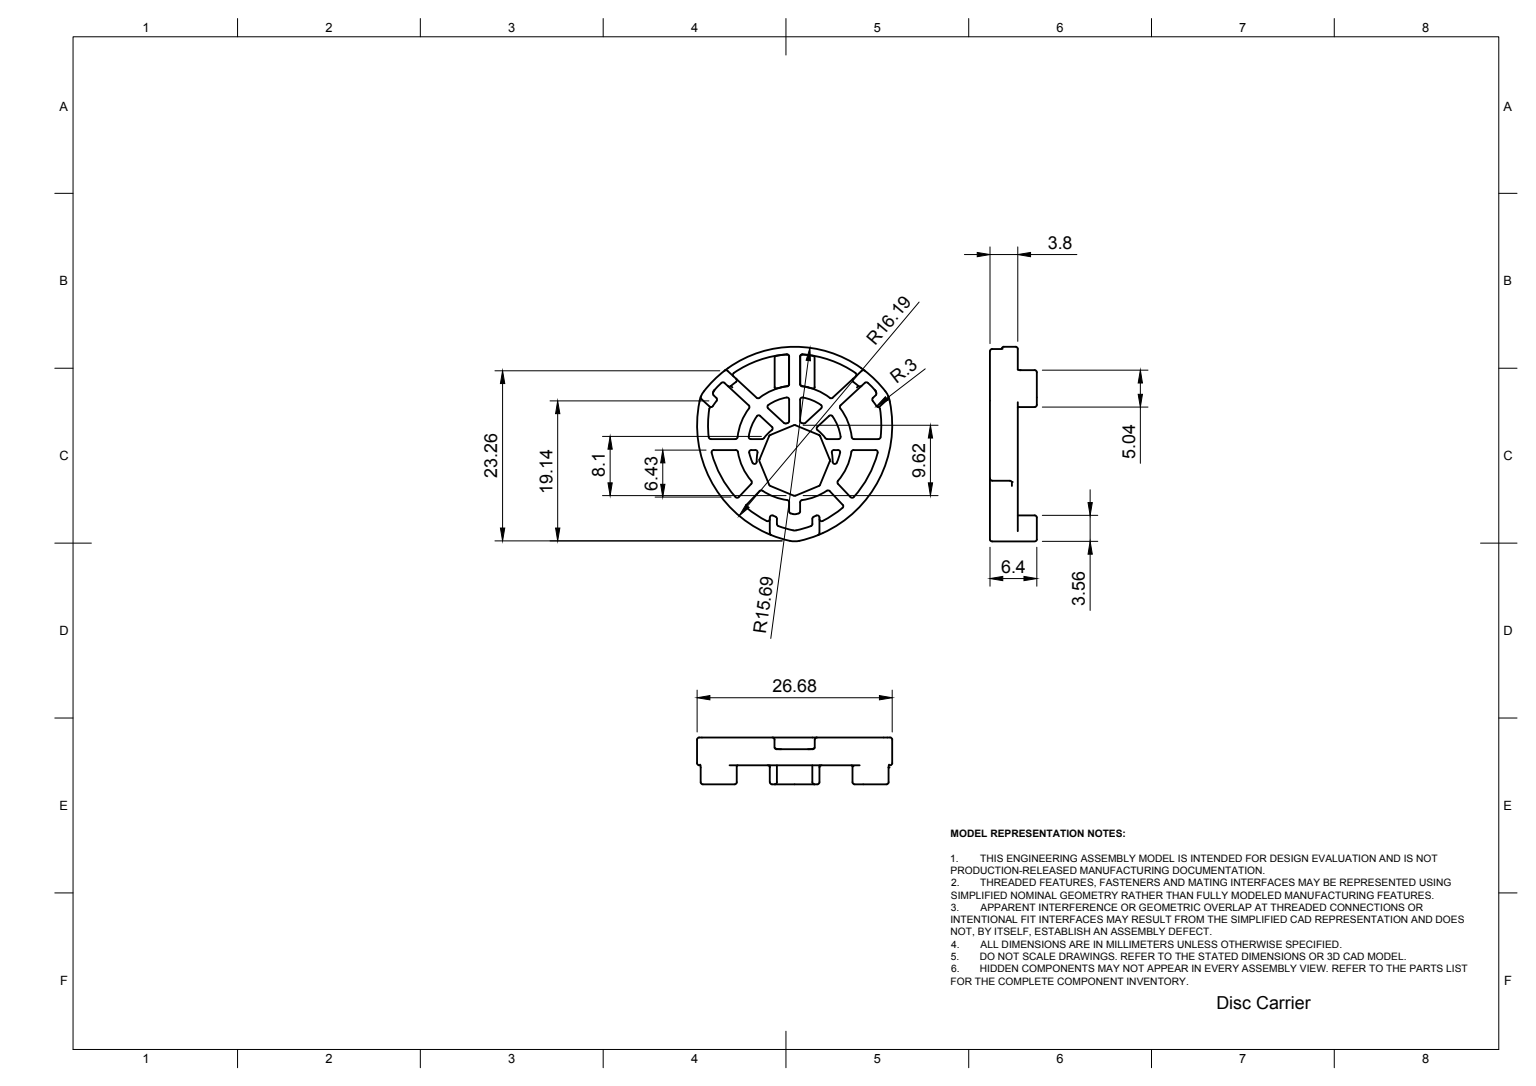
ISO-10303-21;
HEADER;
/* Generated by software containing ST-Developer
 * from STEP Tools, Inc. (www.steptools.com) 
 */

FILE_DESCRIPTION(
/* description */ ('STEP AP214'),
/* implementation_level */ '2;1');

FILE_NAME(
/* name */ 'Disc Carrier.step',
/* time_stamp */ '2026-10-06T00:19:40-07:00',
/* author */ (''),
/* organization */ (''),
/* preprocessor_version */ 'ST-DEVELOPER v20.2',
/* originating_system */ 'Autodesk Translation Framework v15.15.0.0',
/* authorisation */ '');

FILE_SCHEMA (('AUTOMOTIVE_DESIGN { 1 0 10303 214 3 1 1 }'));
ENDSEC;

DATA;
#10=MECHANICAL_DESIGN_GEOMETRIC_PRESENTATION_REPRESENTATION('',(#2070),#98302);
#217=TOROIDAL_SURFACE('',#36633,13.816744254,0.3);
#218=TOROIDAL_SURFACE('',#36640,0.6,0.3);
#219=TOROIDAL_SURFACE('',#36644,14.9875296363,0.3);
#220=TOROIDAL_SURFACE('',#36648,0.6,0.3);
#221=TOROIDAL_SURFACE('',#36651,14.9875296363,0.3);
#222=TOROIDAL_SURFACE('',#36655,0.6,0.3);
#223=TOROIDAL_SURFACE('',#36662,13.816744254,0.3);
#224=TOROIDAL_SURFACE('',#36692,13.9462109523,0.3);
#225=TOROIDAL_SURFACE('',#36699,0.6,0.3);
#226=TOROIDAL_SURFACE('',#36702,14.9875296363,0.3);
#227=TOROIDAL_SURFACE('',#36707,15.8875296363,0.3);
#228=TOROIDAL_SURFACE('',#36711,8.14541841273,0.3);
#229=TOROIDAL_SURFACE('',#36717,14.3875296363,0.3);
#230=TOROIDAL_SURFACE('',#36742,7.54541841273,0.3);
#231=TOROIDAL_SURFACE('',#36753,14.9875296363,0.3);
#232=TOROIDAL_SURFACE('',#36757,0.6,0.3);
#233=TOROIDAL_SURFACE('',#36763,0.6,0.3);
#234=TOROIDAL_SURFACE('',#36765,0.6,0.3);
#235=TOROIDAL_SURFACE('',#36767,0.6,0.3);
#236=TOROIDAL_SURFACE('',#36769,12.2256279976,0.3);
#237=TOROIDAL_SURFACE('',#36775,14.9875296363,0.3);
#238=TOROIDAL_SURFACE('',#36803,15.3875296363,0.3);
#239=TOROIDAL_SURFACE('',#36831,4.89295371933,0.3);
#240=TOROIDAL_SURFACE('',#36836,0.6,0.3);
#241=TOROIDAL_SURFACE('',#36842,0.6,0.3);
#242=TOROIDAL_SURFACE('',#36846,6.64541841273,0.3);
#243=TOROIDAL_SURFACE('',#36850,0.6,0.3);
#244=TOROIDAL_SURFACE('',#36854,0.6,0.3);
#245=TOROIDAL_SURFACE('',#36859,6.64541841273,0.3);
#246=TOROIDAL_SURFACE('',#36866,0.6,0.3);
#247=TOROIDAL_SURFACE('',#36875,4.89295371933,0.3);
#248=TOROIDAL_SURFACE('',#36879,0.6,0.3);
#249=TOROIDAL_SURFACE('',#36883,0.6,0.3);
#250=TOROIDAL_SURFACE('',#36894,4.89295371933,0.3);
#251=TOROIDAL_SURFACE('',#36900,0.6,0.3);
#252=TOROIDAL_SURFACE('',#36906,0.6,0.3);
#253=TOROIDAL_SURFACE('',#36910,6.64541841273,0.3);
#254=TOROIDAL_SURFACE('',#36914,0.6,0.3);
#255=TOROIDAL_SURFACE('',#36918,0.6,0.3);
#256=TOROIDAL_SURFACE('',#36926,6.04541841273,0.3);
#257=TOROIDAL_SURFACE('',#36933,5.49295371933,0.3);
#258=TOROIDAL_SURFACE('',#36946,5.49295371933,0.3);
#259=TOROIDAL_SURFACE('',#36950,0.6,0.3);
#260=TOROIDAL_SURFACE('',#36954,7.54541841273,0.3);
#261=TOROIDAL_SURFACE('',#36958,0.6,0.3);
#262=TOROIDAL_SURFACE('',#36962,0.6,0.3);
#263=TOROIDAL_SURFACE('',#36973,12.8256279976,0.3);
#264=TOROIDAL_SURFACE('',#36978,5.49295371933,0.3);
#265=TOROIDAL_SURFACE('',#36984,15.8875296363,0.3);
#266=TOROIDAL_SURFACE('',#36988,15.3875296363,0.3);
#267=TOROIDAL_SURFACE('',#36993,15.8875296363,0.3);
#268=TOROIDAL_SURFACE('',#36996,0.985778366608,0.3);
#269=TOROIDAL_SURFACE('',#37005,2.7,0.3);
#270=TOROIDAL_SURFACE('',#37007,2.7,0.3);
#271=TOROIDAL_SURFACE('',#37013,15.8875296363,0.3);
#272=TOROIDAL_SURFACE('',#37039,8.14541841273,0.3);
#273=TOROIDAL_SURFACE('',#37053,14.3875296363,0.3);
#274=TOROIDAL_SURFACE('',#37091,6.04541841273,0.3);
#275=TOROIDAL_SURFACE('',#37112,6.04541841273,0.3);
#276=TOROIDAL_SURFACE('',#37118,0.385778366608,0.3);
#277=TOROIDAL_SURFACE('',#37119,0.6,0.3);
#278=TOROIDAL_SURFACE('',#37129,8.14541841273,0.3);
#279=TOROIDAL_SURFACE('',#37134,0.6,0.3);
#280=TOROIDAL_SURFACE('',#37137,13.3462109523,0.3);
#281=TOROIDAL_SURFACE('',#37140,0.6,0.3);
#282=TOROIDAL_SURFACE('',#37149,14.3875296363,0.3);
#283=TOROIDAL_SURFACE('',#37154,14.3875296363,0.3);
#284=TOROIDAL_SURFACE('',#37170,0.6,0.3);
#285=TOROIDAL_SURFACE('',#37173,7.54541841273,0.3);
#286=TOROIDAL_SURFACE('',#37176,0.6,0.3);
#287=TOROIDAL_SURFACE('',#37182,0.6,0.3);
#288=TOROIDAL_SURFACE('',#37185,0.6,0.3);
#289=TOROIDAL_SURFACE('',#37188,14.9875296363,0.3);
#290=TOROIDAL_SURFACE('',#37190,0.6,0.3);
#291=TOROIDAL_SURFACE('',#37193,13.216744254,0.3);
#292=TOROIDAL_SURFACE('',#37205,15.8875296363,0.3);
#293=TOROIDAL_SURFACE('',#37207,1.3,0.3);
#294=TOROIDAL_SURFACE('',#37211,14.9875296363,0.3);
#295=TOROIDAL_SURFACE('',#37215,0.6,0.3);
#296=TOROIDAL_SURFACE('',#37221,0.6,0.3);
#297=TOROIDAL_SURFACE('',#37225,7.54541841273,0.3);
#298=TOROIDAL_SURFACE('',#37229,0.6,0.3);
#299=TOROIDAL_SURFACE('',#37261,14.3875296363,0.3);
#300=TOROIDAL_SURFACE('',#37264,0.7,0.3);
#301=TOROIDAL_SURFACE('',#37270,14.3875296363,0.3);
#302=TOROIDAL_SURFACE('',#37275,14.3875296363,0.3);
#303=TOROIDAL_SURFACE('',#37282,8.14541841273,0.3);
#304=TOROIDAL_SURFACE('',#37289,0.6,0.3);
#305=TOROIDAL_SURFACE('',#37292,13.216744254,0.3);
#306=TOROIDAL_SURFACE('',#37295,0.6,0.3);
#307=TOROIDAL_SURFACE('',#37328,13.816744254,0.3);
#308=TOROIDAL_SURFACE('',#37335,0.6,0.3);
#309=TOROIDAL_SURFACE('',#37339,14.9875296363,0.3);
#310=TOROIDAL_SURFACE('',#37343,0.6,0.3);
#311=TOROIDAL_SURFACE('',#37346,14.9875296363,0.3);
#312=TOROIDAL_SURFACE('',#37350,0.6,0.3);
#313=TOROIDAL_SURFACE('',#37357,13.816744254,0.3);
#314=TOROIDAL_SURFACE('',#37389,13.9462109523,0.3);
#315=TOROIDAL_SURFACE('',#37396,0.6,0.3);
#316=TOROIDAL_SURFACE('',#37400,14.9875296363,0.3);
#317=TOROIDAL_SURFACE('',#37406,15.8875296363,0.3);
#318=TOROIDAL_SURFACE('',#37412,8.14541841273,0.3);
#319=TOROIDAL_SURFACE('',#37417,14.3875296363,0.3);
#320=TOROIDAL_SURFACE('',#37442,7.54541841273,0.3);
#321=TOROIDAL_SURFACE('',#37453,14.9875296363,0.3);
#322=TOROIDAL_SURFACE('',#37457,0.6,0.3);
#323=TOROIDAL_SURFACE('',#37463,0.6,0.3);
#324=TOROIDAL_SURFACE('',#37465,0.6,0.3);
#325=TOROIDAL_SURFACE('',#37467,0.6,0.3);
#326=TOROIDAL_SURFACE('',#37470,12.2256279976,0.3);
#327=TOROIDAL_SURFACE('',#37476,14.9875296363,0.3);
#328=TOROIDAL_SURFACE('',#37511,15.3875296363,0.3);
#329=TOROIDAL_SURFACE('',#37543,4.89295371933,0.3);
#330=TOROIDAL_SURFACE('',#37548,0.6,0.3);
#331=TOROIDAL_SURFACE('',#37554,0.6,0.3);
#332=TOROIDAL_SURFACE('',#37558,6.64541841273,0.3);
#333=TOROIDAL_SURFACE('',#37562,0.6,0.3);
#334=TOROIDAL_SURFACE('',#37566,0.6,0.3);
#335=TOROIDAL_SURFACE('',#37571,6.64541841273,0.3);
#336=TOROIDAL_SURFACE('',#37578,0.6,0.3);
#337=TOROIDAL_SURFACE('',#37586,4.89295371933,0.3);
#338=TOROIDAL_SURFACE('',#37590,0.6,0.3);
#339=TOROIDAL_SURFACE('',#37594,0.6,0.3);
#340=TOROIDAL_SURFACE('',#37605,4.89295371933,0.3);
#341=TOROIDAL_SURFACE('',#37611,0.6,0.3);
#342=TOROIDAL_SURFACE('',#37617,0.6,0.3);
#343=TOROIDAL_SURFACE('',#37621,6.64541841273,0.3);
#344=TOROIDAL_SURFACE('',#37625,0.6,0.3);
#345=TOROIDAL_SURFACE('',#37629,0.6,0.3);
#346=TOROIDAL_SURFACE('',#37637,6.04541841273,0.3);
#347=TOROIDAL_SURFACE('',#37643,5.49295371933,0.3);
#348=TOROIDAL_SURFACE('',#37656,5.49295371933,0.3);
#349=TOROIDAL_SURFACE('',#37659,0.6,0.3);
#350=TOROIDAL_SURFACE('',#37663,7.54541841273,0.3);
#351=TOROIDAL_SURFACE('',#37667,0.6,0.3);
#352=TOROIDAL_SURFACE('',#37671,0.6,0.3);
#353=TOROIDAL_SURFACE('',#37684,12.8256279976,0.3);
#354=TOROIDAL_SURFACE('',#37689,5.49295371933,0.3);
#355=TOROIDAL_SURFACE('',#37696,15.8875296363,0.3);
#356=TOROIDAL_SURFACE('',#37700,15.3875296363,0.3);
#357=TOROIDAL_SURFACE('',#37710,0.4,0.1);
#358=TOROIDAL_SURFACE('',#37715,0.4,0.1);
#359=TOROIDAL_SURFACE('',#37720,0.4,0.1);
#360=TOROIDAL_SURFACE('',#37722,0.4,0.1);
#361=TOROIDAL_SURFACE('',#37727,0.4,0.1);
#362=TOROIDAL_SURFACE('',#37732,0.4,0.1);
#363=TOROIDAL_SURFACE('',#37737,0.4,0.1);
#364=TOROIDAL_SURFACE('',#37742,0.4,0.1);
#365=TOROIDAL_SURFACE('',#37749,15.8875296363,0.3);
#366=TOROIDAL_SURFACE('',#37750,0.985778366608,0.3);
#367=TOROIDAL_SURFACE('',#37759,2.7,0.3);
#368=TOROIDAL_SURFACE('',#37761,2.7,0.3);
#369=TOROIDAL_SURFACE('',#37766,15.8875296363,0.3);
#370=TOROIDAL_SURFACE('',#37779,15.3875296363,0.3);
#371=TOROIDAL_SURFACE('',#37803,8.14541841273,0.3);
#372=TOROIDAL_SURFACE('',#37814,14.3875296363,0.3);
#373=TOROIDAL_SURFACE('',#37850,6.04541841273,0.3);
#374=TOROIDAL_SURFACE('',#37871,6.04541841273,0.3);
#375=TOROIDAL_SURFACE('',#37877,0.385778366608,0.3);
#376=TOROIDAL_SURFACE('',#37878,0.6,0.3);
#377=TOROIDAL_SURFACE('',#37886,8.14541841273,0.3);
#378=TOROIDAL_SURFACE('',#37891,0.6,0.3);
#379=TOROIDAL_SURFACE('',#37894,13.3462109523,0.3);
#380=TOROIDAL_SURFACE('',#37897,0.6,0.3);
#381=TOROIDAL_SURFACE('',#37909,14.3875296363,0.3);
#382=TOROIDAL_SURFACE('',#37914,14.3875296363,0.3);
#383=TOROIDAL_SURFACE('',#37930,0.6,0.3);
#384=TOROIDAL_SURFACE('',#37933,7.54541841273,0.3);
#385=TOROIDAL_SURFACE('',#37936,0.6,0.3);
#386=TOROIDAL_SURFACE('',#37942,0.6,0.3);
#387=TOROIDAL_SURFACE('',#37945,0.6,0.3);
#388=TOROIDAL_SURFACE('',#37948,14.9875296363,0.3);
#389=TOROIDAL_SURFACE('',#37950,0.6,0.3);
#390=TOROIDAL_SURFACE('',#37953,13.216744254,0.3);
#391=TOROIDAL_SURFACE('',#37965,15.8875296363,0.3);
#392=TOROIDAL_SURFACE('',#37967,15.3875296363,0.3);
#393=TOROIDAL_SURFACE('',#37977,0.4,0.1);
#394=TOROIDAL_SURFACE('',#37979,0.4,0.1);
#395=TOROIDAL_SURFACE('',#37984,0.4,0.1);
#396=TOROIDAL_SURFACE('',#37991,0.4,0.1);
#397=TOROIDAL_SURFACE('',#37999,1.3,0.3);
#398=TOROIDAL_SURFACE('',#38003,14.9875296363,0.3);
#399=TOROIDAL_SURFACE('',#38006,0.6,0.3);
#400=TOROIDAL_SURFACE('',#38011,0.6,0.3);
#401=TOROIDAL_SURFACE('',#38014,7.54541841273,0.3);
#402=TOROIDAL_SURFACE('',#38017,0.6,0.3);
#403=TOROIDAL_SURFACE('',#38048,14.3875296363,0.3);
#404=TOROIDAL_SURFACE('',#38051,0.7,0.3);
#405=TOROIDAL_SURFACE('',#38057,14.3875296363,0.3);
#406=TOROIDAL_SURFACE('',#38062,14.3875296363,0.3);
#407=TOROIDAL_SURFACE('',#38071,8.14541841273,0.3);
#408=TOROIDAL_SURFACE('',#38079,0.6,0.3);
#409=TOROIDAL_SURFACE('',#38082,13.216744254,0.3);
#410=TOROIDAL_SURFACE('',#38085,0.6,0.3);
#636=ELLIPSE('',#36609,0.616948377444998,0.596990574629877);
#637=ELLIPSE('',#36774,0.298848892782947,0.2969053606671);
#638=ELLIPSE('',#36784,0.723457342561266,0.612142527579512);
#639=ELLIPSE('',#36787,0.839901750727128,0.325201544662394);
#640=ELLIPSE('',#36791,0.839902765005034,0.32520200920329);
#641=ELLIPSE('',#36792,0.855720879944736,0.334538055133644);
#642=ELLIPSE('',#36796,0.978504400650312,0.43206650732588);
#643=ELLIPSE('',#36807,0.298987522088764,0.297463090341305);
#644=ELLIPSE('',#36864,0.0996163073938246,0.0989684771695573);
#645=ELLIPSE('',#36865,0.0996064607576122,0.098921046723739);
#646=ELLIPSE('',#36870,0.0996019636355457,0.0988979538729398);
#647=ELLIPSE('',#36871,0.83480328877623,0.449020774204173);
#648=ELLIPSE('',#36872,0.0996163010870433,0.0989684579736212);
#649=ELLIPSE('',#36873,0.0996019611035896,0.0988979479073979);
#650=ELLIPSE('',#36874,0.95881614661924,0.545128833125042);
#651=ELLIPSE('',#36888,0.0996019636635876,0.0988979539393061);
#652=ELLIPSE('',#36889,0.834793007766825,0.449012007377356);
#653=ELLIPSE('',#36890,0.0996163011297496,0.0989684580705834);
#654=ELLIPSE('',#36891,0.0996019612880109,0.0988979483606112);
#655=ELLIPSE('',#36892,0.0996163073978892,0.0989684771734698);
#656=ELLIPSE('',#36893,0.842981617008318,0.456043592675208);
#657=ELLIPSE('',#37011,0.298848927783278,0.296905444507015);
#658=ELLIPSE('',#37012,0.299091836143122,0.297812318683333);
#659=ELLIPSE('',#37015,0.299092017159912,0.297812365396506);
#660=ELLIPSE('',#37030,0.298848921977966,0.296905430756493);
#661=ELLIPSE('',#37033,0.358196202460482,0.312309449719818);
#662=ELLIPSE('',#37114,0.299085253265536,0.297791465794382);
#663=ELLIPSE('',#37167,0.298848922572082,0.296905433095193);
#664=ELLIPSE('',#37196,0.48575646188926,0.315209432805966);
#665=ELLIPSE('',#37197,0.298848922223572,0.296905431591445);
#666=ELLIPSE('',#37198,0.298976384440305,0.297423661821599);
#667=ELLIPSE('',#37201,0.298848893179516,0.296905361743558);
#668=ELLIPSE('',#37203,0.298849004322787,0.296905465668005);
#669=ELLIPSE('',#37209,0.299077289129448,0.297765861381808);
#670=ELLIPSE('',#37233,0.2988599234424,0.296955631862372);
#671=ELLIPSE('',#37234,0.311781310291398,0.301461130998388);
#672=ELLIPSE('',#37302,0.616948377444998,0.596990574629877);
#673=ELLIPSE('',#37475,0.298848921980292,0.296905430856554);
#674=ELLIPSE('',#37488,0.723457342561266,0.612142527579512);
#675=ELLIPSE('',#37496,0.855721443648946,0.334538377478706);
#676=ELLIPSE('',#37500,0.839900853126743,0.325201217495182);
#677=ELLIPSE('',#37501,0.855721622372424,0.334538483108095);
#678=ELLIPSE('',#37576,0.0996064588793403,0.0989210426276871);
#679=ELLIPSE('',#37577,0.0996163153029603,0.0989684770999027);
#680=ELLIPSE('',#37582,0.0996163073887366,0.0989684771505584);
#681=ELLIPSE('',#37583,0.842986353714893,0.456047441690848);
#682=ELLIPSE('',#37584,0.0996019612459525,0.0988979482541347);
#683=ELLIPSE('',#37585,0.0996019632515573,0.0988979536268878);
#684=ELLIPSE('',#37599,0.0996163073858426,0.0989684771452112);
#685=ELLIPSE('',#37600,0.84298514231536,0.456046449061635);
#686=ELLIPSE('',#37601,0.0996019612550026,0.0988979482814453);
#687=ELLIPSE('',#37602,0.0996019632510724,0.0988979536158697);
#688=ELLIPSE('',#37603,0.83479393416711,0.449012748427101);
#689=ELLIPSE('',#37604,0.0996163011297535,0.0989684580706061);
#690=ELLIPSE('',#37764,0.299091892234915,0.297812430528943);
#691=ELLIPSE('',#37765,0.298848892822638,0.296905360819338);
#692=ELLIPSE('',#37767,0.298848925852848,0.296905440053724);
#693=ELLIPSE('',#37768,0.299092010660396,0.29781235080905);
#694=ELLIPSE('',#37796,0.358196201537078,0.312309449169694);
#695=ELLIPSE('',#37927,0.298848900003069,0.29690537960284);
#696=ELLIPSE('',#37955,0.298848922307858,0.296905431614744);
#697=ELLIPSE('',#37956,0.298976199239788,0.29742370304314);
#698=ELLIPSE('',#37957,0.298848893194714,0.296905361846251);
#699=ELLIPSE('',#37958,0.48575646188926,0.315209432805966);
#700=ELLIPSE('',#37960,0.298848918312141,0.296905422207127);
#701=ELLIPSE('',#37961,0.298848927446579,0.29690544380809);
#702=ELLIPSE('',#37963,0.298849777080326,0.296906780571315);
#703=ELLIPSE('',#38001,0.299077129594657,0.297765592394515);
#704=ELLIPSE('',#38020,0.311781310291398,0.301461130998388);
#705=ELLIPSE('',#38021,0.2988599234424,0.296955631862372);
#759=SPHERICAL_SURFACE('',#36631,0.3);
#760=SPHERICAL_SURFACE('',#36636,0.3);
#761=SPHERICAL_SURFACE('',#36660,0.3);
#762=SPHERICAL_SURFACE('',#36665,0.3);
#763=SPHERICAL_SURFACE('',#36690,0.3);
#764=SPHERICAL_SURFACE('',#36695,0.3);
#765=SPHERICAL_SURFACE('',#36705,0.3);
#766=SPHERICAL_SURFACE('',#36721,0.3);
#767=SPHERICAL_SURFACE('',#36724,0.3);
#768=SPHERICAL_SURFACE('',#36728,0.3);
#769=SPHERICAL_SURFACE('',#36731,0.3);
#770=SPHERICAL_SURFACE('',#36759,0.3);
#771=SPHERICAL_SURFACE('',#36800,0.3);
#772=SPHERICAL_SURFACE('',#36930,0.3);
#773=SPHERICAL_SURFACE('',#36936,0.3);
#774=SPHERICAL_SURFACE('',#36939,0.3);
#775=SPHERICAL_SURFACE('',#36942,0.3);
#776=SPHERICAL_SURFACE('',#36966,0.3);
#777=SPHERICAL_SURFACE('',#36971,0.3);
#778=SPHERICAL_SURFACE('',#37003,0.3);
#779=SPHERICAL_SURFACE('',#37016,0.3);
#780=SPHERICAL_SURFACE('',#37021,0.3);
#781=SPHERICAL_SURFACE('',#37037,0.3);
#782=SPHERICAL_SURFACE('',#37043,0.3);
#783=SPHERICAL_SURFACE('',#37048,0.3);
#784=SPHERICAL_SURFACE('',#37050,0.3);
#785=SPHERICAL_SURFACE('',#37057,0.3);
#786=SPHERICAL_SURFACE('',#37089,0.3);
#787=SPHERICAL_SURFACE('',#37093,0.3);
#788=SPHERICAL_SURFACE('',#37095,0.3);
#789=SPHERICAL_SURFACE('',#37100,0.3);
#790=SPHERICAL_SURFACE('',#37101,0.3);
#791=SPHERICAL_SURFACE('',#37110,0.3);
#792=SPHERICAL_SURFACE('',#37117,0.3);
#793=SPHERICAL_SURFACE('',#37122,0.3);
#794=SPHERICAL_SURFACE('',#37145,0.3);
#795=SPHERICAL_SURFACE('',#37152,0.3);
#796=SPHERICAL_SURFACE('',#37162,0.3);
#797=SPHERICAL_SURFACE('',#37258,0.3);
#798=SPHERICAL_SURFACE('',#37267,0.3);
#799=SPHERICAL_SURFACE('',#37272,0.3);
#800=SPHERICAL_SURFACE('',#37277,0.3);
#801=SPHERICAL_SURFACE('',#37280,0.3);
#802=SPHERICAL_SURFACE('',#37284,0.3);
#803=SPHERICAL_SURFACE('',#37326,0.3);
#804=SPHERICAL_SURFACE('',#37331,0.3);
#805=SPHERICAL_SURFACE('',#37355,0.3);
#806=SPHERICAL_SURFACE('',#37360,0.3);
#807=SPHERICAL_SURFACE('',#37387,0.3);
#808=SPHERICAL_SURFACE('',#37392,0.3);
#809=SPHERICAL_SURFACE('',#37403,0.3);
#810=SPHERICAL_SURFACE('',#37421,0.3);
#811=SPHERICAL_SURFACE('',#37424,0.3);
#812=SPHERICAL_SURFACE('',#37428,0.3);
#813=SPHERICAL_SURFACE('',#37431,0.3);
#814=SPHERICAL_SURFACE('',#37459,0.3);
#815=SPHERICAL_SURFACE('',#37508,0.3);
#816=SPHERICAL_SURFACE('',#37640,0.3);
#817=SPHERICAL_SURFACE('',#37646,0.3);
#818=SPHERICAL_SURFACE('',#37649,0.3);
#819=SPHERICAL_SURFACE('',#37652,0.3);
#820=SPHERICAL_SURFACE('',#37675,0.3);
#821=SPHERICAL_SURFACE('',#37682,0.3);
#822=SPHERICAL_SURFACE('',#37757,0.3);
#823=SPHERICAL_SURFACE('',#37769,0.3);
#824=SPHERICAL_SURFACE('',#37787,0.3);
#825=SPHERICAL_SURFACE('',#37801,0.3);
#826=SPHERICAL_SURFACE('',#37806,0.3);
#827=SPHERICAL_SURFACE('',#37810,0.3);
#828=SPHERICAL_SURFACE('',#37812,0.3);
#829=SPHERICAL_SURFACE('',#37817,0.3);
#830=SPHERICAL_SURFACE('',#37848,0.3);
#831=SPHERICAL_SURFACE('',#37852,0.3);
#832=SPHERICAL_SURFACE('',#37854,0.3);
#833=SPHERICAL_SURFACE('',#37859,0.3);
#834=SPHERICAL_SURFACE('',#37860,0.3);
#835=SPHERICAL_SURFACE('',#37869,0.3);
#836=SPHERICAL_SURFACE('',#37876,0.3);
#837=SPHERICAL_SURFACE('',#37879,0.3);
#838=SPHERICAL_SURFACE('',#37905,0.3);
#839=SPHERICAL_SURFACE('',#37911,0.3);
#840=SPHERICAL_SURFACE('',#37922,0.3);
#841=SPHERICAL_SURFACE('',#38045,0.3);
#842=SPHERICAL_SURFACE('',#38054,0.3);
#843=SPHERICAL_SURFACE('',#38059,0.3);
#844=SPHERICAL_SURFACE('',#38065,0.3);
#845=SPHERICAL_SURFACE('',#38069,0.3);
#846=SPHERICAL_SURFACE('',#38074,0.3);
#1192=B_SPLINE_SURFACE_WITH_KNOTS('',5,5,((#86287,#86288,#86289,#86290,
#86291,#86292),(#86293,#86294,#86295,#86296,#86297,#86298),(#86299,#86300,
#86301,#86302,#86303,#86304),(#86305,#86306,#86307,#86308,#86309,#86310),
(#86311,#86312,#86313,#86314,#86315,#86316),(#86317,#86318,#86319,#86320,
#86321,#86322),(#86323,#86324,#86325,#86326,#86327,#86328),(#86329,#86330,
#86331,#86332,#86333,#86334),(#86335,#86336,#86337,#86338,#86339,#86340)),
 .UNSPECIFIED.,.F.,.F.,.F.,(6,3,6),(6,6),(1.75158458902,2.2812742412,2.90384942405),
(0.,0.3),.UNSPECIFIED.);
#1193=B_SPLINE_SURFACE_WITH_KNOTS('',5,5,((#86882,#86883,#86884,#86885,
#86886,#86887),(#86888,#86889,#86890,#86891,#86892,#86893),(#86894,#86895,
#86896,#86897,#86898,#86899),(#86900,#86901,#86902,#86903,#86904,#86905),
(#86906,#86907,#86908,#86909,#86910,#86911),(#86912,#86913,#86914,#86915,
#86916,#86917)),.UNSPECIFIED.,.F.,.F.,.F.,(6,6),(6,6),(1.0735101225,1.1089775272),
(0.,0.1),.UNSPECIFIED.);
#1194=B_SPLINE_SURFACE_WITH_KNOTS('',5,5,((#86931,#86932,#86933,#86934,
#86935,#86936),(#86937,#86938,#86939,#86940,#86941,#86942),(#86943,#86944,
#86945,#86946,#86947,#86948),(#86949,#86950,#86951,#86952,#86953,#86954),
(#86955,#86956,#86957,#86958,#86959,#86960),(#86961,#86962,#86963,#86964,
#86965,#86966)),.UNSPECIFIED.,.F.,.F.,.F.,(6,6),(6,6),(1.62703155549,1.68203627825),
(0.,0.1),.UNSPECIFIED.);
#1195=B_SPLINE_SURFACE_WITH_KNOTS('',5,5,((#86972,#86973,#86974,#86975,
#86976,#86977),(#86978,#86979,#86980,#86981,#86982,#86983),(#86984,#86985,
#86986,#86987,#86988,#86989),(#86990,#86991,#86992,#86993,#86994,#86995),
(#86996,#86997,#86998,#86999,#87000,#87001),(#87002,#87003,#87004,#87005,
#87006,#87007)),.UNSPECIFIED.,.F.,.F.,.F.,(6,6),(6,6),(0.205332243373231,
0.603435556801337),(-5.32516463369809E-5,0.1),.UNSPECIFIED.);
#1196=B_SPLINE_SURFACE_WITH_KNOTS('',4,5,((#87038,#87039,#87040,#87041,
#87042,#87043),(#87044,#87045,#87046,#87047,#87048,#87049),(#87050,#87051,
#87052,#87053,#87054,#87055),(#87056,#87057,#87058,#87059,#87060,#87061),
(#87062,#87063,#87064,#87065,#87066,#87067)),.UNSPECIFIED.,.F.,.F.,.F.,
(5,5),(6,6),(2.44731088148,2.46511887948),(0.,0.1),.UNSPECIFIED.);
#1197=B_SPLINE_SURFACE_WITH_KNOTS('',5,5,((#87090,#87091,#87092,#87093,
#87094,#87095),(#87096,#87097,#87098,#87099,#87100,#87101),(#87102,#87103,
#87104,#87105,#87106,#87107),(#87108,#87109,#87110,#87111,#87112,#87113),
(#87114,#87115,#87116,#87117,#87118,#87119),(#87120,#87121,#87122,#87123,
#87124,#87125)),.UNSPECIFIED.,.F.,.F.,.F.,(6,6),(6,6),(1.62703155549,1.68203627825),
(0.,0.1),.UNSPECIFIED.);
#1198=B_SPLINE_SURFACE_WITH_KNOTS('',5,5,((#87131,#87132,#87133,#87134,
#87135,#87136),(#87137,#87138,#87139,#87140,#87141,#87142),(#87143,#87144,
#87145,#87146,#87147,#87148),(#87149,#87150,#87151,#87152,#87153,#87154),
(#87155,#87156,#87157,#87158,#87159,#87160),(#87161,#87162,#87163,#87164,
#87165,#87166)),.UNSPECIFIED.,.F.,.F.,.F.,(6,6),(6,6),(0.205332100976151,
0.60343837439054),(-5.32318455396895E-5,0.1),.UNSPECIFIED.);
#1199=B_SPLINE_SURFACE_WITH_KNOTS('',5,5,((#87197,#87198,#87199,#87200,
#87201,#87202),(#87203,#87204,#87205,#87206,#87207,#87208),(#87209,#87210,
#87211,#87212,#87213,#87214),(#87215,#87216,#87217,#87218,#87219,#87220),
(#87221,#87222,#87223,#87224,#87225,#87226),(#87227,#87228,#87229,#87230,
#87231,#87232)),.UNSPECIFIED.,.F.,.F.,.F.,(6,6),(6,6),(2.44531347319,2.50031756413),
(0.,0.1),.UNSPECIFIED.);
#1200=B_SPLINE_SURFACE_WITH_KNOTS('',5,5,((#88026,#88027,#88028,#88029,
#88030,#88031),(#88032,#88033,#88034,#88035,#88036,#88037),(#88038,#88039,
#88040,#88041,#88042,#88043),(#88044,#88045,#88046,#88047,#88048,#88049),
(#88050,#88051,#88052,#88053,#88054,#88055),(#88056,#88057,#88058,#88059,
#88060,#88061),(#88062,#88063,#88064,#88065,#88066,#88067),(#88068,#88069,
#88070,#88071,#88072,#88073),(#88074,#88075,#88076,#88077,#88078,#88079)),
 .UNSPECIFIED.,.F.,.F.,.F.,(6,3,6),(6,6),(2.86241645295004,3.3764526533,
4.04046842116996),(0.,0.300992369259961),.UNSPECIFIED.);
#1201=B_SPLINE_SURFACE_WITH_KNOTS('',5,5,((#88128,#88129,#88130,#88131,
#88132,#88133),(#88134,#88135,#88136,#88137,#88138,#88139),(#88140,#88141,
#88142,#88143,#88144,#88145),(#88146,#88147,#88148,#88149,#88150,#88151),
(#88152,#88153,#88154,#88155,#88156,#88157),(#88158,#88159,#88160,#88161,
#88162,#88163),(#88164,#88165,#88166,#88167,#88168,#88169),(#88170,#88171,
#88172,#88173,#88174,#88175),(#88176,#88177,#88178,#88179,#88180,#88181)),
 .UNSPECIFIED.,.F.,.F.,.F.,(6,3,6),(6,6),(4.76185240083,5.31344541544,5.93786871511),
(0.,0.3),.UNSPECIFIED.);
#1202=B_SPLINE_SURFACE_WITH_KNOTS('',5,5,((#88250,#88251,#88252,#88253,
#88254,#88255),(#88256,#88257,#88258,#88259,#88260,#88261),(#88262,#88263,
#88264,#88265,#88266,#88267),(#88268,#88269,#88270,#88271,#88272,#88273),
(#88274,#88275,#88276,#88277,#88278,#88279),(#88280,#88281,#88282,#88283,
#88284,#88285),(#88286,#88287,#88288,#88289,#88290,#88291),(#88292,#88293,
#88294,#88295,#88296,#88297),(#88298,#88299,#88300,#88301,#88302,#88303)),
 .UNSPECIFIED.,.F.,.F.,.F.,(6,3,6),(6,6),(1.64208556101,2.12883652195,2.73162696034),
(0.,0.3),.UNSPECIFIED.);
#1203=B_SPLINE_SURFACE_WITH_KNOTS('',5,5,((#88685,#88686,#88687,#88688,
#88689,#88690),(#88691,#88692,#88693,#88694,#88695,#88696),(#88697,#88698,
#88699,#88700,#88701,#88702),(#88703,#88704,#88705,#88706,#88707,#88708),
(#88709,#88710,#88711,#88712,#88713,#88714),(#88715,#88716,#88717,#88718,
#88719,#88720)),.UNSPECIFIED.,.F.,.F.,.F.,(6,6),(6,6),(0.138174465866154,
1.09237668281),(-0.000329517642285316,0.3),.UNSPECIFIED.);
#1204=B_SPLINE_SURFACE_WITH_KNOTS('',5,5,((#88985,#88986,#88987,#88988,
#88989,#88990),(#88991,#88992,#88993,#88994,#88995,#88996),(#88997,#88998,
#88999,#89000,#89001,#89002),(#89003,#89004,#89005,#89006,#89007,#89008),
(#89009,#89010,#89011,#89012,#89013,#89014),(#89015,#89016,#89017,#89018,
#89019,#89020),(#89021,#89022,#89023,#89024,#89025,#89026),(#89027,#89028,
#89029,#89030,#89031,#89032),(#89033,#89034,#89035,#89036,#89037,#89038),
(#89039,#89040,#89041,#89042,#89043,#89044),(#89045,#89046,#89047,#89048,
#89049,#89050),(#89051,#89052,#89053,#89054,#89055,#89056),(#89057,#89058,
#89059,#89060,#89061,#89062),(#89063,#89064,#89065,#89066,#89067,#89068),
(#89069,#89070,#89071,#89072,#89073,#89074),(#89075,#89076,#89077,#89078,
#89079,#89080),(#89081,#89082,#89083,#89084,#89085,#89086),(#89087,#89088,
#89089,#89090,#89091,#89092)),.UNSPECIFIED.,.F.,.F.,.F.,(6,3,3,3,3,6),(6,
6),(0.,0.630653457813,0.794370029612,0.931886828419,1.04715733204,1.10981746796917),
(0.,0.300159997979174),.UNSPECIFIED.);
#1205=B_SPLINE_SURFACE_WITH_KNOTS('',5,5,((#89179,#89180,#89181,#89182,
#89183,#89184),(#89185,#89186,#89187,#89188,#89189,#89190),(#89191,#89192,
#89193,#89194,#89195,#89196),(#89197,#89198,#89199,#89200,#89201,#89202),
(#89203,#89204,#89205,#89206,#89207,#89208),(#89209,#89210,#89211,#89212,
#89213,#89214),(#89215,#89216,#89217,#89218,#89219,#89220),(#89221,#89222,
#89223,#89224,#89225,#89226),(#89227,#89228,#89229,#89230,#89231,#89232)),
 .UNSPECIFIED.,.F.,.F.,.F.,(6,3,6),(6,6),(0.,0.323534265941,0.647068531882),
(0.,0.538062533561),.UNSPECIFIED.);
#1206=B_SPLINE_SURFACE_WITH_KNOTS('',5,5,((#89332,#89333,#89334,#89335,
#89336,#89337),(#89338,#89339,#89340,#89341,#89342,#89343),(#89344,#89345,
#89346,#89347,#89348,#89349),(#89350,#89351,#89352,#89353,#89354,#89355),
(#89356,#89357,#89358,#89359,#89360,#89361),(#89362,#89363,#89364,#89365,
#89366,#89367)),.UNSPECIFIED.,.F.,.F.,.F.,(6,6),(6,6),(2.77894816417,3.04318822375),
(0.,0.3),.UNSPECIFIED.);
#1207=B_SPLINE_SURFACE_WITH_KNOTS('',5,5,((#89373,#89374,#89375,#89376,
#89377,#89378),(#89379,#89380,#89381,#89382,#89383,#89384),(#89385,#89386,
#89387,#89388,#89389,#89390),(#89391,#89392,#89393,#89394,#89395,#89396),
(#89397,#89398,#89399,#89400,#89401,#89402),(#89403,#89404,#89405,#89406,
#89407,#89408),(#89409,#89410,#89411,#89412,#89413,#89414),(#89415,#89416,
#89417,#89418,#89419,#89420),(#89421,#89422,#89423,#89424,#89425,#89426)),
 .UNSPECIFIED.,.F.,.F.,.F.,(6,3,6),(6,6),(1.25405163269,1.6430233414,2.19239180857),
(0.,0.3),.UNSPECIFIED.);
#1208=B_SPLINE_SURFACE_WITH_KNOTS('',5,5,((#89440,#89441,#89442,#89443,
#89444,#89445),(#89446,#89447,#89448,#89449,#89450,#89451),(#89452,#89453,
#89454,#89455,#89456,#89457),(#89458,#89459,#89460,#89461,#89462,#89463),
(#89464,#89465,#89466,#89467,#89468,#89469),(#89470,#89471,#89472,#89473,
#89474,#89475),(#89476,#89477,#89478,#89479,#89480,#89481),(#89482,#89483,
#89484,#89485,#89486,#89487),(#89488,#89489,#89490,#89491,#89492,#89493)),
 .UNSPECIFIED.,.F.,.F.,.F.,(6,3,6),(6,6),(1.69812247662,2.37608580106,2.83469359842),
(0.,0.3),.UNSPECIFIED.);
#1209=B_SPLINE_SURFACE_WITH_KNOTS('',5,5,((#89507,#89508,#89509,#89510,
#89511,#89512),(#89513,#89514,#89515,#89516,#89517,#89518),(#89519,#89520,
#89521,#89522,#89523,#89524),(#89525,#89526,#89527,#89528,#89529,#89530),
(#89531,#89532,#89533,#89534,#89535,#89536),(#89537,#89538,#89539,#89540,
#89541,#89542)),.UNSPECIFIED.,.F.,.F.,.F.,(6,6),(6,6),(1.6338579571,2.7257140478),
(0.,0.3),.UNSPECIFIED.);
#1210=B_SPLINE_SURFACE_WITH_KNOTS('',5,5,((#89651,#89652,#89653,#89654,
#89655,#89656),(#89657,#89658,#89659,#89660,#89661,#89662),(#89663,#89664,
#89665,#89666,#89667,#89668),(#89669,#89670,#89671,#89672,#89673,#89674),
(#89675,#89676,#89677,#89678,#89679,#89680),(#89681,#89682,#89683,#89684,
#89685,#89686),(#89687,#89688,#89689,#89690,#89691,#89692),(#89693,#89694,
#89695,#89696,#89697,#89698),(#89699,#89700,#89701,#89702,#89703,#89704)),
 .UNSPECIFIED.,.F.,.F.,.F.,(6,3,6),(6,6),(1.37442826527,1.83079344184,2.19966814328),
(0.,0.3),.UNSPECIFIED.);
#1211=B_SPLINE_SURFACE_WITH_KNOTS('',5,5,((#89748,#89749,#89750,#89751,
#89752,#89753),(#89754,#89755,#89756,#89757,#89758,#89759),(#89760,#89761,
#89762,#89763,#89764,#89765),(#89766,#89767,#89768,#89769,#89770,#89771),
(#89772,#89773,#89774,#89775,#89776,#89777),(#89778,#89779,#89780,#89781,
#89782,#89783)),.UNSPECIFIED.,.F.,.F.,.F.,(6,6),(6,6),(1.66778051169,1.825176882),
(0.,0.3),.UNSPECIFIED.);
#1212=B_SPLINE_SURFACE_WITH_KNOTS('',5,5,((#89821,#89822,#89823,#89824,
#89825,#89826),(#89827,#89828,#89829,#89830,#89831,#89832),(#89833,#89834,
#89835,#89836,#89837,#89838),(#89839,#89840,#89841,#89842,#89843,#89844),
(#89845,#89846,#89847,#89848,#89849,#89850),(#89851,#89852,#89853,#89854,
#89855,#89856)),.UNSPECIFIED.,.F.,.F.,.F.,(6,6),(6,6),(1.19509008928,1.27929234824),
(0.,0.3),.UNSPECIFIED.);
#1213=B_SPLINE_SURFACE_WITH_KNOTS('',5,5,((#89860,#89861,#89862,#89863,
#89864,#89865),(#89866,#89867,#89868,#89869,#89870,#89871),(#89872,#89873,
#89874,#89875,#89876,#89877),(#89878,#89879,#89880,#89881,#89882,#89883),
(#89884,#89885,#89886,#89887,#89888,#89889),(#89890,#89891,#89892,#89893,
#89894,#89895)),.UNSPECIFIED.,.F.,.F.,.F.,(6,6),(6,6),(0.176101352323,1.24191828283),
(0.,0.3),.UNSPECIFIED.);
#1214=B_SPLINE_SURFACE_WITH_KNOTS('',5,5,((#90678,#90679,#90680,#90681,
#90682,#90683),(#90684,#90685,#90686,#90687,#90688,#90689),(#90690,#90691,
#90692,#90693,#90694,#90695),(#90696,#90697,#90698,#90699,#90700,#90701),
(#90702,#90703,#90704,#90705,#90706,#90707),(#90708,#90709,#90710,#90711,
#90712,#90713)),.UNSPECIFIED.,.F.,.F.,.F.,(6,6),(6,6),(0.,0.788174979856),
(0.,1.),.UNSPECIFIED.);
#1215=B_SPLINE_SURFACE_WITH_KNOTS('',5,5,((#90776,#90777,#90778,#90779,
#90780,#90781),(#90782,#90783,#90784,#90785,#90786,#90787),(#90788,#90789,
#90790,#90791,#90792,#90793),(#90794,#90795,#90796,#90797,#90798,#90799),
(#90800,#90801,#90802,#90803,#90804,#90805),(#90806,#90807,#90808,#90809,
#90810,#90811),(#90812,#90813,#90814,#90815,#90816,#90817),(#90818,#90819,
#90820,#90821,#90822,#90823),(#90824,#90825,#90826,#90827,#90828,#90829),
(#90830,#90831,#90832,#90833,#90834,#90835),(#90836,#90837,#90838,#90839,
#90840,#90841),(#90842,#90843,#90844,#90845,#90846,#90847)),
 .UNSPECIFIED.,.F.,.F.,.F.,(6,3,3,6),(6,6),(0.144241926362,0.436612428829,
0.752300010655,1.24832448076),(0.,3.),.UNSPECIFIED.);
#1216=B_SPLINE_SURFACE_WITH_KNOTS('',5,5,((#91395,#91396,#91397,#91398,
#91399,#91400),(#91401,#91402,#91403,#91404,#91405,#91406),(#91407,#91408,
#91409,#91410,#91411,#91412),(#91413,#91414,#91415,#91416,#91417,#91418),
(#91419,#91420,#91421,#91422,#91423,#91424),(#91425,#91426,#91427,#91428,
#91429,#91430)),.UNSPECIFIED.,.F.,.F.,.F.,(6,6),(6,6),(5.32377368294E-13,
0.720782737349),(0.,1.),.UNSPECIFIED.);
#1217=B_SPLINE_SURFACE_WITH_KNOTS('',5,5,((#91495,#91496,#91497,#91498,
#91499,#91500),(#91501,#91502,#91503,#91504,#91505,#91506),(#91507,#91508,
#91509,#91510,#91511,#91512),(#91513,#91514,#91515,#91516,#91517,#91518),
(#91519,#91520,#91521,#91522,#91523,#91524),(#91525,#91526,#91527,#91528,
#91529,#91530),(#91531,#91532,#91533,#91534,#91535,#91536),(#91537,#91538,
#91539,#91540,#91541,#91542),(#91543,#91544,#91545,#91546,#91547,#91548)),
 .UNSPECIFIED.,.F.,.F.,.F.,(6,3,6),(6,6),(1.75158458902,2.2812742412,2.90384942405),
(0.,0.3),.UNSPECIFIED.);
#1218=B_SPLINE_SURFACE_WITH_KNOTS('',4,5,((#92139,#92140,#92141,#92142,
#92143,#92144),(#92145,#92146,#92147,#92148,#92149,#92150),(#92151,#92152,
#92153,#92154,#92155,#92156),(#92157,#92158,#92159,#92160,#92161,#92162),
(#92163,#92164,#92165,#92166,#92167,#92168)),.UNSPECIFIED.,.F.,.F.,.F.,
(5,5),(6,6),(1.00826496187,1.04373195388),(0.,0.1),.UNSPECIFIED.);
#1219=B_SPLINE_SURFACE_WITH_KNOTS('',5,5,((#92182,#92183,#92184,#92185,
#92186,#92187),(#92188,#92189,#92190,#92191,#92192,#92193),(#92194,#92195,
#92196,#92197,#92198,#92199),(#92200,#92201,#92202,#92203,#92204,#92205),
(#92206,#92207,#92208,#92209,#92210,#92211),(#92212,#92213,#92214,#92215,
#92216,#92217)),.UNSPECIFIED.,.F.,.F.,.F.,(6,6),(6,6),(2.44531347353,2.50031756447),
(0.,0.1),.UNSPECIFIED.);
#1220=B_SPLINE_SURFACE_WITH_KNOTS('',5,5,((#92223,#92224,#92225,#92226,
#92227,#92228),(#92229,#92230,#92231,#92232,#92233,#92234),(#92235,#92236,
#92237,#92238,#92239,#92240),(#92241,#92242,#92243,#92244,#92245,#92246),
(#92247,#92248,#92249,#92250,#92251,#92252),(#92253,#92254,#92255,#92256,
#92257,#92258)),.UNSPECIFIED.,.F.,.F.,.F.,(6,6),(6,6),(0.205331513734207,
0.603439035907376),(-5.33254607926776E-5,0.1),.UNSPECIFIED.);
#1221=B_SPLINE_SURFACE_WITH_KNOTS('',3,5,((#92289,#92290,#92291,#92292,
#92293,#92294),(#92295,#92296,#92297,#92298,#92299,#92300),(#92301,#92302,
#92303,#92304,#92305,#92306),(#92307,#92308,#92309,#92310,#92311,#92312)),
 .UNSPECIFIED.,.F.,.F.,.F.,(4,4),(6,6),(1.66422823568,1.68203627824),(0.,
0.1),.UNSPECIFIED.);
#1222=B_SPLINE_SURFACE_WITH_KNOTS('',5,5,((#92338,#92339,#92340,#92341,
#92342,#92343),(#92344,#92345,#92346,#92347,#92348,#92349),(#92350,#92351,
#92352,#92353,#92354,#92355),(#92356,#92357,#92358,#92359,#92360,#92361),
(#92362,#92363,#92364,#92365,#92366,#92367),(#92368,#92369,#92370,#92371,
#92372,#92373)),.UNSPECIFIED.,.F.,.F.,.F.,(6,6),(6,6),(2.4453134732,2.50031756414),
(0.,0.1),.UNSPECIFIED.);
#1223=B_SPLINE_SURFACE_WITH_KNOTS('',5,5,((#92379,#92380,#92381,#92382,
#92383,#92384),(#92385,#92386,#92387,#92388,#92389,#92390),(#92391,#92392,
#92393,#92394,#92395,#92396),(#92397,#92398,#92399,#92400,#92401,#92402),
(#92403,#92404,#92405,#92406,#92407,#92408),(#92409,#92410,#92411,#92412,
#92413,#92414)),.UNSPECIFIED.,.F.,.F.,.F.,(6,6),(6,6),(0.205331513735948,
0.603439035886987),(-5.3325460052425E-5,0.1),.UNSPECIFIED.);
#1224=B_SPLINE_SURFACE_WITH_KNOTS('',5,5,((#92445,#92446,#92447,#92448,
#92449,#92450),(#92451,#92452,#92453,#92454,#92455,#92456),(#92457,#92458,
#92459,#92460,#92461,#92462),(#92463,#92464,#92465,#92466,#92467,#92468),
(#92469,#92470,#92471,#92472,#92473,#92474),(#92475,#92476,#92477,#92478,
#92479,#92480)),.UNSPECIFIED.,.F.,.F.,.F.,(6,6),(6,6),(1.6270315555,1.68203627826),
(0.,0.1),.UNSPECIFIED.);
#1225=B_SPLINE_SURFACE_WITH_KNOTS('',5,5,((#93064,#93065,#93066,#93067,
#93068,#93069),(#93070,#93071,#93072,#93073,#93074,#93075),(#93076,#93077,
#93078,#93079,#93080,#93081),(#93082,#93083,#93084,#93085,#93086,#93087),
(#93088,#93089,#93090,#93091,#93092,#93093),(#93094,#93095,#93096,#93097,
#93098,#93099)),.UNSPECIFIED.,.F.,.F.,.F.,(6,6),(6,6),(0.,0.833577451733),
(0.,1.),.UNSPECIFIED.);
#1226=B_SPLINE_SURFACE_WITH_KNOTS('',5,5,((#93322,#93323,#93324,#93325,
#93326,#93327),(#93328,#93329,#93330,#93331,#93332,#93333),(#93334,#93335,
#93336,#93337,#93338,#93339),(#93340,#93341,#93342,#93343,#93344,#93345),
(#93346,#93347,#93348,#93349,#93350,#93351),(#93352,#93353,#93354,#93355,
#93356,#93357),(#93358,#93359,#93360,#93361,#93362,#93363),(#93364,#93365,
#93366,#93367,#93368,#93369),(#93370,#93371,#93372,#93373,#93374,#93375),
(#93376,#93377,#93378,#93379,#93380,#93381),(#93382,#93383,#93384,#93385,
#93386,#93387),(#93388,#93389,#93390,#93391,#93392,#93393),(#93394,#93395,
#93396,#93397,#93398,#93399),(#93400,#93401,#93402,#93403,#93404,#93405),
(#93406,#93407,#93408,#93409,#93410,#93411)),.UNSPECIFIED.,.F.,.F.,.F.,
(6,3,3,3,6),(6,6),(0.,0.314441419907,0.663953725274,0.811338767061,1.10181448416),
(0.,3.),.UNSPECIFIED.);
#1227=B_SPLINE_SURFACE_WITH_KNOTS('',5,5,((#93576,#93577,#93578,#93579,
#93580,#93581),(#93582,#93583,#93584,#93585,#93586,#93587),(#93588,#93589,
#93590,#93591,#93592,#93593),(#93594,#93595,#93596,#93597,#93598,#93599),
(#93600,#93601,#93602,#93603,#93604,#93605),(#93606,#93607,#93608,#93609,
#93610,#93611),(#93612,#93613,#93614,#93615,#93616,#93617),(#93618,#93619,
#93620,#93621,#93622,#93623),(#93624,#93625,#93626,#93627,#93628,#93629)),
 .UNSPECIFIED.,.F.,.F.,.F.,(6,3,6),(6,6),(2.86340882221,3.3764526533,4.03947605191),
(0.,0.3),.UNSPECIFIED.);
#1228=B_SPLINE_SURFACE_WITH_KNOTS('',5,5,((#93696,#93697,#93698,#93699,
#93700,#93701),(#93702,#93703,#93704,#93705,#93706,#93707),(#93708,#93709,
#93710,#93711,#93712,#93713),(#93714,#93715,#93716,#93717,#93718,#93719),
(#93720,#93721,#93722,#93723,#93724,#93725),(#93726,#93727,#93728,#93729,
#93730,#93731),(#93732,#93733,#93734,#93735,#93736,#93737),(#93738,#93739,
#93740,#93741,#93742,#93743),(#93744,#93745,#93746,#93747,#93748,#93749)),
 .UNSPECIFIED.,.F.,.F.,.F.,(6,3,6),(6,6),(4.76185240083,5.31344541544,5.93786871511),
(0.,0.3),.UNSPECIFIED.);
#1229=B_SPLINE_SURFACE_WITH_KNOTS('',5,5,((#93875,#93876,#93877,#93878,
#93879,#93880),(#93881,#93882,#93883,#93884,#93885,#93886),(#93887,#93888,
#93889,#93890,#93891,#93892),(#93893,#93894,#93895,#93896,#93897,#93898),
(#93899,#93900,#93901,#93902,#93903,#93904),(#93905,#93906,#93907,#93908,
#93909,#93910),(#93911,#93912,#93913,#93914,#93915,#93916),(#93917,#93918,
#93919,#93920,#93921,#93922),(#93923,#93924,#93925,#93926,#93927,#93928)),
 .UNSPECIFIED.,.F.,.F.,.F.,(6,3,6),(6,6),(1.64208556101,2.12883652195,2.73162696034),
(0.,0.3),.UNSPECIFIED.);
#1230=B_SPLINE_SURFACE_WITH_KNOTS('',5,5,((#94274,#94275,#94276,#94277,
#94278,#94279),(#94280,#94281,#94282,#94283,#94284,#94285),(#94286,#94287,
#94288,#94289,#94290,#94291),(#94292,#94293,#94294,#94295,#94296,#94297),
(#94298,#94299,#94300,#94301,#94302,#94303),(#94304,#94305,#94306,#94307,
#94308,#94309)),.UNSPECIFIED.,.F.,.F.,.F.,(6,6),(6,6),(0.138284020234617,
1.09237668281),(0.,0.300010819481383),.UNSPECIFIED.);
#1231=B_SPLINE_SURFACE_WITH_KNOTS('',4,5,((#94593,#94594,#94595,#94596,
#94597,#94598),(#94599,#94600,#94601,#94602,#94603,#94604),(#94605,#94606,
#94607,#94608,#94609,#94610),(#94611,#94612,#94613,#94614,#94615,#94616),
(#94617,#94618,#94619,#94620,#94621,#94622)),.UNSPECIFIED.,.F.,.F.,.F.,
(5,5),(6,6),(8.31692747129E-16,0.70510501139),(0.,1.),.UNSPECIFIED.);
#1232=B_SPLINE_SURFACE_WITH_KNOTS('',5,5,((#94701,#94702,#94703,#94704,
#94705,#94706),(#94707,#94708,#94709,#94710,#94711,#94712),(#94713,#94714,
#94715,#94716,#94717,#94718),(#94719,#94720,#94721,#94722,#94723,#94724),
(#94725,#94726,#94727,#94728,#94729,#94730),(#94731,#94732,#94733,#94734,
#94735,#94736),(#94737,#94738,#94739,#94740,#94741,#94742),(#94743,#94744,
#94745,#94746,#94747,#94748),(#94749,#94750,#94751,#94752,#94753,#94754),
(#94755,#94756,#94757,#94758,#94759,#94760),(#94761,#94762,#94763,#94764,
#94765,#94766),(#94767,#94768,#94769,#94770,#94771,#94772),(#94773,#94774,
#94775,#94776,#94777,#94778),(#94779,#94780,#94781,#94782,#94783,#94784),
(#94785,#94786,#94787,#94788,#94789,#94790),(#94791,#94792,#94793,#94794,
#94795,#94796),(#94797,#94798,#94799,#94800,#94801,#94802),(#94803,#94804,
#94805,#94806,#94807,#94808)),.UNSPECIFIED.,.F.,.F.,.F.,(6,3,3,3,3,6),(6,
6),(0.,0.630653457813,0.794370029612,0.931886828419,1.04715733204,1.10965746999),
(0.,0.3),.UNSPECIFIED.);
#1233=B_SPLINE_SURFACE_WITH_KNOTS('',5,5,((#94849,#94850,#94851,#94852,
#94853,#94854),(#94855,#94856,#94857,#94858,#94859,#94860),(#94861,#94862,
#94863,#94864,#94865,#94866),(#94867,#94868,#94869,#94870,#94871,#94872),
(#94873,#94874,#94875,#94876,#94877,#94878),(#94879,#94880,#94881,#94882,
#94883,#94884),(#94885,#94886,#94887,#94888,#94889,#94890),(#94891,#94892,
#94893,#94894,#94895,#94896),(#94897,#94898,#94899,#94900,#94901,#94902)),
 .UNSPECIFIED.,.F.,.F.,.F.,(6,3,6),(6,6),(0.,0.323534265941,0.647068531882),
(0.,0.538062533561),.UNSPECIFIED.);
#1234=B_SPLINE_SURFACE_WITH_KNOTS('',5,5,((#94932,#94933,#94934,#94935,
#94936,#94937),(#94938,#94939,#94940,#94941,#94942,#94943),(#94944,#94945,
#94946,#94947,#94948,#94949),(#94950,#94951,#94952,#94953,#94954,#94955),
(#94956,#94957,#94958,#94959,#94960,#94961),(#94962,#94963,#94964,#94965,
#94966,#94967)),.UNSPECIFIED.,.F.,.F.,.F.,(6,6),(6,6),(2.77894816417,3.04318822375),
(0.,0.3),.UNSPECIFIED.);
#1235=B_SPLINE_SURFACE_WITH_KNOTS('',5,5,((#94973,#94974,#94975,#94976,
#94977,#94978),(#94979,#94980,#94981,#94982,#94983,#94984),(#94985,#94986,
#94987,#94988,#94989,#94990),(#94991,#94992,#94993,#94994,#94995,#94996),
(#94997,#94998,#94999,#95000,#95001,#95002),(#95003,#95004,#95005,#95006,
#95007,#95008),(#95009,#95010,#95011,#95012,#95013,#95014),(#95015,#95016,
#95017,#95018,#95019,#95020),(#95021,#95022,#95023,#95024,#95025,#95026)),
 .UNSPECIFIED.,.F.,.F.,.F.,(6,3,6),(6,6),(1.25405163269,1.6430233414,2.19239180857),
(0.,0.3),.UNSPECIFIED.);
#1236=B_SPLINE_SURFACE_WITH_KNOTS('',5,5,((#95059,#95060,#95061,#95062,
#95063,#95064),(#95065,#95066,#95067,#95068,#95069,#95070),(#95071,#95072,
#95073,#95074,#95075,#95076),(#95077,#95078,#95079,#95080,#95081,#95082),
(#95083,#95084,#95085,#95086,#95087,#95088),(#95089,#95090,#95091,#95092,
#95093,#95094),(#95095,#95096,#95097,#95098,#95099,#95100),(#95101,#95102,
#95103,#95104,#95105,#95106),(#95107,#95108,#95109,#95110,#95111,#95112)),
 .UNSPECIFIED.,.F.,.F.,.F.,(6,3,6),(6,6),(1.69812247662,2.37608580106,2.83469359842),
(0.,0.3),.UNSPECIFIED.);
#1237=B_SPLINE_SURFACE_WITH_KNOTS('',5,5,((#95160,#95161,#95162,#95163,
#95164,#95165),(#95166,#95167,#95168,#95169,#95170,#95171),(#95172,#95173,
#95174,#95175,#95176,#95177),(#95178,#95179,#95180,#95181,#95182,#95183),
(#95184,#95185,#95186,#95187,#95188,#95189),(#95190,#95191,#95192,#95193,
#95194,#95195)),.UNSPECIFIED.,.F.,.F.,.F.,(6,6),(6,6),(1.6338579571,2.7257140478),
(0.,0.3),.UNSPECIFIED.);
#1238=B_SPLINE_SURFACE_WITH_KNOTS('',5,5,((#95325,#95326,#95327,#95328,
#95329,#95330),(#95331,#95332,#95333,#95334,#95335,#95336),(#95337,#95338,
#95339,#95340,#95341,#95342),(#95343,#95344,#95345,#95346,#95347,#95348),
(#95349,#95350,#95351,#95352,#95353,#95354),(#95355,#95356,#95357,#95358,
#95359,#95360),(#95361,#95362,#95363,#95364,#95365,#95366),(#95367,#95368,
#95369,#95370,#95371,#95372),(#95373,#95374,#95375,#95376,#95377,#95378)),
 .UNSPECIFIED.,.F.,.F.,.F.,(6,3,6),(6,6),(1.37442826527,1.83079344184,2.19966814328),
(0.,0.3),.UNSPECIFIED.);
#1239=B_SPLINE_SURFACE_WITH_KNOTS('',5,5,((#95504,#95505,#95506,#95507,
#95508,#95509),(#95510,#95511,#95512,#95513,#95514,#95515),(#95516,#95517,
#95518,#95519,#95520,#95521),(#95522,#95523,#95524,#95525,#95526,#95527),
(#95528,#95529,#95530,#95531,#95532,#95533),(#95534,#95535,#95536,#95537,
#95538,#95539)),.UNSPECIFIED.,.F.,.F.,.F.,(6,6),(6,6),(1.66778051169,1.825176882),
(0.,0.3),.UNSPECIFIED.);
#1240=B_SPLINE_SURFACE_WITH_KNOTS('',5,5,((#95565,#95566,#95567,#95568,
#95569,#95570),(#95571,#95572,#95573,#95574,#95575,#95576),(#95577,#95578,
#95579,#95580,#95581,#95582),(#95583,#95584,#95585,#95586,#95587,#95588),
(#95589,#95590,#95591,#95592,#95593,#95594),(#95595,#95596,#95597,#95598,
#95599,#95600)),.UNSPECIFIED.,.F.,.F.,.F.,(6,6),(6,6),(1.19509008928,1.27929234824),
(0.,0.3),.UNSPECIFIED.);
#1241=B_SPLINE_SURFACE_WITH_KNOTS('',5,5,((#95604,#95605,#95606,#95607,
#95608,#95609),(#95610,#95611,#95612,#95613,#95614,#95615),(#95616,#95617,
#95618,#95619,#95620,#95621),(#95622,#95623,#95624,#95625,#95626,#95627),
(#95628,#95629,#95630,#95631,#95632,#95633),(#95634,#95635,#95636,#95637,
#95638,#95639)),.UNSPECIFIED.,.F.,.F.,.F.,(6,6),(6,6),(0.176101352323,1.24191828283),
(0.,0.3),.UNSPECIFIED.);
#1309=FACE_BOUND('',#7201,.T.);
#1310=FACE_BOUND('',#7339,.T.);
#1311=FACE_BOUND('',#7340,.T.);
#1312=FACE_BOUND('',#7341,.T.);
#1313=FACE_BOUND('',#7342,.T.);
#1314=FACE_BOUND('',#7343,.T.);
#1874=B_SPLINE_CURVE_WITH_KNOTS('',5,(#85191,#85192,#85193,#85194,#85195,
#85196,#85197,#85198,#85199,#85200,#85201,#85202,#85203,#85204,#85205,#85206,
#85207,#85208),.UNSPECIFIED.,.F.,.F.,(6,3,3,3,3,6),(0.,0.0563238113023862,
0.160203167534755,0.284130417633147,0.431668352740704,1.),.UNSPECIFIED.);
#1875=B_SPLINE_CURVE_WITH_KNOTS('',3,(#85226,#85227,#85228,#85229,#85230,
#85231,#85232,#85233,#85234,#85235,#85236,#85237,#85238,#85239,#85240,#85241,
#85242,#85243,#85244,#85245,#85246,#85247,#85248,#85249,#85250,#85251,#85252,
#85253,#85254,#85255,#85256,#85257,#85258,#85259,#85260,#85261,#85262,#85263,
#85264,#85265,#85266,#85267,#85268,#85269,#85270,#85271,#85272,#85273,#85274),
 .UNSPECIFIED.,.F.,.F.,(4,3,3,3,3,3,3,3,3,3,3,3,3,3,3,3,4),(0.,0.0625,0.127496488131178,
0.198782619245015,0.25,0.34219327047516,0.429444619020733,0.5,0.567975901527668,
0.632411690271494,0.692807754146875,0.75,0.806943714649852,0.861664292573192,
0.915319845265426,0.967555934138337,1.),.UNSPECIFIED.);
#1876=B_SPLINE_CURVE_WITH_KNOTS('',3,(#85286,#85287,#85288,#85289,#85290,
#85291,#85292,#85293,#85294,#85295,#85296,#85297,#85298,#85299,#85300),
 .UNSPECIFIED.,.F.,.F.,(4,2,2,3,2,2,4),(-0.00622622250198344,-0.00386052358474924,
-0.00164759382340911,0.,0.00161285720621331,0.00376992579683336,0.00622515821920392),
 .UNSPECIFIED.);
#1877=B_SPLINE_CURVE_WITH_KNOTS('',3,(#85334,#85335,#85336,#85337,#85338,
#85339,#85340,#85341,#85342,#85343,#85344,#85345,#85346,#85347,#85348,#85349,
#85350,#85351,#85352,#85353,#85354,#85355,#85356,#85357,#85358,#85359,#85360,
#85361,#85362,#85363,#85364,#85365,#85366,#85367,#85368,#85369,#85370,#85371,
#85372,#85373,#85374,#85375,#85376,#85377,#85378,#85379,#85380,#85381,#85382,
#85383,#85384,#85385,#85386,#85387,#85388),.UNSPECIFIED.,.F.,.F.,(4,3,3,
3,3,3,3,3,3,3,3,3,3,3,3,3,3,3,4),(2.67419613751012E-11,0.0720732721924963,
0.164826904591394,0.250000000000005,0.333767822910639,0.408022771354064,
0.444958736785786,0.468749999999991,0.486035361760652,0.499999999999984,
0.550902044618006,0.620498810264917,0.703215974839016,0.777411981129262,
0.842930292554886,0.899989318083444,0.949994659041722,0.991475269880567,
1.),.UNSPECIFIED.);
#1878=B_SPLINE_CURVE_WITH_KNOTS('',3,(#85403,#85404,#85405,#85406,#85407,
#85408,#85409,#85410,#85411,#85412,#85413,#85414,#85415,#85416,#85417,#85418,
#85419,#85420,#85421,#85422,#85423,#85424,#85425,#85426,#85427,#85428,#85429,
#85430,#85431,#85432,#85433,#85434,#85435,#85436,#85437,#85438,#85439,#85440,
#85441,#85442,#85443,#85444,#85445,#85446,#85447,#85448,#85449,#85450,#85451,
#85452,#85453,#85454),.UNSPECIFIED.,.F.,.F.,(4,3,3,3,3,3,3,3,3,3,3,3,3,
3,3,3,3,4),(0.,0.117683452141709,0.231772170622364,0.250000000000002,0.359974894834341,
0.37499999999999,0.437499999999986,0.468749999999984,0.48313769999903,0.499999999999981,
0.584430981722446,0.667215490861218,0.744913217773219,0.749999999999991,
0.823394141625011,0.894590151515514,0.962832104312354,1.),.UNSPECIFIED.);
#1879=B_SPLINE_CURVE_WITH_KNOTS('',3,(#85511,#85512,#85513,#85514,#85515,
#85516,#85517,#85518,#85519,#85520,#85521,#85522,#85523,#85524,#85525,#85526,
#85527,#85528,#85529,#85530,#85531,#85532,#85533,#85534,#85535,#85536,#85537,
#85538,#85539,#85540,#85541,#85542,#85543,#85544,#85545,#85546,#85547,#85548,
#85549,#85550,#85551,#85552,#85553),.UNSPECIFIED.,.F.,.F.,(4,3,3,3,3,3,
3,3,3,3,3,3,3,3,4),(0.,0.0665912841326879,0.134925436752382,0.20631186892184,
0.249999999999947,0.326272372957872,0.374999999999915,0.437499999999907,
0.468749999999907,0.484929812616762,0.499999999999907,0.610160130828769,
0.730077716451813,0.8574587793753,1.),.UNSPECIFIED.);
#1880=B_SPLINE_CURVE_WITH_KNOTS('',3,(#85570,#85571,#85572,#85573,#85574,
#85575,#85576,#85577,#85578,#85579,#85580,#85581,#85582,#85583,#85584,#85585,
#85586,#85587,#85588,#85589,#85590,#85591,#85592,#85593,#85594,#85595,#85596,
#85597,#85598,#85599,#85600,#85601,#85602,#85603,#85604,#85605,#85606,#85607,
#85608,#85609,#85610,#85611,#85612),.UNSPECIFIED.,.F.,.F.,(4,3,3,3,3,3,
3,3,3,3,3,3,3,3,4),(1.75158458902,1.82585854461461,1.90397349676335,1.93627831766,
2.01926759576981,2.10594778966711,2.14030218981,2.22559412880545,2.2812742412,
2.38564669191982,2.42220846454,2.53792768505673,2.67402562128176,2.83070830556877,
2.90384942405),.UNSPECIFIED.);
#1881=B_SPLINE_CURVE_WITH_KNOTS('',3,(#85645,#85646,#85647,#85648,#85649,
#85650,#85651,#85652,#85653,#85654,#85655,#85656,#85657,#85658,#85659,#85660,
#85661,#85662,#85663,#85664,#85665,#85666,#85667,#85668,#85669,#85670,#85671,
#85672,#85673,#85674,#85675,#85676,#85677,#85678,#85679,#85680,#85681),
 .UNSPECIFIED.,.F.,.F.,(4,3,3,3,3,3,3,3,3,3,3,3,4),(0.,0.0838435767709854,
0.171312435754512,0.25,0.323221763664416,0.398257191635949,0.478149991450796,
0.5,0.613728058543987,0.7328575589571,0.853783659825959,0.974765098059976,
1.),.UNSPECIFIED.);
#1882=B_SPLINE_CURVE_WITH_KNOTS('',5,(#85713,#85714,#85715,#85716,#85717,
#85718),.UNSPECIFIED.,.F.,.F.,(6,6),(0.,1.),.UNSPECIFIED.);
#1883=B_SPLINE_CURVE_WITH_KNOTS('',3,(#85726,#85727,#85728,#85729,#85730,
#85731,#85732,#85733,#85734,#85735,#85736,#85737,#85738,#85739,#85740,#85741,
#85742,#85743,#85744,#85745,#85746,#85747,#85748,#85749,#85750,#85751,#85752,
#85753,#85754,#85755,#85756,#85757,#85758,#85759,#85760,#85761,#85762,#85763,
#85764,#85765,#85766,#85767,#85768,#85769,#85770,#85771,#85772,#85773,#85774,
#85775,#85776,#85777,#85778,#85779,#85780,#85781,#85782,#85783,#85784,#85785,
#85786,#85787,#85788,#85789,#85790,#85791,#85792,#85793,#85794,#85795,#85796,
#85797,#85798,#85799,#85800,#85801,#85802,#85803,#85804,#85805,#85806,#85807,
#85808,#85809,#85810,#85811,#85812,#85813,#85814,#85815,#85816,#85817,#85818,
#85819),.UNSPECIFIED.,.F.,.F.,(4,3,3,3,3,3,3,3,3,3,3,3,3,3,3,3,3,3,3,3,
3,3,3,3,3,3,3,3,3,3,3,4),(0.,0.0748276374910851,0.125000000000074,0.187500000000111,
0.218750000000129,0.250000000000147,0.300925328069866,0.355808241698709,
0.37500000000022,0.429937897165098,0.437500000000255,0.46875000000027,0.484375000000277,
0.492187500000278,0.499376491125885,0.500000000000278,0.575416119571093,
0.625000000000229,0.687500000000202,0.718750000000192,0.731094508404207,
0.734375000000187,0.74218750000018,0.748059577436124,0.750000000000173,
0.777151942597279,0.820855228447611,0.860696859758832,0.905081076278559,
0.952540538139279,0.994179803577402,1.),.UNSPECIFIED.);
#1884=B_SPLINE_CURVE_WITH_KNOTS('',3,(#85827,#85828,#85829,#85830,#85831,
#85832,#85833,#85834,#85835,#85836,#85837,#85838,#85839,#85840,#85841,#85842,
#85843,#85844,#85845,#85846,#85847,#85848,#85849,#85850,#85851,#85852,#85853,
#85854,#85855,#85856,#85857,#85858,#85859,#85860,#85861,#85862,#85863,#85864,
#85865,#85866,#85867,#85868,#85869,#85870,#85871,#85872,#85873,#85874,#85875,
#85876,#85877,#85878,#85879,#85880,#85881,#85882,#85883,#85884,#85885,#85886,
#85887,#85888,#85889,#85890,#85891,#85892,#85893,#85894,#85895,#85896,#85897,
#85898,#85899,#85900,#85901,#85902),.UNSPECIFIED.,.F.,.F.,(4,3,3,3,3,3,
3,3,3,3,3,3,3,3,3,3,3,3,3,3,3,3,3,3,3,4),(0.,0.0240929222738366,0.0491054078753616,
0.0625000000000391,0.088020898963512,0.0937500000000545,0.109375000000062,
0.117187500000066,0.12500000000007,0.175258665507682,0.18750000000008,0.218750000000081,
0.2319234838028,0.245688962683513,0.250000000000082,0.326444716335682,0.375000000000072,
0.437500000000073,0.464386992567282,0.492751176174476,0.500000000000074,
0.592825659779259,0.68928762721816,0.789845932118812,0.894922966059406,
1.),.UNSPECIFIED.);
#1885=B_SPLINE_CURVE_WITH_KNOTS('',3,(#85905,#85906,#85907,#85908,#85909,
#85910,#85911,#85912,#85913,#85914,#85915,#85916,#85917,#85918,#85919,#85920,
#85921,#85922,#85923,#85924,#85925,#85926,#85927,#85928,#85929,#85930,#85931,
#85932,#85933,#85934,#85935,#85936,#85937,#85938,#85939,#85940,#85941,#85942,
#85943,#85944,#85945,#85946,#85947,#85948,#85949,#85950,#85951,#85952,#85953,
#85954,#85955,#85956,#85957,#85958,#85959),.UNSPECIFIED.,.F.,.F.,(4,3,3,
3,3,3,3,3,3,3,3,3,3,3,3,3,3,3,4),(0.,0.0980794130832024,0.195976664920974,
0.250000000000032,0.352035387886095,0.375000000000048,0.437500000000056,
0.465353490760474,0.494109597840485,0.500000000000065,0.57233409034639,
0.641941684786156,0.707653647662655,0.750000000000032,0.812500000000024,
0.87286251821144,0.931708475455832,0.98870050755195,1.),.UNSPECIFIED.);
#1886=B_SPLINE_CURVE_WITH_KNOTS('',3,(#85964,#85965,#85966,#85967,#85968,
#85969,#85970,#85971,#85972,#85973,#85974,#85975,#85976,#85977,#85978,#85979,
#85980,#85981,#85982,#85983,#85984,#85985,#85986,#85987,#85988,#85989,#85990,
#85991,#85992,#85993,#85994,#85995,#85996,#85997,#85998,#85999,#86000,#86001,
#86002,#86003,#86004,#86005,#86006,#86007,#86008,#86009,#86010,#86011,#86012,
#86013,#86014,#86015,#86016,#86017,#86018,#86019,#86020,#86021),
 .UNSPECIFIED.,.F.,.F.,(4,3,3,3,3,3,3,3,3,3,3,3,3,3,3,3,3,3,3,4),(0.,0.099452164972226,
0.198552648607838,0.249999999999997,0.320807489597197,0.390438911073157,
0.456941024049377,0.499999999999994,0.580883873456206,0.624999999999999,
0.687500000000001,0.718750000000002,0.73273662702563,0.747996545880403,
0.750000000000003,0.8052526318332,0.857501453743751,0.907936862272324,0.955604058949788,
1.),.UNSPECIFIED.);
#1887=B_SPLINE_CURVE_WITH_KNOTS('',3,(#86029,#86030,#86031,#86032,#86033,
#86034,#86035,#86036,#86037,#86038,#86039,#86040,#86041,#86042,#86043,#86044,
#86045,#86046,#86047,#86048,#86049,#86050,#86051,#86052,#86053,#86054,#86055,
#86056,#86057,#86058,#86059,#86060,#86061,#86062,#86063,#86064,#86065,#86066,
#86067,#86068,#86069,#86070,#86071,#86072,#86073,#86074),.UNSPECIFIED.,
 .F.,.F.,(4,3,3,3,3,3,3,3,3,3,3,3,3,3,3,4),(0.,0.12308642460795,0.217602621418341,
0.233320563260424,0.330691107811757,0.415188069702116,0.486802780982227,
0.545527895202698,0.591357388167948,0.624286558555176,0.644312028400629,
0.651431743486894,0.746696799313277,0.841963369757472,0.920978246085679,
1.),.UNSPECIFIED.);
#1888=B_SPLINE_CURVE_WITH_KNOTS('',3,(#86082,#86083,#86084,#86085,#86086,
#86087,#86088,#86089,#86090,#86091,#86092,#86093,#86094,#86095,#86096,#86097,
#86098,#86099,#86100,#86101,#86102,#86103,#86104,#86105,#86106,#86107,#86108,
#86109,#86110,#86111,#86112,#86113,#86114,#86115,#86116,#86117,#86118,#86119,
#86120,#86121,#86122,#86123,#86124,#86125,#86126,#86127,#86128,#86129,#86130,
#86131,#86132,#86133,#86134,#86135,#86136,#86137,#86138,#86139,#86140,#86141,
#86142,#86143,#86144,#86145,#86146,#86147,#86148,#86149,#86150,#86151,#86152,
#86153,#86154,#86155,#86156,#86157,#86158,#86159,#86160,#86161,#86162,#86163,
#86164,#86165,#86166,#86167,#86168,#86169,#86170,#86171,#86172,#86173,#86174,
#86175,#86176,#86177,#86178,#86179,#86180,#86181,#86182,#86183,#86184,#86185,
#86186,#86187,#86188,#86189,#86190),.UNSPECIFIED.,.F.,.F.,(4,3,3,3,3,3,
3,3,3,3,3,3,3,3,3,3,3,3,3,3,3,3,3,3,3,3,3,3,3,3,3,3,3,3,3,3,4),(0.,0.0355919704945219,
0.0625000000000467,0.0937500000000701,0.109375000000085,0.117187500000093,
0.124095624449358,0.125000000000101,0.147837211789802,0.179510913752234,
0.187500000000158,0.212407992374527,0.218750000000188,0.234375000000198,
0.242558143933212,0.250000000000209,0.29895865159147,0.312500000000223,
0.343750000000233,0.358265386399709,0.372173812649809,0.375000000000243,
0.396581328937065,0.421228179308561,0.43750000000025,0.468750000000241,
0.482453344550044,0.496856148402139,0.500000000000232,0.618014487413222,
0.625000000000166,0.667542699814932,0.711630271843116,0.750000000000099,
0.849282816651991,0.949069247991813,1.),.UNSPECIFIED.);
#1889=B_SPLINE_CURVE_WITH_KNOTS('',5,(#86275,#86276,#86277,#86278,#86279,
#86280),.UNSPECIFIED.,.F.,.F.,(6,6),(0.,1.),.UNSPECIFIED.);
#1890=B_SPLINE_CURVE_WITH_KNOTS('',5,(#86342,#86343,#86344,#86345,#86346,
#86347),.UNSPECIFIED.,.F.,.F.,(6,6),(0.,1.),.UNSPECIFIED.);
#1891=B_SPLINE_CURVE_WITH_KNOTS('',3,(#86350,#86351,#86352,#86353,#86354,
#86355,#86356,#86357,#86358,#86359,#86360,#86361,#86362,#86363,#86364,#86365,
#86366,#86367,#86368,#86369,#86370,#86371,#86372,#86373,#86374,#86375,#86376,
#86377,#86378,#86379,#86380,#86381,#86382,#86383,#86384,#86385,#86386,#86387,
#86388,#86389,#86390,#86391,#86392,#86393,#86394,#86395,#86396,#86397,#86398,
#86399,#86400,#86401,#86402,#86403,#86404,#86405,#86406,#86407,#86408,#86409,
#86410,#86411,#86412,#86413,#86414,#86415,#86416,#86417,#86418,#86419,#86420,
#86421,#86422,#86423,#86424,#86425),.UNSPECIFIED.,.F.,.F.,(4,3,3,3,3,3,
3,3,3,3,3,3,3,3,3,3,3,3,3,3,3,3,3,3,3,4),(0.,0.0979906433443701,0.199916167668728,
0.24999999999997,0.34212271718657,0.374999999999957,0.437499999999956,0.464543924780552,
0.468749999999952,0.483028853555349,0.498667542585192,0.499999999999948,
0.584290236907723,0.624999999999926,0.687499999999915,0.718749999999904,
0.734374999999899,0.742187499999895,0.748091694014882,0.749999999999891,
0.80006377933794,0.850047834503455,0.898722268222934,0.94559281701662,0.989236405049239,
1.),.UNSPECIFIED.);
#1892=B_SPLINE_CURVE_WITH_KNOTS('',3,(#86448,#86449,#86450,#86451,#86452,
#86453,#86454,#86455,#86456,#86457,#86458,#86459,#86460,#86461,#86462,#86463,
#86464,#86465,#86466,#86467,#86468,#86469,#86470,#86471,#86472,#86473,#86474,
#86475,#86476,#86477,#86478,#86479,#86480,#86481,#86482,#86483,#86484,#86485,
#86486,#86487,#86488,#86489,#86490,#86491,#86492,#86493,#86494,#86495,#86496,
#86497,#86498,#86499,#86500,#86501,#86502,#86503,#86504,#86505),
 .UNSPECIFIED.,.F.,.F.,(4,3,3,3,3,3,3,3,3,3,3,3,3,3,3,3,3,3,3,4),(2.86340882221,
2.96038236608017,2.9912183572,3.08700311846,3.18278787972,3.27460804500358,
3.3634673030912,3.3764526533,3.45865940729474,3.54085709160535,3.57484410128,
3.65773122998381,3.67917202515,3.75805208465002,3.78350088337,3.86115067208,
3.93423338613357,3.93880046079,4.01498217619638,4.03947605191),
 .UNSPECIFIED.);
#1893=B_SPLINE_CURVE_WITH_KNOTS('',3,(#86509,#86510,#86511,#86512,#86513,
#86514,#86515,#86516,#86517,#86518,#86519,#86520,#86521,#86522,#86523,#86524,
#86525,#86526,#86527,#86528,#86529,#86530,#86531,#86532,#86533,#86534,#86535,
#86536,#86537,#86538,#86539,#86540,#86541,#86542,#86543,#86544,#86545,#86546,
#86547,#86548,#86549,#86550,#86551,#86552,#86553,#86554,#86555,#86556,#86557,
#86558,#86559,#86560,#86561,#86562,#86563,#86564,#86565,#86566),
 .UNSPECIFIED.,.F.,.F.,(4,3,3,3,3,3,3,3,3,3,3,3,3,3,3,3,3,3,3,4),(4.76185240083,
4.83763310355387,4.8511070755,4.9237368026632,4.94035737066,5.01616912552097,
5.04125309343,5.11983939701062,5.14214350511,5.21975609722012,5.29603838282238,
5.31344541544,5.40219520324995,5.47351631749,5.56538841319371,5.65858597861109,
5.75320413758695,5.78071175361,5.87661154462981,5.93786871511),
 .UNSPECIFIED.);
#1894=B_SPLINE_CURVE_WITH_KNOTS('',3,(#86577,#86578,#86579,#86580,#86581,
#86582,#86583,#86584,#86585,#86586,#86587,#86588,#86589,#86590,#86591,#86592,
#86593,#86594,#86595,#86596,#86597,#86598,#86599,#86600,#86601,#86602,#86603,
#86604,#86605,#86606,#86607,#86608,#86609,#86610,#86611,#86612,#86613,#86614,
#86615,#86616),.UNSPECIFIED.,.F.,.F.,(4,3,3,3,3,3,3,3,3,3,3,3,3,4),(1.69812247662,
1.82517827643346,1.94835352449351,2.04354239572,2.1493981491557,2.2504202018726,
2.34618007075805,2.37608580106,2.46390218046495,2.55211800019734,2.6379844451379,
2.6897944832,2.77017696446133,2.83469359842),.UNSPECIFIED.);
#1895=B_SPLINE_CURVE_WITH_KNOTS('',3,(#86634,#86635,#86636,#86637,#86638,
#86639,#86640,#86641,#86642,#86643,#86644,#86645,#86646,#86647,#86648,#86649,
#86650,#86651,#86652,#86653,#86654,#86655,#86656,#86657,#86658,#86659,#86660,
#86661,#86662,#86663,#86664,#86665,#86666,#86667,#86668,#86669,#86670,#86671,
#86672,#86673),.UNSPECIFIED.,.F.,.F.,(4,3,3,3,3,3,3,3,3,3,3,3,3,4),(9.16642701788228E-11,
0.0777685045691623,0.155298490954937,0.235788513859965,0.249999999999996,
0.374999999999999,0.425782059261454,0.476666286858019,0.492264924606089,
0.500315380842036,0.647629842965568,0.788859013702841,0.917371668501292,
1.),.UNSPECIFIED.);
#1896=B_SPLINE_CURVE_WITH_KNOTS('',3,(#86689,#86690,#86691,#86692,#86693,
#86694,#86695,#86696,#86697,#86698,#86699,#86700,#86701,#86702,#86703,#86704,
#86705,#86706,#86707,#86708,#86709,#86710,#86711,#86712,#86713,#86714,#86715,
#86716,#86717,#86718,#86719,#86720,#86721,#86722,#86723,#86724,#86725,#86726,
#86727,#86728),.UNSPECIFIED.,.F.,.F.,(4,3,3,3,3,3,3,3,3,3,3,3,3,4),(0.,
0.0777737453085021,0.155308734732268,0.235802705737845,0.250000000000003,
0.375000000000003,0.425780378411465,0.476662994638966,0.49226568581941,
0.500315400257842,0.647633193305892,0.788863146805967,0.917372111358519,
1.),.UNSPECIFIED.);
#1897=B_SPLINE_CURVE_WITH_KNOTS('',5,(#86737,#86738,#86739,#86740,#86741,
#86742),.UNSPECIFIED.,.F.,.F.,(6,6),(-1.1089775272,-1.0735101225),
 .UNSPECIFIED.);
#1898=B_SPLINE_CURVE_WITH_KNOTS('',5,(#86802,#86803,#86804,#86805,#86806,
#86807),.UNSPECIFIED.,.F.,.F.,(6,6),(0.,1.),.UNSPECIFIED.);
#1899=B_SPLINE_CURVE_WITH_KNOTS('',3,(#86921,#86922,#86923,#86924),
 .UNSPECIFIED.,.F.,.F.,(4,4),(-1.1089775272,-1.07351012327562),
 .UNSPECIFIED.);
#1900=B_SPLINE_CURVE_WITH_KNOTS('',3,(#87010,#87011,#87012,#87013,#87014,
#87015,#87016,#87017,#87018,#87019,#87020,#87021,#87022,#87023,#87024,#87025,
#87026,#87027,#87028,#87029,#87030,#87031,#87032,#87033,#87034,#87035,#87036,
#87037),.UNSPECIFIED.,.F.,.F.,(4,3,3,3,3,3,3,3,3,4),(1.39576967731014E-10,
0.1505103555998,0.288268426485318,0.376933003975363,0.503523155116763,0.532699752981522,
0.664316984007422,0.802626544765739,0.950088550067854,1.),.UNSPECIFIED.);
#1901=B_SPLINE_CURVE_WITH_KNOTS('',3,(#87169,#87170,#87171,#87172,#87173,
#87174,#87175,#87176,#87177,#87178,#87179,#87180,#87181,#87182,#87183,#87184,
#87185,#87186,#87187,#87188,#87189,#87190,#87191,#87192,#87193,#87194,#87195,
#87196),.UNSPECIFIED.,.F.,.F.,(4,3,3,3,3,3,3,3,3,4),(3.99334178330209E-9,
0.150506684297317,0.288263057281987,0.376930108117779,0.503520614101364,
0.532697581088335,0.664314707972964,0.802621307209367,0.950075916205342,
1.),.UNSPECIFIED.);
#1902=B_SPLINE_CURVE_WITH_KNOTS('',3,(#87293,#87294,#87295,#87296,#87297,
#87298,#87299,#87300,#87301,#87302,#87303,#87304,#87305,#87306,#87307,#87308,
#87309,#87310,#87311,#87312,#87313,#87314,#87315,#87316,#87317,#87318,#87319,
#87320,#87321,#87322,#87323,#87324,#87325,#87326,#87327,#87328,#87329,#87330,
#87331,#87332,#87333,#87334,#87335,#87336,#87337,#87338,#87339,#87340,#87341,
#87342,#87343,#87344,#87345,#87346,#87347,#87348,#87349,#87350,#87351,#87352,
#87353,#87354,#87355,#87356,#87357,#87358,#87359,#87360,#87361,#87362,#87363,
#87364,#87365,#87366,#87367,#87368,#87369,#87370,#87371),.UNSPECIFIED.,
 .F.,.F.,(4,3,3,3,3,3,3,3,3,3,3,3,3,3,3,3,3,3,3,3,3,3,3,3,3,3,4),(0.,0.0355362144885678,
0.0624999999999996,0.0937499999999993,0.107276596424941,0.120331439252964,
0.124999999999999,0.163762141652132,0.203173805928779,0.244559237814547,
0.249999999999999,0.325460882975541,0.375,0.415174481039151,0.457587240519576,
0.497815749000596,0.5,0.552880648155298,0.608960672555796,0.625,0.675510724434953,
0.724578356810552,0.750000000000001,0.809241727425364,0.871851356636048,
0.935925678318024,1.),.UNSPECIFIED.);
#1903=B_SPLINE_CURVE_WITH_KNOTS('',3,(#87376,#87377,#87378,#87379,#87380,
#87381,#87382,#87383,#87384,#87385,#87386,#87387,#87388,#87389,#87390,#87391,
#87392,#87393,#87394,#87395,#87396,#87397,#87398,#87399,#87400,#87401,#87402,
#87403,#87404,#87405,#87406,#87407,#87408,#87409,#87410,#87411,#87412,#87413,
#87414,#87415,#87416,#87417,#87418,#87419,#87420,#87421,#87422,#87423,#87424,
#87425,#87426,#87427,#87428,#87429,#87430,#87431,#87432,#87433,#87434,#87435,
#87436),.UNSPECIFIED.,.F.,.F.,(4,3,3,3,3,3,3,3,3,3,3,3,3,3,3,3,3,3,3,3,
4),(0.,0.124999999999991,0.242509431927007,0.249999999999983,0.364359301276675,
0.374999999999985,0.422328004362009,0.469735704085969,0.499999999999987,
0.585785621366277,0.624999999999989,0.687499999999998,0.718749999999998,
0.732488337520169,0.74772746595688,0.749999999999999,0.812499999999999,
0.869532237334179,0.924605486450739,0.976916884333088,1.),.UNSPECIFIED.);
#1904=B_SPLINE_CURVE_WITH_KNOTS('',3,(#87443,#87444,#87445,#87446,#87447,
#87448,#87449,#87450,#87451,#87452,#87453,#87454,#87455,#87456,#87457,#87458,
#87459,#87460,#87461,#87462,#87463,#87464,#87465,#87466,#87467,#87468,#87469,
#87470,#87471,#87472,#87473,#87474,#87475,#87476,#87477,#87478,#87479,#87480,
#87481,#87482,#87483,#87484,#87485,#87486,#87487,#87488,#87489,#87490,#87491,
#87492,#87493,#87494,#87495,#87496,#87497,#87498,#87499,#87500,#87501,#87502,
#87503,#87504,#87505,#87506,#87507,#87508,#87509,#87510,#87511,#87512,#87513,
#87514,#87515,#87516,#87517,#87518,#87519,#87520,#87521,#87522,#87523,#87524,
#87525,#87526,#87527,#87528,#87529,#87530,#87531,#87532,#87533,#87534,#87535,
#87536,#87537,#87538,#87539,#87540,#87541,#87542),.UNSPECIFIED.,.F.,.F.,
(4,3,3,3,3,3,3,3,3,3,3,3,3,3,3,3,3,3,3,3,3,3,3,3,3,3,3,3,3,3,3,3,3,4),(0.,
0.0958472142403171,0.183853112222453,0.249999999999939,0.374999999999948,
0.437499999999953,0.469467566143704,0.49837783867004,0.499999999999958,
0.5841637537743,0.624999999999968,0.687499999999974,0.718749999999991,0.734374999999999,
0.744227145958902,0.750000000000008,0.78820713890752,0.812499999999997,
0.843749999999993,0.859374999999992,0.867187499999991,0.87441427028628,
0.87499999999999,0.896435606631704,0.906249999999993,0.921874999999993,
0.929687499999994,0.933825830539164,0.937499999999995,0.951631947114754,
0.965077849015114,0.978069978143163,0.990363804263242,1.),.UNSPECIFIED.);
#1905=B_SPLINE_CURVE_WITH_KNOTS('',3,(#87555,#87556,#87557,#87558,#87559,
#87560,#87561,#87562,#87563,#87564,#87565,#87566,#87567,#87568,#87569,#87570,
#87571,#87572,#87573,#87574,#87575,#87576,#87577,#87578,#87579,#87580,#87581,
#87582,#87583,#87584,#87585,#87586,#87587,#87588,#87589,#87590,#87591,#87592,
#87593,#87594,#87595,#87596,#87597,#87598,#87599,#87600,#87601,#87602,#87603,
#87604,#87605,#87606,#87607,#87608,#87609,#87610,#87611,#87612,#87613,#87614,
#87615,#87616,#87617,#87618,#87619,#87620,#87621,#87622,#87623,#87624,#87625,
#87626,#87627),.UNSPECIFIED.,.F.,.F.,(4,3,3,3,3,3,3,3,3,3,3,3,3,3,3,3,3,
3,3,3,3,3,3,3,4),(0.,0.0966099788589137,0.125000000000007,0.17130877196425,
0.215592241170992,0.250000000000015,0.361544036934436,0.375000000000022,
0.437500000000026,0.465511784233522,0.492096554438188,0.50000000000003,
0.57608153399594,0.62500000000002,0.687500000000008,0.718750000000006,0.733471387992378,
0.749161313096158,0.750000000000005,0.799727105623058,0.849795329217294,
0.894862691334285,0.93837411729665,0.979784735280439,1.),.UNSPECIFIED.);
#1906=B_SPLINE_CURVE_WITH_KNOTS('',3,(#87689,#87690,#87691,#87692,#87693,
#87694,#87695,#87696,#87697,#87698,#87699,#87700,#87701,#87702,#87703,#87704,
#87705,#87706,#87707,#87708,#87709,#87710,#87711,#87712,#87713,#87714,#87715,
#87716,#87717,#87718),.UNSPECIFIED.,.F.,.F.,(4,2,2,1,1,2,2,2,1,1,2,2,2,
1,1,2,2,4),(0.,0.124999999999985,0.187499999999977,0.218749999999974,0.234374999999974,
0.242187499999973,0.249999999999972,0.374999999999976,0.437499999999979,
0.468749999999981,0.484374999999981,0.499999999999982,0.624999999999999,
0.687500000000007,0.718750000000012,0.734375000000014,0.750000000000015,
1.),.UNSPECIFIED.);
#1907=B_SPLINE_CURVE_WITH_KNOTS('',5,(#87719,#87720,#87721,#87722,#87723,
#87724),.UNSPECIFIED.,.F.,.F.,(6,6),(0.,1.),.UNSPECIFIED.);
#1908=B_SPLINE_CURVE_WITH_KNOTS('',3,(#87738,#87739,#87740,#87741,#87742,
#87743,#87744,#87745,#87746,#87747,#87748,#87749,#87750,#87751,#87752,#87753,
#87754,#87755,#87756,#87757,#87758,#87759,#87760,#87761,#87762,#87763,#87764,
#87765,#87766,#87767,#87768,#87769,#87770,#87771,#87772,#87773,#87774,#87775,
#87776,#87777,#87778,#87779,#87780,#87781,#87782,#87783,#87784,#87785,#87786,
#87787,#87788,#87789,#87790,#87791,#87792,#87793,#87794,#87795),
 .UNSPECIFIED.,.F.,.F.,(4,3,3,3,3,3,3,3,3,3,3,3,3,3,3,3,3,3,3,4),(0.,0.100609639419896,
0.200720123081653,0.249999999999981,0.32470459539465,0.398051288913321,
0.468246679183588,0.499999999999963,0.581413825455905,0.624999999999953,
0.687499999999949,0.718749999999946,0.732699964043024,0.747947399939569,
0.749999999999944,0.805776737616528,0.858544229418813,0.909482024872923,
0.9576486572329,1.),.UNSPECIFIED.);
#1909=B_SPLINE_CURVE_WITH_KNOTS('',3,(#87819,#87820,#87821,#87822,#87823,
#87824,#87825,#87826,#87827,#87828,#87829,#87830,#87831,#87832,#87833,#87834,
#87835,#87836,#87837,#87838,#87839,#87840,#87841,#87842,#87843,#87844,#87845,
#87846,#87847,#87848,#87849,#87850,#87851,#87852,#87853,#87854,#87855,#87856,
#87857,#87858,#87859,#87860,#87861,#87862,#87863,#87864,#87865,#87866,#87867,
#87868,#87869,#87870,#87871,#87872,#87873,#87874,#87875,#87876,#87877,#87878,
#87879,#87880,#87881,#87882,#87883,#87884,#87885,#87886,#87887,#87888,#87889,
#87890,#87891,#87892,#87893,#87894,#87895,#87896,#87897,#87898,#87899,#87900,
#87901,#87902,#87903,#87904,#87905,#87906,#87907,#87908,#87909),
 .UNSPECIFIED.,.F.,.F.,(4,3,3,3,3,3,3,3,3,3,3,3,3,3,3,3,3,3,3,3,3,3,3,3,
3,3,3,3,3,3,4),(0.,0.0397814237123525,0.0877360660119328,0.124999999999976,
0.165730845336603,0.187499999999964,0.218749999999958,0.234374999999955,
0.242187499999953,0.247641935945892,0.249999999999951,0.267411966703376,
0.322992096802285,0.374999999999974,0.411075296464987,0.437499999999989,
0.468749999999994,0.484374999999995,0.492187499999993,0.498855130311395,
0.499999999999992,0.567142758786176,0.624999999999997,0.687499999999998,
0.718742348599412,0.723042232423563,0.749999999999999,0.817189597240934,
0.893554069690658,0.97480672873194,1.),.UNSPECIFIED.);
#1910=B_SPLINE_CURVE_WITH_KNOTS('',3,(#87915,#87916,#87917,#87918,#87919,
#87920,#87921,#87922,#87923,#87924,#87925,#87926,#87927,#87928,#87929,#87930,
#87931,#87932,#87933,#87934,#87935,#87936,#87937,#87938,#87939,#87940,#87941,
#87942,#87943,#87944,#87945,#87946,#87947,#87948,#87949,#87950,#87951,#87952,
#87953,#87954,#87955,#87956,#87957,#87958,#87959,#87960,#87961,#87962,#87963,
#87964,#87965,#87966,#87967,#87968,#87969,#87970,#87971,#87972),
 .UNSPECIFIED.,.F.,.F.,(4,3,3,3,3,3,3,3,3,3,3,3,3,3,3,3,3,3,3,4),(0.,0.0356451281179679,
0.0693279121910458,0.100412016848408,0.125000000000114,0.161875456310924,
0.187500000000171,0.2187500000002,0.234375000000204,0.243649194272616,0.250000000000208,
0.30872348200964,0.371020762472332,0.437204595886178,0.500000000000135,
0.5983757256371,0.703843588454204,0.81350499211572,0.93003274416397,1.),
 .UNSPECIFIED.);
#1911=B_SPLINE_CURVE_WITH_KNOTS('',3,(#87992,#87993,#87994,#87995,#87996,
#87997,#87998,#87999,#88000,#88001,#88002,#88003,#88004,#88005,#88006,#88007,
#88008,#88009,#88010,#88011,#88012,#88013,#88014,#88015,#88016,#88017,#88018,
#88019,#88020,#88021,#88022,#88023,#88024,#88025),.UNSPECIFIED.,.F.,.F.,
(4,3,3,3,3,3,3,3,3,3,3,4),(1.25405163269,1.32643264163,1.4055803165725,
1.48574465294545,1.56752327448427,1.6430233414,1.72858124378027,1.81406569145,
1.90733041601598,1.99715560017,2.09477370437,2.19239180857),
 .UNSPECIFIED.);
#1912=B_SPLINE_CURVE_WITH_KNOTS('',3,(#88081,#88082,#88083,#88084,#88085,
#88086,#88087,#88088,#88089,#88090,#88091,#88092,#88093,#88094,#88095,#88096,
#88097,#88098,#88099,#88100,#88101,#88102,#88103,#88104,#88105,#88106,#88107,
#88108,#88109,#88110,#88111,#88112,#88113,#88114,#88115,#88116,#88117,#88118,
#88119,#88120,#88121,#88122,#88123),.UNSPECIFIED.,.F.,.F.,(4,3,3,3,3,3,
3,3,3,3,3,3,3,3,4),(4.39679769916515E-10,0.0896494939985405,0.177741271167206,
0.265221869705284,0.352748440567542,0.43623682229533,0.506707219508413,
0.574976714664183,0.643034716691638,0.710667694098751,0.77742624196382,
0.842035244579551,0.905067000126942,0.965268347329118,1.),.UNSPECIFIED.);
#1913=B_SPLINE_CURVE_WITH_KNOTS('',3,(#88183,#88184,#88185,#88186,#88187,
#88188,#88189,#88190,#88191,#88192,#88193,#88194,#88195,#88196,#88197,#88198,
#88199,#88200,#88201,#88202,#88203,#88204,#88205,#88206,#88207,#88208,#88209,
#88210,#88211,#88212,#88213,#88214,#88215,#88216,#88217,#88218,#88219,#88220,
#88221,#88222),.UNSPECIFIED.,.F.,.F.,(4,3,3,3,3,3,3,3,3,3,3,3,3,4),(0.,
0.0586293965389953,0.118458772750461,0.181450715788032,0.248647653214792,
0.323992525315228,0.399761183556369,0.469035172311963,0.559603022429232,
0.654066796784159,0.752582807186012,0.8505413511493,0.944145001536187,1.),
 .UNSPECIFIED.);
#1914=B_SPLINE_CURVE_WITH_KNOTS('',5,(#88305,#88306,#88307,#88308,#88309,
#88310,#88311,#88312,#88313),.UNSPECIFIED.,.F.,.F.,(6,3,6),(0.,0.446748477147653,
1.),.UNSPECIFIED.);
#1915=B_SPLINE_CURVE_WITH_KNOTS('',3,(#88316,#88317,#88318,#88319,#88320,
#88321,#88322,#88323,#88324,#88325,#88326,#88327,#88328,#88329,#88330,#88331,
#88332,#88333,#88334,#88335,#88336,#88337,#88338,#88339,#88340,#88341,#88342,
#88343,#88344,#88345,#88346,#88347,#88348,#88349,#88350,#88351,#88352,#88353,
#88354,#88355),.UNSPECIFIED.,.F.,.F.,(4,3,3,3,3,3,3,3,3,3,3,3,3,4),(1.81673175559521E-10,
0.0836057555609339,0.174429967985735,0.268968220557755,0.366735443263493,
0.446902605260138,0.500000000000001,0.597735980402653,0.707686006743452,
0.75,0.824579319188729,0.899060478571651,0.971802328054873,1.),
 .UNSPECIFIED.);
#1916=B_SPLINE_CURVE_WITH_KNOTS('',3,(#88364,#88365,#88366,#88367,#88368,
#88369,#88370,#88371,#88372,#88373,#88374,#88375,#88376,#88377,#88378,#88379,
#88380,#88381,#88382,#88383,#88384,#88385,#88386),.UNSPECIFIED.,.F.,.F.,
(4,2,2,2,3,2,2,2,2,2,4),(0.223210461888191,0.223397147217863,0.223717290566587,
0.224391037089802,0.228125629041838,0.234943871134553,0.243585952736414,
0.25309083829967,0.263261316553702,0.27431000560614,0.277820240597038),
 .UNSPECIFIED.);
#1917=B_SPLINE_CURVE_WITH_KNOTS('',3,(#88401,#88402,#88403,#88404,#88405,
#88406,#88407,#88408,#88409,#88410,#88411,#88412,#88413,#88414,#88415,#88416),
 .UNSPECIFIED.,.F.,.F.,(4,2,2,2,2,2,2,4),(0.0329698156679733,0.0333695174810278,
0.0386982857933801,0.0439884179233323,0.0499284327972441,0.0577713467846448,
0.0633464558735427,0.0721131672795402),.UNSPECIFIED.);
#1918=B_SPLINE_CURVE_WITH_KNOTS('',3,(#88418,#88419,#88420,#88421,#88422,
#88423,#88424,#88425,#88426,#88427),.UNSPECIFIED.,.F.,.F.,(4,2,2,2,4),(0.271351380209749,
0.293031113526595,0.302969887271488,0.308596889767683,0.311849694512603),
 .UNSPECIFIED.);
#1919=B_SPLINE_CURVE_WITH_KNOTS('',3,(#88520,#88521,#88522,#88523,#88524,
#88525,#88526,#88527,#88528,#88529,#88530,#88531,#88532,#88533,#88534,#88535,
#88536,#88537,#88538,#88539,#88540,#88541,#88542,#88543,#88544,#88545,#88546,
#88547,#88548,#88549,#88550,#88551,#88552,#88553,#88554,#88555,#88556,#88557,
#88558,#88559,#88560,#88561,#88562,#88563,#88564,#88565,#88566,#88567,#88568,
#88569,#88570,#88571,#88572,#88573,#88574,#88575,#88576,#88577),
 .UNSPECIFIED.,.F.,.F.,(4,3,3,3,3,3,3,3,3,3,3,3,3,3,3,3,3,3,3,4),(0.,0.0897308056971427,
0.179444739745368,0.250000000000193,0.336421147132234,0.375000000000287,
0.437500000000334,0.468750000000357,0.484375000000361,0.493366966257959,
0.500000000000365,0.607568988871737,0.625000000000288,0.687500000000249,
0.714210713960481,0.742118754756523,0.750000000000211,0.864717251909047,
0.990112105797021,1.),.UNSPECIFIED.);
#1920=B_SPLINE_CURVE_WITH_KNOTS('',3,(#88604,#88605,#88606,#88607,#88608,
#88609,#88610,#88611,#88612,#88613,#88614,#88615,#88616,#88617,#88618,#88619,
#88620,#88621,#88622,#88623,#88624,#88625,#88626,#88627,#88628,#88629,#88630,
#88631,#88632,#88633,#88634,#88635,#88636,#88637,#88638,#88639,#88640,#88641,
#88642,#88643,#88644,#88645,#88646,#88647,#88648,#88649,#88650,#88651,#88652,
#88653,#88654,#88655,#88656,#88657,#88658,#88659,#88660,#88661,#88662,#88663,
#88664,#88665,#88666,#88667,#88668,#88669,#88670,#88671,#88672,#88673,#88674,
#88675,#88676,#88677,#88678,#88679,#88680,#88681,#88682),.UNSPECIFIED.,
 .F.,.F.,(4,3,3,3,3,3,3,3,3,3,3,3,3,3,3,3,3,3,3,3,3,3,3,3,3,3,4),(0.,0.0355771815476919,
0.0624999999999976,0.0937499999999986,0.10728274018591,0.120341032646476,
0.125,0.16393206809617,0.203518656130192,0.245075225467878,0.250000000000004,
0.32548942661256,0.375000000000008,0.415134282467528,0.45756714123377,0.497745693090781,
0.500000000000012,0.552904193134679,0.60901082343741,0.625000000000016,
0.675540464737087,0.72463970904679,0.75000000000002,0.809244134152876,0.871848389017905,
0.935924194508953,1.),.UNSPECIFIED.);
#1921=B_SPLINE_CURVE_WITH_KNOTS('',3,(#88721,#88722,#88723,#88724,#88725,
#88726,#88727,#88728,#88729,#88730,#88731,#88732,#88733,#88734,#88735,#88736,
#88737,#88738,#88739,#88740,#88741,#88742,#88743,#88744,#88745,#88746,#88747,
#88748,#88749,#88750,#88751,#88752,#88753,#88754,#88755,#88756,#88757,#88758,
#88759,#88760,#88761,#88762,#88763,#88764,#88765,#88766,#88767,#88768,#88769),
 .UNSPECIFIED.,.F.,.F.,(4,3,3,3,3,3,3,3,3,3,3,3,3,3,3,3,4),(0.,0.0648620446179728,
0.132474572992778,0.205862839558522,0.25,0.336375995977143,0.420555151483361,
0.5,0.569903495187839,0.636422109127358,0.69901012047123,0.75,0.80922275929286,
0.866139446326761,0.921929236615715,0.976271344364284,1.),.UNSPECIFIED.);
#1922=B_SPLINE_CURVE_WITH_KNOTS('',3,(#88771,#88772,#88773,#88774,#88775,
#88776,#88777,#88778,#88779,#88780,#88781,#88782,#88783,#88784,#88785,#88786,
#88787,#88788,#88789,#88790,#88791,#88792,#88793,#88794,#88795,#88796,#88797,
#88798,#88799,#88800,#88801,#88802,#88803,#88804,#88805,#88806,#88807,#88808,
#88809,#88810,#88811,#88812,#88813,#88814,#88815,#88816,#88817,#88818,#88819,
#88820,#88821,#88822),.UNSPECIFIED.,.F.,.F.,(4,3,3,3,3,3,3,3,3,3,3,3,3,
3,3,3,3,4),(0.,0.0899334399923707,0.179889344622198,0.250000000000184,0.33993343999114,
0.375000000000275,0.437500000000322,0.468750000000345,0.484375000000349,
0.493754678879357,0.500000000000354,0.625000000000273,0.687500000000233,
0.716107443505401,0.746125713318513,0.750000000000193,0.922212000166891,
1.),.UNSPECIFIED.);
#1923=B_SPLINE_CURVE_WITH_KNOTS('',3,(#88877,#88878,#88879,#88880,#88881,
#88882,#88883,#88884,#88885,#88886,#88887,#88888,#88889,#88890,#88891,#88892,
#88893,#88894,#88895,#88896,#88897,#88898,#88899,#88900,#88901,#88902,#88903,
#88904,#88905,#88906,#88907,#88908,#88909,#88910,#88911,#88912,#88913,#88914,
#88915,#88916,#88917,#88918,#88919,#88920,#88921,#88922,#88923,#88924,#88925,
#88926,#88927,#88928,#88929,#88930,#88931,#88932,#88933,#88934,#88935,#88936,
#88937,#88938,#88939,#88940,#88941,#88942,#88943,#88944,#88945,#88946,#88947,
#88948,#88949,#88950,#88951,#88952),.UNSPECIFIED.,.F.,.F.,(4,3,3,3,3,3,
3,3,3,3,3,3,3,3,3,3,3,3,3,3,3,3,3,3,3,4),(0.,0.0242541900995737,0.0494242354737045,
0.0625000000000132,0.0881719402073255,0.0937500000000197,0.109375000000023,
0.117187500000025,0.125000000000026,0.175610976137408,0.18750000000002,
0.218750000000019,0.232039870493069,0.245916517104364,0.250000000000018,
0.326620952260722,0.375000000000008,0.437500000000007,0.464652777920398,
0.493263921870045,0.500000000000005,0.592910275330305,0.68947296384216,
0.79016606190966,0.89508303095483,1.),.UNSPECIFIED.);
#1924=B_SPLINE_CURVE_WITH_KNOTS('',4,(#88961,#88962,#88963,#88964,#88965),
 .UNSPECIFIED.,.F.,.F.,(5,5),(0.,1.),.UNSPECIFIED.);
#1925=B_SPLINE_CURVE_WITH_KNOTS('',3,(#89095,#89096,#89097,#89098,#89099,
#89100,#89101,#89102,#89103,#89104,#89105,#89106,#89107,#89108,#89109,#89110,
#89111,#89112,#89113,#89114,#89115,#89116,#89117,#89118,#89119,#89120,#89121,
#89122,#89123,#89124,#89125,#89126,#89127,#89128,#89129,#89130,#89131,#89132,
#89133,#89134,#89135,#89136,#89137,#89138,#89139,#89140,#89141,#89142,#89143,
#89144,#89145,#89146,#89147,#89148,#89149,#89150,#89151,#89152,#89153,#89154,
#89155,#89156,#89157,#89158),.UNSPECIFIED.,.F.,.F.,(4,3,3,3,3,3,3,3,3,3,
3,3,3,3,3,3,3,3,3,3,3,4),(0.,0.0770514482651851,0.124999999999956,0.187499999999936,
0.218749999999927,0.234374999999922,0.242981604744465,0.249999999999918,
0.349959099836821,0.374999999999869,0.437499999999847,0.468749999999839,
0.484374999999837,0.492187499999836,0.49913066454904,0.499999999999836,
0.599155572574395,0.699366679430796,0.788911175184783,0.875447489871574,
0.957947680405176,1.),.UNSPECIFIED.);
#1926=B_SPLINE_CURVE_WITH_KNOTS('',3,(#89235,#89236,#89237,#89238,#89239,
#89240,#89241,#89242,#89243,#89244,#89245,#89246,#89247,#89248,#89249,#89250,
#89251,#89252,#89253,#89254,#89255,#89256,#89257,#89258,#89259,#89260,#89261,
#89262,#89263,#89264,#89265,#89266,#89267,#89268,#89269,#89270,#89271,#89272,
#89273,#89274,#89275,#89276,#89277,#89278,#89279,#89280,#89281,#89282,#89283,
#89284,#89285,#89286,#89287,#89288,#89289,#89290,#89291,#89292,#89293,#89294,
#89295,#89296,#89297,#89298,#89299,#89300,#89301,#89302,#89303,#89304,#89305,
#89306,#89307,#89308,#89309,#89310,#89311,#89312,#89313),.UNSPECIFIED.,
 .F.,.F.,(4,3,3,3,3,3,3,3,3,3,3,3,3,3,3,3,3,3,3,3,3,3,3,3,3,3,4),(0.,0.0229442921754058,
0.0473003732270936,0.0624999999999992,0.124999999999998,0.201744637631312,
0.249999999999976,0.273460893851431,0.298548973900594,0.312499999999973,
0.37499999999997,0.458890962622535,0.499232024585504,0.499999999999961,
0.525549380903742,0.551794820739131,0.562499999999962,0.624999999999963,
0.687812610496059,0.749999999999973,0.772533298335757,0.796386956349032,
0.809112771577217,0.815844489583874,0.907922244791937,0.984801127701866,
1.),.UNSPECIFIED.);
#1927=B_SPLINE_CURVE_WITH_KNOTS('',5,(#89427,#89428,#89429,#89430,#89431,
#89432,#89433,#89434,#89435),.UNSPECIFIED.,.F.,.F.,(6,3,6),(0.,0.414531657823574,
1.),.UNSPECIFIED.);
#1928=B_SPLINE_CURVE_WITH_KNOTS('',5,(#89495,#89496,#89497,#89498,#89499,
#89500,#89501,#89502,#89503),.UNSPECIFIED.,.F.,.F.,(6,3,6),(0.,0.596498812468772,
1.),.UNSPECIFIED.);
#1929=B_SPLINE_CURVE_WITH_KNOTS('',3,(#89544,#89545,#89546,#89547,#89548,
#89549,#89550,#89551,#89552,#89553,#89554,#89555,#89556,#89557,#89558,#89559,
#89560,#89561,#89562,#89563,#89564,#89565,#89566,#89567,#89568,#89569,#89570,
#89571,#89572,#89573,#89574),.UNSPECIFIED.,.F.,.F.,(4,3,3,3,3,3,3,3,3,3,
4),(0.,0.113410126173201,0.231212941658119,0.348973287565832,0.464312568640331,
0.575973606578693,0.68198020493402,0.784775801213408,0.884955399662714,
0.981955778398047,1.),.UNSPECIFIED.);
#1930=B_SPLINE_CURVE_WITH_KNOTS('',3,(#89576,#89577,#89578,#89579,#89580,
#89581,#89582,#89583,#89584,#89585,#89586,#89587,#89588,#89589,#89590,#89591,
#89592,#89593,#89594,#89595,#89596,#89597,#89598,#89599,#89600,#89601,#89602,
#89603,#89604,#89605,#89606,#89607,#89608,#89609,#89610,#89611,#89612,#89613,
#89614,#89615,#89616,#89617,#89618,#89619,#89620,#89621),.UNSPECIFIED.,
 .F.,.F.,(4,3,3,3,3,3,3,3,3,3,3,3,3,3,3,4),(0.,0.0726706660714167,0.146103743511138,
0.220234233777271,0.294302581364791,0.36741929699253,0.43789481134854,0.499999999999996,
0.562499999999997,0.624791030327762,0.68739551516388,0.749999999999998,
0.819280964853742,0.888670436886782,0.956283877925322,1.),.UNSPECIFIED.);
#1931=B_SPLINE_CURVE_WITH_KNOTS('',3,(#89629,#89630,#89631,#89632,#89633,
#89634,#89635,#89636,#89637,#89638),.UNSPECIFIED.,.F.,.F.,(4,3,3,4),(0.,
0.1405201788765,0.24888377189969,0.281040357753),.UNSPECIFIED.);
#1932=B_SPLINE_CURVE_WITH_KNOTS('',3,(#89640,#89641,#89642,#89643,#89644,
#89645,#89646,#89647,#89648,#89649),.UNSPECIFIED.,.F.,.F.,(4,3,3,4),(0.,
0.143504699996,0.239445459249327,0.287009399992),.UNSPECIFIED.);
#1933=B_SPLINE_CURVE_WITH_KNOTS('',5,(#89708,#89709,#89710,#89711,#89712,
#89713,#89714,#89715,#89716),.UNSPECIFIED.,.F.,.F.,(6,3,6),(0.,0.446990882614049,
1.),.UNSPECIFIED.);
#1934=B_SPLINE_CURVE_WITH_KNOTS('',3,(#89717,#89718,#89719,#89720,#89721,
#89722,#89723,#89724,#89725,#89726,#89727,#89728,#89729,#89730,#89731,#89732,
#89733,#89734,#89735,#89736,#89737,#89738,#89739,#89740,#89741,#89742,#89743,
#89744,#89745,#89746,#89747),.UNSPECIFIED.,.F.,.F.,(4,3,3,3,3,3,3,3,3,3,
4),(0.,0.103606039248823,0.209200414240004,0.317311627182045,0.426434884947521,
0.535929191910951,0.645077668364686,0.752572851887125,0.858664995979,0.962443523493216,
0.99999999982195),.UNSPECIFIED.);
#1935=B_SPLINE_CURVE_WITH_KNOTS('',3,(#89896,#89897,#89898,#89899,#89900,
#89901,#89902,#89903,#89904,#89905,#89906,#89907,#89908,#89909,#89910,#89911,
#89912,#89913,#89914,#89915,#89916,#89917,#89918,#89919,#89920,#89921,#89922,
#89923,#89924,#89925,#89926,#89927,#89928,#89929,#89930,#89931,#89932,#89933,
#89934,#89935,#89936,#89937,#89938,#89939,#89940,#89941,#89942,#89943,#89944,
#89945,#89946,#89947,#89948,#89949,#89950,#89951,#89952,#89953,#89954,#89955,
#89956,#89957,#89958,#89959),.UNSPECIFIED.,.F.,.F.,(4,3,3,3,3,3,3,3,3,3,
3,3,3,3,3,3,3,3,3,3,3,4),(0.,0.0373481272818948,0.0788425197254873,0.126446182104601,
0.184791907568511,0.249999999999852,0.345027571690437,0.37499999999978,
0.437499999999744,0.46874999999973,0.484374999999732,0.492187499999735,
0.496093749999737,0.499999999999739,0.558498464864831,0.635836688781905,
0.709773405775254,0.774182065715002,0.837817143450719,0.903585214268584,
0.976677578999226,1.),.UNSPECIFIED.);
#1936=B_SPLINE_CURVE_WITH_KNOTS('',3,(#90034,#90035,#90036,#90037,#90038,
#90039,#90040,#90041,#90042,#90043,#90044,#90045,#90046,#90047,#90048,#90049,
#90050,#90051,#90052,#90053,#90054,#90055,#90056,#90057,#90058,#90059,#90060,
#90061,#90062,#90063,#90064,#90065,#90066,#90067,#90068,#90069,#90070,#90071,
#90072,#90073,#90074,#90075,#90076,#90077,#90078,#90079,#90080,#90081,#90082,
#90083,#90084,#90085,#90086,#90087,#90088),.UNSPECIFIED.,.F.,.F.,(4,3,3,
3,3,3,3,3,3,3,3,3,3,3,3,3,3,3,4),(0.,0.098399225567126,0.19657706045254,
0.249999999999997,0.352225838661693,0.374999999999982,0.437499999999986,
0.465071769090119,0.493567955054625,0.499999999999991,0.572560372932883,
0.642387385962301,0.708319172777275,0.749999999999995,0.812499999999996,
0.873077503807693,0.932131369198034,0.989328858099031,1.),.UNSPECIFIED.);
#1937=B_SPLINE_CURVE_WITH_KNOTS('',3,(#90094,#90095,#90096,#90097,#90098,
#90099,#90100,#90101,#90102,#90103,#90104,#90105,#90106,#90107,#90108,#90109,
#90110,#90111,#90112,#90113,#90114,#90115,#90116,#90117,#90118,#90119,#90120,
#90121,#90122,#90123,#90124,#90125,#90126,#90127,#90128,#90129,#90130,#90131,
#90132,#90133,#90134,#90135,#90136,#90137,#90138,#90139,#90140,#90141,#90142,
#90143,#90144,#90145,#90146,#90147,#90148),.UNSPECIFIED.,.F.,.F.,(4,3,3,
3,3,3,3,3,3,3,3,3,3,3,3,3,3,3,4),(0.,0.0982911914765156,0.196374277996715,
0.249999999999955,0.352161291291609,0.374999999999919,0.437499999999913,
0.46516384899836,0.49374496091657,0.499999999999907,0.572485440727802,0.642240217270967,
0.708099740992737,0.749999999999953,0.812499999999965,0.873008011417871,
0.931994642694371,0.989124166280261,1.),.UNSPECIFIED.);
#1938=B_SPLINE_CURVE_WITH_KNOTS('',3,(#90154,#90155,#90156,#90157,#90158,
#90159,#90160,#90161,#90162,#90163,#90164,#90165,#90166,#90167,#90168,#90169,
#90170,#90171,#90172,#90173,#90174,#90175,#90176,#90177,#90178,#90179,#90180,
#90181,#90182,#90183,#90184,#90185,#90186,#90187,#90188,#90189,#90190,#90191,
#90192,#90193,#90194,#90195,#90196,#90197,#90198,#90199,#90200,#90201,#90202,
#90203,#90204,#90205,#90206,#90207,#90208),.UNSPECIFIED.,.F.,.F.,(4,3,3,
3,3,3,3,3,3,3,3,3,3,3,3,3,3,3,4),(0.,0.0979870042878743,0.195803163964628,
0.250000000000044,0.35198064201211,0.375000000000053,0.437500000000046,
0.465440224692129,0.49427640578226,0.500000000000039,0.572265990346262,
0.641807673307847,0.707452286294341,0.750000000000019,0.812500000000015,
0.872799047234052,0.931582772210694,0.988509432123743,1.),.UNSPECIFIED.);
#1939=B_SPLINE_CURVE_WITH_KNOTS('',3,(#90238,#90239,#90240,#90241,#90242,
#90243,#90244,#90245,#90246,#90247,#90248,#90249,#90250,#90251,#90252,#90253,
#90254,#90255,#90256,#90257,#90258,#90259,#90260,#90261,#90262,#90263,#90264,
#90265,#90266,#90267,#90268,#90269,#90270,#90271,#90272,#90273,#90274,#90275,
#90276,#90277,#90278,#90279,#90280,#90281,#90282,#90283,#90284,#90285,#90286,
#90287,#90288,#90289,#90290,#90291,#90292,#90293,#90294,#90295,#90296,#90297,
#90298,#90299,#90300,#90301),.UNSPECIFIED.,.F.,.F.,(4,3,3,3,3,3,3,3,3,3,
3,3,3,3,3,3,3,3,3,3,3,4),(0.,0.0770564969196051,0.125000000000011,0.187500000000016,
0.218750000000018,0.23437500000002,0.242979652755323,0.250000000000023,
0.349688054350686,0.37500000000004,0.437500000000054,0.468750000000063,
0.484375000000066,0.492187500000072,0.499123753949107,0.500000000000079,
0.599066518850846,0.694261407782884,0.783895704985616,0.870510325616442,
0.953023907192251,1.),.UNSPECIFIED.);
#1940=B_SPLINE_CURVE_WITH_KNOTS('',3,(#90315,#90316,#90317,#90318,#90319,
#90320,#90321,#90322,#90323,#90324,#90325,#90326,#90327,#90328,#90329,#90330,
#90331,#90332,#90333,#90334,#90335,#90336,#90337,#90338,#90339,#90340,#90341,
#90342,#90343,#90344,#90345,#90346,#90347,#90348,#90349,#90350,#90351,#90352,
#90353,#90354,#90355,#90356,#90357,#90358,#90359,#90360,#90361,#90362,#90363,
#90364,#90365,#90366,#90367,#90368,#90369,#90370,#90371,#90372,#90373,#90374,
#90375,#90376,#90377,#90378,#90379,#90380,#90381,#90382,#90383,#90384,#90385,
#90386,#90387),.UNSPECIFIED.,.F.,.F.,(4,3,3,3,3,3,3,3,3,3,3,3,3,3,3,3,3,
3,3,3,3,3,3,3,4),(0.,0.037326049608827,0.0787965281334718,0.126371615676831,
0.184686823653943,0.249999999999854,0.344927243284897,0.37499999999978,
0.437499999999741,0.468749999999728,0.484374999999721,0.492187499999724,
0.496093749999726,0.498062133788789,0.499042481183733,0.499846118883597,
0.500303114481398,0.558840468960887,0.636460597139664,0.710206569093606,
0.774575228181004,0.838206096083458,0.903983913595566,0.977097659626974,
1.),.UNSPECIFIED.);
#1941=B_SPLINE_CURVE_WITH_KNOTS('',3,(#90391,#90392,#90393,#90394,#90395,
#90396,#90397,#90398,#90399,#90400,#90401,#90402,#90403,#90404,#90405),
 .UNSPECIFIED.,.F.,.F.,(4,2,2,3,2,2,4),(0.0594203506933311,0.0618755831119208,
0.064032651702581,0.0656455089088016,0.0672931027322027,0.0695060324935049,
0.0718717314145315),.UNSPECIFIED.);
#1942=B_SPLINE_CURVE_WITH_KNOTS('',3,(#90414,#90415,#90416,#90417,#90418,
#90419,#90420,#90421,#90422,#90423,#90424,#90425,#90426,#90427,#90428,#90429,
#90430,#90431,#90432,#90433,#90434,#90435,#90436,#90437,#90438,#90439,#90440,
#90441,#90442,#90443,#90444,#90445,#90446,#90447),.UNSPECIFIED.,.F.,.F.,
(4,3,3,3,3,3,3,3,3,3,3,4),(0.,0.0934837719039178,0.19091394803162,0.250000000000001,
0.32133120909575,0.39420774789555,0.471882415487507,0.500000000000003,0.625000000000002,
0.750831352586427,0.878474380660453,1.),.UNSPECIFIED.);
#1943=B_SPLINE_CURVE_WITH_KNOTS('',5,(#90477,#90478,#90479,#90480,#90481,
#90482,#90483,#90484,#90485),.UNSPECIFIED.,.F.,.F.,(6,3,6),(0.,0.446990882614049,
1.),.UNSPECIFIED.);
#1944=B_SPLINE_CURVE_WITH_KNOTS('',3,(#90570,#90571,#90572,#90573,#90574,
#90575,#90576,#90577,#90578,#90579,#90580,#90581,#90582,#90583,#90584,#90585,
#90586,#90587,#90588,#90589,#90590,#90591,#90592,#90593,#90594,#90595,#90596,
#90597,#90598,#90599,#90600,#90601,#90602,#90603,#90604,#90605,#90606,#90607,
#90608,#90609,#90610,#90611,#90612),.UNSPECIFIED.,.F.,.F.,(4,3,3,3,3,3,
3,3,3,3,3,3,3,3,4),(1.75158458902,1.82585854461461,1.90397349676335,1.93627831766,
2.01926759576981,2.10594778966711,2.14030218981,2.22559412880545,2.2812742412,
2.38564669191982,2.42220846454,2.53792768505673,2.67402562128176,2.83070830556877,
2.90384942405),.UNSPECIFIED.);
#1945=B_SPLINE_CURVE_WITH_KNOTS('',3,(#90716,#90717,#90718,#90719,#90720,
#90721,#90722,#90723,#90724,#90725,#90726,#90727,#90728,#90729,#90730,#90731,
#90732,#90733,#90734,#90735,#90736,#90737,#90738,#90739,#90740,#90741,#90742,
#90743,#90744,#90745,#90746,#90747,#90748,#90749,#90750,#90751,#90752,#90753,
#90754,#90755,#90756,#90757,#90758,#90759,#90760,#90761,#90762,#90763,#90764,
#90765,#90766,#90767,#90768,#90769,#90770),.UNSPECIFIED.,.F.,.F.,(4,3,3,
3,3,3,3,3,3,3,3,3,3,3,3,3,3,3,4),(1.90916034578814E-14,0.0632531835392224,
0.125000000000021,0.187500000000027,0.21717261086244,0.245838615885173,
0.250000000000034,0.330431396343107,0.375000000000042,0.437500000000041,
0.468750000000041,0.484375000000041,0.498404612002756,0.500000000000041,
0.600061730332378,0.710615960364526,0.819438906035603,0.918207455217059,
1.),.UNSPECIFIED.);
#1946=B_SPLINE_CURVE_WITH_KNOTS('',3,(#90849,#90850,#90851,#90852,#90853,
#90854,#90855,#90856,#90857,#90858,#90859,#90860,#90861,#90862,#90863,#90864,
#90865,#90866,#90867,#90868,#90869,#90870,#90871,#90872,#90873,#90874,#90875,
#90876,#90877,#90878,#90879,#90880,#90881,#90882,#90883,#90884,#90885,#90886,
#90887,#90888,#90889,#90890,#90891,#90892,#90893,#90894,#90895,#90896,#90897,
#90898,#90899,#90900,#90901,#90902,#90903,#90904,#90905,#90906),
 .UNSPECIFIED.,.F.,.F.,(4,3,3,3,3,3,3,3,3,3,3,3,3,3,3,3,3,3,3,4),(0.,0.0968230900403072,
0.201906635741557,0.306544326813906,0.403561202366286,0.449263932419849,
0.499999999999999,0.574890464499785,0.62962833045408,0.678442829509228,
0.722855417361369,0.73519144804672,0.7684367799326,0.803987925548705,0.841333943790706,
0.877807153721906,0.91063890722932,0.941813275174746,0.970955904576958,
1.),.UNSPECIFIED.);
#1947=B_SPLINE_CURVE_WITH_KNOTS('',3,(#90919,#90920,#90921,#90922,#90923,
#90924,#90925,#90926,#90927,#90928,#90929,#90930,#90931,#90932,#90933,#90934,
#90935,#90936,#90937,#90938,#90939,#90940,#90941,#90942,#90943,#90944,#90945,
#90946,#90947,#90948,#90949,#90950,#90951,#90952,#90953,#90954,#90955,#90956,
#90957,#90958,#90959,#90960,#90961,#90962,#90963,#90964,#90965,#90966,#90967,
#90968,#90969,#90970,#90971,#90972,#90973,#90974,#90975,#90976,#90977,#90978,
#90979,#90980,#90981,#90982,#90983,#90984,#90985,#90986,#90987,#90988,#90989,
#90990,#90991,#90992,#90993,#90994,#90995,#90996,#90997,#90998,#90999,#91000,
#91001,#91002,#91003,#91004,#91005,#91006,#91007,#91008,#91009,#91010,#91011,
#91012,#91013,#91014,#91015,#91016,#91017,#91018,#91019,#91020,#91021,#91022,
#91023,#91024,#91025,#91026,#91027,#91028,#91029,#91030,#91031,#91032,#91033,
#91034,#91035,#91036,#91037,#91038,#91039,#91040,#91041,#91042,#91043,#91044,
#91045,#91046,#91047,#91048,#91049,#91050,#91051,#91052,#91053,#91054,#91055,
#91056,#91057),.UNSPECIFIED.,.F.,.F.,(4,3,3,3,3,3,3,3,3,3,3,3,3,3,3,3,3,
3,3,3,3,3,3,3,3,3,3,3,3,3,3,3,3,3,3,3,3,3,3,3,3,3,3,3,3,3,4),(0.,0.0625000000000785,
0.086696354991142,0.11143417047313,0.125000000000157,0.187500000000235,
0.218750000000271,0.234375000000292,0.242187500000302,0.24708318045769,
0.250000000000312,0.262692941916091,0.265625000000332,0.273437500000337,
0.278246584391903,0.281250000000343,0.300621388827372,0.312500000000354,
0.343750000000357,0.375000000000361,0.403949752381917,0.433650417141628,
0.437500000000369,0.468750000000382,0.484375000000398,0.492502293593455,
0.500000000000413,0.521207465216726,0.531250000000391,0.546875000000378,
0.554732671383366,0.562500000000365,0.614860839166667,0.625000000000341,
0.687500000000317,0.718750000000291,0.734375000000279,0.743278564543908,
0.750000000000267,0.772730668789083,0.781250000000243,0.796875000000232,
0.805294656260953,0.812500000000222,0.856624166056844,0.875000000000148,
1.),.UNSPECIFIED.);
#1948=B_SPLINE_CURVE_WITH_KNOTS('',3,(#91061,#91062,#91063,#91064,#91065,
#91066,#91067,#91068,#91069,#91070,#91071,#91072,#91073,#91074,#91075,#91076,
#91077,#91078,#91079,#91080,#91081,#91082,#91083,#91084,#91085,#91086,#91087,
#91088,#91089,#91090,#91091,#91092,#91093,#91094,#91095,#91096,#91097,#91098,
#91099,#91100,#91101,#91102,#91103,#91104,#91105,#91106,#91107,#91108,#91109,
#91110,#91111,#91112,#91113,#91114,#91115),.UNSPECIFIED.,.F.,.F.,(4,3,3,
3,3,3,3,3,3,3,3,3,3,3,3,3,3,3,4),(0.,0.0980793331889885,0.195976519023509,
0.250000000000014,0.352035260039166,0.375000000000008,0.437500000000004,
0.465353490595414,0.494109597505518,0.500000000000001,0.572333705374357,
0.641941232753823,0.707651845844047,0.75,0.8125,0.872864157449969,0.931710851416161,
0.988699096048787,1.),.UNSPECIFIED.);
#1949=B_SPLINE_CURVE_WITH_KNOTS('',3,(#91123,#91124,#91125,#91126,#91127,
#91128,#91129,#91130,#91131,#91132,#91133,#91134,#91135,#91136,#91137,#91138,
#91139,#91140,#91141,#91142,#91143,#91144,#91145,#91146,#91147,#91148,#91149,
#91150,#91151,#91152,#91153,#91154,#91155,#91156,#91157,#91158,#91159,#91160,
#91161,#91162,#91163,#91164,#91165,#91166,#91167,#91168,#91169,#91170,#91171,
#91172,#91173,#91174,#91175,#91176,#91177,#91178,#91179,#91180),
 .UNSPECIFIED.,.F.,.F.,(4,3,3,3,3,3,3,3,3,3,3,3,3,3,3,3,3,3,3,4),(0.,0.0994522270089912,
0.19855275762107,0.249999999999961,0.320807500310168,0.390438933372071,
0.456941047442724,0.499999999999922,0.580884161076493,0.624999999999912,
0.687499999999914,0.718749999999915,0.732736627016244,0.747996545903896,
0.749999999999915,0.805252631848376,0.857501453771511,0.90793686231154,
0.955604059001085,1.),.UNSPECIFIED.);
#1950=B_SPLINE_CURVE_WITH_KNOTS('',3,(#91184,#91185,#91186,#91187,#91188,
#91189,#91190,#91191,#91192,#91193,#91194,#91195,#91196,#91197,#91198,#91199,
#91200,#91201,#91202,#91203,#91204,#91205,#91206,#91207,#91208,#91209,#91210,
#91211,#91212,#91213,#91214,#91215,#91216,#91217,#91218,#91219,#91220,#91221,
#91222,#91223,#91224,#91225,#91226,#91227,#91228,#91229,#91230,#91231,#91232,
#91233,#91234,#91235,#91236,#91237,#91238,#91239,#91240,#91241,#91242,#91243,
#91244,#91245,#91246,#91247,#91248,#91249,#91250),.UNSPECIFIED.,.F.,.F.,
(4,3,3,3,3,3,3,3,3,3,3,3,3,3,3,3,3,3,3,3,3,3,4),(0.,0.0338071905107698,
0.0625000000000105,0.0937500000000157,0.109375000000018,0.118222061923896,
0.125000000000021,0.171255468817826,0.220321915300574,0.250000000000024,
0.320854902327379,0.375000000000027,0.437500000000027,0.46328755320113,
0.490851192655088,0.500000000000028,0.625000000000029,0.669712733186267,
0.715775887477275,0.75000000000003,0.845897353941236,0.944150142413249,
1.),.UNSPECIFIED.);
#1951=B_SPLINE_CURVE_WITH_KNOTS('',3,(#91254,#91255,#91256,#91257,#91258,
#91259,#91260,#91261,#91262,#91263,#91264,#91265,#91266,#91267,#91268,#91269,
#91270,#91271,#91272,#91273,#91274,#91275,#91276,#91277,#91278,#91279,#91280,
#91281,#91282,#91283,#91284,#91285,#91286,#91287,#91288,#91289,#91290,#91291,
#91292,#91293,#91294,#91295,#91296,#91297,#91298,#91299,#91300,#91301,#91302,
#91303,#91304,#91305,#91306,#91307,#91308,#91309,#91310,#91311),
 .UNSPECIFIED.,.F.,.F.,(4,3,3,3,3,3,3,3,3,3,3,3,3,3,3,3,3,3,3,4),(0.,0.0451092776599689,
0.0925039027641494,0.12500000000001,0.174913836077685,0.187500000000022,
0.218750000000022,0.234375000000022,0.248604010257293,0.250000000000022,
0.318607877079331,0.375000000000026,0.41738420156605,0.462520462216422,
0.50000000000003,0.59283675164862,0.689308660068251,0.789872400074604,0.894936200037302,
1.),.UNSPECIFIED.);
#1952=B_SPLINE_CURVE_WITH_KNOTS('',3,(#91433,#91434,#91435,#91436,#91437,
#91438,#91439,#91440,#91441,#91442,#91443,#91444,#91445,#91446,#91447,#91448,
#91449,#91450,#91451,#91452,#91453,#91454,#91455,#91456,#91457,#91458,#91459,
#91460,#91461,#91462,#91463,#91464,#91465,#91466,#91467,#91468,#91469,#91470,
#91471,#91472,#91473,#91474,#91475,#91476,#91477,#91478,#91479,#91480,#91481,
#91482,#91483,#91484,#91485,#91486,#91487),.UNSPECIFIED.,.F.,.F.,(4,3,3,
3,3,3,3,3,3,3,3,3,3,3,3,3,3,3,4),(0.,0.102320181390481,0.201694320732233,
0.249999999999988,0.345937965973561,0.374999999999982,0.43749999999998,
0.468749999999972,0.484374999999968,0.492839606007928,0.499999999999964,
0.576579098012344,0.651305076097686,0.722730977064833,0.749999999999982,
0.81633078076096,0.880405936123099,0.941174730499775,1.),.UNSPECIFIED.);
#1953=B_SPLINE_CURVE_WITH_KNOTS('',5,(#91551,#91552,#91553,#91554,#91555,
#91556,#91557,#91558,#91559),.UNSPECIFIED.,.F.,.F.,(6,3,6),(0.,0.459694365459143,
1.),.UNSPECIFIED.);
#1954=B_SPLINE_CURVE_WITH_KNOTS('',3,(#91561,#91562,#91563,#91564,#91565,
#91566,#91567,#91568,#91569,#91570,#91571,#91572,#91573,#91574,#91575,#91576,
#91577,#91578,#91579,#91580,#91581,#91582,#91583,#91584,#91585,#91586,#91587,
#91588,#91589,#91590,#91591,#91592,#91593,#91594,#91595,#91596,#91597),
 .UNSPECIFIED.,.F.,.F.,(4,3,3,3,3,3,3,3,3,3,3,3,4),(0.,0.0831702685280121,
0.167847262437448,0.25483900256361,0.342953378583159,0.432342539351743,
0.5,0.589502114356238,0.678232387149981,0.76504398598027,0.850564991306322,
0.933989360303386,1.),.UNSPECIFIED.);
#1955=B_SPLINE_CURVE_WITH_KNOTS('',3,(#91622,#91623,#91624,#91625,#91626,
#91627,#91628,#91629,#91630,#91631,#91632,#91633,#91634,#91635,#91636,#91637,
#91638,#91639,#91640,#91641,#91642,#91643,#91644,#91645,#91646,#91647,#91648,
#91649,#91650,#91651,#91652,#91653,#91654,#91655,#91656,#91657,#91658,#91659,
#91660,#91661),.UNSPECIFIED.,.F.,.F.,(4,3,3,3,3,3,3,3,3,3,3,3,3,4),(1.69812247662,
1.82517827643346,1.94835352449351,2.04354239572,2.1493981491557,2.2504202018726,
2.34618007075805,2.37608580106,2.46390218046495,2.55211800019734,2.6379844451379,
2.6897944832,2.77017696446133,2.83469359842),.UNSPECIFIED.);
#1956=B_SPLINE_CURVE_WITH_KNOTS('',3,(#91673,#91674,#91675,#91676,#91677,
#91678,#91679,#91680,#91681,#91682,#91683,#91684,#91685,#91686,#91687,#91688,
#91689,#91690,#91691,#91692,#91693,#91694,#91695,#91696,#91697,#91698,#91699,
#91700,#91701,#91702,#91703,#91704,#91705,#91706,#91707,#91708,#91709,#91710,
#91711,#91712,#91713,#91714,#91715,#91716,#91717,#91718,#91719,#91720,#91721,
#91722,#91723,#91724,#91725,#91726,#91727,#91728,#91729,#91730),
 .UNSPECIFIED.,.F.,.F.,(4,3,3,3,3,3,3,3,3,3,3,3,3,3,3,3,3,3,3,4),(4.76185240083,
4.83763310355387,4.8511070755,4.9237368026632,4.94035737066,5.01616912552097,
5.04125309343,5.11983939701062,5.14214350511,5.21975609722012,5.29603838282238,
5.31344541544,5.40219520324995,5.47351631749,5.56538841319371,5.65858597861109,
5.75320413758695,5.78071175361,5.87661154462981,5.93786871511),
 .UNSPECIFIED.);
#1957=B_SPLINE_CURVE_WITH_KNOTS('',3,(#91734,#91735,#91736,#91737,#91738,
#91739,#91740,#91741,#91742,#91743,#91744,#91745,#91746,#91747,#91748,#91749,
#91750,#91751,#91752,#91753,#91754,#91755,#91756,#91757,#91758,#91759,#91760,
#91761,#91762,#91763,#91764,#91765,#91766,#91767,#91768,#91769,#91770,#91771,
#91772,#91773,#91774,#91775,#91776,#91777,#91778,#91779,#91780,#91781,#91782,
#91783,#91784,#91785,#91786,#91787,#91788,#91789,#91790,#91791),
 .UNSPECIFIED.,.F.,.F.,(4,3,3,3,3,3,3,3,3,3,3,3,3,3,3,3,3,3,3,4),(2.86340882221,
2.96038236608018,2.9912183572,3.08700311846,3.18278787972,3.27460804500352,
3.36346730309093,3.3764526533,3.45865940729478,3.54085709160542,3.57484410128,
3.65773122998382,3.67917202515,3.75805208465001,3.78350088337,3.86115067208,
3.93423338613355,3.93880046079,4.01498217619634,4.03947605191),
 .UNSPECIFIED.);
#1958=B_SPLINE_CURVE_WITH_KNOTS('',3,(#91813,#91814,#91815,#91816,#91817,
#91818,#91819,#91820,#91821,#91822,#91823,#91824,#91825,#91826,#91827,#91828,
#91829,#91830,#91831,#91832,#91833,#91834,#91835,#91836,#91837,#91838,#91839,
#91840,#91841,#91842,#91843,#91844,#91845,#91846,#91847,#91848,#91849),
 .UNSPECIFIED.,.F.,.F.,(4,3,3,3,3,3,3,3,3,3,3,3,4),(9.16687616257107E-11,
0.0777713091928336,0.155304544748419,0.235796293739508,0.250000000000001,
0.375000000000002,0.426033233674526,0.476997002990943,0.500000000000003,
0.647319737369125,0.788544793198841,0.917036474768495,1.),.UNSPECIFIED.);
#1959=B_SPLINE_CURVE_WITH_KNOTS('',3,(#91865,#91866,#91867,#91868,#91869,
#91870,#91871,#91872,#91873,#91874,#91875,#91876,#91877,#91878,#91879,#91880,
#91881,#91882,#91883,#91884,#91885,#91886,#91887,#91888,#91889,#91890,#91891,
#91892,#91893,#91894,#91895,#91896,#91897,#91898,#91899,#91900,#91901),
 .UNSPECIFIED.,.F.,.F.,(4,3,3,3,3,3,3,3,3,3,3,3,4),(9.16667455825459E-11,
0.0777713111959483,0.1553045487284,0.235796299444816,0.249999999999999,
0.374999999999999,0.426033234695566,0.476997005066265,0.499999999999998,
0.647319737403808,0.788544793261829,0.917036474850319,1.),.UNSPECIFIED.);
#1960=B_SPLINE_CURVE_WITH_KNOTS('',3,(#91905,#91906,#91907,#91908),
 .UNSPECIFIED.,.F.,.F.,(4,4),(-1.68203627824,-1.66422823568),
 .UNSPECIFIED.);
#1961=B_SPLINE_CURVE_WITH_KNOTS('',3,(#91910,#91911,#91912,#91913),
 .UNSPECIFIED.,.F.,.F.,(4,4),(-1.04373195388,-1.00826496187),
 .UNSPECIFIED.);
#1962=B_SPLINE_CURVE_WITH_KNOTS('',5,(#91938,#91939,#91940,#91941,#91942,
#91943),.UNSPECIFIED.,.F.,.F.,(6,6),(0.,1.),.UNSPECIFIED.);
#1963=B_SPLINE_CURVE_WITH_KNOTS('',3,(#91948,#91949,#91950,#91951,#91952,
#91953,#91954,#91955,#91956,#91957,#91958,#91959,#91960,#91961,#91962,#91963,
#91964,#91965,#91966,#91967,#91968,#91969,#91970,#91971,#91972,#91973,#91974,
#91975,#91976,#91977,#91978,#91979,#91980,#91981,#91982,#91983,#91984,#91985,
#91986,#91987),.UNSPECIFIED.,.F.,.F.,(4,3,3,3,3,3,3,3,3,3,3,3,3,4),(1.64208556101,
1.72926070554228,1.73827899693,1.8278907907593,1.92154711062456,2.01700443389081,
2.1132071936736,2.12883652195,2.23557388803073,2.32877794125,2.44459839436569,
2.5306802585,2.66108985588594,2.73162696034),.UNSPECIFIED.);
#1964=B_SPLINE_CURVE_WITH_KNOTS('',3,(#92031,#92032,#92033,#92034,#92035,
#92036,#92037,#92038,#92039,#92040,#92041,#92042,#92043,#92044,#92045,#92046,
#92047,#92048,#92049,#92050,#92051,#92052,#92053,#92054,#92055,#92056,#92057,
#92058,#92059,#92060,#92061),.UNSPECIFIED.,.F.,.F.,(4,3,3,3,3,3,3,3,3,3,
4),(0.,0.0955467215590676,0.196660041169301,0.296253107708768,0.398126553854384,
0.5,0.601416708013665,0.701415344786851,0.800181615448635,0.900090807724317,
1.),.UNSPECIFIED.);
#1965=B_SPLINE_CURVE_WITH_KNOTS('',3,(#92172,#92173,#92174,#92175),
 .UNSPECIFIED.,.F.,.F.,(4,4),(-1.04373195388,-1.00826496187),
 .UNSPECIFIED.);
#1966=B_SPLINE_CURVE_WITH_KNOTS('',3,(#92260,#92261,#92262,#92263,#92264,
#92265,#92266,#92267,#92268,#92269,#92270,#92271,#92272,#92273,#92274,#92275,
#92276,#92277,#92278,#92279,#92280,#92281,#92282,#92283,#92284,#92285,#92286,
#92287),.UNSPECIFIED.,.F.,.F.,(4,3,3,3,3,3,3,3,3,4),(3.98942132494305E-9,
0.150497117185246,0.288254537029539,0.376907505501659,0.503498889679138,
0.532680629126244,0.664294493152615,0.802603697848191,0.950070961802982,
1.),.UNSPECIFIED.);
#1967=B_SPLINE_CURVE_WITH_KNOTS('',3,(#92313,#92314,#92315,#92316),
 .UNSPECIFIED.,.F.,.F.,(4,4),(-1.68203627824,-1.66422823568),
 .UNSPECIFIED.);
#1968=B_SPLINE_CURVE_WITH_KNOTS('',3,(#92416,#92417,#92418,#92419,#92420,
#92421,#92422,#92423,#92424,#92425,#92426,#92427,#92428,#92429,#92430,#92431,
#92432,#92433,#92434,#92435,#92436,#92437,#92438,#92439,#92440,#92441,#92442,
#92443),.UNSPECIFIED.,.F.,.F.,(4,3,3,3,3,3,3,3,3,4),(3.98063301892076E-9,
0.150497117191435,0.288254537058802,0.376907505472153,0.503498889669673,
0.532680629104115,0.664294493113039,0.802603697754453,0.950070961594217,
1.),.UNSPECIFIED.);
#1969=B_SPLINE_CURVE_WITH_KNOTS('',3,(#92536,#92537,#92538,#92539,#92540,
#92541,#92542,#92543,#92544,#92545,#92546,#92547,#92548,#92549,#92550,#92551,
#92552,#92553,#92554,#92555,#92556,#92557,#92558,#92559,#92560,#92561,#92562,
#92563,#92564,#92565,#92566,#92567,#92568,#92569,#92570,#92571,#92572,#92573,
#92574,#92575,#92576,#92577,#92578,#92579,#92580,#92581,#92582,#92583,#92584,
#92585,#92586,#92587,#92588,#92589,#92590,#92591,#92592,#92593,#92594,#92595,
#92596,#92597,#92598,#92599,#92600,#92601,#92602,#92603,#92604,#92605,#92606,
#92607,#92608,#92609,#92610,#92611),.UNSPECIFIED.,.F.,.F.,(4,3,3,3,3,3,
3,3,3,3,3,3,3,3,3,3,3,3,3,3,3,3,3,3,3,4),(0.,0.0937499999999247,0.183615921210463,
0.273457967111046,0.363302606689923,0.374999999999699,0.437499999999654,
0.468749999999633,0.481912351571244,0.496444815995831,0.499999999999611,
0.562499999999591,0.593749999999593,0.609374999999607,0.618302120244718,
0.624999999999621,0.650015547301732,0.656249999999664,0.671050151688994,
0.685059338020028,0.687499999999707,0.714547929086675,0.744158092899608,
0.749999999999772,0.922985773999486,1.),.UNSPECIFIED.);
#1970=B_SPLINE_CURVE_WITH_KNOTS('',3,(#92615,#92616,#92617,#92618,#92619,
#92620,#92621,#92622,#92623,#92624,#92625,#92626,#92627,#92628,#92629,#92630,
#92631,#92632,#92633,#92634,#92635,#92636,#92637,#92638,#92639,#92640,#92641,
#92642,#92643,#92644,#92645,#92646,#92647,#92648,#92649,#92650,#92651,#92652,
#92653,#92654,#92655,#92656,#92657,#92658,#92659,#92660,#92661,#92662,#92663,
#92664,#92665,#92666,#92667,#92668,#92669,#92670,#92671,#92672),
 .UNSPECIFIED.,.F.,.F.,(4,3,3,3,3,3,3,3,3,3,3,3,3,3,3,3,3,3,3,4),(0.,0.0443451168985777,
0.0909483516403088,0.125000000000021,0.174152759844734,0.187500000000031,
0.21875000000003,0.234375000000029,0.248688920390979,0.250000000000029,
0.318111984407296,0.375000000000013,0.415894282087958,0.459570458469752,
0.499999999999998,0.592678771259659,0.688958966630604,0.78925342781995,
0.894626713909975,1.),.UNSPECIFIED.);
#1971=B_SPLINE_CURVE_WITH_KNOTS('',3,(#92683,#92684,#92685,#92686,#92687,
#92688,#92689,#92690,#92691,#92692,#92693,#92694,#92695,#92696,#92697,#92698,
#92699,#92700,#92701,#92702,#92703,#92704,#92705,#92706,#92707,#92708,#92709,
#92710,#92711,#92712,#92713,#92714,#92715,#92716,#92717,#92718,#92719,#92720,
#92721,#92722,#92723,#92724,#92725,#92726,#92727,#92728,#92729,#92730,#92731,
#92732,#92733,#92734,#92735,#92736,#92737,#92738,#92739,#92740,#92741,#92742,
#92743,#92744,#92745,#92746,#92747,#92748,#92749,#92750,#92751,#92752,#92753,
#92754,#92755),.UNSPECIFIED.,.F.,.F.,(4,3,3,3,3,3,3,3,3,3,3,3,3,3,3,3,3,
3,3,3,3,3,3,3,4),(0.,0.0943040666939272,0.18898259270498,0.250000000000074,
0.350492487940872,0.375000000000096,0.437500000000093,0.464977671236868,
0.490762671002707,0.500000000000091,0.579331802709907,0.625000000000066,
0.665840272931786,0.707920136465913,0.745842552516937,0.750000000000041,
0.812500000000029,0.843750000000022,0.856467201676309,0.870123765069302,
0.875000000000016,0.912439301208134,0.948859469697768,0.983548250663145,
1.),.UNSPECIFIED.);
#1972=B_SPLINE_CURVE_WITH_KNOTS('',3,(#92759,#92760,#92761,#92762,#92763,
#92764,#92765,#92766,#92767,#92768,#92769,#92770,#92771,#92772,#92773,#92774,
#92775,#92776,#92777,#92778,#92779,#92780,#92781,#92782,#92783,#92784,#92785,
#92786,#92787,#92788,#92789,#92790,#92791,#92792,#92793,#92794,#92795,#92796,
#92797,#92798,#92799,#92800,#92801,#92802,#92803,#92804,#92805,#92806,#92807,
#92808,#92809,#92810,#92811,#92812,#92813,#92814,#92815,#92816,#92817,#92818,
#92819,#92820,#92821,#92822,#92823,#92824,#92825),.UNSPECIFIED.,.F.,.F.,
(4,3,3,3,3,3,3,3,3,3,3,3,3,3,3,3,3,3,3,3,3,3,4),(0.,0.12499999999999,0.188571899414555,
0.24999999999998,0.37499999999997,0.437500000000004,0.466500812528174,0.50000000000004,
0.541171395769626,0.583085697884828,0.62500000000003,0.665266761660683,
0.704453084784077,0.741405254291436,0.776868942642716,0.810906560932425,
0.843624402352047,0.875137715833154,0.906353286874866,0.935335899732279,
0.963556417430368,0.990779891878734,1.),.UNSPECIFIED.);
#1973=B_SPLINE_CURVE_WITH_KNOTS('',3,(#92834,#92835,#92836,#92837,#92838,
#92839,#92840,#92841,#92842,#92843,#92844,#92845,#92846,#92847,#92848,#92849,
#92850,#92851,#92852,#92853,#92854,#92855,#92856,#92857,#92858,#92859,#92860,
#92861,#92862,#92863,#92864,#92865,#92866,#92867,#92868,#92869,#92870,#92871,
#92872,#92873,#92874,#92875,#92876,#92877,#92878,#92879,#92880,#92881,#92882,
#92883,#92884,#92885,#92886,#92887,#92888,#92889,#92890,#92891,#92892,#92893,
#92894,#92895,#92896,#92897,#92898,#92899,#92900,#92901,#92902,#92903,#92904,
#92905,#92906,#92907,#92908,#92909,#92910,#92911,#92912,#92913,#92914,#92915,
#92916,#92917,#92918,#92919,#92920,#92921,#92922,#92923,#92924,#92925,#92926,
#92927,#92928,#92929,#92930,#92931,#92932,#92933,#92934,#92935,#92936,#92937,
#92938,#92939,#92940,#92941,#92942,#92943,#92944,#92945),.UNSPECIFIED.,
 .F.,.F.,(4,3,3,3,3,3,3,3,3,3,3,3,3,3,3,3,3,3,3,3,3,3,3,3,3,3,3,3,3,3,3,
3,3,3,3,3,3,4),(0.,0.125000000002865,0.187500000004281,0.216128186234356,
0.243284284702797,0.250000000005696,0.352348172379624,0.375000000008529,
0.437500000009947,0.462030398295331,0.485130811504489,0.500000000011365,
0.562500000012783,0.593750000013494,0.609375000013851,0.617187500014019,
0.622662434262975,0.625000000014188,0.642795177114311,0.656250000014155,
0.671875000014138,0.678967911692179,0.686342149067149,0.687500000014121,
0.718750000014078,0.734375000014051,0.742187500014035,0.747488512167396,
0.75000000001402,0.781436979920065,0.813065815197281,0.844518835992743,
0.87500000000701,0.904533702371711,0.932006850722208,0.958333127878501,
0.983097804372786,1.),.UNSPECIFIED.);
#1974=B_SPLINE_CURVE_WITH_KNOTS('',3,(#92966,#92967,#92968,#92969,#92970,
#92971,#92972,#92973,#92974,#92975,#92976,#92977,#92978,#92979,#92980,#92981,
#92982,#92983,#92984,#92985,#92986,#92987,#92988,#92989,#92990,#92991,#92992,
#92993,#92994,#92995,#92996,#92997,#92998,#92999,#93000,#93001,#93002,#93003,
#93004,#93005,#93006,#93007,#93008,#93009,#93010,#93011,#93012,#93013,#93014,
#93015,#93016,#93017,#93018,#93019,#93020,#93021,#93022,#93023),
 .UNSPECIFIED.,.F.,.F.,(4,3,3,3,3,3,3,3,3,3,3,3,3,3,3,3,3,3,3,4),(0.,0.125000000000002,
0.250000000000005,0.365236498453909,0.375000000000007,0.421011993194877,
0.467170215472028,0.50000000000001,0.58605609992678,0.625000000000013,0.687500000000008,
0.71875,0.73247917279936,0.747722802633476,0.749999999999991,0.812499999999993,
0.869829956013398,0.925192869595088,0.977789571163086,1.),.UNSPECIFIED.);
#1975=B_SPLINE_CURVE_WITH_KNOTS('',3,(#93100,#93101,#93102,#93103,#93104,
#93105,#93106,#93107,#93108,#93109,#93110,#93111,#93112,#93113,#93114,#93115,
#93116,#93117,#93118,#93119,#93120,#93121,#93122,#93123,#93124,#93125,#93126,
#93127,#93128,#93129,#93130,#93131,#93132,#93133,#93134,#93135,#93136,#93137,
#93138,#93139,#93140,#93141,#93142,#93143,#93144,#93145,#93146,#93147,#93148,
#93149,#93150,#93151,#93152,#93153,#93154,#93155,#93156,#93157,#93158,#93159,
#93160,#93161,#93162,#93163),.UNSPECIFIED.,.F.,.F.,(4,3,3,3,3,3,3,3,3,3,
3,3,3,3,3,3,3,3,3,3,3,4),(1.30569972989664E-13,0.0394023736834368,0.0822011868417158,
0.124999999999995,0.167289105223367,0.187499999999992,0.209945720373917,
0.23456433282999,0.249999999999988,0.325623787343657,0.374999999999979,
0.437499999999978,0.468749999999984,0.484374999999988,0.493888833934045,
0.499999999999991,0.597586484903761,0.69843638032809,0.791729532747611,
0.881731622630255,0.968663051431044,1.),.UNSPECIFIED.);
#1976=B_SPLINE_CURVE_WITH_KNOTS('',3,(#93166,#93167,#93168,#93169,#93170,
#93171,#93172,#93173,#93174,#93175,#93176,#93177,#93178,#93179,#93180,#93181,
#93182,#93183,#93184,#93185,#93186,#93187,#93188,#93189,#93190,#93191,#93192,
#93193,#93194,#93195,#93196,#93197,#93198,#93199,#93200,#93201,#93202,#93203,
#93204,#93205,#93206,#93207,#93208,#93209,#93210,#93211,#93212,#93213,#93214),
 .UNSPECIFIED.,.F.,.F.,(4,3,3,3,3,3,3,3,3,3,3,3,3,3,3,3,4),(0.,0.0646375542710448,
0.131986214404462,0.205237786349825,0.25,0.3363751967743,0.420131595217952,
0.5,0.569501845294344,0.635666297979706,0.697934450928747,0.75,0.808915454001482,
0.865550018011427,0.92107127627776,0.975154358484857,1.),.UNSPECIFIED.);
#1977=B_SPLINE_CURVE_WITH_KNOTS('',3,(#93412,#93413,#93414,#93415,#93416,
#93417,#93418,#93419,#93420,#93421,#93422,#93423,#93424,#93425,#93426,#93427,
#93428,#93429,#93430,#93431,#93432,#93433,#93434,#93435,#93436,#93437,#93438,
#93439,#93440,#93441,#93442,#93443,#93444,#93445,#93446,#93447,#93448,#93449,
#93450,#93451,#93452,#93453,#93454,#93455,#93456,#93457,#93458,#93459,#93460,
#93461,#93462,#93463,#93464,#93465,#93466,#93467,#93468,#93469,#93470,#93471,
#93472,#93473,#93474,#93475),.UNSPECIFIED.,.F.,.F.,(4,3,3,3,3,3,3,3,3,3,
3,3,3,3,3,3,3,3,3,3,3,4),(0.,0.0313265556561311,0.0639694708706069,0.0991532878456469,
0.125000000000003,0.161981198945146,0.197636162313631,0.230727451571766,
0.250000000000005,0.263633961320155,0.302088741633232,0.352565680645548,
0.397399712184553,0.468832078691233,0.500000000000002,0.586077893149075,
0.674777857656565,0.714614915280701,0.807100572165139,0.903550286082569,
0.980940289322871,1.),.UNSPECIFIED.);
#1978=B_SPLINE_CURVE_WITH_KNOTS('',3,(#93477,#93478,#93479,#93480,#93481,
#93482,#93483,#93484,#93485,#93486,#93487,#93488,#93489,#93490,#93491,#93492,
#93493,#93494,#93495,#93496,#93497,#93498,#93499,#93500,#93501,#93502,#93503,
#93504,#93505,#93506,#93507,#93508,#93509,#93510,#93511,#93512,#93513,#93514,
#93515,#93516,#93517,#93518,#93519,#93520,#93521,#93522),.UNSPECIFIED.,
 .F.,.F.,(4,3,3,3,3,3,3,3,3,3,3,3,3,3,3,4),(0.,0.0676469801677771,0.137106796073644,
0.209683116828569,0.250000000000043,0.327522831121316,0.375000000000065,
0.437500000000081,0.468750000000089,0.484661840756592,0.500000000000098,
0.609757695881578,0.72628120414161,0.847292917845917,0.975661564746343,
1.),.UNSPECIFIED.);
#1979=B_SPLINE_CURVE_WITH_KNOTS('',3,(#93542,#93543,#93544,#93545,#93546,
#93547,#93548,#93549,#93550,#93551,#93552,#93553,#93554,#93555,#93556,#93557,
#93558,#93559,#93560,#93561,#93562,#93563,#93564,#93565,#93566,#93567,#93568,
#93569,#93570,#93571,#93572,#93573,#93574,#93575),.UNSPECIFIED.,.F.,.F.,
(4,3,3,3,3,3,3,3,3,3,3,4),(1.25405163269,1.32643264163,1.4055803165725,
1.48574465294545,1.56752327448427,1.6430233414,1.72858124378027,1.81406569145,
1.90733041601598,1.99715560017,2.09477370437,2.19239180857),
 .UNSPECIFIED.);
#1980=B_SPLINE_CURVE_WITH_KNOTS('',3,(#93633,#93634,#93635,#93636,#93637,
#93638,#93639,#93640,#93641,#93642,#93643,#93644,#93645,#93646,#93647,#93648,
#93649,#93650,#93651,#93652,#93653,#93654,#93655,#93656,#93657,#93658,#93659,
#93660,#93661,#93662,#93663,#93664,#93665,#93666,#93667,#93668,#93669,#93670,
#93671,#93672,#93673,#93674,#93675,#93676,#93677,#93678,#93679,#93680,#93681,
#93682,#93683,#93684,#93685,#93686,#93687,#93688,#93689,#93690,#93691,#93692,
#93693),.UNSPECIFIED.,.F.,.F.,(4,3,3,3,3,3,3,3,3,3,3,3,3,3,3,3,3,3,3,3,
4),(0.,0.0757360115643633,0.153309514148711,0.232749548769837,0.249999999999913,
0.329782774192022,0.374999999999877,0.42601283745248,0.437499999999857,
0.468749999999847,0.484374999999842,0.493943320438178,0.499999999999837,
0.562810053136719,0.62772503823603,0.695349843164152,0.749999999999919,
0.823320223135299,0.899885323406126,0.981080192972812,1.),.UNSPECIFIED.);
#1981=B_SPLINE_CURVE_WITH_KNOTS('',3,(#93752,#93753,#93754,#93755,#93756,
#93757,#93758,#93759,#93760,#93761,#93762,#93763,#93764,#93765,#93766,#93767,
#93768,#93769,#93770,#93771,#93772,#93773,#93774,#93775,#93776,#93777,#93778,
#93779,#93780,#93781,#93782,#93783,#93784,#93785,#93786,#93787,#93788,#93789,
#93790,#93791,#93792,#93793,#93794,#93795,#93796,#93797,#93798,#93799,#93800,
#93801,#93802,#93803,#93804,#93805,#93806,#93807,#93808,#93809),
 .UNSPECIFIED.,.F.,.F.,(4,3,3,3,3,3,3,3,3,3,3,3,3,3,3,3,3,3,3,4),(0.,0.0795529238434195,
0.156039645963624,0.227878159961086,0.250000000000057,0.319021097031273,
0.375000000000083,0.4375000000001,0.468750000000104,0.474796994033287,0.484375000000107,
0.493485330168561,0.500000000000109,0.585436846623337,0.667718423311696,
0.750000000000055,0.829338336199628,0.906967603645166,0.981482011220185,
1.),.UNSPECIFIED.);
#1982=B_SPLINE_CURVE_WITH_KNOTS('',3,(#93826,#93827,#93828,#93829,#93830,
#93831,#93832,#93833,#93834,#93835,#93836,#93837),.UNSPECIFIED.,.F.,.F.,
(4,2,2,2,2,4),(-0.2526817413658,-0.252144968685117,-0.231701265952628,-0.221146902348503,
-0.215214602553632,-0.211845320308325),.UNSPECIFIED.);
#1983=B_SPLINE_CURVE_WITH_KNOTS('',5,(#93866,#93867,#93868,#93869,#93870,
#93871),.UNSPECIFIED.,.F.,.F.,(6,6),(0.,0.999999959271343),
 .UNSPECIFIED.);
#1984=B_SPLINE_CURVE_WITH_KNOTS('',3,(#93929,#93930,#93931,#93932,#93933,
#93934,#93935,#93936,#93937,#93938,#93939,#93940,#93941,#93942,#93943,#93944,
#93945,#93946,#93947,#93948,#93949,#93950,#93951,#93952,#93953,#93954,#93955,
#93956,#93957,#93958,#93959,#93960,#93961,#93962,#93963,#93964,#93965,#93966,
#93967,#93968,#93969,#93970,#93971,#93972,#93973,#93974,#93975,#93976,#93977,
#93978,#93979,#93980,#93981,#93982,#93983,#93984,#93985,#93986,#93987,#93988,
#93989,#93990,#93991,#93992),.UNSPECIFIED.,.F.,.F.,(4,3,3,3,3,3,3,3,3,3,
3,3,3,3,3,3,3,3,3,3,3,4),(0.,0.103653379061186,0.20361411417021,0.249999999999959,
0.345078024193049,0.374999999999938,0.437499999999928,0.452274762523055,
0.468749999999922,0.483386774211928,0.499999999999916,0.578583158147426,
0.624999999999938,0.671874999999946,0.684061297709991,0.690640429806601,
0.714634449294438,0.732469796213536,0.74919043395019,0.752709571352447,
0.878649898165962,1.),.UNSPECIFIED.);
#1985=B_SPLINE_CURVE_WITH_KNOTS('',3,(#93995,#93996,#93997,#93998,#93999,
#94000,#94001,#94002,#94003,#94004,#94005,#94006,#94007,#94008,#94009,#94010,
#94011,#94012,#94013,#94014,#94015,#94016,#94017),.UNSPECIFIED.,.F.,.F.,
(4,2,2,2,3,2,2,2,2,2,4),(-0.00491026743302993,-0.00473849995762558,-0.00442749851885031,
-0.00379135806062017,0.,0.00898521807370431,0.01430350641162,0.0224007619062803,
0.0339277546976348,0.0458917612396366,0.0502751707719722),.UNSPECIFIED.);
#1986=B_SPLINE_CURVE_WITH_KNOTS('',3,(#94032,#94033,#94034,#94035,#94036,
#94037,#94038,#94039,#94040,#94041,#94042,#94043,#94044,#94045,#94046,#94047),
 .UNSPECIFIED.,.F.,.F.,(4,2,2,2,2,2,2,4),(-0.120393885459129,-0.119994183646075,
-0.114665415333723,-0.109375283203773,-0.103435268329857,-0.0955923543424567,
-0.0900172452535582,-0.0812505338475646),.UNSPECIFIED.);
#1987=B_SPLINE_CURVE_WITH_KNOTS('',3,(#94132,#94133,#94134,#94135,#94136,
#94137,#94138,#94139,#94140,#94141,#94142,#94143,#94144,#94145,#94146,#94147,
#94148,#94149,#94150,#94151,#94152,#94153,#94154,#94155,#94156,#94157,#94158,
#94159,#94160,#94161,#94162,#94163,#94164,#94165,#94166,#94167,#94168,#94169,
#94170,#94171,#94172,#94173,#94174,#94175,#94176,#94177,#94178,#94179,#94180,
#94181,#94182,#94183,#94184,#94185,#94186,#94187,#94188,#94189,#94190,#94191,
#94192,#94193,#94194,#94195,#94196,#94197,#94198,#94199,#94200,#94201,#94202,
#94203,#94204),.UNSPECIFIED.,.F.,.F.,(4,3,3,3,3,3,3,3,3,3,3,3,3,3,3,3,3,
3,3,3,3,3,3,3,4),(0.,0.0392604588675547,0.0796928782844232,0.121900173659216,
0.124999999999999,0.170760900465759,0.187499999999994,0.218749999999994,
0.234374999999993,0.248731529201415,0.249999999999993,0.315888335880771,
0.375000000000004,0.437500000000008,0.462804796365139,0.489494576915244,
0.500000000000012,0.596805346167588,0.625000000000016,0.666607772440218,
0.70933182444373,0.75000000000002,0.841508009635831,0.936057229296371,1.),
 .UNSPECIFIED.);
#1988=B_SPLINE_CURVE_WITH_KNOTS('',3,(#94232,#94233,#94234,#94235,#94236,
#94237,#94238,#94239,#94240,#94241,#94242,#94243,#94244,#94245,#94246,#94247,
#94248,#94249,#94250,#94251,#94252,#94253,#94254,#94255,#94256,#94257,#94258,
#94259,#94260,#94261,#94262,#94263,#94264,#94265,#94266,#94267,#94268,#94269,
#94270,#94271),.UNSPECIFIED.,.F.,.F.,(4,3,3,3,3,3,3,3,3,3,3,3,3,4),(0.,
0.0879907258885037,0.106017412003521,0.203661923636243,0.212034824007045,
0.318052236010566,0.424069648014091,0.530087060017611,0.636104472021133,
0.699133885047539,0.756356915627061,0.859124793049096,0.929561688516431,
1.),.UNSPECIFIED.);
#1989=B_SPLINE_CURVE_WITH_KNOTS('',3,(#94310,#94311,#94312,#94313,#94314,
#94315,#94316,#94317,#94318,#94319,#94320,#94321,#94322,#94323,#94324,#94325,
#94326,#94327,#94328,#94329,#94330,#94331),.UNSPECIFIED.,.F.,.F.,(4,2,2,
1,1,2,2,2,1,1,2,2,4),(0.,0.250000000000018,0.375000000000027,0.437500000000035,
0.468750000000039,0.484375000000039,0.500000000000038,0.625000000000014,
0.687500000000002,0.71874999999999,0.734374999999992,0.749999999999994,
1.),.UNSPECIFIED.);
#1990=B_SPLINE_CURVE_WITH_KNOTS('',3,(#94333,#94334,#94335,#94336,#94337,
#94338,#94339,#94340,#94341,#94342,#94343,#94344,#94345,#94346,#94347,#94348,
#94349,#94350,#94351,#94352,#94353,#94354,#94355,#94356,#94357,#94358,#94359,
#94360,#94361,#94362,#94363,#94364,#94365,#94366,#94367,#94368,#94369,#94370,
#94371,#94372,#94373,#94374,#94375,#94376,#94377,#94378,#94379,#94380,#94381,
#94382,#94383,#94384,#94385,#94386,#94387,#94388,#94389,#94390,#94391,#94392,
#94393,#94394,#94395,#94396,#94397,#94398,#94399,#94400,#94401,#94402),
 .UNSPECIFIED.,.F.,.F.,(4,3,3,3,3,3,3,3,3,3,3,3,3,3,3,3,3,3,3,3,3,3,3,4),
(0.,0.0421685283686954,0.0866369744043819,0.125000000000004,0.17094832665189,
0.187500000000006,0.218750000000007,0.234375000000007,0.249140524228546,
0.250000000000008,0.321912311030012,0.37500000000001,0.437500000000019,
0.463805676895858,0.491767464400642,0.500000000000027,0.610538966377814,
0.62500000000002,0.669599302244168,0.715427682662428,0.750000000000014,
0.84562680526609,0.943611528143267,1.),.UNSPECIFIED.);
#1991=B_SPLINE_CURVE_WITH_KNOTS('',3,(#94457,#94458,#94459,#94460,#94461,
#94462,#94463,#94464,#94465,#94466,#94467,#94468,#94469,#94470,#94471,#94472,
#94473,#94474,#94475,#94476,#94477,#94478,#94479,#94480,#94481,#94482,#94483,
#94484,#94485,#94486,#94487,#94488,#94489,#94490,#94491,#94492,#94493,#94494,
#94495,#94496,#94497,#94498,#94499,#94500,#94501,#94502,#94503,#94504,#94505,
#94506,#94507,#94508,#94509,#94510,#94511,#94512,#94513,#94514,#94515,#94516,
#94517,#94518,#94519,#94520,#94521,#94522,#94523,#94524,#94525,#94526,#94527,
#94528,#94529,#94530,#94531,#94532,#94533,#94534,#94535,#94536,#94537,#94538,
#94539,#94540,#94541,#94542,#94543,#94544,#94545,#94546,#94547,#94548,#94549,
#94550,#94551,#94552,#94553,#94554,#94555,#94556,#94557,#94558,#94559,#94560,
#94561,#94562,#94563,#94564,#94565,#94566,#94567,#94568,#94569,#94570,#94571,
#94572,#94573,#94574,#94575,#94576,#94577,#94578,#94579,#94580,#94581,#94582,
#94583,#94584,#94585,#94586,#94587,#94588,#94589),.UNSPECIFIED.,.F.,.F.,
(4,3,3,3,3,3,3,3,3,3,3,3,3,3,3,3,3,3,3,3,3,3,3,3,3,3,3,3,3,3,3,3,3,3,3,
3,3,3,3,3,3,3,3,3,4),(0.,0.0624999999997391,0.086998109193101,0.11203275765394,
0.124999999999478,0.187499999999217,0.218749999999087,0.234374999999018,
0.242187499998983,0.247169612134524,0.249999999998949,0.277080795441728,
0.304102886341549,0.312499999998351,0.339182658907482,0.343749999998052,
0.359374999997902,0.367187499997823,0.371093749997786,0.373793883282339,
0.374999999997749,0.402703373425489,0.430374081715073,0.437499999998162,
0.464932402230747,0.468749999998366,0.484374999998472,0.492187499998521,
0.496849922230597,0.49999999999857,0.562499999998951,0.593749999999141,
0.609374999999225,0.618172379943541,0.62499999999931,0.649448676894499,
0.656249999999368,0.670823410234943,0.684559368754563,0.687499999999426,
0.713282747156612,0.741514803940786,0.749999999999541,0.912813131310412,
1.),.UNSPECIFIED.);
#1992=B_SPLINE_CURVE_WITH_KNOTS('',3,(#94624,#94625,#94626,#94627,#94628,
#94629,#94630,#94631,#94632,#94633,#94634,#94635,#94636,#94637,#94638,#94639,
#94640,#94641,#94642,#94643,#94644,#94645,#94646,#94647,#94648,#94649,#94650,
#94651,#94652,#94653,#94654,#94655,#94656,#94657,#94658,#94659,#94660,#94661,
#94662,#94663,#94664,#94665,#94666,#94667,#94668,#94669,#94670,#94671,#94672,
#94673,#94674,#94675,#94676,#94677,#94678),.UNSPECIFIED.,.F.,.F.,(4,3,3,
3,3,3,3,3,3,3,3,3,3,3,3,3,3,3,4),(0.,0.104226424951023,0.205570362215172,
0.250000000000015,0.348038393048773,0.375000000000023,0.437500000000026,
0.468750000000028,0.484375000000025,0.49311565096605,0.500000000000022,
0.578310819460716,0.654062706344688,0.726911775043978,0.795296105809942,
0.861362444821956,0.925281294150355,0.98649217487535,1.),.UNSPECIFIED.);
#1993=B_SPLINE_CURVE_WITH_KNOTS('',5,(#94810,#94811,#94812,#94813,#94814,
#94815,#94816,#94817,#94818,#94819,#94820,#94821,#94822,#94823,#94824,#94825,
#94826,#94827),.UNSPECIFIED.,.F.,.F.,(6,3,3,3,3,6),(0.,0.0563238113023862,
0.160203167534755,0.284130417633147,0.431668352740704,1.),.UNSPECIFIED.);
#1994=B_SPLINE_CURVE_WITH_KNOTS('',5,(#94904,#94905,#94906,#94907,#94908,
#94909,#94910,#94911,#94912),.UNSPECIFIED.,.F.,.F.,(6,3,6),(0.,0.5,1.),
 .UNSPECIFIED.);
#1995=B_SPLINE_CURVE_WITH_KNOTS('',3,(#95027,#95028,#95029,#95030,#95031,
#95032,#95033,#95034,#95035,#95036,#95037,#95038,#95039,#95040,#95041,#95042,
#95043,#95044,#95045,#95046,#95047,#95048,#95049,#95050,#95051,#95052,#95053,
#95054),.UNSPECIFIED.,.F.,.F.,(4,3,3,3,3,3,3,3,3,4),(0.,0.117491825204254,
0.243957063533135,0.37738327291059,0.43527831132456,0.5,0.625775888363041,
0.755819993836895,0.89307218585744,1.),.UNSPECIFIED.);
#1996=B_SPLINE_CURVE_WITH_KNOTS('',3,(#95115,#95116,#95117,#95118,#95119,
#95120,#95121,#95122,#95123,#95124,#95125,#95126,#95127,#95128,#95129,#95130,
#95131,#95132,#95133,#95134,#95135,#95136,#95137,#95138,#95139,#95140,#95141,
#95142,#95143,#95144,#95145,#95146,#95147,#95148,#95149,#95150,#95151,#95152,
#95153,#95154,#95155,#95156,#95157),.UNSPECIFIED.,.F.,.F.,(4,3,3,3,3,3,
3,3,3,3,3,3,3,3,4),(0.,0.0808464238153753,0.164273806551171,0.252181192896881,
0.34484059644842,0.437499999999959,0.468749999999961,0.484374999999962,
0.49822022793353,0.499999999999963,0.589386967039654,0.695533234255982,
0.797674047058454,0.898837023529225,0.999999999999996),.UNSPECIFIED.);
#1997=B_SPLINE_CURVE_WITH_KNOTS('',3,(#95198,#95199,#95200,#95201,#95202,
#95203,#95204,#95205,#95206,#95207,#95208,#95209,#95210,#95211,#95212,#95213,
#95214,#95215,#95216,#95217,#95218,#95219,#95220,#95221,#95222,#95223,#95224,
#95225,#95226,#95227,#95228,#95229,#95230,#95231,#95232,#95233,#95234,#95235,
#95236,#95237,#95238,#95239,#95240),.UNSPECIFIED.,.F.,.F.,(4,3,3,3,3,3,
3,3,3,3,3,3,3,3,4),(0.,0.0938007173938139,0.185901855972414,0.249999999999996,
0.343989025885857,0.374999999999996,0.437499999999994,0.46874999999999,
0.485689475824231,0.499999999999987,0.611288654097174,0.721466525856065,
0.831135504101467,0.939753775588306,1.),.UNSPECIFIED.);
#1998=B_SPLINE_CURVE_WITH_KNOTS('',3,(#95305,#95306,#95307,#95308,#95309,
#95310,#95311,#95312,#95313,#95314),.UNSPECIFIED.,.F.,.F.,(4,3,3,4),(0.,
0.143504699996,0.239445459249329,0.287009399992),.UNSPECIFIED.);
#1999=B_SPLINE_CURVE_WITH_KNOTS('',3,(#95315,#95316,#95317,#95318,#95319,
#95320,#95321,#95322,#95323,#95324),.UNSPECIFIED.,.F.,.F.,(4,3,3,4),(0.,
0.1405201788765,0.248883771899673,0.281040357753),.UNSPECIFIED.);
#2000=B_SPLINE_CURVE_WITH_KNOTS('',3,(#95380,#95381,#95382,#95383,#95384,
#95385,#95386,#95387,#95388,#95389,#95390,#95391,#95392,#95393,#95394,#95395,
#95396,#95397,#95398,#95399,#95400,#95401,#95402,#95403,#95404,#95405,#95406,
#95407,#95408,#95409,#95410),.UNSPECIFIED.,.F.,.F.,(4,3,3,3,3,3,3,3,3,3,
4),(0.,0.103606039248823,0.209200414239989,0.317311627182029,0.426434884947508,
0.535929191910942,0.645077668364674,0.752572851887113,0.858664995978984,
0.962443523493205,0.999999999821951),.UNSPECIFIED.);
#2001=B_SPLINE_CURVE_WITH_KNOTS('',3,(#95412,#95413,#95414,#95415,#95416,
#95417,#95418,#95419,#95420,#95421,#95422,#95423,#95424,#95425,#95426,#95427,
#95428,#95429,#95430,#95431,#95432,#95433,#95434,#95435,#95436,#95437,#95438,
#95439,#95440,#95441,#95442,#95443,#95444,#95445,#95446,#95447,#95448,#95449,
#95450,#95451,#95452,#95453,#95454,#95455,#95456,#95457,#95458,#95459,#95460,
#95461,#95462,#95463,#95464,#95465,#95466,#95467,#95468,#95469,#95470,#95471,
#95472,#95473,#95474,#95475,#95476,#95477,#95478,#95479,#95480,#95481,#95482,
#95483,#95484,#95485,#95486,#95487,#95488,#95489,#95490,#95491,#95492,#95493,
#95494,#95495,#95496,#95497,#95498,#95499,#95500,#95501,#95502),
 .UNSPECIFIED.,.F.,.F.,(4,3,3,3,3,3,3,3,3,3,3,3,3,3,3,3,3,3,3,3,3,3,3,3,
3,3,3,3,3,3,4),(0.,0.0913074651431097,0.114032014272892,0.126273024521462,
0.171275187346726,0.215654286164605,0.250000000000023,0.298193111621357,
0.344962894394445,0.375000000000034,0.437500000000026,0.445173235143761,
0.458879926357822,0.464179160278983,0.46791323451339,0.470646179065875,
0.486232403511859,0.500000000000003,0.55761265328308,0.613032492495676,
0.624999999999972,0.687499999999956,0.71874999999996,0.732930979089932,
0.745933459125306,0.749999999999964,0.825581397342451,0.901338193120674,
0.950669096560337,0.994252840936779,1.),.UNSPECIFIED.);
#2002=B_SPLINE_CURVE_WITH_KNOTS('',3,(#95640,#95641,#95642,#95643,#95644,
#95645,#95646,#95647,#95648,#95649,#95650,#95651,#95652,#95653,#95654,#95655,
#95656,#95657,#95658,#95659,#95660,#95661,#95662,#95663,#95664,#95665,#95666,
#95667,#95668,#95669,#95670,#95671,#95672,#95673,#95674,#95675,#95676,#95677,
#95678,#95679,#95680,#95681,#95682,#95683,#95684,#95685,#95686,#95687,#95688),
 .UNSPECIFIED.,.F.,.F.,(4,3,3,3,3,3,3,3,3,3,3,3,3,3,3,3,4),(0.,0.0625,0.127496392454565,
0.198782421033528,0.25,0.342193251507051,0.429444529148827,0.5,0.567975878480713,
0.632411656728602,0.69280772499897,0.75,0.806943791318981,0.86166436072903,
0.915319828375331,0.967555661113252,1.),.UNSPECIFIED.);
#2050=SHAPE_REPRESENTATION_RELATIONSHIP('SRR','None',#98347,#2060);
#2060=ADVANCED_BREP_SHAPE_REPRESENTATION('',(#2079),#98299);
#2070=STYLED_ITEM('',(#98399),#2079);
#2079=MANIFOLD_SOLID_BREP('Body1',#34176);
#2374=PLANE('',#36617);
#2375=PLANE('',#36627);
#2376=PLANE('',#36668);
#2377=PLANE('',#36671);
#2378=PLANE('',#36681);
#2379=PLANE('',#36723);
#2380=PLANE('',#36730);
#2381=PLANE('',#36773);
#2382=PLANE('',#36779);
#2383=PLANE('',#36786);
#2384=PLANE('',#36790);
#2385=PLANE('',#36795);
#2386=PLANE('',#36808);
#2387=PLANE('',#36819);
#2388=PLANE('',#36981);
#2389=PLANE('',#37029);
#2390=PLANE('',#37056);
#2391=PLANE('',#37059);
#2392=PLANE('',#37063);
#2393=PLANE('',#37070);
#2394=PLANE('',#37076);
#2395=PLANE('',#37079);
#2396=PLANE('',#37088);
#2397=PLANE('',#37098);
#2398=PLANE('',#37105);
#2399=PLANE('',#37106);
#2400=PLANE('',#37165);
#2401=PLANE('',#37248);
#2402=PLANE('',#37255);
#2403=PLANE('',#37297);
#2404=PLANE('',#37311);
#2405=PLANE('',#37321);
#2406=PLANE('',#37364);
#2407=PLANE('',#37367);
#2408=PLANE('',#37377);
#2409=PLANE('',#37409);
#2410=PLANE('',#37423);
#2411=PLANE('',#37430);
#2412=PLANE('',#37474);
#2413=PLANE('',#37483);
#2414=PLANE('',#37495);
#2415=PLANE('',#37499);
#2416=PLANE('',#37504);
#2417=PLANE('',#37520);
#2418=PLANE('',#37531);
#2419=PLANE('',#37693);
#2420=PLANE('',#37744);
#2421=PLANE('',#37776);
#2422=PLANE('',#37782);
#2423=PLANE('',#37794);
#2424=PLANE('',#37816);
#2425=PLANE('',#37818);
#2426=PLANE('',#37822);
#2427=PLANE('',#37829);
#2428=PLANE('',#37835);
#2429=PLANE('',#37838);
#2430=PLANE('',#37847);
#2431=PLANE('',#37857);
#2432=PLANE('',#37864);
#2433=PLANE('',#37865);
#2434=PLANE('',#37902);
#2435=PLANE('',#37925);
#2436=PLANE('',#37993);
#2437=PLANE('',#38035);
#2438=PLANE('',#38042);
#2439=PLANE('',#38087);
#2941=CYLINDRICAL_SURFACE('',#36603,0.3);
#2942=CYLINDRICAL_SURFACE('',#36606,13.516744254);
#2943=CYLINDRICAL_SURFACE('',#36610,0.3);
#2944=CYLINDRICAL_SURFACE('',#36612,0.300000000000001);
#2945=CYLINDRICAL_SURFACE('',#36614,0.3);
#2946=CYLINDRICAL_SURFACE('',#36618,0.3);
#2947=CYLINDRICAL_SURFACE('',#36621,13.516744254);
#2948=CYLINDRICAL_SURFACE('',#36624,0.3);
#2949=CYLINDRICAL_SURFACE('',#36629,0.3);
#2950=CYLINDRICAL_SURFACE('',#36638,0.3);
#2951=CYLINDRICAL_SURFACE('',#36658,0.3);
#2952=CYLINDRICAL_SURFACE('',#36667,0.300000000000002);
#2953=CYLINDRICAL_SURFACE('',#36672,0.3);
#2954=CYLINDRICAL_SURFACE('',#36675,13.6462109523);
#2955=CYLINDRICAL_SURFACE('',#36678,0.3);
#2956=CYLINDRICAL_SURFACE('',#36682,0.3);
#2957=CYLINDRICAL_SURFACE('',#36684,0.3);
#2958=CYLINDRICAL_SURFACE('',#36687,0.3);
#2959=CYLINDRICAL_SURFACE('',#36697,0.300000000000002);
#2960=CYLINDRICAL_SURFACE('',#36710,0.3);
#2961=CYLINDRICAL_SURFACE('',#36715,0.300000000000002);
#2962=CYLINDRICAL_SURFACE('',#36726,7.84541841273);
#2963=CYLINDRICAL_SURFACE('',#36733,14.6875296363);
#2964=CYLINDRICAL_SURFACE('',#36735,0.3);
#2965=CYLINDRICAL_SURFACE('',#36737,0.3);
#2966=CYLINDRICAL_SURFACE('',#36740,0.3);
#2967=CYLINDRICAL_SURFACE('',#36746,0.3);
#2968=CYLINDRICAL_SURFACE('',#36748,0.300000000000002);
#2969=CYLINDRICAL_SURFACE('',#36751,0.300000000000001);
#2970=CYLINDRICAL_SURFACE('',#36780,16.1875296363);
#2971=CYLINDRICAL_SURFACE('',#36788,0.3);
#2972=CYLINDRICAL_SURFACE('',#36793,0.3);
#2973=CYLINDRICAL_SURFACE('',#36797,0.3);
#2974=CYLINDRICAL_SURFACE('',#36806,0.3);
#2975=CYLINDRICAL_SURFACE('',#36810,0.3);
#2976=CYLINDRICAL_SURFACE('',#36813,7.84541841273);
#2977=CYLINDRICAL_SURFACE('',#36816,0.3);
#2978=CYLINDRICAL_SURFACE('',#36820,0.3);
#2979=CYLINDRICAL_SURFACE('',#36822,0.3);
#2980=CYLINDRICAL_SURFACE('',#36825,14.6875296363);
#2981=CYLINDRICAL_SURFACE('',#36828,0.3);
#2982=CYLINDRICAL_SURFACE('',#36840,0.300000000000002);
#2983=CYLINDRICAL_SURFACE('',#36858,0.300000000000002);
#2984=CYLINDRICAL_SURFACE('',#36887,0.3);
#2985=CYLINDRICAL_SURFACE('',#36904,0.299999999999999);
#2986=CYLINDRICAL_SURFACE('',#36922,0.300000000000002);
#2987=CYLINDRICAL_SURFACE('',#36923,0.3);
#2988=CYLINDRICAL_SURFACE('',#36925,0.300000000000002);
#2989=CYLINDRICAL_SURFACE('',#36945,0.3);
#2990=CYLINDRICAL_SURFACE('',#36969,12.5256279976);
#2991=CYLINDRICAL_SURFACE('',#36975,0.3);
#2992=CYLINDRICAL_SURFACE('',#37000,0.3);
#2993=CYLINDRICAL_SURFACE('',#37010,3.);
#2994=CYLINDRICAL_SURFACE('',#37018,0.3);
#2995=CYLINDRICAL_SURFACE('',#37019,0.3);
#2996=CYLINDRICAL_SURFACE('',#37025,0.3);
#2997=CYLINDRICAL_SURFACE('',#37027,0.3);
#2998=CYLINDRICAL_SURFACE('',#37031,0.3);
#2999=CYLINDRICAL_SURFACE('',#37034,0.299999999999999);
#3000=CYLINDRICAL_SURFACE('',#37046,0.3);
#3001=CYLINDRICAL_SURFACE('',#37060,5.19295371933);
#3002=CYLINDRICAL_SURFACE('',#37061,0.3);
#3003=CYLINDRICAL_SURFACE('',#37064,0.3);
#3004=CYLINDRICAL_SURFACE('',#37066,6.34541841273);
#3005=CYLINDRICAL_SURFACE('',#37068,0.3);
#3006=CYLINDRICAL_SURFACE('',#37069,0.3);
#3007=CYLINDRICAL_SURFACE('',#37071,6.34541841273);
#3008=CYLINDRICAL_SURFACE('',#37072,0.3);
#3009=CYLINDRICAL_SURFACE('',#37073,5.19295371933);
#3010=CYLINDRICAL_SURFACE('',#37074,0.3);
#3011=CYLINDRICAL_SURFACE('',#37075,0.3);
#3012=CYLINDRICAL_SURFACE('',#37077,5.19295371933);
#3013=CYLINDRICAL_SURFACE('',#37078,0.3);
#3014=CYLINDRICAL_SURFACE('',#37080,0.3);
#3015=CYLINDRICAL_SURFACE('',#37082,6.34541841273);
#3016=CYLINDRICAL_SURFACE('',#37084,0.3);
#3017=CYLINDRICAL_SURFACE('',#37086,0.3);
#3018=CYLINDRICAL_SURFACE('',#37097,0.300000000000002);
#3019=CYLINDRICAL_SURFACE('',#37107,0.3);
#3020=CYLINDRICAL_SURFACE('',#37108,0.685778366608);
#3021=CYLINDRICAL_SURFACE('',#37113,0.3);
#3022=CYLINDRICAL_SURFACE('',#37115,0.300000000000002);
#3023=CYLINDRICAL_SURFACE('',#37116,0.3);
#3024=CYLINDRICAL_SURFACE('',#37126,0.3);
#3025=CYLINDRICAL_SURFACE('',#37127,7.84541841273);
#3026=CYLINDRICAL_SURFACE('',#37131,0.3);
#3027=CYLINDRICAL_SURFACE('',#37143,0.300000000000002);
#3028=CYLINDRICAL_SURFACE('',#37157,0.3);
#3029=CYLINDRICAL_SURFACE('',#37158,14.6875296363);
#3030=CYLINDRICAL_SURFACE('',#37159,14.6875296363);
#3031=CYLINDRICAL_SURFACE('',#37160,0.3);
#3032=CYLINDRICAL_SURFACE('',#37164,0.300000000000002);
#3033=CYLINDRICAL_SURFACE('',#37166,0.300000000000002);
#3034=CYLINDRICAL_SURFACE('',#37168,0.299999999999999);
#3035=CYLINDRICAL_SURFACE('',#37179,0.3);
#3036=CYLINDRICAL_SURFACE('',#37199,0.300000000000002);
#3037=CYLINDRICAL_SURFACE('',#37202,0.3);
#3038=CYLINDRICAL_SURFACE('',#37204,0.299999999999999);
#3039=CYLINDRICAL_SURFACE('',#37219,0.3);
#3040=CYLINDRICAL_SURFACE('',#37235,0.300000000000002);
#3041=CYLINDRICAL_SURFACE('',#37236,14.6875296363);
#3042=CYLINDRICAL_SURFACE('',#37238,0.999999999999999);
#3043=CYLINDRICAL_SURFACE('',#37240,14.6875296363);
#3044=CYLINDRICAL_SURFACE('',#37242,0.3);
#3045=CYLINDRICAL_SURFACE('',#37244,14.6875296363);
#3046=CYLINDRICAL_SURFACE('',#37246,0.3);
#3047=CYLINDRICAL_SURFACE('',#37249,0.3);
#3048=CYLINDRICAL_SURFACE('',#37251,7.84541841273);
#3049=CYLINDRICAL_SURFACE('',#37253,0.3);
#3050=CYLINDRICAL_SURFACE('',#37256,0.3);
#3051=CYLINDRICAL_SURFACE('',#37279,0.3);
#3052=CYLINDRICAL_SURFACE('',#37286,0.300000000000002);
#3053=CYLINDRICAL_SURFACE('',#37287,0.3);
#3054=CYLINDRICAL_SURFACE('',#37298,0.3);
#3055=CYLINDRICAL_SURFACE('',#37301,13.516744254);
#3056=CYLINDRICAL_SURFACE('',#37305,0.3);
#3057=CYLINDRICAL_SURFACE('',#37307,0.300000000000001);
#3058=CYLINDRICAL_SURFACE('',#37309,0.3);
#3059=CYLINDRICAL_SURFACE('',#37312,0.3);
#3060=CYLINDRICAL_SURFACE('',#37315,13.516744254);
#3061=CYLINDRICAL_SURFACE('',#37318,0.3);
#3062=CYLINDRICAL_SURFACE('',#37323,0.3);
#3063=CYLINDRICAL_SURFACE('',#37333,0.3);
#3064=CYLINDRICAL_SURFACE('',#37353,0.3);
#3065=CYLINDRICAL_SURFACE('',#37362,0.300000000000002);
#3066=CYLINDRICAL_SURFACE('',#37368,0.3);
#3067=CYLINDRICAL_SURFACE('',#37371,13.6462109523);
#3068=CYLINDRICAL_SURFACE('',#37374,0.3);
#3069=CYLINDRICAL_SURFACE('',#37378,0.3);
#3070=CYLINDRICAL_SURFACE('',#37381,0.3);
#3071=CYLINDRICAL_SURFACE('',#37384,0.3);
#3072=CYLINDRICAL_SURFACE('',#37394,0.300000000000002);
#3073=CYLINDRICAL_SURFACE('',#37410,0.3);
#3074=CYLINDRICAL_SURFACE('',#37416,0.300000000000002);
#3075=CYLINDRICAL_SURFACE('',#37426,7.84541841273);
#3076=CYLINDRICAL_SURFACE('',#37433,14.6875296363);
#3077=CYLINDRICAL_SURFACE('',#37435,0.3);
#3078=CYLINDRICAL_SURFACE('',#37437,0.3);
#3079=CYLINDRICAL_SURFACE('',#37440,0.3);
#3080=CYLINDRICAL_SURFACE('',#37446,0.3);
#3081=CYLINDRICAL_SURFACE('',#37448,0.300000000000002);
#3082=CYLINDRICAL_SURFACE('',#37451,0.300000000000001);
#3083=CYLINDRICAL_SURFACE('',#37480,0.3);
#3084=CYLINDRICAL_SURFACE('',#37484,3.);
#3085=CYLINDRICAL_SURFACE('',#37486,16.1875296363);
#3086=CYLINDRICAL_SURFACE('',#37492,0.3);
#3087=CYLINDRICAL_SURFACE('',#37497,0.3);
#3088=CYLINDRICAL_SURFACE('',#37502,0.3);
#3089=CYLINDRICAL_SURFACE('',#37505,0.3);
#3090=CYLINDRICAL_SURFACE('',#37514,15.6875296363);
#3091=CYLINDRICAL_SURFACE('',#37518,0.3);
#3092=CYLINDRICAL_SURFACE('',#37522,0.3);
#3093=CYLINDRICAL_SURFACE('',#37525,7.84541841273);
#3094=CYLINDRICAL_SURFACE('',#37528,0.3);
#3095=CYLINDRICAL_SURFACE('',#37532,0.3);
#3096=CYLINDRICAL_SURFACE('',#37534,0.3);
#3097=CYLINDRICAL_SURFACE('',#37537,14.6875296363);
#3098=CYLINDRICAL_SURFACE('',#37540,0.3);
#3099=CYLINDRICAL_SURFACE('',#37552,0.300000000000002);
#3100=CYLINDRICAL_SURFACE('',#37570,0.300000000000002);
#3101=CYLINDRICAL_SURFACE('',#37598,0.3);
#3102=CYLINDRICAL_SURFACE('',#37615,0.299999999999999);
#3103=CYLINDRICAL_SURFACE('',#37633,0.300000000000002);
#3104=CYLINDRICAL_SURFACE('',#37634,0.3);
#3105=CYLINDRICAL_SURFACE('',#37635,0.300000000000002);
#3106=CYLINDRICAL_SURFACE('',#37655,0.3);
#3107=CYLINDRICAL_SURFACE('',#37678,1.);
#3108=CYLINDRICAL_SURFACE('',#37680,12.5256279976);
#3109=CYLINDRICAL_SURFACE('',#37686,0.3);
#3110=CYLINDRICAL_SURFACE('',#37704,0.0999999999999999);
#3111=CYLINDRICAL_SURFACE('',#37707,0.0999999999999999);
#3112=CYLINDRICAL_SURFACE('',#37713,0.0999999999999999);
#3113=CYLINDRICAL_SURFACE('',#37718,0.0999999999999999);
#3114=CYLINDRICAL_SURFACE('',#37725,0.0999999999999994);
#3115=CYLINDRICAL_SURFACE('',#37730,0.0999999999999994);
#3116=CYLINDRICAL_SURFACE('',#37735,0.0999999999999994);
#3117=CYLINDRICAL_SURFACE('',#37740,0.0999999999999994);
#3118=CYLINDRICAL_SURFACE('',#37754,0.3);
#3119=CYLINDRICAL_SURFACE('',#37763,3.);
#3120=CYLINDRICAL_SURFACE('',#37771,0.3);
#3121=CYLINDRICAL_SURFACE('',#37772,0.3);
#3122=CYLINDRICAL_SURFACE('',#37774,0.300000000000002);
#3123=CYLINDRICAL_SURFACE('',#37777,0.300000000000002);
#3124=CYLINDRICAL_SURFACE('',#37791,0.3);
#3125=CYLINDRICAL_SURFACE('',#37793,0.3);
#3126=CYLINDRICAL_SURFACE('',#37795,0.3);
#3127=CYLINDRICAL_SURFACE('',#37798,0.299999999999999);
#3128=CYLINDRICAL_SURFACE('',#37808,0.3);
#3129=CYLINDRICAL_SURFACE('',#37819,5.19295371933);
#3130=CYLINDRICAL_SURFACE('',#37820,0.3);
#3131=CYLINDRICAL_SURFACE('',#37823,0.3);
#3132=CYLINDRICAL_SURFACE('',#37825,6.34541841273);
#3133=CYLINDRICAL_SURFACE('',#37827,0.3);
#3134=CYLINDRICAL_SURFACE('',#37828,0.3);
#3135=CYLINDRICAL_SURFACE('',#37830,6.34541841273);
#3136=CYLINDRICAL_SURFACE('',#37831,0.3);
#3137=CYLINDRICAL_SURFACE('',#37832,5.19295371933);
#3138=CYLINDRICAL_SURFACE('',#37833,0.3);
#3139=CYLINDRICAL_SURFACE('',#37834,0.3);
#3140=CYLINDRICAL_SURFACE('',#37836,5.19295371933);
#3141=CYLINDRICAL_SURFACE('',#37837,0.3);
#3142=CYLINDRICAL_SURFACE('',#37839,0.3);
#3143=CYLINDRICAL_SURFACE('',#37841,6.34541841273);
#3144=CYLINDRICAL_SURFACE('',#37843,0.3);
#3145=CYLINDRICAL_SURFACE('',#37845,0.3);
#3146=CYLINDRICAL_SURFACE('',#37856,0.300000000000002);
#3147=CYLINDRICAL_SURFACE('',#37866,0.3);
#3148=CYLINDRICAL_SURFACE('',#37867,0.685778366608);
#3149=CYLINDRICAL_SURFACE('',#37872,0.3);
#3150=CYLINDRICAL_SURFACE('',#37874,0.300000000000002);
#3151=CYLINDRICAL_SURFACE('',#37875,0.3);
#3152=CYLINDRICAL_SURFACE('',#37883,0.3);
#3153=CYLINDRICAL_SURFACE('',#37884,7.84541841273);
#3154=CYLINDRICAL_SURFACE('',#37888,0.3);
#3155=CYLINDRICAL_SURFACE('',#37900,0.300000000000002);
#3156=CYLINDRICAL_SURFACE('',#37916,0.3);
#3157=CYLINDRICAL_SURFACE('',#37917,14.6875296363);
#3158=CYLINDRICAL_SURFACE('',#37918,0.999999999999999);
#3159=CYLINDRICAL_SURFACE('',#37919,14.6875296363);
#3160=CYLINDRICAL_SURFACE('',#37920,0.3);
#3161=CYLINDRICAL_SURFACE('',#37924,0.300000000000002);
#3162=CYLINDRICAL_SURFACE('',#37926,0.300000000000002);
#3163=CYLINDRICAL_SURFACE('',#37928,0.299999999999999);
#3164=CYLINDRICAL_SURFACE('',#37939,0.3);
#3165=CYLINDRICAL_SURFACE('',#37959,0.300000000000002);
#3166=CYLINDRICAL_SURFACE('',#37962,0.3);
#3167=CYLINDRICAL_SURFACE('',#37964,0.299999999999999);
#3168=CYLINDRICAL_SURFACE('',#37969,0.0999999999999994);
#3169=CYLINDRICAL_SURFACE('',#37972,0.0999999999999994);
#3170=CYLINDRICAL_SURFACE('',#37974,0.0999999999999994);
#3171=CYLINDRICAL_SURFACE('',#37975,0.0999999999999994);
#3172=CYLINDRICAL_SURFACE('',#37982,0.0999999999999999);
#3173=CYLINDRICAL_SURFACE('',#37987,0.0999999999999999);
#3174=CYLINDRICAL_SURFACE('',#37988,0.0999999999999999);
#3175=CYLINDRICAL_SURFACE('',#37989,0.0999999999999999);
#3176=CYLINDRICAL_SURFACE('',#38009,0.3);
#3177=CYLINDRICAL_SURFACE('',#38022,0.300000000000002);
#3178=CYLINDRICAL_SURFACE('',#38023,14.6875296363);
#3179=CYLINDRICAL_SURFACE('',#38025,0.999999999999999);
#3180=CYLINDRICAL_SURFACE('',#38027,14.6875296363);
#3181=CYLINDRICAL_SURFACE('',#38029,0.3);
#3182=CYLINDRICAL_SURFACE('',#38031,14.6875296363);
#3183=CYLINDRICAL_SURFACE('',#38033,0.3);
#3184=CYLINDRICAL_SURFACE('',#38036,0.3);
#3185=CYLINDRICAL_SURFACE('',#38038,7.84541841273);
#3186=CYLINDRICAL_SURFACE('',#38040,0.3);
#3187=CYLINDRICAL_SURFACE('',#38043,0.3);
#3188=CYLINDRICAL_SURFACE('',#38067,0.3);
#3189=CYLINDRICAL_SURFACE('',#38076,0.300000000000002);
#3190=CYLINDRICAL_SURFACE('',#38077,0.3);
#4537=FACE_OUTER_BOUND('',#6732,.T.);
#4538=FACE_OUTER_BOUND('',#6733,.T.);
#4539=FACE_OUTER_BOUND('',#6734,.T.);
#4540=FACE_OUTER_BOUND('',#6735,.T.);
#4541=FACE_OUTER_BOUND('',#6736,.T.);
#4542=FACE_OUTER_BOUND('',#6737,.T.);
#4543=FACE_OUTER_BOUND('',#6738,.T.);
#4544=FACE_OUTER_BOUND('',#6739,.T.);
#4545=FACE_OUTER_BOUND('',#6740,.T.);
#4546=FACE_OUTER_BOUND('',#6741,.T.);
#4547=FACE_OUTER_BOUND('',#6742,.T.);
#4548=FACE_OUTER_BOUND('',#6743,.T.);
#4549=FACE_OUTER_BOUND('',#6744,.T.);
#4550=FACE_OUTER_BOUND('',#6745,.T.);
#4551=FACE_OUTER_BOUND('',#6746,.T.);
#4552=FACE_OUTER_BOUND('',#6747,.T.);
#4553=FACE_OUTER_BOUND('',#6748,.T.);
#4554=FACE_OUTER_BOUND('',#6749,.T.);
#4555=FACE_OUTER_BOUND('',#6750,.T.);
#4556=FACE_OUTER_BOUND('',#6751,.T.);
#4557=FACE_OUTER_BOUND('',#6752,.T.);
#4558=FACE_OUTER_BOUND('',#6753,.T.);
#4559=FACE_OUTER_BOUND('',#6754,.T.);
#4560=FACE_OUTER_BOUND('',#6755,.T.);
#4561=FACE_OUTER_BOUND('',#6756,.T.);
#4562=FACE_OUTER_BOUND('',#6757,.T.);
#4563=FACE_OUTER_BOUND('',#6758,.T.);
#4564=FACE_OUTER_BOUND('',#6759,.T.);
#4565=FACE_OUTER_BOUND('',#6760,.T.);
#4566=FACE_OUTER_BOUND('',#6761,.T.);
#4567=FACE_OUTER_BOUND('',#6762,.T.);
#4568=FACE_OUTER_BOUND('',#6763,.T.);
#4569=FACE_OUTER_BOUND('',#6764,.T.);
#4570=FACE_OUTER_BOUND('',#6765,.T.);
#4571=FACE_OUTER_BOUND('',#6766,.T.);
#4572=FACE_OUTER_BOUND('',#6767,.T.);
#4573=FACE_OUTER_BOUND('',#6768,.T.);
#4574=FACE_OUTER_BOUND('',#6769,.T.);
#4575=FACE_OUTER_BOUND('',#6770,.T.);
#4576=FACE_OUTER_BOUND('',#6771,.T.);
#4577=FACE_OUTER_BOUND('',#6772,.T.);
#4578=FACE_OUTER_BOUND('',#6773,.T.);
#4579=FACE_OUTER_BOUND('',#6774,.T.);
#4580=FACE_OUTER_BOUND('',#6775,.T.);
#4581=FACE_OUTER_BOUND('',#6776,.T.);
#4582=FACE_OUTER_BOUND('',#6777,.T.);
#4583=FACE_OUTER_BOUND('',#6778,.T.);
#4584=FACE_OUTER_BOUND('',#6779,.T.);
#4585=FACE_OUTER_BOUND('',#6780,.T.);
#4586=FACE_OUTER_BOUND('',#6781,.T.);
#4587=FACE_OUTER_BOUND('',#6782,.T.);
#4588=FACE_OUTER_BOUND('',#6783,.T.);
#4589=FACE_OUTER_BOUND('',#6784,.T.);
#4590=FACE_OUTER_BOUND('',#6785,.T.);
#4591=FACE_OUTER_BOUND('',#6786,.T.);
#4592=FACE_OUTER_BOUND('',#6787,.T.);
#4593=FACE_OUTER_BOUND('',#6788,.T.);
#4594=FACE_OUTER_BOUND('',#6789,.T.);
#4595=FACE_OUTER_BOUND('',#6790,.T.);
#4596=FACE_OUTER_BOUND('',#6791,.T.);
#4597=FACE_OUTER_BOUND('',#6792,.T.);
#4598=FACE_OUTER_BOUND('',#6793,.T.);
#4599=FACE_OUTER_BOUND('',#6794,.T.);
#4600=FACE_OUTER_BOUND('',#6795,.T.);
#4601=FACE_OUTER_BOUND('',#6796,.T.);
#4602=FACE_OUTER_BOUND('',#6797,.T.);
#4603=FACE_OUTER_BOUND('',#6798,.T.);
#4604=FACE_OUTER_BOUND('',#6799,.T.);
#4605=FACE_OUTER_BOUND('',#6800,.T.);
#4606=FACE_OUTER_BOUND('',#6801,.T.);
#4607=FACE_OUTER_BOUND('',#6802,.T.);
#4608=FACE_OUTER_BOUND('',#6803,.T.);
#4609=FACE_OUTER_BOUND('',#6804,.T.);
#4610=FACE_OUTER_BOUND('',#6805,.T.);
#4611=FACE_OUTER_BOUND('',#6806,.T.);
#4612=FACE_OUTER_BOUND('',#6807,.T.);
#4613=FACE_OUTER_BOUND('',#6808,.T.);
#4614=FACE_OUTER_BOUND('',#6809,.T.);
#4615=FACE_OUTER_BOUND('',#6810,.T.);
#4616=FACE_OUTER_BOUND('',#6811,.T.);
#4617=FACE_OUTER_BOUND('',#6812,.T.);
#4618=FACE_OUTER_BOUND('',#6813,.T.);
#4619=FACE_OUTER_BOUND('',#6814,.T.);
#4620=FACE_OUTER_BOUND('',#6815,.T.);
#4621=FACE_OUTER_BOUND('',#6816,.T.);
#4622=FACE_OUTER_BOUND('',#6817,.T.);
#4623=FACE_OUTER_BOUND('',#6818,.T.);
#4624=FACE_OUTER_BOUND('',#6819,.T.);
#4625=FACE_OUTER_BOUND('',#6820,.T.);
#4626=FACE_OUTER_BOUND('',#6821,.T.);
#4627=FACE_OUTER_BOUND('',#6822,.T.);
#4628=FACE_OUTER_BOUND('',#6823,.T.);
#4629=FACE_OUTER_BOUND('',#6824,.T.);
#4630=FACE_OUTER_BOUND('',#6825,.T.);
#4631=FACE_OUTER_BOUND('',#6826,.T.);
#4632=FACE_OUTER_BOUND('',#6827,.T.);
#4633=FACE_OUTER_BOUND('',#6828,.T.);
#4634=FACE_OUTER_BOUND('',#6829,.T.);
#4635=FACE_OUTER_BOUND('',#6830,.T.);
#4636=FACE_OUTER_BOUND('',#6831,.T.);
#4637=FACE_OUTER_BOUND('',#6832,.T.);
#4638=FACE_OUTER_BOUND('',#6833,.T.);
#4639=FACE_OUTER_BOUND('',#6834,.T.);
#4640=FACE_OUTER_BOUND('',#6835,.T.);
#4641=FACE_OUTER_BOUND('',#6836,.T.);
#4642=FACE_OUTER_BOUND('',#6837,.T.);
#4643=FACE_OUTER_BOUND('',#6838,.T.);
#4644=FACE_OUTER_BOUND('',#6839,.T.);
#4645=FACE_OUTER_BOUND('',#6840,.T.);
#4646=FACE_OUTER_BOUND('',#6841,.T.);
#4647=FACE_OUTER_BOUND('',#6842,.T.);
#4648=FACE_OUTER_BOUND('',#6843,.T.);
#4649=FACE_OUTER_BOUND('',#6844,.T.);
#4650=FACE_OUTER_BOUND('',#6845,.T.);
#4651=FACE_OUTER_BOUND('',#6846,.T.);
#4652=FACE_OUTER_BOUND('',#6847,.T.);
#4653=FACE_OUTER_BOUND('',#6848,.T.);
#4654=FACE_OUTER_BOUND('',#6849,.T.);
#4655=FACE_OUTER_BOUND('',#6850,.T.);
#4656=FACE_OUTER_BOUND('',#6851,.T.);
#4657=FACE_OUTER_BOUND('',#6852,.T.);
#4658=FACE_OUTER_BOUND('',#6853,.T.);
#4659=FACE_OUTER_BOUND('',#6854,.T.);
#4660=FACE_OUTER_BOUND('',#6855,.T.);
#4661=FACE_OUTER_BOUND('',#6856,.T.);
#4662=FACE_OUTER_BOUND('',#6857,.T.);
#4663=FACE_OUTER_BOUND('',#6858,.T.);
#4664=FACE_OUTER_BOUND('',#6859,.T.);
#4665=FACE_OUTER_BOUND('',#6860,.T.);
#4666=FACE_OUTER_BOUND('',#6861,.T.);
#4667=FACE_OUTER_BOUND('',#6862,.T.);
#4668=FACE_OUTER_BOUND('',#6863,.T.);
#4669=FACE_OUTER_BOUND('',#6864,.T.);
#4670=FACE_OUTER_BOUND('',#6865,.T.);
#4671=FACE_OUTER_BOUND('',#6866,.T.);
#4672=FACE_OUTER_BOUND('',#6867,.T.);
#4673=FACE_OUTER_BOUND('',#6868,.T.);
#4674=FACE_OUTER_BOUND('',#6869,.T.);
#4675=FACE_OUTER_BOUND('',#6870,.T.);
#4676=FACE_OUTER_BOUND('',#6871,.T.);
#4677=FACE_OUTER_BOUND('',#6872,.T.);
#4678=FACE_OUTER_BOUND('',#6873,.T.);
#4679=FACE_OUTER_BOUND('',#6874,.T.);
#4680=FACE_OUTER_BOUND('',#6875,.T.);
#4681=FACE_OUTER_BOUND('',#6876,.T.);
#4682=FACE_OUTER_BOUND('',#6877,.T.);
#4683=FACE_OUTER_BOUND('',#6878,.T.);
#4684=FACE_OUTER_BOUND('',#6879,.T.);
#4685=FACE_OUTER_BOUND('',#6880,.T.);
#4686=FACE_OUTER_BOUND('',#6881,.T.);
#4687=FACE_OUTER_BOUND('',#6882,.T.);
#4688=FACE_OUTER_BOUND('',#6883,.T.);
#4689=FACE_OUTER_BOUND('',#6884,.T.);
#4690=FACE_OUTER_BOUND('',#6885,.T.);
#4691=FACE_OUTER_BOUND('',#6886,.T.);
#4692=FACE_OUTER_BOUND('',#6887,.T.);
#4693=FACE_OUTER_BOUND('',#6888,.T.);
#4694=FACE_OUTER_BOUND('',#6889,.T.);
#4695=FACE_OUTER_BOUND('',#6890,.T.);
#4696=FACE_OUTER_BOUND('',#6891,.T.);
#4697=FACE_OUTER_BOUND('',#6892,.T.);
#4698=FACE_OUTER_BOUND('',#6893,.T.);
#4699=FACE_OUTER_BOUND('',#6894,.T.);
#4700=FACE_OUTER_BOUND('',#6895,.T.);
#4701=FACE_OUTER_BOUND('',#6896,.T.);
#4702=FACE_OUTER_BOUND('',#6897,.T.);
#4703=FACE_OUTER_BOUND('',#6898,.T.);
#4704=FACE_OUTER_BOUND('',#6899,.T.);
#4705=FACE_OUTER_BOUND('',#6900,.T.);
#4706=FACE_OUTER_BOUND('',#6901,.T.);
#4707=FACE_OUTER_BOUND('',#6902,.T.);
#4708=FACE_OUTER_BOUND('',#6903,.T.);
#4709=FACE_OUTER_BOUND('',#6904,.T.);
#4710=FACE_OUTER_BOUND('',#6905,.T.);
#4711=FACE_OUTER_BOUND('',#6906,.T.);
#4712=FACE_OUTER_BOUND('',#6907,.T.);
#4713=FACE_OUTER_BOUND('',#6908,.T.);
#4714=FACE_OUTER_BOUND('',#6909,.T.);
#4715=FACE_OUTER_BOUND('',#6910,.T.);
#4716=FACE_OUTER_BOUND('',#6911,.T.);
#4717=FACE_OUTER_BOUND('',#6912,.T.);
#4718=FACE_OUTER_BOUND('',#6913,.T.);
#4719=FACE_OUTER_BOUND('',#6914,.T.);
#4720=FACE_OUTER_BOUND('',#6915,.T.);
#4721=FACE_OUTER_BOUND('',#6916,.T.);
#4722=FACE_OUTER_BOUND('',#6917,.T.);
#4723=FACE_OUTER_BOUND('',#6918,.T.);
#4724=FACE_OUTER_BOUND('',#6919,.T.);
#4725=FACE_OUTER_BOUND('',#6920,.T.);
#4726=FACE_OUTER_BOUND('',#6921,.T.);
#4727=FACE_OUTER_BOUND('',#6922,.T.);
#4728=FACE_OUTER_BOUND('',#6923,.T.);
#4729=FACE_OUTER_BOUND('',#6924,.T.);
#4730=FACE_OUTER_BOUND('',#6925,.T.);
#4731=FACE_OUTER_BOUND('',#6926,.T.);
#4732=FACE_OUTER_BOUND('',#6927,.T.);
#4733=FACE_OUTER_BOUND('',#6928,.T.);
#4734=FACE_OUTER_BOUND('',#6929,.T.);
#4735=FACE_OUTER_BOUND('',#6930,.T.);
#4736=FACE_OUTER_BOUND('',#6931,.T.);
#4737=FACE_OUTER_BOUND('',#6932,.T.);
#4738=FACE_OUTER_BOUND('',#6933,.T.);
#4739=FACE_OUTER_BOUND('',#6934,.T.);
#4740=FACE_OUTER_BOUND('',#6935,.T.);
#4741=FACE_OUTER_BOUND('',#6936,.T.);
#4742=FACE_OUTER_BOUND('',#6937,.T.);
#4743=FACE_OUTER_BOUND('',#6938,.T.);
#4744=FACE_OUTER_BOUND('',#6939,.T.);
#4745=FACE_OUTER_BOUND('',#6940,.T.);
#4746=FACE_OUTER_BOUND('',#6941,.T.);
#4747=FACE_OUTER_BOUND('',#6942,.T.);
#4748=FACE_OUTER_BOUND('',#6943,.T.);
#4749=FACE_OUTER_BOUND('',#6944,.T.);
#4750=FACE_OUTER_BOUND('',#6945,.T.);
#4751=FACE_OUTER_BOUND('',#6946,.T.);
#4752=FACE_OUTER_BOUND('',#6947,.T.);
#4753=FACE_OUTER_BOUND('',#6948,.T.);
#4754=FACE_OUTER_BOUND('',#6949,.T.);
#4755=FACE_OUTER_BOUND('',#6950,.T.);
#4756=FACE_OUTER_BOUND('',#6951,.T.);
#4757=FACE_OUTER_BOUND('',#6952,.T.);
#4758=FACE_OUTER_BOUND('',#6953,.T.);
#4759=FACE_OUTER_BOUND('',#6954,.T.);
#4760=FACE_OUTER_BOUND('',#6955,.T.);
#4761=FACE_OUTER_BOUND('',#6956,.T.);
#4762=FACE_OUTER_BOUND('',#6957,.T.);
#4763=FACE_OUTER_BOUND('',#6958,.T.);
#4764=FACE_OUTER_BOUND('',#6959,.T.);
#4765=FACE_OUTER_BOUND('',#6960,.T.);
#4766=FACE_OUTER_BOUND('',#6961,.T.);
#4767=FACE_OUTER_BOUND('',#6962,.T.);
#4768=FACE_OUTER_BOUND('',#6963,.T.);
#4769=FACE_OUTER_BOUND('',#6964,.T.);
#4770=FACE_OUTER_BOUND('',#6965,.T.);
#4771=FACE_OUTER_BOUND('',#6966,.T.);
#4772=FACE_OUTER_BOUND('',#6967,.T.);
#4773=FACE_OUTER_BOUND('',#6968,.T.);
#4774=FACE_OUTER_BOUND('',#6969,.T.);
#4775=FACE_OUTER_BOUND('',#6970,.T.);
#4776=FACE_OUTER_BOUND('',#6971,.T.);
#4777=FACE_OUTER_BOUND('',#6972,.T.);
#4778=FACE_OUTER_BOUND('',#6973,.T.);
#4779=FACE_OUTER_BOUND('',#6974,.T.);
#4780=FACE_OUTER_BOUND('',#6975,.T.);
#4781=FACE_OUTER_BOUND('',#6976,.T.);
#4782=FACE_OUTER_BOUND('',#6977,.T.);
#4783=FACE_OUTER_BOUND('',#6978,.T.);
#4784=FACE_OUTER_BOUND('',#6979,.T.);
#4785=FACE_OUTER_BOUND('',#6980,.T.);
#4786=FACE_OUTER_BOUND('',#6981,.T.);
#4787=FACE_OUTER_BOUND('',#6982,.T.);
#4788=FACE_OUTER_BOUND('',#6983,.T.);
#4789=FACE_OUTER_BOUND('',#6984,.T.);
#4790=FACE_OUTER_BOUND('',#6985,.T.);
#4791=FACE_OUTER_BOUND('',#6986,.T.);
#4792=FACE_OUTER_BOUND('',#6987,.T.);
#4793=FACE_OUTER_BOUND('',#6988,.T.);
#4794=FACE_OUTER_BOUND('',#6989,.T.);
#4795=FACE_OUTER_BOUND('',#6990,.T.);
#4796=FACE_OUTER_BOUND('',#6991,.T.);
#4797=FACE_OUTER_BOUND('',#6992,.T.);
#4798=FACE_OUTER_BOUND('',#6993,.T.);
#4799=FACE_OUTER_BOUND('',#6994,.T.);
#4800=FACE_OUTER_BOUND('',#6995,.T.);
#4801=FACE_OUTER_BOUND('',#6996,.T.);
#4802=FACE_OUTER_BOUND('',#6997,.T.);
#4803=FACE_OUTER_BOUND('',#6998,.T.);
#4804=FACE_OUTER_BOUND('',#6999,.T.);
#4805=FACE_OUTER_BOUND('',#7000,.T.);
#4806=FACE_OUTER_BOUND('',#7001,.T.);
#4807=FACE_OUTER_BOUND('',#7002,.T.);
#4808=FACE_OUTER_BOUND('',#7003,.T.);
#4809=FACE_OUTER_BOUND('',#7004,.T.);
#4810=FACE_OUTER_BOUND('',#7005,.T.);
#4811=FACE_OUTER_BOUND('',#7006,.T.);
#4812=FACE_OUTER_BOUND('',#7007,.T.);
#4813=FACE_OUTER_BOUND('',#7008,.T.);
#4814=FACE_OUTER_BOUND('',#7009,.T.);
#4815=FACE_OUTER_BOUND('',#7010,.T.);
#4816=FACE_OUTER_BOUND('',#7011,.T.);
#4817=FACE_OUTER_BOUND('',#7012,.T.);
#4818=FACE_OUTER_BOUND('',#7013,.T.);
#4819=FACE_OUTER_BOUND('',#7014,.T.);
#4820=FACE_OUTER_BOUND('',#7015,.T.);
#4821=FACE_OUTER_BOUND('',#7016,.T.);
#4822=FACE_OUTER_BOUND('',#7017,.T.);
#4823=FACE_OUTER_BOUND('',#7018,.T.);
#4824=FACE_OUTER_BOUND('',#7019,.T.);
#4825=FACE_OUTER_BOUND('',#7020,.T.);
#4826=FACE_OUTER_BOUND('',#7021,.T.);
#4827=FACE_OUTER_BOUND('',#7022,.T.);
#4828=FACE_OUTER_BOUND('',#7023,.T.);
#4829=FACE_OUTER_BOUND('',#7024,.T.);
#4830=FACE_OUTER_BOUND('',#7025,.T.);
#4831=FACE_OUTER_BOUND('',#7026,.T.);
#4832=FACE_OUTER_BOUND('',#7027,.T.);
#4833=FACE_OUTER_BOUND('',#7028,.T.);
#4834=FACE_OUTER_BOUND('',#7029,.T.);
#4835=FACE_OUTER_BOUND('',#7030,.T.);
#4836=FACE_OUTER_BOUND('',#7031,.T.);
#4837=FACE_OUTER_BOUND('',#7032,.T.);
#4838=FACE_OUTER_BOUND('',#7033,.T.);
#4839=FACE_OUTER_BOUND('',#7034,.T.);
#4840=FACE_OUTER_BOUND('',#7035,.T.);
#4841=FACE_OUTER_BOUND('',#7036,.T.);
#4842=FACE_OUTER_BOUND('',#7037,.T.);
#4843=FACE_OUTER_BOUND('',#7038,.T.);
#4844=FACE_OUTER_BOUND('',#7039,.T.);
#4845=FACE_OUTER_BOUND('',#7040,.T.);
#4846=FACE_OUTER_BOUND('',#7041,.T.);
#4847=FACE_OUTER_BOUND('',#7042,.T.);
#4848=FACE_OUTER_BOUND('',#7043,.T.);
#4849=FACE_OUTER_BOUND('',#7044,.T.);
#4850=FACE_OUTER_BOUND('',#7045,.T.);
#4851=FACE_OUTER_BOUND('',#7046,.T.);
#4852=FACE_OUTER_BOUND('',#7047,.T.);
#4853=FACE_OUTER_BOUND('',#7048,.T.);
#4854=FACE_OUTER_BOUND('',#7049,.T.);
#4855=FACE_OUTER_BOUND('',#7050,.T.);
#4856=FACE_OUTER_BOUND('',#7051,.T.);
#4857=FACE_OUTER_BOUND('',#7052,.T.);
#4858=FACE_OUTER_BOUND('',#7053,.T.);
#4859=FACE_OUTER_BOUND('',#7054,.T.);
#4860=FACE_OUTER_BOUND('',#7055,.T.);
#4861=FACE_OUTER_BOUND('',#7056,.T.);
#4862=FACE_OUTER_BOUND('',#7057,.T.);
#4863=FACE_OUTER_BOUND('',#7058,.T.);
#4864=FACE_OUTER_BOUND('',#7059,.T.);
#4865=FACE_OUTER_BOUND('',#7060,.T.);
#4866=FACE_OUTER_BOUND('',#7061,.T.);
#4867=FACE_OUTER_BOUND('',#7062,.T.);
#4868=FACE_OUTER_BOUND('',#7063,.T.);
#4869=FACE_OUTER_BOUND('',#7064,.T.);
#4870=FACE_OUTER_BOUND('',#7065,.T.);
#4871=FACE_OUTER_BOUND('',#7066,.T.);
#4872=FACE_OUTER_BOUND('',#7067,.T.);
#4873=FACE_OUTER_BOUND('',#7068,.T.);
#4874=FACE_OUTER_BOUND('',#7069,.T.);
#4875=FACE_OUTER_BOUND('',#7070,.T.);
#4876=FACE_OUTER_BOUND('',#7071,.T.);
#4877=FACE_OUTER_BOUND('',#7072,.T.);
#4878=FACE_OUTER_BOUND('',#7073,.T.);
#4879=FACE_OUTER_BOUND('',#7074,.T.);
#4880=FACE_OUTER_BOUND('',#7075,.T.);
#4881=FACE_OUTER_BOUND('',#7076,.T.);
#4882=FACE_OUTER_BOUND('',#7077,.T.);
#4883=FACE_OUTER_BOUND('',#7078,.T.);
#4884=FACE_OUTER_BOUND('',#7079,.T.);
#4885=FACE_OUTER_BOUND('',#7080,.T.);
#4886=FACE_OUTER_BOUND('',#7081,.T.);
#4887=FACE_OUTER_BOUND('',#7082,.T.);
#4888=FACE_OUTER_BOUND('',#7083,.T.);
#4889=FACE_OUTER_BOUND('',#7084,.T.);
#4890=FACE_OUTER_BOUND('',#7085,.T.);
#4891=FACE_OUTER_BOUND('',#7086,.T.);
#4892=FACE_OUTER_BOUND('',#7087,.T.);
#4893=FACE_OUTER_BOUND('',#7088,.T.);
#4894=FACE_OUTER_BOUND('',#7089,.T.);
#4895=FACE_OUTER_BOUND('',#7090,.T.);
#4896=FACE_OUTER_BOUND('',#7091,.T.);
#4897=FACE_OUTER_BOUND('',#7092,.T.);
#4898=FACE_OUTER_BOUND('',#7093,.T.);
#4899=FACE_OUTER_BOUND('',#7094,.T.);
#4900=FACE_OUTER_BOUND('',#7095,.T.);
#4901=FACE_OUTER_BOUND('',#7096,.T.);
#4902=FACE_OUTER_BOUND('',#7097,.T.);
#4903=FACE_OUTER_BOUND('',#7098,.T.);
#4904=FACE_OUTER_BOUND('',#7099,.T.);
#4905=FACE_OUTER_BOUND('',#7100,.T.);
#4906=FACE_OUTER_BOUND('',#7101,.T.);
#4907=FACE_OUTER_BOUND('',#7102,.T.);
#4908=FACE_OUTER_BOUND('',#7103,.T.);
#4909=FACE_OUTER_BOUND('',#7104,.T.);
#4910=FACE_OUTER_BOUND('',#7105,.T.);
#4911=FACE_OUTER_BOUND('',#7106,.T.);
#4912=FACE_OUTER_BOUND('',#7107,.T.);
#4913=FACE_OUTER_BOUND('',#7108,.T.);
#4914=FACE_OUTER_BOUND('',#7109,.T.);
#4915=FACE_OUTER_BOUND('',#7110,.T.);
#4916=FACE_OUTER_BOUND('',#7111,.T.);
#4917=FACE_OUTER_BOUND('',#7112,.T.);
#4918=FACE_OUTER_BOUND('',#7113,.T.);
#4919=FACE_OUTER_BOUND('',#7114,.T.);
#4920=FACE_OUTER_BOUND('',#7115,.T.);
#4921=FACE_OUTER_BOUND('',#7116,.T.);
#4922=FACE_OUTER_BOUND('',#7117,.T.);
#4923=FACE_OUTER_BOUND('',#7118,.T.);
#4924=FACE_OUTER_BOUND('',#7119,.T.);
#4925=FACE_OUTER_BOUND('',#7120,.T.);
#4926=FACE_OUTER_BOUND('',#7121,.T.);
#4927=FACE_OUTER_BOUND('',#7122,.T.);
#4928=FACE_OUTER_BOUND('',#7123,.T.);
#4929=FACE_OUTER_BOUND('',#7124,.T.);
#4930=FACE_OUTER_BOUND('',#7125,.T.);
#4931=FACE_OUTER_BOUND('',#7126,.T.);
#4932=FACE_OUTER_BOUND('',#7127,.T.);
#4933=FACE_OUTER_BOUND('',#7128,.T.);
#4934=FACE_OUTER_BOUND('',#7129,.T.);
#4935=FACE_OUTER_BOUND('',#7130,.T.);
#4936=FACE_OUTER_BOUND('',#7131,.T.);
#4937=FACE_OUTER_BOUND('',#7132,.T.);
#4938=FACE_OUTER_BOUND('',#7133,.T.);
#4939=FACE_OUTER_BOUND('',#7134,.T.);
#4940=FACE_OUTER_BOUND('',#7135,.T.);
#4941=FACE_OUTER_BOUND('',#7136,.T.);
#4942=FACE_OUTER_BOUND('',#7137,.T.);
#4943=FACE_OUTER_BOUND('',#7138,.T.);
#4944=FACE_OUTER_BOUND('',#7139,.T.);
#4945=FACE_OUTER_BOUND('',#7140,.T.);
#4946=FACE_OUTER_BOUND('',#7141,.T.);
#4947=FACE_OUTER_BOUND('',#7142,.T.);
#4948=FACE_OUTER_BOUND('',#7143,.T.);
#4949=FACE_OUTER_BOUND('',#7144,.T.);
#4950=FACE_OUTER_BOUND('',#7145,.T.);
#4951=FACE_OUTER_BOUND('',#7146,.T.);
#4952=FACE_OUTER_BOUND('',#7147,.T.);
#4953=FACE_OUTER_BOUND('',#7148,.T.);
#4954=FACE_OUTER_BOUND('',#7149,.T.);
#4955=FACE_OUTER_BOUND('',#7150,.T.);
#4956=FACE_OUTER_BOUND('',#7151,.T.);
#4957=FACE_OUTER_BOUND('',#7152,.T.);
#4958=FACE_OUTER_BOUND('',#7153,.T.);
#4959=FACE_OUTER_BOUND('',#7154,.T.);
#4960=FACE_OUTER_BOUND('',#7155,.T.);
#4961=FACE_OUTER_BOUND('',#7156,.T.);
#4962=FACE_OUTER_BOUND('',#7157,.T.);
#4963=FACE_OUTER_BOUND('',#7158,.T.);
#4964=FACE_OUTER_BOUND('',#7159,.T.);
#4965=FACE_OUTER_BOUND('',#7160,.T.);
#4966=FACE_OUTER_BOUND('',#7161,.T.);
#4967=FACE_OUTER_BOUND('',#7162,.T.);
#4968=FACE_OUTER_BOUND('',#7163,.T.);
#4969=FACE_OUTER_BOUND('',#7164,.T.);
#4970=FACE_OUTER_BOUND('',#7165,.T.);
#4971=FACE_OUTER_BOUND('',#7166,.T.);
#4972=FACE_OUTER_BOUND('',#7167,.T.);
#4973=FACE_OUTER_BOUND('',#7168,.T.);
#4974=FACE_OUTER_BOUND('',#7169,.T.);
#4975=FACE_OUTER_BOUND('',#7170,.T.);
#4976=FACE_OUTER_BOUND('',#7171,.T.);
#4977=FACE_OUTER_BOUND('',#7172,.T.);
#4978=FACE_OUTER_BOUND('',#7173,.T.);
#4979=FACE_OUTER_BOUND('',#7174,.T.);
#4980=FACE_OUTER_BOUND('',#7175,.T.);
#4981=FACE_OUTER_BOUND('',#7176,.T.);
#4982=FACE_OUTER_BOUND('',#7177,.T.);
#4983=FACE_OUTER_BOUND('',#7178,.T.);
#4984=FACE_OUTER_BOUND('',#7179,.T.);
#4985=FACE_OUTER_BOUND('',#7180,.T.);
#4986=FACE_OUTER_BOUND('',#7181,.T.);
#4987=FACE_OUTER_BOUND('',#7182,.T.);
#4988=FACE_OUTER_BOUND('',#7183,.T.);
#4989=FACE_OUTER_BOUND('',#7184,.T.);
#4990=FACE_OUTER_BOUND('',#7185,.T.);
#4991=FACE_OUTER_BOUND('',#7186,.T.);
#4992=FACE_OUTER_BOUND('',#7187,.T.);
#4993=FACE_OUTER_BOUND('',#7188,.T.);
#4994=FACE_OUTER_BOUND('',#7189,.T.);
#4995=FACE_OUTER_BOUND('',#7190,.T.);
#4996=FACE_OUTER_BOUND('',#7191,.T.);
#4997=FACE_OUTER_BOUND('',#7192,.T.);
#4998=FACE_OUTER_BOUND('',#7193,.T.);
#4999=FACE_OUTER_BOUND('',#7194,.T.);
#5000=FACE_OUTER_BOUND('',#7195,.T.);
#5001=FACE_OUTER_BOUND('',#7196,.T.);
#5002=FACE_OUTER_BOUND('',#7197,.T.);
#5003=FACE_OUTER_BOUND('',#7198,.T.);
#5004=FACE_OUTER_BOUND('',#7199,.T.);
#5005=FACE_OUTER_BOUND('',#7200,.T.);
#5006=FACE_OUTER_BOUND('',#7202,.T.);
#5007=FACE_OUTER_BOUND('',#7203,.T.);
#5008=FACE_OUTER_BOUND('',#7204,.T.);
#5009=FACE_OUTER_BOUND('',#7205,.T.);
#5010=FACE_OUTER_BOUND('',#7206,.T.);
#5011=FACE_OUTER_BOUND('',#7207,.T.);
#5012=FACE_OUTER_BOUND('',#7208,.T.);
#5013=FACE_OUTER_BOUND('',#7209,.T.);
#5014=FACE_OUTER_BOUND('',#7210,.T.);
#5015=FACE_OUTER_BOUND('',#7211,.T.);
#5016=FACE_OUTER_BOUND('',#7212,.T.);
#5017=FACE_OUTER_BOUND('',#7213,.T.);
#5018=FACE_OUTER_BOUND('',#7214,.T.);
#5019=FACE_OUTER_BOUND('',#7215,.T.);
#5020=FACE_OUTER_BOUND('',#7216,.T.);
#5021=FACE_OUTER_BOUND('',#7217,.T.);
#5022=FACE_OUTER_BOUND('',#7218,.T.);
#5023=FACE_OUTER_BOUND('',#7219,.T.);
#5024=FACE_OUTER_BOUND('',#7220,.T.);
#5025=FACE_OUTER_BOUND('',#7221,.T.);
#5026=FACE_OUTER_BOUND('',#7222,.T.);
#5027=FACE_OUTER_BOUND('',#7223,.T.);
#5028=FACE_OUTER_BOUND('',#7224,.T.);
#5029=FACE_OUTER_BOUND('',#7225,.T.);
#5030=FACE_OUTER_BOUND('',#7226,.T.);
#5031=FACE_OUTER_BOUND('',#7227,.T.);
#5032=FACE_OUTER_BOUND('',#7228,.T.);
#5033=FACE_OUTER_BOUND('',#7229,.T.);
#5034=FACE_OUTER_BOUND('',#7230,.T.);
#5035=FACE_OUTER_BOUND('',#7231,.T.);
#5036=FACE_OUTER_BOUND('',#7232,.T.);
#5037=FACE_OUTER_BOUND('',#7233,.T.);
#5038=FACE_OUTER_BOUND('',#7234,.T.);
#5039=FACE_OUTER_BOUND('',#7235,.T.);
#5040=FACE_OUTER_BOUND('',#7236,.T.);
#5041=FACE_OUTER_BOUND('',#7237,.T.);
#5042=FACE_OUTER_BOUND('',#7238,.T.);
#5043=FACE_OUTER_BOUND('',#7239,.T.);
#5044=FACE_OUTER_BOUND('',#7240,.T.);
#5045=FACE_OUTER_BOUND('',#7241,.T.);
#5046=FACE_OUTER_BOUND('',#7242,.T.);
#5047=FACE_OUTER_BOUND('',#7243,.T.);
#5048=FACE_OUTER_BOUND('',#7244,.T.);
#5049=FACE_OUTER_BOUND('',#7245,.T.);
#5050=FACE_OUTER_BOUND('',#7246,.T.);
#5051=FACE_OUTER_BOUND('',#7247,.T.);
#5052=FACE_OUTER_BOUND('',#7248,.T.);
#5053=FACE_OUTER_BOUND('',#7249,.T.);
#5054=FACE_OUTER_BOUND('',#7250,.T.);
#5055=FACE_OUTER_BOUND('',#7251,.T.);
#5056=FACE_OUTER_BOUND('',#7252,.T.);
#5057=FACE_OUTER_BOUND('',#7253,.T.);
#5058=FACE_OUTER_BOUND('',#7254,.T.);
#5059=FACE_OUTER_BOUND('',#7255,.T.);
#5060=FACE_OUTER_BOUND('',#7256,.T.);
#5061=FACE_OUTER_BOUND('',#7257,.T.);
#5062=FACE_OUTER_BOUND('',#7258,.T.);
#5063=FACE_OUTER_BOUND('',#7259,.T.);
#5064=FACE_OUTER_BOUND('',#7260,.T.);
#5065=FACE_OUTER_BOUND('',#7261,.T.);
#5066=FACE_OUTER_BOUND('',#7262,.T.);
#5067=FACE_OUTER_BOUND('',#7263,.T.);
#5068=FACE_OUTER_BOUND('',#7264,.T.);
#5069=FACE_OUTER_BOUND('',#7265,.T.);
#5070=FACE_OUTER_BOUND('',#7266,.T.);
#5071=FACE_OUTER_BOUND('',#7267,.T.);
#5072=FACE_OUTER_BOUND('',#7268,.T.);
#5073=FACE_OUTER_BOUND('',#7269,.T.);
#5074=FACE_OUTER_BOUND('',#7270,.T.);
#5075=FACE_OUTER_BOUND('',#7271,.T.);
#5076=FACE_OUTER_BOUND('',#7272,.T.);
#5077=FACE_OUTER_BOUND('',#7273,.T.);
#5078=FACE_OUTER_BOUND('',#7274,.T.);
#5079=FACE_OUTER_BOUND('',#7275,.T.);
#5080=FACE_OUTER_BOUND('',#7276,.T.);
#5081=FACE_OUTER_BOUND('',#7277,.T.);
#5082=FACE_OUTER_BOUND('',#7278,.T.);
#5083=FACE_OUTER_BOUND('',#7279,.T.);
#5084=FACE_OUTER_BOUND('',#7280,.T.);
#5085=FACE_OUTER_BOUND('',#7281,.T.);
#5086=FACE_OUTER_BOUND('',#7282,.T.);
#5087=FACE_OUTER_BOUND('',#7283,.T.);
#5088=FACE_OUTER_BOUND('',#7284,.T.);
#5089=FACE_OUTER_BOUND('',#7285,.T.);
#5090=FACE_OUTER_BOUND('',#7286,.T.);
#5091=FACE_OUTER_BOUND('',#7287,.T.);
#5092=FACE_OUTER_BOUND('',#7288,.T.);
#5093=FACE_OUTER_BOUND('',#7289,.T.);
#5094=FACE_OUTER_BOUND('',#7290,.T.);
#5095=FACE_OUTER_BOUND('',#7291,.T.);
#5096=FACE_OUTER_BOUND('',#7292,.T.);
#5097=FACE_OUTER_BOUND('',#7293,.T.);
#5098=FACE_OUTER_BOUND('',#7294,.T.);
#5099=FACE_OUTER_BOUND('',#7295,.T.);
#5100=FACE_OUTER_BOUND('',#7296,.T.);
#5101=FACE_OUTER_BOUND('',#7297,.T.);
#5102=FACE_OUTER_BOUND('',#7298,.T.);
#5103=FACE_OUTER_BOUND('',#7299,.T.);
#5104=FACE_OUTER_BOUND('',#7300,.T.);
#5105=FACE_OUTER_BOUND('',#7301,.T.);
#5106=FACE_OUTER_BOUND('',#7302,.T.);
#5107=FACE_OUTER_BOUND('',#7303,.T.);
#5108=FACE_OUTER_BOUND('',#7304,.T.);
#5109=FACE_OUTER_BOUND('',#7305,.T.);
#5110=FACE_OUTER_BOUND('',#7306,.T.);
#5111=FACE_OUTER_BOUND('',#7307,.T.);
#5112=FACE_OUTER_BOUND('',#7308,.T.);
#5113=FACE_OUTER_BOUND('',#7309,.T.);
#5114=FACE_OUTER_BOUND('',#7310,.T.);
#5115=FACE_OUTER_BOUND('',#7311,.T.);
#5116=FACE_OUTER_BOUND('',#7312,.T.);
#5117=FACE_OUTER_BOUND('',#7313,.T.);
#5118=FACE_OUTER_BOUND('',#7314,.T.);
#5119=FACE_OUTER_BOUND('',#7315,.T.);
#5120=FACE_OUTER_BOUND('',#7316,.T.);
#5121=FACE_OUTER_BOUND('',#7317,.T.);
#5122=FACE_OUTER_BOUND('',#7318,.T.);
#5123=FACE_OUTER_BOUND('',#7319,.T.);
#5124=FACE_OUTER_BOUND('',#7320,.T.);
#5125=FACE_OUTER_BOUND('',#7321,.T.);
#5126=FACE_OUTER_BOUND('',#7322,.T.);
#5127=FACE_OUTER_BOUND('',#7323,.T.);
#5128=FACE_OUTER_BOUND('',#7324,.T.);
#5129=FACE_OUTER_BOUND('',#7325,.T.);
#5130=FACE_OUTER_BOUND('',#7326,.T.);
#5131=FACE_OUTER_BOUND('',#7327,.T.);
#5132=FACE_OUTER_BOUND('',#7328,.T.);
#5133=FACE_OUTER_BOUND('',#7329,.T.);
#5134=FACE_OUTER_BOUND('',#7330,.T.);
#5135=FACE_OUTER_BOUND('',#7331,.T.);
#5136=FACE_OUTER_BOUND('',#7332,.T.);
#5137=FACE_OUTER_BOUND('',#7333,.T.);
#5138=FACE_OUTER_BOUND('',#7334,.T.);
#5139=FACE_OUTER_BOUND('',#7335,.T.);
#5140=FACE_OUTER_BOUND('',#7336,.T.);
#5141=FACE_OUTER_BOUND('',#7337,.T.);
#5142=FACE_OUTER_BOUND('',#7338,.T.);
#5143=FACE_OUTER_BOUND('',#7344,.T.);
#5144=FACE_OUTER_BOUND('',#7345,.T.);
#5145=FACE_OUTER_BOUND('',#7346,.T.);
#5146=FACE_OUTER_BOUND('',#7347,.T.);
#5147=FACE_OUTER_BOUND('',#7348,.T.);
#5148=FACE_OUTER_BOUND('',#7349,.T.);
#5149=FACE_OUTER_BOUND('',#7350,.T.);
#5150=FACE_OUTER_BOUND('',#7351,.T.);
#5151=FACE_OUTER_BOUND('',#7352,.T.);
#5152=FACE_OUTER_BOUND('',#7353,.T.);
#5153=FACE_OUTER_BOUND('',#7354,.T.);
#5154=FACE_OUTER_BOUND('',#7355,.T.);
#5155=FACE_OUTER_BOUND('',#7356,.T.);
#5156=FACE_OUTER_BOUND('',#7357,.T.);
#5157=FACE_OUTER_BOUND('',#7358,.T.);
#5158=FACE_OUTER_BOUND('',#7359,.T.);
#5159=FACE_OUTER_BOUND('',#7360,.T.);
#5160=FACE_OUTER_BOUND('',#7361,.T.);
#5161=FACE_OUTER_BOUND('',#7362,.T.);
#5162=FACE_OUTER_BOUND('',#7363,.T.);
#5163=FACE_OUTER_BOUND('',#7364,.T.);
#5164=FACE_OUTER_BOUND('',#7365,.T.);
#5165=FACE_OUTER_BOUND('',#7366,.T.);
#5166=FACE_OUTER_BOUND('',#7367,.T.);
#5167=FACE_OUTER_BOUND('',#7368,.T.);
#5168=FACE_OUTER_BOUND('',#7369,.T.);
#5169=FACE_OUTER_BOUND('',#7370,.T.);
#5170=FACE_OUTER_BOUND('',#7371,.T.);
#5171=FACE_OUTER_BOUND('',#7372,.T.);
#5172=FACE_OUTER_BOUND('',#7373,.T.);
#5173=FACE_OUTER_BOUND('',#7374,.T.);
#5174=FACE_OUTER_BOUND('',#7375,.T.);
#5175=FACE_OUTER_BOUND('',#7376,.T.);
#5176=FACE_OUTER_BOUND('',#7377,.T.);
#5177=FACE_OUTER_BOUND('',#7378,.T.);
#5178=FACE_OUTER_BOUND('',#7379,.T.);
#5179=FACE_OUTER_BOUND('',#7380,.T.);
#5180=FACE_OUTER_BOUND('',#7381,.T.);
#5181=FACE_OUTER_BOUND('',#7382,.T.);
#5182=FACE_OUTER_BOUND('',#7383,.T.);
#5183=FACE_OUTER_BOUND('',#7384,.T.);
#5184=FACE_OUTER_BOUND('',#7385,.T.);
#6732=EDGE_LOOP('',(#27993,#27994,#27995,#27996,#27997));
#6733=EDGE_LOOP('',(#27998,#27999,#28000,#28001,#28002));
#6734=EDGE_LOOP('',(#28003,#28004,#28005,#28006));
#6735=EDGE_LOOP('',(#28007,#28008,#28009,#28010));
#6736=EDGE_LOOP('',(#28011,#28012,#28013,#28014));
#6737=EDGE_LOOP('',(#28015,#28016,#28017,#28018));
#6738=EDGE_LOOP('',(#28019,#28020,#28021,#28022));
#6739=EDGE_LOOP('',(#28023,#28024,#28025,#28026));
#6740=EDGE_LOOP('',(#28027,#28028,#28029,#28030,#28031,#28032));
#6741=EDGE_LOOP('',(#28033,#28034,#28035,#28036,#28037));
#6742=EDGE_LOOP('',(#28038,#28039,#28040,#28041));
#6743=EDGE_LOOP('',(#28042,#28043,#28044));
#6744=EDGE_LOOP('',(#28045,#28046,#28047,#28048));
#6745=EDGE_LOOP('',(#28049,#28050,#28051));
#6746=EDGE_LOOP('',(#28052,#28053,#28054,#28055));
#6747=EDGE_LOOP('',(#28056,#28057,#28058,#28059));
#6748=EDGE_LOOP('',(#28060,#28061,#28062,#28063));
#6749=EDGE_LOOP('',(#28064,#28065,#28066,#28067));
#6750=EDGE_LOOP('',(#28068,#28069,#28070,#28071));
#6751=EDGE_LOOP('',(#28072,#28073,#28074,#28075));
#6752=EDGE_LOOP('',(#28076,#28077,#28078,#28079));
#6753=EDGE_LOOP('',(#28080,#28081,#28082));
#6754=EDGE_LOOP('',(#28083,#28084,#28085,#28086));
#6755=EDGE_LOOP('',(#28087,#28088,#28089));
#6756=EDGE_LOOP('',(#28090,#28091,#28092,#28093));
#6757=EDGE_LOOP('',(#28094,#28095,#28096,#28097,#28098,#28099,#28100,#28101,
#28102,#28103,#28104,#28105,#28106));
#6758=EDGE_LOOP('',(#28107,#28108,#28109,#28110,#28111,#28112,#28113));
#6759=EDGE_LOOP('',(#28114,#28115,#28116,#28117));
#6760=EDGE_LOOP('',(#28118,#28119,#28120,#28121));
#6761=EDGE_LOOP('',(#28122,#28123,#28124,#28125));
#6762=EDGE_LOOP('',(#28126,#28127,#28128,#28129));
#6763=EDGE_LOOP('',(#28130,#28131,#28132,#28133));
#6764=EDGE_LOOP('',(#28134,#28135,#28136,#28137));
#6765=EDGE_LOOP('',(#28138,#28139,#28140,#28141));
#6766=EDGE_LOOP('',(#28142,#28143,#28144));
#6767=EDGE_LOOP('',(#28145,#28146,#28147,#28148));
#6768=EDGE_LOOP('',(#28149,#28150,#28151));
#6769=EDGE_LOOP('',(#28152,#28153,#28154,#28155));
#6770=EDGE_LOOP('',(#28156,#28157,#28158,#28159));
#6771=EDGE_LOOP('',(#28160,#28161,#28162,#28163));
#6772=EDGE_LOOP('',(#28164,#28165,#28166));
#6773=EDGE_LOOP('',(#28167,#28168,#28169,#28170));
#6774=EDGE_LOOP('',(#28171,#28172,#28173,#28174));
#6775=EDGE_LOOP('',(#28175,#28176,#28177,#28178));
#6776=EDGE_LOOP('',(#28179,#28180,#28181,#28182));
#6777=EDGE_LOOP('',(#28183,#28184,#28185,#28186));
#6778=EDGE_LOOP('',(#28187,#28188,#28189));
#6779=EDGE_LOOP('',(#28190,#28191,#28192,#28193));
#6780=EDGE_LOOP('',(#28194,#28195,#28196));
#6781=EDGE_LOOP('',(#28197,#28198,#28199,#28200));
#6782=EDGE_LOOP('',(#28201,#28202,#28203));
#6783=EDGE_LOOP('',(#28204,#28205,#28206,#28207));
#6784=EDGE_LOOP('',(#28208,#28209,#28210));
#6785=EDGE_LOOP('',(#28211,#28212,#28213,#28214));
#6786=EDGE_LOOP('',(#28215,#28216,#28217,#28218));
#6787=EDGE_LOOP('',(#28219,#28220,#28221,#28222));
#6788=EDGE_LOOP('',(#28223,#28224,#28225,#28226));
#6789=EDGE_LOOP('',(#28227,#28228,#28229,#28230));
#6790=EDGE_LOOP('',(#28231,#28232,#28233,#28234));
#6791=EDGE_LOOP('',(#28235,#28236,#28237,#28238));
#6792=EDGE_LOOP('',(#28239,#28240,#28241,#28242));
#6793=EDGE_LOOP('',(#28243,#28244,#28245,#28246));
#6794=EDGE_LOOP('',(#28247,#28248,#28249,#28250));
#6795=EDGE_LOOP('',(#28251,#28252,#28253));
#6796=EDGE_LOOP('',(#28254,#28255,#28256,#28257));
#6797=EDGE_LOOP('',(#28258,#28259,#28260,#28261));
#6798=EDGE_LOOP('',(#28262,#28263,#28264,#28265));
#6799=EDGE_LOOP('',(#28266,#28267,#28268,#28269));
#6800=EDGE_LOOP('',(#28270,#28271,#28272,#28273));
#6801=EDGE_LOOP('',(#28274,#28275,#28276,#28277));
#6802=EDGE_LOOP('',(#28278,#28279,#28280,#28281));
#6803=EDGE_LOOP('',(#28282,#28283,#28284,#28285));
#6804=EDGE_LOOP('',(#28286,#28287,#28288,#28289,#28290,#28291,#28292,#28293,
#28294,#28295,#28296,#28297,#28298,#28299));
#6805=EDGE_LOOP('',(#28300,#28301,#28302,#28303,#28304));
#6806=EDGE_LOOP('',(#28305,#28306,#28307,#28308));
#6807=EDGE_LOOP('',(#28309,#28310,#28311,#28312,#28313,#28314));
#6808=EDGE_LOOP('',(#28315,#28316,#28317,#28318));
#6809=EDGE_LOOP('',(#28319,#28320,#28321,#28322,#28323,#28324));
#6810=EDGE_LOOP('',(#28325,#28326,#28327,#28328));
#6811=EDGE_LOOP('',(#28329,#28330,#28331));
#6812=EDGE_LOOP('',(#28332,#28333,#28334,#28335));
#6813=EDGE_LOOP('',(#28336,#28337,#28338,#28339));
#6814=EDGE_LOOP('',(#28340,#28341,#28342,#28343,#28344,#28345,#28346,#28347,
#28348));
#6815=EDGE_LOOP('',(#28349,#28350,#28351,#28352));
#6816=EDGE_LOOP('',(#28353,#28354,#28355,#28356));
#6817=EDGE_LOOP('',(#28357,#28358,#28359,#28360));
#6818=EDGE_LOOP('',(#28361,#28362,#28363,#28364));
#6819=EDGE_LOOP('',(#28365,#28366,#28367,#28368));
#6820=EDGE_LOOP('',(#28369,#28370,#28371,#28372));
#6821=EDGE_LOOP('',(#28373,#28374,#28375,#28376));
#6822=EDGE_LOOP('',(#28377,#28378,#28379,#28380));
#6823=EDGE_LOOP('',(#28381,#28382,#28383,#28384));
#6824=EDGE_LOOP('',(#28385,#28386,#28387,#28388));
#6825=EDGE_LOOP('',(#28389,#28390,#28391,#28392));
#6826=EDGE_LOOP('',(#28393,#28394,#28395,#28396));
#6827=EDGE_LOOP('',(#28397,#28398,#28399,#28400));
#6828=EDGE_LOOP('',(#28401,#28402,#28403,#28404));
#6829=EDGE_LOOP('',(#28405,#28406,#28407,#28408));
#6830=EDGE_LOOP('',(#28409,#28410,#28411,#28412));
#6831=EDGE_LOOP('',(#28413,#28414,#28415,#28416));
#6832=EDGE_LOOP('',(#28417,#28418,#28419,#28420));
#6833=EDGE_LOOP('',(#28421,#28422,#28423,#28424,#28425));
#6834=EDGE_LOOP('',(#28426,#28427,#28428,#28429));
#6835=EDGE_LOOP('',(#28430,#28431,#28432,#28433));
#6836=EDGE_LOOP('',(#28434,#28435,#28436,#28437));
#6837=EDGE_LOOP('',(#28438,#28439,#28440,#28441,#28442,#28443,#28444));
#6838=EDGE_LOOP('',(#28445,#28446,#28447,#28448));
#6839=EDGE_LOOP('',(#28449,#28450,#28451,#28452));
#6840=EDGE_LOOP('',(#28453,#28454,#28455,#28456));
#6841=EDGE_LOOP('',(#28457,#28458,#28459,#28460));
#6842=EDGE_LOOP('',(#28461,#28462,#28463,#28464));
#6843=EDGE_LOOP('',(#28465,#28466,#28467,#28468));
#6844=EDGE_LOOP('',(#28469,#28470,#28471,#28472,#28473,#28474,#28475,#28476));
#6845=EDGE_LOOP('',(#28477,#28478,#28479,#28480));
#6846=EDGE_LOOP('',(#28481,#28482,#28483,#28484));
#6847=EDGE_LOOP('',(#28485,#28486,#28487,#28488));
#6848=EDGE_LOOP('',(#28489,#28490,#28491,#28492));
#6849=EDGE_LOOP('',(#28493,#28494,#28495,#28496));
#6850=EDGE_LOOP('',(#28497,#28498,#28499,#28500));
#6851=EDGE_LOOP('',(#28501,#28502,#28503,#28504));
#6852=EDGE_LOOP('',(#28505,#28506,#28507,#28508));
#6853=EDGE_LOOP('',(#28509,#28510,#28511,#28512));
#6854=EDGE_LOOP('',(#28513,#28514,#28515,#28516));
#6855=EDGE_LOOP('',(#28517,#28518,#28519));
#6856=EDGE_LOOP('',(#28520,#28521,#28522,#28523));
#6857=EDGE_LOOP('',(#28524,#28525,#28526));
#6858=EDGE_LOOP('',(#28527,#28528,#28529));
#6859=EDGE_LOOP('',(#28530,#28531,#28532));
#6860=EDGE_LOOP('',(#28533,#28534,#28535,#28536));
#6861=EDGE_LOOP('',(#28537,#28538,#28539,#28540));
#6862=EDGE_LOOP('',(#28541,#28542,#28543,#28544));
#6863=EDGE_LOOP('',(#28545,#28546,#28547,#28548));
#6864=EDGE_LOOP('',(#28549,#28550,#28551,#28552));
#6865=EDGE_LOOP('',(#28553,#28554,#28555,#28556));
#6866=EDGE_LOOP('',(#28557,#28558,#28559));
#6867=EDGE_LOOP('',(#28560,#28561,#28562,#28563));
#6868=EDGE_LOOP('',(#28564,#28565,#28566));
#6869=EDGE_LOOP('',(#28567,#28568,#28569,#28570));
#6870=EDGE_LOOP('',(#28571,#28572,#28573,#28574));
#6871=EDGE_LOOP('',(#28575,#28576,#28577,#28578));
#6872=EDGE_LOOP('',(#28579,#28580));
#6873=EDGE_LOOP('',(#28581,#28582,#28583,#28584));
#6874=EDGE_LOOP('',(#28585,#28586,#28587,#28588));
#6875=EDGE_LOOP('',(#28589,#28590,#28591,#28592));
#6876=EDGE_LOOP('',(#28593,#28594,#28595,#28596));
#6877=EDGE_LOOP('',(#28597,#28598,#28599,#28600));
#6878=EDGE_LOOP('',(#28601,#28602,#28603));
#6879=EDGE_LOOP('',(#28604,#28605,#28606,#28607));
#6880=EDGE_LOOP('',(#28608,#28609,#28610,#28611));
#6881=EDGE_LOOP('',(#28612,#28613,#28614,#28615,#28616,#28617));
#6882=EDGE_LOOP('',(#28618,#28619,#28620,#28621));
#6883=EDGE_LOOP('',(#28622,#28623,#28624,#28625));
#6884=EDGE_LOOP('',(#28626,#28627,#28628,#28629));
#6885=EDGE_LOOP('',(#28630,#28631,#28632));
#6886=EDGE_LOOP('',(#28633,#28634,#28635,#28636));
#6887=EDGE_LOOP('',(#28637,#28638,#28639,#28640));
#6888=EDGE_LOOP('',(#28641,#28642,#28643,#28644,#28645));
#6889=EDGE_LOOP('',(#28646,#28647,#28648,#28649));
#6890=EDGE_LOOP('',(#28650,#28651,#28652,#28653));
#6891=EDGE_LOOP('',(#28654,#28655,#28656,#28657));
#6892=EDGE_LOOP('',(#28658,#28659,#28660,#28661));
#6893=EDGE_LOOP('',(#28662,#28663,#28664,#28665,#28666,#28667,#28668));
#6894=EDGE_LOOP('',(#28669,#28670,#28671,#28672));
#6895=EDGE_LOOP('',(#28673,#28674,#28675));
#6896=EDGE_LOOP('',(#28676,#28677,#28678,#28679,#28680,#28681,#28682,#28683));
#6897=EDGE_LOOP('',(#28684,#28685,#28686,#28687));
#6898=EDGE_LOOP('',(#28688,#28689,#28690,#28691));
#6899=EDGE_LOOP('',(#28692,#28693,#28694));
#6900=EDGE_LOOP('',(#28695,#28696,#28697,#28698));
#6901=EDGE_LOOP('',(#28699,#28700,#28701,#28702,#28703,#28704));
#6902=EDGE_LOOP('',(#28705,#28706,#28707,#28708));
#6903=EDGE_LOOP('',(#28709,#28710,#28711,#28712));
#6904=EDGE_LOOP('',(#28713,#28714,#28715,#28716));
#6905=EDGE_LOOP('',(#28717,#28718,#28719,#28720));
#6906=EDGE_LOOP('',(#28721,#28722,#28723,#28724));
#6907=EDGE_LOOP('',(#28725,#28726,#28727,#28728));
#6908=EDGE_LOOP('',(#28729,#28730,#28731,#28732));
#6909=EDGE_LOOP('',(#28733,#28734,#28735,#28736));
#6910=EDGE_LOOP('',(#28737,#28738,#28739,#28740));
#6911=EDGE_LOOP('',(#28741,#28742,#28743,#28744));
#6912=EDGE_LOOP('',(#28745,#28746,#28747,#28748));
#6913=EDGE_LOOP('',(#28749,#28750,#28751,#28752));
#6914=EDGE_LOOP('',(#28753,#28754,#28755,#28756));
#6915=EDGE_LOOP('',(#28757,#28758,#28759,#28760));
#6916=EDGE_LOOP('',(#28761,#28762,#28763,#28764));
#6917=EDGE_LOOP('',(#28765,#28766,#28767,#28768));
#6918=EDGE_LOOP('',(#28769,#28770,#28771,#28772));
#6919=EDGE_LOOP('',(#28773,#28774,#28775,#28776));
#6920=EDGE_LOOP('',(#28777,#28778,#28779,#28780));
#6921=EDGE_LOOP('',(#28781,#28782,#28783,#28784));
#6922=EDGE_LOOP('',(#28785,#28786,#28787,#28788));
#6923=EDGE_LOOP('',(#28789,#28790,#28791,#28792));
#6924=EDGE_LOOP('',(#28793,#28794,#28795,#28796));
#6925=EDGE_LOOP('',(#28797,#28798,#28799,#28800));
#6926=EDGE_LOOP('',(#28801,#28802,#28803,#28804));
#6927=EDGE_LOOP('',(#28805,#28806,#28807));
#6928=EDGE_LOOP('',(#28808,#28809,#28810,#28811));
#6929=EDGE_LOOP('',(#28812,#28813,#28814));
#6930=EDGE_LOOP('',(#28815,#28816,#28817));
#6931=EDGE_LOOP('',(#28818,#28819,#28820,#28821));
#6932=EDGE_LOOP('',(#28822,#28823,#28824,#28825));
#6933=EDGE_LOOP('',(#28826,#28827,#28828));
#6934=EDGE_LOOP('',(#28829,#28830,#28831));
#6935=EDGE_LOOP('',(#28832,#28833,#28834));
#6936=EDGE_LOOP('',(#28835,#28836,#28837,#28838));
#6937=EDGE_LOOP('',(#28839,#28840,#28841,#28842));
#6938=EDGE_LOOP('',(#28843,#28844,#28845,#28846));
#6939=EDGE_LOOP('',(#28847,#28848,#28849));
#6940=EDGE_LOOP('',(#28850,#28851,#28852,#28853));
#6941=EDGE_LOOP('',(#28854,#28855,#28856,#28857));
#6942=EDGE_LOOP('',(#28858,#28859,#28860));
#6943=EDGE_LOOP('',(#28861,#28862,#28863,#28864));
#6944=EDGE_LOOP('',(#28865,#28866,#28867,#28868));
#6945=EDGE_LOOP('',(#28869,#28870,#28871));
#6946=EDGE_LOOP('',(#28872,#28873,#28874,#28875));
#6947=EDGE_LOOP('',(#28876,#28877,#28878,#28879));
#6948=EDGE_LOOP('',(#28880,#28881,#28882));
#6949=EDGE_LOOP('',(#28883,#28884,#28885,#28886));
#6950=EDGE_LOOP('',(#28887,#28888,#28889,#28890));
#6951=EDGE_LOOP('',(#28891,#28892,#28893,#28894));
#6952=EDGE_LOOP('',(#28895,#28896,#28897,#28898));
#6953=EDGE_LOOP('',(#28899,#28900,#28901,#28902));
#6954=EDGE_LOOP('',(#28903,#28904,#28905,#28906));
#6955=EDGE_LOOP('',(#28907,#28908,#28909,#28910));
#6956=EDGE_LOOP('',(#28911,#28912,#28913,#28914));
#6957=EDGE_LOOP('',(#28915,#28916,#28917,#28918,#28919));
#6958=EDGE_LOOP('',(#28920,#28921,#28922,#28923));
#6959=EDGE_LOOP('',(#28924,#28925,#28926));
#6960=EDGE_LOOP('',(#28927,#28928,#28929,#28930));
#6961=EDGE_LOOP('',(#28931,#28932,#28933,#28934));
#6962=EDGE_LOOP('',(#28935,#28936,#28937,#28938));
#6963=EDGE_LOOP('',(#28939,#28940,#28941,#28942));
#6964=EDGE_LOOP('',(#28943,#28944,#28945,#28946));
#6965=EDGE_LOOP('',(#28947,#28948,#28949));
#6966=EDGE_LOOP('',(#28950,#28951,#28952,#28953));
#6967=EDGE_LOOP('',(#28954,#28955,#28956,#28957));
#6968=EDGE_LOOP('',(#28958,#28959,#28960,#28961));
#6969=EDGE_LOOP('',(#28962,#28963,#28964));
#6970=EDGE_LOOP('',(#28965,#28966,#28967,#28968));
#6971=EDGE_LOOP('',(#28969,#28970,#28971,#28972));
#6972=EDGE_LOOP('',(#28973,#28974,#28975,#28976));
#6973=EDGE_LOOP('',(#28977,#28978,#28979,#28980));
#6974=EDGE_LOOP('',(#28981,#28982,#28983,#28984));
#6975=EDGE_LOOP('',(#28985,#28986,#28987,#28988));
#6976=EDGE_LOOP('',(#28989,#28990,#28991));
#6977=EDGE_LOOP('',(#28992,#28993,#28994,#28995));
#6978=EDGE_LOOP('',(#28996,#28997,#28998,#28999));
#6979=EDGE_LOOP('',(#29000,#29001,#29002,#29003));
#6980=EDGE_LOOP('',(#29004,#29005,#29006,#29007));
#6981=EDGE_LOOP('',(#29008,#29009,#29010,#29011));
#6982=EDGE_LOOP('',(#29012,#29013,#29014,#29015));
#6983=EDGE_LOOP('',(#29016,#29017,#29018,#29019,#29020));
#6984=EDGE_LOOP('',(#29021,#29022,#29023,#29024));
#6985=EDGE_LOOP('',(#29025,#29026,#29027,#29028));
#6986=EDGE_LOOP('',(#29029,#29030,#29031,#29032));
#6987=EDGE_LOOP('',(#29033,#29034,#29035,#29036));
#6988=EDGE_LOOP('',(#29037,#29038,#29039,#29040));
#6989=EDGE_LOOP('',(#29041,#29042,#29043,#29044));
#6990=EDGE_LOOP('',(#29045,#29046,#29047,#29048));
#6991=EDGE_LOOP('',(#29049,#29050,#29051,#29052));
#6992=EDGE_LOOP('',(#29053,#29054,#29055,#29056,#29057));
#6993=EDGE_LOOP('',(#29058,#29059,#29060,#29061));
#6994=EDGE_LOOP('',(#29062,#29063,#29064,#29065));
#6995=EDGE_LOOP('',(#29066,#29067,#29068,#29069));
#6996=EDGE_LOOP('',(#29070,#29071,#29072,#29073));
#6997=EDGE_LOOP('',(#29074,#29075,#29076,#29077));
#6998=EDGE_LOOP('',(#29078,#29079,#29080,#29081));
#6999=EDGE_LOOP('',(#29082,#29083,#29084));
#7000=EDGE_LOOP('',(#29085,#29086,#29087,#29088,#29089));
#7001=EDGE_LOOP('',(#29090,#29091,#29092,#29093,#29094,#29095));
#7002=EDGE_LOOP('',(#29096,#29097,#29098,#29099));
#7003=EDGE_LOOP('',(#29100,#29101,#29102,#29103,#29104,#29105));
#7004=EDGE_LOOP('',(#29106,#29107,#29108,#29109));
#7005=EDGE_LOOP('',(#29110,#29111,#29112,#29113));
#7006=EDGE_LOOP('',(#29114,#29115,#29116,#29117));
#7007=EDGE_LOOP('',(#29118,#29119,#29120,#29121));
#7008=EDGE_LOOP('',(#29122,#29123,#29124,#29125));
#7009=EDGE_LOOP('',(#29126,#29127,#29128,#29129));
#7010=EDGE_LOOP('',(#29130,#29131,#29132,#29133));
#7011=EDGE_LOOP('',(#29134,#29135,#29136,#29137,#29138,#29139));
#7012=EDGE_LOOP('',(#29140,#29141,#29142,#29143));
#7013=EDGE_LOOP('',(#29144,#29145,#29146));
#7014=EDGE_LOOP('',(#29147,#29148,#29149,#29150));
#7015=EDGE_LOOP('',(#29151,#29152,#29153,#29154));
#7016=EDGE_LOOP('',(#29155,#29156,#29157));
#7017=EDGE_LOOP('',(#29158,#29159,#29160,#29161));
#7018=EDGE_LOOP('',(#29162,#29163,#29164));
#7019=EDGE_LOOP('',(#29165,#29166,#29167,#29168));
#7020=EDGE_LOOP('',(#29169,#29170,#29171));
#7021=EDGE_LOOP('',(#29172,#29173,#29174,#29175));
#7022=EDGE_LOOP('',(#29176,#29177,#29178));
#7023=EDGE_LOOP('',(#29179,#29180,#29181,#29182));
#7024=EDGE_LOOP('',(#29183,#29184,#29185));
#7025=EDGE_LOOP('',(#29186,#29187,#29188,#29189));
#7026=EDGE_LOOP('',(#29190,#29191,#29192,#29193));
#7027=EDGE_LOOP('',(#29194,#29195,#29196,#29197));
#7028=EDGE_LOOP('',(#29198,#29199,#29200,#29201));
#7029=EDGE_LOOP('',(#29202,#29203,#29204,#29205));
#7030=EDGE_LOOP('',(#29206,#29207,#29208,#29209,#29210,#29211,#29212,#29213,
#29214,#29215,#29216));
#7031=EDGE_LOOP('',(#29217,#29218,#29219,#29220,#29221));
#7032=EDGE_LOOP('',(#29222,#29223,#29224,#29225,#29226));
#7033=EDGE_LOOP('',(#29227,#29228,#29229,#29230));
#7034=EDGE_LOOP('',(#29231,#29232,#29233,#29234));
#7035=EDGE_LOOP('',(#29235,#29236,#29237,#29238));
#7036=EDGE_LOOP('',(#29239,#29240,#29241,#29242));
#7037=EDGE_LOOP('',(#29243,#29244,#29245,#29246));
#7038=EDGE_LOOP('',(#29247,#29248,#29249,#29250));
#7039=EDGE_LOOP('',(#29251,#29252,#29253,#29254,#29255,#29256));
#7040=EDGE_LOOP('',(#29257,#29258,#29259,#29260,#29261));
#7041=EDGE_LOOP('',(#29262,#29263,#29264,#29265));
#7042=EDGE_LOOP('',(#29266,#29267,#29268));
#7043=EDGE_LOOP('',(#29269,#29270,#29271,#29272));
#7044=EDGE_LOOP('',(#29273,#29274,#29275));
#7045=EDGE_LOOP('',(#29276,#29277,#29278,#29279));
#7046=EDGE_LOOP('',(#29280,#29281,#29282,#29283));
#7047=EDGE_LOOP('',(#29284,#29285,#29286,#29287));
#7048=EDGE_LOOP('',(#29288,#29289,#29290,#29291));
#7049=EDGE_LOOP('',(#29292,#29293,#29294,#29295));
#7050=EDGE_LOOP('',(#29296,#29297,#29298,#29299));
#7051=EDGE_LOOP('',(#29300,#29301,#29302,#29303));
#7052=EDGE_LOOP('',(#29304,#29305,#29306));
#7053=EDGE_LOOP('',(#29307,#29308,#29309,#29310));
#7054=EDGE_LOOP('',(#29311,#29312,#29313));
#7055=EDGE_LOOP('',(#29314,#29315,#29316,#29317));
#7056=EDGE_LOOP('',(#29318,#29319,#29320,#29321,#29322,#29323,#29324,#29325,
#29326,#29327,#29328,#29329,#29330));
#7057=EDGE_LOOP('',(#29331,#29332,#29333,#29334,#29335,#29336,#29337));
#7058=EDGE_LOOP('',(#29338,#29339,#29340,#29341));
#7059=EDGE_LOOP('',(#29342,#29343,#29344,#29345));
#7060=EDGE_LOOP('',(#29346,#29347,#29348,#29349));
#7061=EDGE_LOOP('',(#29350,#29351,#29352,#29353));
#7062=EDGE_LOOP('',(#29354,#29355,#29356,#29357));
#7063=EDGE_LOOP('',(#29358,#29359,#29360,#29361));
#7064=EDGE_LOOP('',(#29362,#29363,#29364,#29365));
#7065=EDGE_LOOP('',(#29366,#29367,#29368));
#7066=EDGE_LOOP('',(#29369,#29370,#29371,#29372));
#7067=EDGE_LOOP('',(#29373,#29374,#29375));
#7068=EDGE_LOOP('',(#29376,#29377,#29378,#29379));
#7069=EDGE_LOOP('',(#29380,#29381,#29382,#29383));
#7070=EDGE_LOOP('',(#29384,#29385,#29386));
#7071=EDGE_LOOP('',(#29387,#29388,#29389,#29390));
#7072=EDGE_LOOP('',(#29391,#29392,#29393));
#7073=EDGE_LOOP('',(#29394,#29395,#29396));
#7074=EDGE_LOOP('',(#29397,#29398,#29399,#29400));
#7075=EDGE_LOOP('',(#29401,#29402,#29403,#29404,#29405,#29406,#29407,#29408,
#29409,#29410,#29411,#29412));
#7076=EDGE_LOOP('',(#29413,#29414,#29415,#29416));
#7077=EDGE_LOOP('',(#29417,#29418,#29419,#29420));
#7078=EDGE_LOOP('',(#29421,#29422,#29423,#29424));
#7079=EDGE_LOOP('',(#29425,#29426,#29427,#29428));
#7080=EDGE_LOOP('',(#29429,#29430,#29431));
#7081=EDGE_LOOP('',(#29432,#29433,#29434,#29435));
#7082=EDGE_LOOP('',(#29436,#29437,#29438));
#7083=EDGE_LOOP('',(#29439,#29440,#29441,#29442));
#7084=EDGE_LOOP('',(#29443,#29444,#29445));
#7085=EDGE_LOOP('',(#29446,#29447,#29448,#29449));
#7086=EDGE_LOOP('',(#29450,#29451,#29452));
#7087=EDGE_LOOP('',(#29453,#29454,#29455,#29456));
#7088=EDGE_LOOP('',(#29457,#29458,#29459,#29460));
#7089=EDGE_LOOP('',(#29461,#29462,#29463,#29464));
#7090=EDGE_LOOP('',(#29465,#29466,#29467,#29468));
#7091=EDGE_LOOP('',(#29469,#29470,#29471,#29472));
#7092=EDGE_LOOP('',(#29473,#29474,#29475,#29476));
#7093=EDGE_LOOP('',(#29477,#29478,#29479,#29480));
#7094=EDGE_LOOP('',(#29481,#29482,#29483,#29484));
#7095=EDGE_LOOP('',(#29485,#29486,#29487,#29488));
#7096=EDGE_LOOP('',(#29489,#29490,#29491,#29492));
#7097=EDGE_LOOP('',(#29493,#29494,#29495));
#7098=EDGE_LOOP('',(#29496,#29497,#29498,#29499));
#7099=EDGE_LOOP('',(#29500,#29501,#29502,#29503));
#7100=EDGE_LOOP('',(#29504,#29505,#29506,#29507));
#7101=EDGE_LOOP('',(#29508,#29509,#29510));
#7102=EDGE_LOOP('',(#29511,#29512,#29513,#29514));
#7103=EDGE_LOOP('',(#29515,#29516,#29517,#29518));
#7104=EDGE_LOOP('',(#29519,#29520,#29521,#29522));
#7105=EDGE_LOOP('',(#29523,#29524,#29525,#29526));
#7106=EDGE_LOOP('',(#29527,#29528,#29529,#29530));
#7107=EDGE_LOOP('',(#29531,#29532,#29533,#29534));
#7108=EDGE_LOOP('',(#29535,#29536,#29537,#29538));
#7109=EDGE_LOOP('',(#29539,#29540,#29541,#29542,#29543,#29544,#29545,#29546,
#29547,#29548,#29549,#29550,#29551,#29552));
#7110=EDGE_LOOP('',(#29553,#29554,#29555,#29556));
#7111=EDGE_LOOP('',(#29557,#29558,#29559,#29560,#29561));
#7112=EDGE_LOOP('',(#29562,#29563,#29564,#29565));
#7113=EDGE_LOOP('',(#29566,#29567,#29568,#29569,#29570,#29571));
#7114=EDGE_LOOP('',(#29572,#29573,#29574,#29575));
#7115=EDGE_LOOP('',(#29576,#29577,#29578,#29579,#29580,#29581));
#7116=EDGE_LOOP('',(#29582,#29583,#29584,#29585));
#7117=EDGE_LOOP('',(#29586,#29587,#29588));
#7118=EDGE_LOOP('',(#29589,#29590,#29591,#29592));
#7119=EDGE_LOOP('',(#29593,#29594,#29595,#29596,#29597,#29598,#29599,#29600,
#29601,#29602,#29603,#29604,#29605,#29606,#29607,#29608));
#7120=EDGE_LOOP('',(#29609,#29610,#29611,#29612));
#7121=EDGE_LOOP('',(#29613,#29614,#29615,#29616,#29617,#29618,#29619,#29620,
#29621));
#7122=EDGE_LOOP('',(#29622,#29623,#29624,#29625));
#7123=EDGE_LOOP('',(#29626,#29627,#29628,#29629));
#7124=EDGE_LOOP('',(#29630,#29631,#29632,#29633));
#7125=EDGE_LOOP('',(#29634,#29635,#29636,#29637));
#7126=EDGE_LOOP('',(#29638,#29639,#29640,#29641));
#7127=EDGE_LOOP('',(#29642,#29643,#29644,#29645));
#7128=EDGE_LOOP('',(#29646,#29647,#29648,#29649));
#7129=EDGE_LOOP('',(#29650,#29651,#29652,#29653));
#7130=EDGE_LOOP('',(#29654,#29655,#29656,#29657));
#7131=EDGE_LOOP('',(#29658,#29659,#29660,#29661));
#7132=EDGE_LOOP('',(#29662,#29663,#29664,#29665));
#7133=EDGE_LOOP('',(#29666,#29667,#29668,#29669));
#7134=EDGE_LOOP('',(#29670,#29671,#29672,#29673));
#7135=EDGE_LOOP('',(#29674,#29675,#29676,#29677));
#7136=EDGE_LOOP('',(#29678,#29679,#29680,#29681));
#7137=EDGE_LOOP('',(#29682,#29683,#29684,#29685));
#7138=EDGE_LOOP('',(#29686,#29687,#29688,#29689));
#7139=EDGE_LOOP('',(#29690,#29691,#29692,#29693));
#7140=EDGE_LOOP('',(#29694,#29695,#29696,#29697,#29698));
#7141=EDGE_LOOP('',(#29699,#29700,#29701,#29702));
#7142=EDGE_LOOP('',(#29703,#29704,#29705,#29706));
#7143=EDGE_LOOP('',(#29707,#29708,#29709,#29710));
#7144=EDGE_LOOP('',(#29711,#29712,#29713,#29714,#29715,#29716,#29717));
#7145=EDGE_LOOP('',(#29718,#29719,#29720,#29721));
#7146=EDGE_LOOP('',(#29722,#29723,#29724,#29725));
#7147=EDGE_LOOP('',(#29726,#29727,#29728,#29729));
#7148=EDGE_LOOP('',(#29730,#29731,#29732,#29733));
#7149=EDGE_LOOP('',(#29734,#29735,#29736,#29737));
#7150=EDGE_LOOP('',(#29738,#29739,#29740,#29741));
#7151=EDGE_LOOP('',(#29742,#29743,#29744,#29745,#29746,#29747,#29748,#29749));
#7152=EDGE_LOOP('',(#29750,#29751,#29752,#29753));
#7153=EDGE_LOOP('',(#29754,#29755,#29756,#29757));
#7154=EDGE_LOOP('',(#29758,#29759,#29760,#29761));
#7155=EDGE_LOOP('',(#29762,#29763,#29764,#29765));
#7156=EDGE_LOOP('',(#29766,#29767,#29768,#29769));
#7157=EDGE_LOOP('',(#29770,#29771,#29772,#29773));
#7158=EDGE_LOOP('',(#29774,#29775,#29776,#29777));
#7159=EDGE_LOOP('',(#29778,#29779,#29780,#29781));
#7160=EDGE_LOOP('',(#29782,#29783,#29784,#29785));
#7161=EDGE_LOOP('',(#29786,#29787,#29788,#29789));
#7162=EDGE_LOOP('',(#29790,#29791,#29792));
#7163=EDGE_LOOP('',(#29793,#29794,#29795,#29796));
#7164=EDGE_LOOP('',(#29797,#29798,#29799));
#7165=EDGE_LOOP('',(#29800,#29801,#29802));
#7166=EDGE_LOOP('',(#29803,#29804,#29805));
#7167=EDGE_LOOP('',(#29806,#29807,#29808,#29809));
#7168=EDGE_LOOP('',(#29810,#29811,#29812,#29813));
#7169=EDGE_LOOP('',(#29814,#29815,#29816,#29817));
#7170=EDGE_LOOP('',(#29818,#29819,#29820,#29821));
#7171=EDGE_LOOP('',(#29822,#29823,#29824,#29825));
#7172=EDGE_LOOP('',(#29826,#29827,#29828,#29829));
#7173=EDGE_LOOP('',(#29830,#29831,#29832));
#7174=EDGE_LOOP('',(#29833,#29834,#29835,#29836));
#7175=EDGE_LOOP('',(#29837,#29838,#29839,#29840));
#7176=EDGE_LOOP('',(#29841,#29842,#29843));
#7177=EDGE_LOOP('',(#29844,#29845,#29846));
#7178=EDGE_LOOP('',(#29847,#29848,#29849,#29850));
#7179=EDGE_LOOP('',(#29851,#29852,#29853,#29854));
#7180=EDGE_LOOP('',(#29855,#29856,#29857,#29858));
#7181=EDGE_LOOP('',(#29859,#29860));
#7182=EDGE_LOOP('',(#29861,#29862,#29863,#29864));
#7183=EDGE_LOOP('',(#29865,#29866,#29867,#29868));
#7184=EDGE_LOOP('',(#29869,#29870,#29871,#29872));
#7185=EDGE_LOOP('',(#29873,#29874,#29875,#29876));
#7186=EDGE_LOOP('',(#29877,#29878,#29879,#29880));
#7187=EDGE_LOOP('',(#29881,#29882,#29883,#29884));
#7188=EDGE_LOOP('',(#29885,#29886,#29887,#29888));
#7189=EDGE_LOOP('',(#29889,#29890,#29891,#29892));
#7190=EDGE_LOOP('',(#29893,#29894,#29895,#29896));
#7191=EDGE_LOOP('',(#29897,#29898,#29899,#29900));
#7192=EDGE_LOOP('',(#29901,#29902,#29903,#29904));
#7193=EDGE_LOOP('',(#29905,#29906,#29907,#29908));
#7194=EDGE_LOOP('',(#29909,#29910,#29911,#29912));
#7195=EDGE_LOOP('',(#29913,#29914,#29915,#29916));
#7196=EDGE_LOOP('',(#29917,#29918,#29919,#29920));
#7197=EDGE_LOOP('',(#29921,#29922,#29923,#29924));
#7198=EDGE_LOOP('',(#29925,#29926,#29927,#29928));
#7199=EDGE_LOOP('',(#29929,#29930,#29931,#29932));
#7200=EDGE_LOOP('',(#29933,#29934,#29935,#29936,#29937,#29938,#29939,#29940,
#29941,#29942,#29943,#29944,#29945,#29946,#29947));
#7201=EDGE_LOOP('',(#29948,#29949,#29950,#29951,#29952,#29953,#29954,#29955,
#29956,#29957,#29958,#29959,#29960,#29961,#29962,#29963));
#7202=EDGE_LOOP('',(#29964,#29965,#29966));
#7203=EDGE_LOOP('',(#29967,#29968,#29969,#29970));
#7204=EDGE_LOOP('',(#29971,#29972,#29973,#29974));
#7205=EDGE_LOOP('',(#29975,#29976,#29977,#29978));
#7206=EDGE_LOOP('',(#29979,#29980,#29981));
#7207=EDGE_LOOP('',(#29982,#29983,#29984,#29985));
#7208=EDGE_LOOP('',(#29986,#29987,#29988,#29989));
#7209=EDGE_LOOP('',(#29990,#29991,#29992,#29993,#29994,#29995));
#7210=EDGE_LOOP('',(#29996,#29997,#29998,#29999));
#7211=EDGE_LOOP('',(#30000,#30001,#30002,#30003));
#7212=EDGE_LOOP('',(#30004,#30005,#30006,#30007));
#7213=EDGE_LOOP('',(#30008,#30009,#30010));
#7214=EDGE_LOOP('',(#30011,#30012,#30013,#30014));
#7215=EDGE_LOOP('',(#30015,#30016,#30017,#30018));
#7216=EDGE_LOOP('',(#30019,#30020,#30021,#30022));
#7217=EDGE_LOOP('',(#30023,#30024,#30025,#30026));
#7218=EDGE_LOOP('',(#30027,#30028,#30029,#30030,#30031,#30032));
#7219=EDGE_LOOP('',(#30033,#30034,#30035,#30036));
#7220=EDGE_LOOP('',(#30037,#30038,#30039,#30040,#30041,#30042,#30043,#30044,
#30045,#30046,#30047,#30048,#30049,#30050));
#7221=EDGE_LOOP('',(#30051,#30052,#30053,#30054,#30055));
#7222=EDGE_LOOP('',(#30056,#30057,#30058,#30059));
#7223=EDGE_LOOP('',(#30060,#30061,#30062,#30063));
#7224=EDGE_LOOP('',(#30064,#30065,#30066,#30067));
#7225=EDGE_LOOP('',(#30068,#30069,#30070,#30071));
#7226=EDGE_LOOP('',(#30072,#30073,#30074,#30075,#30076,#30077,#30078));
#7227=EDGE_LOOP('',(#30079,#30080,#30081,#30082));
#7228=EDGE_LOOP('',(#30083,#30084,#30085));
#7229=EDGE_LOOP('',(#30086,#30087,#30088,#30089,#30090,#30091,#30092,#30093));
#7230=EDGE_LOOP('',(#30094,#30095,#30096,#30097));
#7231=EDGE_LOOP('',(#30098,#30099,#30100,#30101));
#7232=EDGE_LOOP('',(#30102,#30103,#30104));
#7233=EDGE_LOOP('',(#30105,#30106,#30107,#30108));
#7234=EDGE_LOOP('',(#30109,#30110,#30111,#30112,#30113,#30114));
#7235=EDGE_LOOP('',(#30115,#30116,#30117,#30118));
#7236=EDGE_LOOP('',(#30119,#30120,#30121,#30122));
#7237=EDGE_LOOP('',(#30123,#30124,#30125,#30126));
#7238=EDGE_LOOP('',(#30127,#30128,#30129,#30130));
#7239=EDGE_LOOP('',(#30131,#30132,#30133,#30134));
#7240=EDGE_LOOP('',(#30135,#30136,#30137,#30138));
#7241=EDGE_LOOP('',(#30139,#30140,#30141,#30142));
#7242=EDGE_LOOP('',(#30143,#30144,#30145,#30146));
#7243=EDGE_LOOP('',(#30147,#30148,#30149,#30150));
#7244=EDGE_LOOP('',(#30151,#30152,#30153,#30154));
#7245=EDGE_LOOP('',(#30155,#30156,#30157,#30158));
#7246=EDGE_LOOP('',(#30159,#30160,#30161,#30162));
#7247=EDGE_LOOP('',(#30163,#30164,#30165,#30166));
#7248=EDGE_LOOP('',(#30167,#30168,#30169,#30170));
#7249=EDGE_LOOP('',(#30171,#30172,#30173,#30174));
#7250=EDGE_LOOP('',(#30175,#30176,#30177,#30178));
#7251=EDGE_LOOP('',(#30179,#30180,#30181,#30182));
#7252=EDGE_LOOP('',(#30183,#30184,#30185,#30186));
#7253=EDGE_LOOP('',(#30187,#30188,#30189,#30190));
#7254=EDGE_LOOP('',(#30191,#30192,#30193,#30194));
#7255=EDGE_LOOP('',(#30195,#30196,#30197,#30198));
#7256=EDGE_LOOP('',(#30199,#30200,#30201,#30202));
#7257=EDGE_LOOP('',(#30203,#30204,#30205,#30206));
#7258=EDGE_LOOP('',(#30207,#30208,#30209,#30210));
#7259=EDGE_LOOP('',(#30211,#30212,#30213,#30214));
#7260=EDGE_LOOP('',(#30215,#30216,#30217));
#7261=EDGE_LOOP('',(#30218,#30219,#30220,#30221));
#7262=EDGE_LOOP('',(#30222,#30223,#30224));
#7263=EDGE_LOOP('',(#30225,#30226,#30227));
#7264=EDGE_LOOP('',(#30228,#30229,#30230,#30231));
#7265=EDGE_LOOP('',(#30232,#30233,#30234,#30235));
#7266=EDGE_LOOP('',(#30236,#30237,#30238));
#7267=EDGE_LOOP('',(#30239,#30240,#30241));
#7268=EDGE_LOOP('',(#30242,#30243,#30244));
#7269=EDGE_LOOP('',(#30245,#30246,#30247,#30248));
#7270=EDGE_LOOP('',(#30249,#30250,#30251,#30252));
#7271=EDGE_LOOP('',(#30253,#30254,#30255,#30256));
#7272=EDGE_LOOP('',(#30257,#30258,#30259));
#7273=EDGE_LOOP('',(#30260,#30261,#30262,#30263));
#7274=EDGE_LOOP('',(#30264,#30265,#30266,#30267));
#7275=EDGE_LOOP('',(#30268,#30269,#30270));
#7276=EDGE_LOOP('',(#30271,#30272,#30273,#30274));
#7277=EDGE_LOOP('',(#30275,#30276,#30277,#30278));
#7278=EDGE_LOOP('',(#30279,#30280,#30281));
#7279=EDGE_LOOP('',(#30282,#30283,#30284,#30285));
#7280=EDGE_LOOP('',(#30286,#30287,#30288,#30289));
#7281=EDGE_LOOP('',(#30290,#30291,#30292));
#7282=EDGE_LOOP('',(#30293,#30294,#30295,#30296));
#7283=EDGE_LOOP('',(#30297,#30298,#30299,#30300));
#7284=EDGE_LOOP('',(#30301,#30302,#30303,#30304));
#7285=EDGE_LOOP('',(#30305,#30306,#30307,#30308));
#7286=EDGE_LOOP('',(#30309,#30310,#30311,#30312));
#7287=EDGE_LOOP('',(#30313,#30314,#30315,#30316));
#7288=EDGE_LOOP('',(#30317,#30318,#30319,#30320));
#7289=EDGE_LOOP('',(#30321,#30322,#30323,#30324));
#7290=EDGE_LOOP('',(#30325,#30326,#30327,#30328,#30329,#30330,#30331,#30332,
#30333,#30334,#30335,#30336,#30337,#30338,#30339,#30340,#30341,#30342,#30343,
#30344,#30345,#30346));
#7291=EDGE_LOOP('',(#30347,#30348,#30349,#30350,#30351));
#7292=EDGE_LOOP('',(#30352,#30353,#30354,#30355));
#7293=EDGE_LOOP('',(#30356,#30357,#30358));
#7294=EDGE_LOOP('',(#30359,#30360,#30361));
#7295=EDGE_LOOP('',(#30362,#30363,#30364,#30365));
#7296=EDGE_LOOP('',(#30366,#30367,#30368,#30369));
#7297=EDGE_LOOP('',(#30370,#30371,#30372,#30373));
#7298=EDGE_LOOP('',(#30374,#30375,#30376,#30377));
#7299=EDGE_LOOP('',(#30378,#30379,#30380,#30381));
#7300=EDGE_LOOP('',(#30382,#30383,#30384,#30385));
#7301=EDGE_LOOP('',(#30386,#30387,#30388));
#7302=EDGE_LOOP('',(#30389,#30390,#30391,#30392));
#7303=EDGE_LOOP('',(#30393,#30394,#30395,#30396));
#7304=EDGE_LOOP('',(#30397,#30398,#30399,#30400));
#7305=EDGE_LOOP('',(#30401,#30402,#30403));
#7306=EDGE_LOOP('',(#30404,#30405,#30406,#30407));
#7307=EDGE_LOOP('',(#30408,#30409,#30410,#30411));
#7308=EDGE_LOOP('',(#30412,#30413,#30414,#30415));
#7309=EDGE_LOOP('',(#30416,#30417,#30418,#30419));
#7310=EDGE_LOOP('',(#30420,#30421,#30422,#30423));
#7311=EDGE_LOOP('',(#30424,#30425,#30426,#30427));
#7312=EDGE_LOOP('',(#30428,#30429,#30430));
#7313=EDGE_LOOP('',(#30431,#30432,#30433,#30434));
#7314=EDGE_LOOP('',(#30435,#30436,#30437,#30438));
#7315=EDGE_LOOP('',(#30439,#30440,#30441,#30442));
#7316=EDGE_LOOP('',(#30443,#30444,#30445,#30446));
#7317=EDGE_LOOP('',(#30447,#30448,#30449,#30450));
#7318=EDGE_LOOP('',(#30451,#30452,#30453,#30454));
#7319=EDGE_LOOP('',(#30455,#30456,#30457,#30458,#30459));
#7320=EDGE_LOOP('',(#30460,#30461,#30462,#30463));
#7321=EDGE_LOOP('',(#30464,#30465,#30466,#30467));
#7322=EDGE_LOOP('',(#30468,#30469,#30470,#30471));
#7323=EDGE_LOOP('',(#30472,#30473,#30474,#30475));
#7324=EDGE_LOOP('',(#30476,#30477,#30478,#30479));
#7325=EDGE_LOOP('',(#30480,#30481,#30482,#30483));
#7326=EDGE_LOOP('',(#30484,#30485,#30486,#30487));
#7327=EDGE_LOOP('',(#30488,#30489,#30490,#30491));
#7328=EDGE_LOOP('',(#30492,#30493,#30494,#30495));
#7329=EDGE_LOOP('',(#30496,#30497,#30498,#30499));
#7330=EDGE_LOOP('',(#30500,#30501,#30502,#30503));
#7331=EDGE_LOOP('',(#30504,#30505,#30506,#30507));
#7332=EDGE_LOOP('',(#30508,#30509,#30510,#30511));
#7333=EDGE_LOOP('',(#30512,#30513,#30514,#30515));
#7334=EDGE_LOOP('',(#30516,#30517,#30518,#30519));
#7335=EDGE_LOOP('',(#30520,#30521,#30522,#30523));
#7336=EDGE_LOOP('',(#30524,#30525,#30526,#30527));
#7337=EDGE_LOOP('',(#30528,#30529,#30530,#30531));
#7338=EDGE_LOOP('',(#30532,#30533,#30534,#30535,#30536,#30537,#30538,#30539,
#30540,#30541,#30542,#30543,#30544,#30545,#30546,#30547,#30548,#30549,#30550,
#30551,#30552,#30553,#30554,#30555,#30556,#30557,#30558,#30559,#30560,#30561,
#30562,#30563,#30564,#30565,#30566,#30567,#30568,#30569,#30570,#30571,#30572,
#30573,#30574,#30575,#30576,#30577,#30578,#30579,#30580,#30581,#30582,#30583,
#30584,#30585,#30586,#30587,#30588,#30589,#30590));
#7339=EDGE_LOOP('',(#30591,#30592,#30593,#30594,#30595,#30596,#30597,#30598));
#7340=EDGE_LOOP('',(#30599,#30600,#30601,#30602,#30603,#30604,#30605,#30606));
#7341=EDGE_LOOP('',(#30607,#30608,#30609,#30610,#30611,#30612,#30613,#30614));
#7342=EDGE_LOOP('',(#30615,#30616,#30617,#30618,#30619,#30620,#30621,#30622,
#30623,#30624,#30625,#30626,#30627,#30628,#30629,#30630,#30631,#30632,#30633,
#30634,#30635,#30636,#30637,#30638,#30639,#30640,#30641,#30642,#30643,#30644,
#30645,#30646,#30647,#30648,#30649,#30650,#30651,#30652,#30653,#30654,#30655,
#30656));
#7343=EDGE_LOOP('',(#30657,#30658,#30659,#30660,#30661,#30662,#30663,#30664));
#7344=EDGE_LOOP('',(#30665,#30666,#30667,#30668));
#7345=EDGE_LOOP('',(#30669,#30670,#30671,#30672));
#7346=EDGE_LOOP('',(#30673,#30674,#30675,#30676));
#7347=EDGE_LOOP('',(#30677,#30678,#30679,#30680,#30681));
#7348=EDGE_LOOP('',(#30682,#30683,#30684,#30685));
#7349=EDGE_LOOP('',(#30686,#30687,#30688,#30689));
#7350=EDGE_LOOP('',(#30690,#30691,#30692,#30693));
#7351=EDGE_LOOP('',(#30694,#30695,#30696,#30697));
#7352=EDGE_LOOP('',(#30698,#30699,#30700,#30701));
#7353=EDGE_LOOP('',(#30702,#30703,#30704,#30705));
#7354=EDGE_LOOP('',(#30706,#30707,#30708));
#7355=EDGE_LOOP('',(#30709,#30710,#30711,#30712,#30713));
#7356=EDGE_LOOP('',(#30714,#30715,#30716,#30717,#30718,#30719));
#7357=EDGE_LOOP('',(#30720,#30721,#30722,#30723));
#7358=EDGE_LOOP('',(#30724,#30725,#30726,#30727,#30728,#30729));
#7359=EDGE_LOOP('',(#30730,#30731,#30732,#30733));
#7360=EDGE_LOOP('',(#30734,#30735,#30736,#30737));
#7361=EDGE_LOOP('',(#30738,#30739,#30740,#30741));
#7362=EDGE_LOOP('',(#30742,#30743,#30744,#30745));
#7363=EDGE_LOOP('',(#30746,#30747,#30748,#30749));
#7364=EDGE_LOOP('',(#30750,#30751,#30752,#30753));
#7365=EDGE_LOOP('',(#30754,#30755,#30756,#30757));
#7366=EDGE_LOOP('',(#30758,#30759,#30760,#30761,#30762,#30763));
#7367=EDGE_LOOP('',(#30764,#30765,#30766,#30767));
#7368=EDGE_LOOP('',(#30768,#30769,#30770));
#7369=EDGE_LOOP('',(#30771,#30772,#30773,#30774));
#7370=EDGE_LOOP('',(#30775,#30776,#30777,#30778));
#7371=EDGE_LOOP('',(#30779,#30780,#30781));
#7372=EDGE_LOOP('',(#30782,#30783,#30784,#30785));
#7373=EDGE_LOOP('',(#30786,#30787,#30788));
#7374=EDGE_LOOP('',(#30789,#30790,#30791,#30792));
#7375=EDGE_LOOP('',(#30793,#30794,#30795));
#7376=EDGE_LOOP('',(#30796,#30797,#30798,#30799));
#7377=EDGE_LOOP('',(#30800,#30801,#30802));
#7378=EDGE_LOOP('',(#30803,#30804,#30805,#30806));
#7379=EDGE_LOOP('',(#30807,#30808,#30809));
#7380=EDGE_LOOP('',(#30810,#30811,#30812,#30813));
#7381=EDGE_LOOP('',(#30814,#30815,#30816,#30817));
#7382=EDGE_LOOP('',(#30818,#30819,#30820,#30821));
#7383=EDGE_LOOP('',(#30822,#30823,#30824,#30825));
#7384=EDGE_LOOP('',(#30826,#30827,#30828,#30829));
#7385=EDGE_LOOP('',(#30830,#30831,#30832,#30833,#30834,#30835,#30836,#30837,
#30838,#30839,#30840));
#8812=LINE('',#85212,#10652);
#8813=LINE('',#85215,#10653);
#8814=LINE('',#85219,#10654);
#8815=LINE('',#85276,#10655);
#8816=LINE('',#85281,#10656);
#8817=LINE('',#85285,#10657);
#8818=LINE('',#85304,#10658);
#8819=LINE('',#85308,#10659);
#8820=LINE('',#85313,#10660);
#8821=LINE('',#85314,#10661);
#8822=LINE('',#85315,#10662);
#8823=LINE('',#85320,#10663);
#8824=LINE('',#85325,#10664);
#8825=LINE('',#85332,#10665);
#8826=LINE('',#85390,#10666);
#8827=LINE('',#85395,#10667);
#8828=LINE('',#85396,#10668);
#8829=LINE('',#85399,#10669);
#8830=LINE('',#85455,#10670);
#8831=LINE('',#85458,#10671);
#8832=LINE('',#85469,#10672);
#8833=LINE('',#85471,#10673);
#8834=LINE('',#85499,#10674);
#8835=LINE('',#85554,#10675);
#8836=LINE('',#85562,#10676);
#8837=LINE('',#85564,#10677);
#8838=LINE('',#85566,#10678);
#8839=LINE('',#85568,#10679);
#8840=LINE('',#85614,#10680);
#8841=LINE('',#85615,#10681);
#8842=LINE('',#85620,#10682);
#8843=LINE('',#85625,#10683);
#8844=LINE('',#85632,#10684);
#8845=LINE('',#85636,#10685);
#8846=LINE('',#85638,#10686);
#8847=LINE('',#85639,#10687);
#8848=LINE('',#85643,#10688);
#8849=LINE('',#85687,#10689);
#8850=LINE('',#85691,#10690);
#8851=LINE('',#85704,#10691);
#8852=LINE('',#85825,#10692);
#8853=LINE('',#85904,#10693);
#8854=LINE('',#86027,#10694);
#8855=LINE('',#86076,#10695);
#8856=LINE('',#86198,#10696);
#8857=LINE('',#86199,#10697);
#8858=LINE('',#86200,#10698);
#8859=LINE('',#86207,#10699);
#8860=LINE('',#86208,#10700);
#8861=LINE('',#86213,#10701);
#8862=LINE('',#86215,#10702);
#8863=LINE('',#86216,#10703);
#8864=LINE('',#86221,#10704);
#8865=LINE('',#86223,#10705);
#8866=LINE('',#86231,#10706);
#8867=LINE('',#86247,#10707);
#8868=LINE('',#86435,#10708);
#8869=LINE('',#86437,#10709);
#8870=LINE('',#86439,#10710);
#8871=LINE('',#86440,#10711);
#8872=LINE('',#86446,#10712);
#8873=LINE('',#86568,#10713);
#8874=LINE('',#86572,#10714);
#8875=LINE('',#86617,#10715);
#8876=LINE('',#86621,#10716);
#8877=LINE('',#86623,#10717);
#8878=LINE('',#86627,#10718);
#8879=LINE('',#86628,#10719);
#8880=LINE('',#86633,#10720);
#8881=LINE('',#86676,#10721);
#8882=LINE('',#86678,#10722);
#8883=LINE('',#86682,#10723);
#8884=LINE('',#86688,#10724);
#8885=LINE('',#86731,#10725);
#8886=LINE('',#86733,#10726);
#8887=LINE('',#86735,#10727);
#8888=LINE('',#86757,#10728);
#8889=LINE('',#86759,#10729);
#8890=LINE('',#86763,#10730);
#8891=LINE('',#86767,#10731);
#8892=LINE('',#86769,#10732);
#8893=LINE('',#86771,#10733);
#8894=LINE('',#86772,#10734);
#8895=LINE('',#86777,#10735);
#8896=LINE('',#86784,#10736);
#8897=LINE('',#86789,#10737);
#8898=LINE('',#86793,#10738);
#8899=LINE('',#86795,#10739);
#8900=LINE('',#86796,#10740);
#8901=LINE('',#86800,#10741);
#8902=LINE('',#86812,#10742);
#8903=LINE('',#86820,#10743);
#8904=LINE('',#86823,#10744);
#8905=LINE('',#86842,#10745);
#8906=LINE('',#86844,#10746);
#8907=LINE('',#86871,#10747);
#8908=LINE('',#86872,#10748);
#8909=LINE('',#87088,#10749);
#8910=LINE('',#87089,#10750);
#8911=LINE('',#87254,#10751);
#8912=LINE('',#87256,#10752);
#8913=LINE('',#87283,#10753);
#8914=LINE('',#87284,#10754);
#8915=LINE('',#87288,#10755);
#8916=LINE('',#87292,#10756);
#8917=LINE('',#87374,#10757);
#8918=LINE('',#87437,#10758);
#8919=LINE('',#87641,#10759);
#8920=LINE('',#87642,#10760);
#8921=LINE('',#87681,#10761);
#8922=LINE('',#87682,#10762);
#8923=LINE('',#87728,#10763);
#8924=LINE('',#87732,#10764);
#8925=LINE('',#87981,#10765);
#8926=LINE('',#87991,#10766);
#8927=LINE('',#88227,#10767);
#8928=LINE('',#88229,#10768);
#8929=LINE('',#88239,#10769);
#8930=LINE('',#88241,#10770);
#8931=LINE('',#88244,#10771);
#8932=LINE('',#88247,#10772);
#8933=LINE('',#88249,#10773);
#8934=LINE('',#88362,#10774);
#8935=LINE('',#88387,#10775);
#8936=LINE('',#88393,#10776);
#8937=LINE('',#88435,#10777);
#8938=LINE('',#88451,#10778);
#8939=LINE('',#88453,#10779);
#8940=LINE('',#88454,#10780);
#8941=LINE('',#88456,#10781);
#8942=LINE('',#88457,#10782);
#8943=LINE('',#88461,#10783);
#8944=LINE('',#88464,#10784);
#8945=LINE('',#88465,#10785);
#8946=LINE('',#88469,#10786);
#8947=LINE('',#88472,#10787);
#8948=LINE('',#88474,#10788);
#8949=LINE('',#88476,#10789);
#8950=LINE('',#88479,#10790);
#8951=LINE('',#88480,#10791);
#8952=LINE('',#88482,#10792);
#8953=LINE('',#88484,#10793);
#8954=LINE('',#88486,#10794);
#8955=LINE('',#88488,#10795);
#8956=LINE('',#88491,#10796);
#8957=LINE('',#88492,#10797);
#8958=LINE('',#88494,#10798);
#8959=LINE('',#88496,#10799);
#8960=LINE('',#88500,#10800);
#8961=LINE('',#88504,#10801);
#8962=LINE('',#88507,#10802);
#8963=LINE('',#88512,#10803);
#8964=LINE('',#88514,#10804);
#8965=LINE('',#88583,#10805);
#8966=LINE('',#88586,#10806);
#8967=LINE('',#88598,#10807);
#8968=LINE('',#88824,#10808);
#8969=LINE('',#88839,#10809);
#8970=LINE('',#88840,#10810);
#8971=LINE('',#88850,#10811);
#8972=LINE('',#88866,#10812);
#8973=LINE('',#88967,#10813);
#8974=LINE('',#88969,#10814);
#8975=LINE('',#88971,#10815);
#8976=LINE('',#88974,#10816);
#8977=LINE('',#88979,#10817);
#8978=LINE('',#88980,#10818);
#8979=LINE('',#88982,#10819);
#8980=LINE('',#88984,#10820);
#8981=LINE('',#89162,#10821);
#8982=LINE('',#89178,#10822);
#8983=LINE('',#89439,#10823);
#8984=LINE('',#89506,#10824);
#8985=LINE('',#89624,#10825);
#8986=LINE('',#89799,#10826);
#8987=LINE('',#89802,#10827);
#8988=LINE('',#89961,#10828);
#8989=LINE('',#89962,#10829);
#8990=LINE('',#89965,#10830);
#8991=LINE('',#89968,#10831);
#8992=LINE('',#89972,#10832);
#8993=LINE('',#89978,#10833);
#8994=LINE('',#89982,#10834);
#8995=LINE('',#89986,#10835);
#8996=LINE('',#89989,#10836);
#8997=LINE('',#89990,#10837);
#8998=LINE('',#89994,#10838);
#8999=LINE('',#89998,#10839);
#9000=LINE('',#90002,#10840);
#9001=LINE('',#90005,#10841);
#9002=LINE('',#90006,#10842);
#9003=LINE('',#90093,#10843);
#9004=LINE('',#90212,#10844);
#9005=LINE('',#90215,#10845);
#9006=LINE('',#90231,#10846);
#9007=LINE('',#90235,#10847);
#9008=LINE('',#90309,#10848);
#9009=LINE('',#90314,#10849);
#9010=LINE('',#90407,#10850);
#9011=LINE('',#90410,#10851);
#9012=LINE('',#90449,#10852);
#9013=LINE('',#90452,#10853);
#9014=LINE('',#90455,#10854);
#9015=LINE('',#90457,#10855);
#9016=LINE('',#90458,#10856);
#9017=LINE('',#90463,#10857);
#9018=LINE('',#90470,#10858);
#9019=LINE('',#90475,#10859);
#9020=LINE('',#90487,#10860);
#9021=LINE('',#90492,#10861);
#9022=LINE('',#90495,#10862);
#9023=LINE('',#90496,#10863);
#9024=LINE('',#90500,#10864);
#9025=LINE('',#90503,#10865);
#9026=LINE('',#90517,#10866);
#9027=LINE('',#90518,#10867);
#9028=LINE('',#90546,#10868);
#9029=LINE('',#90557,#10869);
#9030=LINE('',#90566,#10870);
#9031=LINE('',#90568,#10871);
#9032=LINE('',#90614,#10872);
#9033=LINE('',#90616,#10873);
#9034=LINE('',#90618,#10874);
#9035=LINE('',#90619,#10875);
#9036=LINE('',#90624,#10876);
#9037=LINE('',#90631,#10877);
#9038=LINE('',#90636,#10878);
#9039=LINE('',#90640,#10879);
#9040=LINE('',#90642,#10880);
#9041=LINE('',#90643,#10881);
#9042=LINE('',#90649,#10882);
#9043=LINE('',#90653,#10883);
#9044=LINE('',#90661,#10884);
#9045=LINE('',#90673,#10885);
#9046=LINE('',#90917,#10886);
#9047=LINE('',#91058,#10887);
#9048=LINE('',#91182,#10888);
#9049=LINE('',#91251,#10889);
#9050=LINE('',#91320,#10890);
#9051=LINE('',#91322,#10891);
#9052=LINE('',#91323,#10892);
#9053=LINE('',#91328,#10893);
#9054=LINE('',#91330,#10894);
#9055=LINE('',#91337,#10895);
#9056=LINE('',#91338,#10896);
#9057=LINE('',#91339,#10897);
#9058=LINE('',#91346,#10898);
#9059=LINE('',#91347,#10899);
#9060=LINE('',#91354,#10900);
#9061=LINE('',#91370,#10901);
#9062=LINE('',#91608,#10902);
#9063=LINE('',#91613,#10903);
#9064=LINE('',#91614,#10904);
#9065=LINE('',#91615,#10905);
#9066=LINE('',#91618,#10906);
#9067=LINE('',#91667,#10907);
#9068=LINE('',#91671,#10908);
#9069=LINE('',#91793,#10909);
#9070=LINE('',#91800,#10910);
#9071=LINE('',#91803,#10911);
#9072=LINE('',#91807,#10912);
#9073=LINE('',#91808,#10913);
#9074=LINE('',#91850,#10914);
#9075=LINE('',#91855,#10915);
#9076=LINE('',#91859,#10916);
#9077=LINE('',#91860,#10917);
#9078=LINE('',#91902,#10918);
#9079=LINE('',#91915,#10919);
#9080=LINE('',#91917,#10920);
#9081=LINE('',#91918,#10921);
#9082=LINE('',#91934,#10922);
#9083=LINE('',#91936,#10923);
#9084=LINE('',#91988,#10924);
#9085=LINE('',#91992,#10925);
#9086=LINE('',#91995,#10926);
#9087=LINE('',#91997,#10927);
#9088=LINE('',#91999,#10928);
#9089=LINE('',#92001,#10929);
#9090=LINE('',#92004,#10930);
#9091=LINE('',#92009,#10931);
#9092=LINE('',#92014,#10932);
#9093=LINE('',#92021,#10933);
#9094=LINE('',#92026,#10934);
#9095=LINE('',#92027,#10935);
#9096=LINE('',#92028,#10936);
#9097=LINE('',#92064,#10937);
#9098=LINE('',#92069,#10938);
#9099=LINE('',#92078,#10939);
#9100=LINE('',#92081,#10940);
#9101=LINE('',#92101,#10941);
#9102=LINE('',#92102,#10942);
#9103=LINE('',#92128,#10943);
#9104=LINE('',#92129,#10944);
#9105=LINE('',#92336,#10945);
#9106=LINE('',#92337,#10946);
#9107=LINE('',#92504,#10947);
#9108=LINE('',#92505,#10948);
#9109=LINE('',#92531,#10949);
#9110=LINE('',#92532,#10950);
#9111=LINE('',#92613,#10951);
#9112=LINE('',#92673,#10952);
#9113=LINE('',#92676,#10953);
#9114=LINE('',#92679,#10954);
#9115=LINE('',#92961,#10955);
#9116=LINE('',#92962,#10956);
#9117=LINE('',#93057,#10957);
#9118=LINE('',#93060,#10958);
#9119=LINE('',#93221,#10959);
#9120=LINE('',#93224,#10960);
#9121=LINE('',#93252,#10961);
#9122=LINE('',#93258,#10962);
#9123=LINE('',#93266,#10963);
#9124=LINE('',#93274,#10964);
#9125=LINE('',#93284,#10965);
#9126=LINE('',#93293,#10966);
#9127=LINE('',#93301,#10967);
#9128=LINE('',#93309,#10968);
#9129=LINE('',#93315,#10969);
#9130=LINE('',#93318,#10970);
#9131=LINE('',#93533,#10971);
#9132=LINE('',#93813,#10972);
#9133=LINE('',#93816,#10973);
#9134=LINE('',#93819,#10974);
#9135=LINE('',#93821,#10975);
#9136=LINE('',#93838,#10976);
#9137=LINE('',#93849,#10977);
#9138=LINE('',#93854,#10978);
#9139=LINE('',#93862,#10979);
#9140=LINE('',#93872,#10980);
#9141=LINE('',#93874,#10981);
#9142=LINE('',#94019,#10982);
#9143=LINE('',#94026,#10983);
#9144=LINE('',#94064,#10984);
#9145=LINE('',#94066,#10985);
#9146=LINE('',#94067,#10986);
#9147=LINE('',#94069,#10987);
#9148=LINE('',#94070,#10988);
#9149=LINE('',#94073,#10989);
#9150=LINE('',#94077,#10990);
#9151=LINE('',#94078,#10991);
#9152=LINE('',#94081,#10992);
#9153=LINE('',#94084,#10993);
#9154=LINE('',#94087,#10994);
#9155=LINE('',#94089,#10995);
#9156=LINE('',#94092,#10996);
#9157=LINE('',#94093,#10997);
#9158=LINE('',#94095,#10998);
#9159=LINE('',#94097,#10999);
#9160=LINE('',#94099,#11000);
#9161=LINE('',#94101,#11001);
#9162=LINE('',#94104,#11002);
#9163=LINE('',#94105,#11003);
#9164=LINE('',#94107,#11004);
#9165=LINE('',#94109,#11005);
#9166=LINE('',#94112,#11006);
#9167=LINE('',#94116,#11007);
#9168=LINE('',#94121,#11008);
#9169=LINE('',#94124,#11009);
#9170=LINE('',#94127,#11010);
#9171=LINE('',#94211,#11011);
#9172=LINE('',#94215,#11012);
#9173=LINE('',#94226,#11013);
#9174=LINE('',#94404,#11014);
#9175=LINE('',#94416,#11015);
#9176=LINE('',#94417,#11016);
#9177=LINE('',#94425,#11017);
#9178=LINE('',#94442,#11018);
#9179=LINE('',#94447,#11019);
#9180=LINE('',#94683,#11020);
#9181=LINE('',#94685,#11021);
#9182=LINE('',#94687,#11022);
#9183=LINE('',#94692,#11023);
#9184=LINE('',#94696,#11024);
#9185=LINE('',#94698,#11025);
#9186=LINE('',#94700,#11026);
#9187=LINE('',#94831,#11027);
#9188=LINE('',#94847,#11028);
#9189=LINE('',#95057,#11029);
#9190=LINE('',#95159,#11030);
#9191=LINE('',#95242,#11031);
#9192=LINE('',#95251,#11032);
#9193=LINE('',#95255,#11033);
#9194=LINE('',#95258,#11034);
#9195=LINE('',#95262,#11035);
#9196=LINE('',#95272,#11036);
#9197=LINE('',#95278,#11037);
#9198=LINE('',#95280,#11038);
#9199=LINE('',#95283,#11039);
#9200=LINE('',#95289,#11040);
#9201=LINE('',#95297,#11041);
#9202=LINE('',#95552,#11042);
#9203=LINE('',#95690,#11043);
#9204=LINE('',#95693,#11044);
#9205=LINE('',#95696,#11045);
#9206=LINE('',#95699,#11046);
#9207=LINE('',#95705,#11047);
#9208=LINE('',#95709,#11048);
#9209=LINE('',#95713,#11049);
#9210=LINE('',#95717,#11050);
#9211=LINE('',#95718,#11051);
#9212=LINE('',#95721,#11052);
#9213=LINE('',#95725,#11053);
#9214=LINE('',#95729,#11054);
#9215=LINE('',#95733,#11055);
#9216=LINE('',#95734,#11056);
#9217=LINE('',#95768,#11057);
#9218=LINE('',#95778,#11058);
#9219=LINE('',#95782,#11059);
#10652=VECTOR('',#44421,1000.);
#10653=VECTOR('',#44424,1000.);
#10654=VECTOR('',#44427,1000.);
#10655=VECTOR('',#44436,1000.);
#10656=VECTOR('',#44441,1000.);
#10657=VECTOR('',#44444,1000.);
#10658=VECTOR('',#44447,1000.);
#10659=VECTOR('',#44450,1000.);
#10660=VECTOR('',#44455,1000.);
#10661=VECTOR('',#44456,1000.);
#10662=VECTOR('',#44457,1000.);
#10663=VECTOR('',#44462,1000.);
#10664=VECTOR('',#44467,1000.);
#10665=VECTOR('',#44476,1000.);
#10666=VECTOR('',#44477,1000.);
#10667=VECTOR('',#44482,1000.);
#10668=VECTOR('',#44483,1000.);
#10669=VECTOR('',#44486,1000.);
#10670=VECTOR('',#44489,1000.);
#10671=VECTOR('',#44492,1000.);
#10672=VECTOR('',#44509,1000.);
#10673=VECTOR('',#44510,1000.);
#10674=VECTOR('',#44551,1000.);
#10675=VECTOR('',#44570,1000.);
#10676=VECTOR('',#44579,1000.);
#10677=VECTOR('',#44580,1000.);
#10678=VECTOR('',#44581,1000.);
#10679=VECTOR('',#44582,1000.);
#10680=VECTOR('',#44583,1000.);
#10681=VECTOR('',#44584,1000.);
#10682=VECTOR('',#44589,1000.);
#10683=VECTOR('',#44594,1000.);
#10684=VECTOR('',#44603,1000.);
#10685=VECTOR('',#44608,1000.);
#10686=VECTOR('',#44609,1000.);
#10687=VECTOR('',#44610,1000.);
#10688=VECTOR('',#44613,1000.);
#10689=VECTOR('',#44622,1000.);
#10690=VECTOR('',#44625,1000.);
#10691=VECTOR('',#44646,1000.);
#10692=VECTOR('',#44673,1000.);
#10693=VECTOR('',#44674,1000.);
#10694=VECTOR('',#44685,1000.);
#10695=VECTOR('',#44686,1000.);
#10696=VECTOR('',#44703,1000.);
#10697=VECTOR('',#44704,1000.);
#10698=VECTOR('',#44705,1000.);
#10699=VECTOR('',#44714,1000.);
#10700=VECTOR('',#44715,1000.);
#10701=VECTOR('',#44722,1000.);
#10702=VECTOR('',#44723,1000.);
#10703=VECTOR('',#44724,1000.);
#10704=VECTOR('',#44731,1000.);
#10705=VECTOR('',#44732,1000.);
#10706=VECTOR('',#44743,1000.);
#10707=VECTOR('',#44766,1000.);
#10708=VECTOR('',#44827,1000.);
#10709=VECTOR('',#44828,1000.);
#10710=VECTOR('',#44829,1000.);
#10711=VECTOR('',#44830,1000.);
#10712=VECTOR('',#44835,1000.);
#10713=VECTOR('',#44838,1000.);
#10714=VECTOR('',#44841,1000.);
#10715=VECTOR('',#44846,1000.);
#10716=VECTOR('',#44849,1000.);
#10717=VECTOR('',#44850,1000.);
#10718=VECTOR('',#44853,1000.);
#10719=VECTOR('',#44854,1000.);
#10720=VECTOR('',#44859,1000.);
#10721=VECTOR('',#44862,1000.);
#10722=VECTOR('',#44863,1000.);
#10723=VECTOR('',#44866,1000.);
#10724=VECTOR('',#44873,1000.);
#10725=VECTOR('',#44876,1000.);
#10726=VECTOR('',#44877,1000.);
#10727=VECTOR('',#44878,1000.);
#10728=VECTOR('',#44901,1000.);
#10729=VECTOR('',#44902,1000.);
#10730=VECTOR('',#44907,1000.);
#10731=VECTOR('',#44910,1000.);
#10732=VECTOR('',#44911,1000.);
#10733=VECTOR('',#44912,1000.);
#10734=VECTOR('',#44913,1000.);
#10735=VECTOR('',#44918,1000.);
#10736=VECTOR('',#44927,1000.);
#10737=VECTOR('',#44932,1000.);
#10738=VECTOR('',#44937,1000.);
#10739=VECTOR('',#44938,1000.);
#10740=VECTOR('',#44939,1000.);
#10741=VECTOR('',#44942,1000.);
#10742=VECTOR('',#44949,1000.);
#10743=VECTOR('',#44960,1000.);
#10744=VECTOR('',#44963,1000.);
#10745=VECTOR('',#44986,1000.);
#10746=VECTOR('',#44987,1000.);
#10747=VECTOR('',#45024,1000.);
#10748=VECTOR('',#45025,1000.);
#10749=VECTOR('',#45084,1000.);
#10750=VECTOR('',#45085,1000.);
#10751=VECTOR('',#45120,1000.);
#10752=VECTOR('',#45121,1000.);
#10753=VECTOR('',#45158,1000.);
#10754=VECTOR('',#45159,1000.);
#10755=VECTOR('',#45162,1000.);
#10756=VECTOR('',#45165,1000.);
#10757=VECTOR('',#45168,1000.);
#10758=VECTOR('',#45169,1000.);
#10759=VECTOR('',#45210,1000.);
#10760=VECTOR('',#45211,1000.);
#10761=VECTOR('',#45262,1000.);
#10762=VECTOR('',#45263,1000.);
#10763=VECTOR('',#45274,1000.);
#10764=VECTOR('',#45277,1000.);
#10765=VECTOR('',#45328,1000.);
#10766=VECTOR('',#45347,1000.);
#10767=VECTOR('',#45364,1000.);
#10768=VECTOR('',#45367,1000.);
#10769=VECTOR('',#45380,1000.);
#10770=VECTOR('',#45383,1000.);
#10771=VECTOR('',#45386,1000.);
#10772=VECTOR('',#45389,1000.);
#10773=VECTOR('',#45392,1000.);
#10774=VECTOR('',#45401,1000.);
#10775=VECTOR('',#45402,1000.);
#10776=VECTOR('',#45409,1000.);
#10777=VECTOR('',#45430,1000.);
#10778=VECTOR('',#45457,1000.);
#10779=VECTOR('',#45458,1000.);
#10780=VECTOR('',#45459,1000.);
#10781=VECTOR('',#45462,1000.);
#10782=VECTOR('',#45463,1000.);
#10783=VECTOR('',#45468,1000.);
#10784=VECTOR('',#45471,1000.);
#10785=VECTOR('',#45472,1000.);
#10786=VECTOR('',#45477,1000.);
#10787=VECTOR('',#45482,1000.);
#10788=VECTOR('',#45485,1000.);
#10789=VECTOR('',#45488,1000.);
#10790=VECTOR('',#45493,1000.);
#10791=VECTOR('',#45494,1000.);
#10792=VECTOR('',#45497,1000.);
#10793=VECTOR('',#45500,1000.);
#10794=VECTOR('',#45503,1000.);
#10795=VECTOR('',#45506,1000.);
#10796=VECTOR('',#45511,1000.);
#10797=VECTOR('',#45512,1000.);
#10798=VECTOR('',#45515,1000.);
#10799=VECTOR('',#45518,1000.);
#10800=VECTOR('',#45523,1000.);
#10801=VECTOR('',#45528,1000.);
#10802=VECTOR('',#45531,1000.);
#10803=VECTOR('',#45538,1000.);
#10804=VECTOR('',#45541,1000.);
#10805=VECTOR('',#45560,1000.);
#10806=VECTOR('',#45563,1000.);
#10807=VECTOR('',#45582,1000.);
#10808=VECTOR('',#45601,1000.);
#10809=VECTOR('',#45622,1000.);
#10810=VECTOR('',#45623,1000.);
#10811=VECTOR('',#45638,1000.);
#10812=VECTOR('',#45661,1000.);
#10813=VECTOR('',#45688,1000.);
#10814=VECTOR('',#45691,1000.);
#10815=VECTOR('',#45694,1000.);
#10816=VECTOR('',#45697,1000.);
#10817=VECTOR('',#45706,1000.);
#10818=VECTOR('',#45707,1000.);
#10819=VECTOR('',#45710,1000.);
#10820=VECTOR('',#45713,1000.);
#10821=VECTOR('',#45720,1000.);
#10822=VECTOR('',#45743,1000.);
#10823=VECTOR('',#45784,1000.);
#10824=VECTOR('',#45789,1000.);
#10825=VECTOR('',#45794,1000.);
#10826=VECTOR('',#45825,1000.);
#10827=VECTOR('',#45828,1000.);
#10828=VECTOR('',#45859,1000.);
#10829=VECTOR('',#45860,1000.);
#10830=VECTOR('',#45863,1000.);
#10831=VECTOR('',#45866,1000.);
#10832=VECTOR('',#45871,1000.);
#10833=VECTOR('',#45880,1000.);
#10834=VECTOR('',#45885,1000.);
#10835=VECTOR('',#45890,1000.);
#10836=VECTOR('',#45893,1000.);
#10837=VECTOR('',#45894,1000.);
#10838=VECTOR('',#45899,1000.);
#10839=VECTOR('',#45904,1000.);
#10840=VECTOR('',#45909,1000.);
#10841=VECTOR('',#45912,1000.);
#10842=VECTOR('',#45913,1000.);
#10843=VECTOR('',#45962,1000.);
#10844=VECTOR('',#45977,1000.);
#10845=VECTOR('',#45980,1000.);
#10846=VECTOR('',#46003,1000.);
#10847=VECTOR('',#46006,1000.);
#10848=VECTOR('',#46017,1000.);
#10849=VECTOR('',#46022,1000.);
#10850=VECTOR('',#46025,1000.);
#10851=VECTOR('',#46028,1000.);
#10852=VECTOR('',#46031,1000.);
#10853=VECTOR('',#46034,1000.);
#10854=VECTOR('',#46037,1000.);
#10855=VECTOR('',#46038,1000.);
#10856=VECTOR('',#46039,1000.);
#10857=VECTOR('',#46044,1000.);
#10858=VECTOR('',#46053,1000.);
#10859=VECTOR('',#46058,1000.);
#10860=VECTOR('',#46059,1000.);
#10861=VECTOR('',#46064,1000.);
#10862=VECTOR('',#46067,1000.);
#10863=VECTOR('',#46068,1000.);
#10864=VECTOR('',#46071,1000.);
#10865=VECTOR('',#46074,1000.);
#10866=VECTOR('',#46095,1000.);
#10867=VECTOR('',#46096,1000.);
#10868=VECTOR('',#46137,1000.);
#10869=VECTOR('',#46154,1000.);
#10870=VECTOR('',#46165,1000.);
#10871=VECTOR('',#46166,1000.);
#10872=VECTOR('',#46167,1000.);
#10873=VECTOR('',#46168,1000.);
#10874=VECTOR('',#46169,1000.);
#10875=VECTOR('',#46170,1000.);
#10876=VECTOR('',#46175,1000.);
#10877=VECTOR('',#46184,1000.);
#10878=VECTOR('',#46189,1000.);
#10879=VECTOR('',#46194,1000.);
#10880=VECTOR('',#46195,1000.);
#10881=VECTOR('',#46196,1000.);
#10882=VECTOR('',#46203,1000.);
#10883=VECTOR('',#46206,1000.);
#10884=VECTOR('',#46217,1000.);
#10885=VECTOR('',#46236,1000.);
#10886=VECTOR('',#46269,1000.);
#10887=VECTOR('',#46270,1000.);
#10888=VECTOR('',#46281,1000.);
#10889=VECTOR('',#46282,1000.);
#10890=VECTOR('',#46297,1000.);
#10891=VECTOR('',#46298,1000.);
#10892=VECTOR('',#46299,1000.);
#10893=VECTOR('',#46306,1000.);
#10894=VECTOR('',#46307,1000.);
#10895=VECTOR('',#46316,1000.);
#10896=VECTOR('',#46317,1000.);
#10897=VECTOR('',#46318,1000.);
#10898=VECTOR('',#46327,1000.);
#10899=VECTOR('',#46328,1000.);
#10900=VECTOR('',#46337,1000.);
#10901=VECTOR('',#46360,1000.);
#10902=VECTOR('',#46425,1000.);
#10903=VECTOR('',#46430,1000.);
#10904=VECTOR('',#46431,1000.);
#10905=VECTOR('',#46432,1000.);
#10906=VECTOR('',#46435,1000.);
#10907=VECTOR('',#46444,1000.);
#10908=VECTOR('',#46447,1000.);
#10909=VECTOR('',#46450,1000.);
#10910=VECTOR('',#46459,1000.);
#10911=VECTOR('',#46462,1000.);
#10912=VECTOR('',#46465,1000.);
#10913=VECTOR('',#46466,1000.);
#10914=VECTOR('',#46471,1000.);
#10915=VECTOR('',#46476,1000.);
#10916=VECTOR('',#46479,1000.);
#10917=VECTOR('',#46480,1000.);
#10918=VECTOR('',#46485,1000.);
#10919=VECTOR('',#46488,1000.);
#10920=VECTOR('',#46489,1000.);
#10921=VECTOR('',#46490,1000.);
#10922=VECTOR('',#46513,1000.);
#10923=VECTOR('',#46514,1000.);
#10924=VECTOR('',#46519,1000.);
#10925=VECTOR('',#46524,1000.);
#10926=VECTOR('',#46527,1000.);
#10927=VECTOR('',#46528,1000.);
#10928=VECTOR('',#46529,1000.);
#10929=VECTOR('',#46530,1000.);
#10930=VECTOR('',#46533,1000.);
#10931=VECTOR('',#46538,1000.);
#10932=VECTOR('',#46543,1000.);
#10933=VECTOR('',#46552,1000.);
#10934=VECTOR('',#46557,1000.);
#10935=VECTOR('',#46558,1000.);
#10936=VECTOR('',#46559,1000.);
#10937=VECTOR('',#46564,1000.);
#10938=VECTOR('',#46569,1000.);
#10939=VECTOR('',#46582,1000.);
#10940=VECTOR('',#46585,1000.);
#10941=VECTOR('',#46608,1000.);
#10942=VECTOR('',#46609,1000.);
#10943=VECTOR('',#46644,1000.);
#10944=VECTOR('',#46645,1000.);
#10945=VECTOR('',#46702,1000.);
#10946=VECTOR('',#46703,1000.);
#10947=VECTOR('',#46740,1000.);
#10948=VECTOR('',#46741,1000.);
#10949=VECTOR('',#46776,1000.);
#10950=VECTOR('',#46777,1000.);
#10951=VECTOR('',#46780,1000.);
#10952=VECTOR('',#46781,1000.);
#10953=VECTOR('',#46784,1000.);
#10954=VECTOR('',#46787,1000.);
#10955=VECTOR('',#46826,1000.);
#10956=VECTOR('',#46827,1000.);
#10957=VECTOR('',#46876,1000.);
#10958=VECTOR('',#46879,1000.);
#10959=VECTOR('',#46894,1000.);
#10960=VECTOR('',#46897,1000.);
#10961=VECTOR('',#46932,1000.);
#10962=VECTOR('',#46939,1000.);
#10963=VECTOR('',#46950,1000.);
#10964=VECTOR('',#46961,1000.);
#10965=VECTOR('',#46976,1000.);
#10966=VECTOR('',#46989,1000.);
#10967=VECTOR('',#47000,1000.);
#10968=VECTOR('',#47011,1000.);
#10969=VECTOR('',#47020,1000.);
#10970=VECTOR('',#47023,1000.);
#10971=VECTOR('',#47042,1000.);
#10972=VECTOR('',#47075,1000.);
#10973=VECTOR('',#47080,1000.);
#10974=VECTOR('',#47085,1000.);
#10975=VECTOR('',#47088,1000.);
#10976=VECTOR('',#47093,1000.);
#10977=VECTOR('',#47106,1000.);
#10978=VECTOR('',#47111,1000.);
#10979=VECTOR('',#47122,1000.);
#10980=VECTOR('',#47127,1000.);
#10981=VECTOR('',#47130,1000.);
#10982=VECTOR('',#47133,1000.);
#10983=VECTOR('',#47140,1000.);
#10984=VECTOR('',#47181,1000.);
#10985=VECTOR('',#47182,1000.);
#10986=VECTOR('',#47183,1000.);
#10987=VECTOR('',#47186,1000.);
#10988=VECTOR('',#47187,1000.);
#10989=VECTOR('',#47190,1000.);
#10990=VECTOR('',#47195,1000.);
#10991=VECTOR('',#47196,1000.);
#10992=VECTOR('',#47199,1000.);
#10993=VECTOR('',#47204,1000.);
#10994=VECTOR('',#47209,1000.);
#10995=VECTOR('',#47212,1000.);
#10996=VECTOR('',#47217,1000.);
#10997=VECTOR('',#47218,1000.);
#10998=VECTOR('',#47221,1000.);
#10999=VECTOR('',#47224,1000.);
#11000=VECTOR('',#47227,1000.);
#11001=VECTOR('',#47230,1000.);
#11002=VECTOR('',#47235,1000.);
#11003=VECTOR('',#47236,1000.);
#11004=VECTOR('',#47239,1000.);
#11005=VECTOR('',#47242,1000.);
#11006=VECTOR('',#47245,1000.);
#11007=VECTOR('',#47250,1000.);
#11008=VECTOR('',#47257,1000.);
#11009=VECTOR('',#47260,1000.);
#11010=VECTOR('',#47265,1000.);
#11011=VECTOR('',#47284,1000.);
#11012=VECTOR('',#47289,1000.);
#11013=VECTOR('',#47306,1000.);
#11014=VECTOR('',#47325,1000.);
#11015=VECTOR('',#47342,1000.);
#11016=VECTOR('',#47343,1000.);
#11017=VECTOR('',#47354,1000.);
#11018=VECTOR('',#47379,1000.);
#11019=VECTOR('',#47386,1000.);
#11020=VECTOR('',#47413,1000.);
#11021=VECTOR('',#47416,1000.);
#11022=VECTOR('',#47419,1000.);
#11023=VECTOR('',#47426,1000.);
#11024=VECTOR('',#47433,1000.);
#11025=VECTOR('',#47436,1000.);
#11026=VECTOR('',#47439,1000.);
#11027=VECTOR('',#47444,1000.);
#11028=VECTOR('',#47467,1000.);
#11029=VECTOR('',#47508,1000.);
#11030=VECTOR('',#47515,1000.);
#11031=VECTOR('',#47520,1000.);
#11032=VECTOR('',#47533,1000.);
#11033=VECTOR('',#47538,1000.);
#11034=VECTOR('',#47543,1000.);
#11035=VECTOR('',#47548,1000.);
#11036=VECTOR('',#47563,1000.);
#11037=VECTOR('',#47572,1000.);
#11038=VECTOR('',#47575,1000.);
#11039=VECTOR('',#47578,1000.);
#11040=VECTOR('',#47587,1000.);
#11041=VECTOR('',#47594,1000.);
#11042=VECTOR('',#47623,1000.);
#11043=VECTOR('',#47648,1000.);
#11044=VECTOR('',#47651,1000.);
#11045=VECTOR('',#47654,1000.);
#11046=VECTOR('',#47657,1000.);
#11047=VECTOR('',#47666,1000.);
#11048=VECTOR('',#47671,1000.);
#11049=VECTOR('',#47676,1000.);
#11050=VECTOR('',#47681,1000.);
#11051=VECTOR('',#47682,1000.);
#11052=VECTOR('',#47685,1000.);
#11053=VECTOR('',#47690,1000.);
#11054=VECTOR('',#47695,1000.);
#11055=VECTOR('',#47700,1000.);
#11056=VECTOR('',#47701,1000.);
#11057=VECTOR('',#47754,1000.);
#11058=VECTOR('',#47771,1000.);
#11059=VECTOR('',#47776,1000.);
#12518=CIRCLE('',#36604,0.3);
#12519=CIRCLE('',#36605,0.3);
#12520=CIRCLE('',#36607,13.516744254);
#12521=CIRCLE('',#36608,13.516744254);
#12522=CIRCLE('',#36611,0.3);
#12523=CIRCLE('',#36613,0.3);
#12524=CIRCLE('',#36615,0.3);
#12525=CIRCLE('',#36616,0.300000000000007);
#12526=CIRCLE('',#36619,0.3);
#12527=CIRCLE('',#36620,0.3);
#12528=CIRCLE('',#36622,13.516744254);
#12529=CIRCLE('',#36623,13.516744254);
#12530=CIRCLE('',#36625,0.3);
#12531=CIRCLE('',#36626,0.3);
#12532=CIRCLE('',#36628,0.861212043428353);
#12533=CIRCLE('',#36630,0.3);
#12534=CIRCLE('',#36632,0.299999999999999);
#12535=CIRCLE('',#36634,13.816744254);
#12536=CIRCLE('',#36635,0.3);
#12537=CIRCLE('',#36637,0.3);
#12538=CIRCLE('',#36639,0.3);
#12539=CIRCLE('',#36641,0.6);
#12540=CIRCLE('',#36642,0.3);
#12541=CIRCLE('',#36643,0.3);
#12542=CIRCLE('',#36645,14.9875296363);
#12543=CIRCLE('',#36646,14.6875296363);
#12544=CIRCLE('',#36647,0.300000000000001);
#12545=CIRCLE('',#36649,0.6);
#12546=CIRCLE('',#36650,0.299999999999999);
#12547=CIRCLE('',#36652,14.9875296363);
#12548=CIRCLE('',#36653,14.6875296363);
#12549=CIRCLE('',#36654,0.300000000000001);
#12550=CIRCLE('',#36656,0.6);
#12551=CIRCLE('',#36657,0.3);
#12552=CIRCLE('',#36659,0.3);
#12553=CIRCLE('',#36661,0.299999999999999);
#12554=CIRCLE('',#36663,13.816744254);
#12555=CIRCLE('',#36664,0.299999999999999);
#12556=CIRCLE('',#36666,0.3);
#12557=CIRCLE('',#36669,2.7);
#12558=CIRCLE('',#36670,15.3875296363);
#12559=CIRCLE('',#36673,0.3);
#12560=CIRCLE('',#36674,0.3);
#12561=CIRCLE('',#36676,13.6462109523);
#12562=CIRCLE('',#36677,13.6462109523);
#12563=CIRCLE('',#36679,0.3);
#12564=CIRCLE('',#36680,0.3);
#12565=CIRCLE('',#36683,0.3);
#12566=CIRCLE('',#36685,0.299999999999999);
#12567=CIRCLE('',#36686,0.3);
#12568=CIRCLE('',#36688,0.3);
#12569=CIRCLE('',#36689,0.3);
#12570=CIRCLE('',#36691,0.3);
#12571=CIRCLE('',#36693,13.9462109523);
#12572=CIRCLE('',#36694,0.3);
#12573=CIRCLE('',#36696,0.3);
#12574=CIRCLE('',#36698,0.3);
#12575=CIRCLE('',#36700,0.6);
#12576=CIRCLE('',#36701,0.3);
#12577=CIRCLE('',#36703,14.9875296363);
#12578=CIRCLE('',#36704,14.6875296363);
#12579=CIRCLE('',#36706,0.3);
#12580=CIRCLE('',#36708,16.1875296363);
#12581=CIRCLE('',#36709,15.8875296363);
#12582=CIRCLE('',#36712,8.14541841273);
#12583=CIRCLE('',#36713,7.84541841273);
#12584=CIRCLE('',#36714,0.299999999999994);
#12585=CIRCLE('',#36716,0.300000000000002);
#12586=CIRCLE('',#36718,14.6875296363);
#12587=CIRCLE('',#36719,14.3875296363);
#12588=CIRCLE('',#36720,0.299999999999999);
#12589=CIRCLE('',#36722,0.3);
#12590=CIRCLE('',#36725,0.3);
#12591=CIRCLE('',#36727,7.84541841273);
#12592=CIRCLE('',#36729,0.3);
#12593=CIRCLE('',#36732,0.3);
#12594=CIRCLE('',#36734,14.6875296363);
#12595=CIRCLE('',#36736,0.3);
#12596=CIRCLE('',#36738,0.3);
#12597=CIRCLE('',#36739,0.3);
#12598=CIRCLE('',#36741,0.3);
#12599=CIRCLE('',#36743,0.3);
#12600=CIRCLE('',#36744,7.54541841273);
#12601=CIRCLE('',#36745,0.3);
#12602=CIRCLE('',#36747,0.3);
#12603=CIRCLE('',#36749,0.300000000000002);
#12604=CIRCLE('',#36750,0.300000000000002);
#12605=CIRCLE('',#36752,0.3);
#12606=CIRCLE('',#36754,0.3);
#12607=CIRCLE('',#36755,14.9875296363);
#12608=CIRCLE('',#36756,0.300000000000001);
#12609=CIRCLE('',#36758,0.6);
#12610=CIRCLE('',#36760,0.3);
#12611=CIRCLE('',#36761,0.3);
#12612=CIRCLE('',#36762,0.299999999999999);
#12613=CIRCLE('',#36764,0.6);
#12614=CIRCLE('',#36766,0.6);
#12615=CIRCLE('',#36768,0.6);
#12616=CIRCLE('',#36770,12.5256279976);
#12617=CIRCLE('',#36771,0.3);
#12618=CIRCLE('',#36772,12.2256279976);
#12619=CIRCLE('',#36776,14.9875296363);
#12620=CIRCLE('',#36777,0.3);
#12621=CIRCLE('',#36778,14.6875296363);
#12622=CIRCLE('',#36781,16.1875296363);
#12623=CIRCLE('',#36782,16.1875296363);
#12624=CIRCLE('',#36783,16.1875296363);
#12625=CIRCLE('',#36785,16.1875296363);
#12626=CIRCLE('',#36789,0.3);
#12627=CIRCLE('',#36794,0.3);
#12628=CIRCLE('',#36798,0.3);
#12629=CIRCLE('',#36799,0.3);
#12630=CIRCLE('',#36801,0.3);
#12631=CIRCLE('',#36802,0.3);
#12632=CIRCLE('',#36804,0.300000000000001);
#12633=CIRCLE('',#36805,15.6875296363);
#12634=CIRCLE('',#36809,0.599999999902816);
#12635=CIRCLE('',#36811,0.3);
#12636=CIRCLE('',#36812,0.3);
#12637=CIRCLE('',#36814,7.84541841273);
#12638=CIRCLE('',#36815,7.84541841273);
#12639=CIRCLE('',#36817,0.3);
#12640=CIRCLE('',#36818,0.3);
#12641=CIRCLE('',#36821,0.3);
#12642=CIRCLE('',#36823,0.3);
#12643=CIRCLE('',#36824,0.3);
#12644=CIRCLE('',#36826,14.6875296363);
#12645=CIRCLE('',#36827,14.6875296363);
#12646=CIRCLE('',#36829,0.3);
#12647=CIRCLE('',#36830,0.3);
#12648=CIRCLE('',#36832,4.89295371933);
#12649=CIRCLE('',#36833,0.3);
#12650=CIRCLE('',#36834,5.19295371933);
#12651=CIRCLE('',#36835,0.3);
#12652=CIRCLE('',#36837,0.6);
#12653=CIRCLE('',#36838,0.3);
#12654=CIRCLE('',#36839,0.3);
#12655=CIRCLE('',#36841,0.3);
#12656=CIRCLE('',#36843,0.6);
#12657=CIRCLE('',#36844,0.3);
#12658=CIRCLE('',#36845,0.299999999999999);
#12659=CIRCLE('',#36847,6.64541841273);
#12660=CIRCLE('',#36848,6.34541841273);
#12661=CIRCLE('',#36849,0.3);
#12662=CIRCLE('',#36851,0.6);
#12663=CIRCLE('',#36852,0.3);
#12664=CIRCLE('',#36853,0.3);
#12665=CIRCLE('',#36855,0.6);
#12666=CIRCLE('',#36856,0.3);
#12667=CIRCLE('',#36857,0.3);
#12668=CIRCLE('',#36860,6.34541841273);
#12669=CIRCLE('',#36861,0.3);
#12670=CIRCLE('',#36862,6.64541841273);
#12671=CIRCLE('',#36863,0.3);
#12672=CIRCLE('',#36867,0.6);
#12673=CIRCLE('',#36868,0.3);
#12674=CIRCLE('',#36869,0.3);
#12675=CIRCLE('',#36876,5.19295371933);
#12676=CIRCLE('',#36877,0.3);
#12677=CIRCLE('',#36878,4.89295371933);
#12678=CIRCLE('',#36880,0.3);
#12679=CIRCLE('',#36881,0.6);
#12680=CIRCLE('',#36882,0.300000000000002);
#12681=CIRCLE('',#36884,0.3);
#12682=CIRCLE('',#36885,0.300000000000002);
#12683=CIRCLE('',#36886,0.6);
#12684=CIRCLE('',#36895,4.89295371933);
#12685=CIRCLE('',#36896,0.3);
#12686=CIRCLE('',#36897,5.19295371933);
#12687=CIRCLE('',#36898,0.3);
#12688=CIRCLE('',#36899,4.89295371933);
#12689=CIRCLE('',#36901,0.6);
#12690=CIRCLE('',#36902,0.3);
#12691=CIRCLE('',#36903,0.3);
#12692=CIRCLE('',#36905,0.3);
#12693=CIRCLE('',#36907,0.6);
#12694=CIRCLE('',#36908,0.3);
#12695=CIRCLE('',#36909,0.3);
#12696=CIRCLE('',#36911,6.64541841273);
#12697=CIRCLE('',#36912,6.34541841273);
#12698=CIRCLE('',#36913,0.3);
#12699=CIRCLE('',#36915,0.6);
#12700=CIRCLE('',#36916,0.300000000000002);
#12701=CIRCLE('',#36917,0.3);
#12702=CIRCLE('',#36919,0.6);
#12703=CIRCLE('',#36920,0.3);
#12704=CIRCLE('',#36921,0.300000000000002);
#12705=CIRCLE('',#36924,0.299999999999996);
#12706=CIRCLE('',#36927,6.04541841273);
#12707=CIRCLE('',#36928,6.34541841273);
#12708=CIRCLE('',#36929,0.300000000000002);
#12709=CIRCLE('',#36931,0.3);
#12710=CIRCLE('',#36932,0.3);
#12711=CIRCLE('',#36934,5.19295371933);
#12712=CIRCLE('',#36935,5.49295371933);
#12713=CIRCLE('',#36937,0.3);
#12714=CIRCLE('',#36938,0.300000000000002);
#12715=CIRCLE('',#36940,0.3);
#12716=CIRCLE('',#36941,0.300000000000002);
#12717=CIRCLE('',#36943,0.3);
#12718=CIRCLE('',#36944,0.3);
#12719=CIRCLE('',#36947,5.49295371933);
#12720=CIRCLE('',#36948,5.19295371933);
#12721=CIRCLE('',#36949,0.299999999999998);
#12722=CIRCLE('',#36951,0.3);
#12723=CIRCLE('',#36952,0.3);
#12724=CIRCLE('',#36953,0.6);
#12725=CIRCLE('',#36955,7.84541841273);
#12726=CIRCLE('',#36956,0.3);
#12727=CIRCLE('',#36957,7.54541841273);
#12728=CIRCLE('',#36959,0.3);
#12729=CIRCLE('',#36960,0.6);
#12730=CIRCLE('',#36961,0.3);
#12731=CIRCLE('',#36963,0.3);
#12732=CIRCLE('',#36964,0.3);
#12733=CIRCLE('',#36965,0.6);
#12734=CIRCLE('',#36967,0.3);
#12735=CIRCLE('',#36968,0.3);
#12736=CIRCLE('',#36970,12.5256279976);
#12737=CIRCLE('',#36972,0.3);
#12738=CIRCLE('',#36974,12.8256279976);
#12739=CIRCLE('',#36976,0.3);
#12740=CIRCLE('',#36977,0.3);
#12741=CIRCLE('',#36979,5.49295371933);
#12742=CIRCLE('',#36980,5.19295371933);
#12743=CIRCLE('',#36982,15.8875296363);
#12744=CIRCLE('',#36983,0.385778366608001);
#12745=CIRCLE('',#36985,15.8875296363);
#12746=CIRCLE('',#36986,0.299999999999999);
#12747=CIRCLE('',#36987,0.3);
#12748=CIRCLE('',#36989,15.3875296363);
#12749=CIRCLE('',#36990,0.3);
#12750=CIRCLE('',#36991,15.6875296363);
#12751=CIRCLE('',#36992,0.3);
#12752=CIRCLE('',#36994,15.8875296363);
#12753=CIRCLE('',#36995,0.300000000000006);
#12754=CIRCLE('',#36997,0.685778366608001);
#12755=CIRCLE('',#36998,0.3);
#12756=CIRCLE('',#36999,0.985778366608001);
#12757=CIRCLE('',#37001,0.300000000000012);
#12758=CIRCLE('',#37002,0.3);
#12759=CIRCLE('',#37004,0.3);
#12760=CIRCLE('',#37006,3.);
#12761=CIRCLE('',#37008,2.7);
#12762=CIRCLE('',#37009,3.);
#12763=CIRCLE('',#37014,0.299999999999996);
#12764=CIRCLE('',#37017,0.3);
#12765=CIRCLE('',#37020,0.3);
#12766=CIRCLE('',#37022,0.3);
#12767=CIRCLE('',#37023,0.3);
#12768=CIRCLE('',#37024,0.3);
#12769=CIRCLE('',#37026,0.3);
#12770=CIRCLE('',#37028,0.300000000000014);
#12771=CIRCLE('',#37032,0.3);
#12772=CIRCLE('',#37035,0.299999999999999);
#12773=CIRCLE('',#37036,0.3);
#12774=CIRCLE('',#37038,0.3);
#12775=CIRCLE('',#37040,0.3);
#12776=CIRCLE('',#37041,8.14541841273);
#12777=CIRCLE('',#37042,7.86257590088);
#12778=CIRCLE('',#37044,0.282842511848);
#12779=CIRCLE('',#37045,0.3);
#12780=CIRCLE('',#37047,0.3);
#12781=CIRCLE('',#37049,0.3);
#12782=CIRCLE('',#37051,0.282842712475);
#12783=CIRCLE('',#37052,0.3);
#12784=CIRCLE('',#37054,14.3875296363);
#12785=CIRCLE('',#37055,14.670372344);
#12786=CIRCLE('',#37058,0.300000000000002);
#12787=CIRCLE('',#37062,0.3);
#12788=CIRCLE('',#37065,0.3);
#12789=CIRCLE('',#37067,6.34541841273);
#12790=CIRCLE('',#37081,0.3);
#12791=CIRCLE('',#37083,6.34541841273);
#12792=CIRCLE('',#37085,0.3);
#12793=CIRCLE('',#37087,0.3);
#12794=CIRCLE('',#37090,0.3);
#12795=CIRCLE('',#37092,6.04541841273);
#12796=CIRCLE('',#37094,0.300000000000002);
#12797=CIRCLE('',#37096,0.300000000000002);
#12798=CIRCLE('',#37099,6.04541841273);
#12799=CIRCLE('',#37102,0.3);
#12800=CIRCLE('',#37103,0.3);
#12801=CIRCLE('',#37104,0.3);
#12802=CIRCLE('',#37109,0.685778366608001);
#12803=CIRCLE('',#37111,0.3);
#12804=CIRCLE('',#37120,0.6);
#12805=CIRCLE('',#37121,0.300000000000002);
#12806=CIRCLE('',#37123,0.3);
#12807=CIRCLE('',#37124,0.3);
#12808=CIRCLE('',#37125,0.3);
#12809=CIRCLE('',#37128,7.84541841273);
#12810=CIRCLE('',#37130,8.14541841273);
#12811=CIRCLE('',#37132,0.3);
#12812=CIRCLE('',#37133,0.3);
#12813=CIRCLE('',#37135,0.3);
#12814=CIRCLE('',#37136,0.6);
#12815=CIRCLE('',#37138,0.3);
#12816=CIRCLE('',#37139,13.3462109523);
#12817=CIRCLE('',#37141,0.3);
#12818=CIRCLE('',#37142,0.6);
#12819=CIRCLE('',#37144,0.3);
#12820=CIRCLE('',#37146,0.3);
#12821=CIRCLE('',#37147,0.3);
#12822=CIRCLE('',#37148,0.300000000000001);
#12823=CIRCLE('',#37150,14.6875296363);
#12824=CIRCLE('',#37151,14.3875296363);
#12825=CIRCLE('',#37153,0.3);
#12826=CIRCLE('',#37155,14.6875296363);
#12827=CIRCLE('',#37156,14.3875296363);
#12828=CIRCLE('',#37161,0.3);
#12829=CIRCLE('',#37163,0.3);
#12830=CIRCLE('',#37169,0.299999999999999);
#12831=CIRCLE('',#37171,0.3);
#12832=CIRCLE('',#37172,0.6);
#12833=CIRCLE('',#37174,0.3);
#12834=CIRCLE('',#37175,7.54541841273);
#12835=CIRCLE('',#37177,0.3);
#12836=CIRCLE('',#37178,0.6);
#12837=CIRCLE('',#37180,0.3);
#12838=CIRCLE('',#37181,0.3);
#12839=CIRCLE('',#37183,0.6);
#12840=CIRCLE('',#37184,0.3);
#12841=CIRCLE('',#37186,0.300000000000002);
#12842=CIRCLE('',#37187,0.6);
#12843=CIRCLE('',#37189,14.9875296363);
#12844=CIRCLE('',#37191,0.299999999999999);
#12845=CIRCLE('',#37192,0.6);
#12846=CIRCLE('',#37194,0.299999999999998);
#12847=CIRCLE('',#37195,13.216744254);
#12848=CIRCLE('',#37200,0.300000000000002);
#12849=CIRCLE('',#37206,15.8875296363);
#12850=CIRCLE('',#37208,0.999999999999999);
#12851=CIRCLE('',#37210,0.825178907983792);
#12852=CIRCLE('',#37212,14.6875296363);
#12853=CIRCLE('',#37213,0.299999999999999);
#12854=CIRCLE('',#37214,14.9875296363);
#12855=CIRCLE('',#37216,0.3);
#12856=CIRCLE('',#37217,0.300000000000002);
#12857=CIRCLE('',#37218,0.6);
#12858=CIRCLE('',#37220,0.300000000000002);
#12859=CIRCLE('',#37222,0.3);
#12860=CIRCLE('',#37223,0.3);
#12861=CIRCLE('',#37224,0.6);
#12862=CIRCLE('',#37226,7.84541841273);
#12863=CIRCLE('',#37227,0.3);
#12864=CIRCLE('',#37228,7.54541841273);
#12865=CIRCLE('',#37230,0.3);
#12866=CIRCLE('',#37231,0.299999999999999);
#12867=CIRCLE('',#37232,0.6);
#12868=CIRCLE('',#37237,14.6875296363);
#12869=CIRCLE('',#37239,0.999999999999999);
#12870=CIRCLE('',#37241,14.6875296363);
#12871=CIRCLE('',#37243,0.3);
#12872=CIRCLE('',#37245,14.6875296363);
#12873=CIRCLE('',#37247,0.3);
#12874=CIRCLE('',#37250,0.3);
#12875=CIRCLE('',#37252,7.84541841273);
#12876=CIRCLE('',#37254,0.3);
#12877=CIRCLE('',#37257,0.3);
#12878=CIRCLE('',#37259,0.3);
#12879=CIRCLE('',#37260,0.3);
#12880=CIRCLE('',#37262,14.3875296363);
#12881=CIRCLE('',#37263,0.3);
#12882=CIRCLE('',#37265,0.699999999999999);
#12883=CIRCLE('',#37266,0.3);
#12884=CIRCLE('',#37268,0.300000000000001);
#12885=CIRCLE('',#37269,0.3);
#12886=CIRCLE('',#37271,14.3875296363);
#12887=CIRCLE('',#37273,0.3);
#12888=CIRCLE('',#37274,0.3);
#12889=CIRCLE('',#37276,14.3875296363);
#12890=CIRCLE('',#37278,0.300000000000002);
#12891=CIRCLE('',#37281,0.3);
#12892=CIRCLE('',#37283,8.14541841273);
#12893=CIRCLE('',#37285,0.3);
#12894=CIRCLE('',#37288,0.3);
#12895=CIRCLE('',#37290,0.6);
#12896=CIRCLE('',#37291,0.299999999999999);
#12897=CIRCLE('',#37293,13.216744254);
#12898=CIRCLE('',#37294,0.299999999999999);
#12899=CIRCLE('',#37296,0.6);
#12900=CIRCLE('',#37299,0.3);
#12901=CIRCLE('',#37300,0.3);
#12902=CIRCLE('',#37303,13.516744254);
#12903=CIRCLE('',#37304,13.516744254);
#12904=CIRCLE('',#37306,0.3);
#12905=CIRCLE('',#37308,0.3);
#12906=CIRCLE('',#37310,0.3);
#12907=CIRCLE('',#37313,0.3);
#12908=CIRCLE('',#37314,0.3);
#12909=CIRCLE('',#37316,13.516744254);
#12910=CIRCLE('',#37317,13.516744254);
#12911=CIRCLE('',#37319,0.3);
#12912=CIRCLE('',#37320,0.3);
#12913=CIRCLE('',#37322,0.861212043428353);
#12914=CIRCLE('',#37324,0.3);
#12915=CIRCLE('',#37325,0.300000000000002);
#12916=CIRCLE('',#37327,0.299999999999999);
#12917=CIRCLE('',#37329,0.3);
#12918=CIRCLE('',#37330,13.816744254);
#12919=CIRCLE('',#37332,0.3);
#12920=CIRCLE('',#37334,0.3);
#12921=CIRCLE('',#37336,0.3);
#12922=CIRCLE('',#37337,0.3);
#12923=CIRCLE('',#37338,0.6);
#12924=CIRCLE('',#37340,0.300000000000001);
#12925=CIRCLE('',#37341,14.6875296363);
#12926=CIRCLE('',#37342,14.9875296363);
#12927=CIRCLE('',#37344,0.299999999999999);
#12928=CIRCLE('',#37345,0.6);
#12929=CIRCLE('',#37347,0.300000000000001);
#12930=CIRCLE('',#37348,14.6875296363);
#12931=CIRCLE('',#37349,14.9875296363);
#12932=CIRCLE('',#37351,0.3);
#12933=CIRCLE('',#37352,0.6);
#12934=CIRCLE('',#37354,0.3);
#12935=CIRCLE('',#37356,0.299999999999999);
#12936=CIRCLE('',#37358,0.299999999999999);
#12937=CIRCLE('',#37359,13.816744254);
#12938=CIRCLE('',#37361,0.3);
#12939=CIRCLE('',#37363,0.300000000000007);
#12940=CIRCLE('',#37365,15.3875296363);
#12941=CIRCLE('',#37366,2.7);
#12942=CIRCLE('',#37369,0.3);
#12943=CIRCLE('',#37370,0.3);
#12944=CIRCLE('',#37372,13.6462109523);
#12945=CIRCLE('',#37373,13.6462109523);
#12946=CIRCLE('',#37375,0.3);
#12947=CIRCLE('',#37376,0.3);
#12948=CIRCLE('',#37379,0.300000000000001);
#12949=CIRCLE('',#37380,0.3);
#12950=CIRCLE('',#37382,0.3);
#12951=CIRCLE('',#37383,0.29999999999957);
#12952=CIRCLE('',#37385,0.3);
#12953=CIRCLE('',#37386,0.3);
#12954=CIRCLE('',#37388,0.3);
#12955=CIRCLE('',#37390,0.3);
#12956=CIRCLE('',#37391,13.9462109523);
#12957=CIRCLE('',#37393,0.3);
#12958=CIRCLE('',#37395,0.3);
#12959=CIRCLE('',#37397,0.3);
#12960=CIRCLE('',#37398,0.6);
#12961=CIRCLE('',#37399,1.);
#12962=CIRCLE('',#37401,14.6875296363);
#12963=CIRCLE('',#37402,14.9875296363);
#12964=CIRCLE('',#37404,0.3);
#12965=CIRCLE('',#37405,3.);
#12966=CIRCLE('',#37407,15.8875296363);
#12967=CIRCLE('',#37408,16.1875296363);
#12968=CIRCLE('',#37411,0.299999999999998);
#12969=CIRCLE('',#37413,7.84541841273);
#12970=CIRCLE('',#37414,0.299999999999989);
#12971=CIRCLE('',#37415,8.14541841273);
#12972=CIRCLE('',#37418,14.3875296363);
#12973=CIRCLE('',#37419,0.300000000000001);
#12974=CIRCLE('',#37420,14.6875296363);
#12975=CIRCLE('',#37422,0.3);
#12976=CIRCLE('',#37425,0.3);
#12977=CIRCLE('',#37427,7.84541841273);
#12978=CIRCLE('',#37429,0.3);
#12979=CIRCLE('',#37432,0.3);
#12980=CIRCLE('',#37434,14.6875296363);
#12981=CIRCLE('',#37436,0.3);
#12982=CIRCLE('',#37438,0.3);
#12983=CIRCLE('',#37439,0.3);
#12984=CIRCLE('',#37441,0.3);
#12985=CIRCLE('',#37443,0.3);
#12986=CIRCLE('',#37444,7.54541841273);
#12987=CIRCLE('',#37445,0.3);
#12988=CIRCLE('',#37447,0.3);
#12989=CIRCLE('',#37449,0.300000000000002);
#12990=CIRCLE('',#37450,0.300000000000002);
#12991=CIRCLE('',#37452,0.3);
#12992=CIRCLE('',#37454,0.300000000000001);
#12993=CIRCLE('',#37455,14.9875296363);
#12994=CIRCLE('',#37456,0.3);
#12995=CIRCLE('',#37458,0.6);
#12996=CIRCLE('',#37460,0.299999999999999);
#12997=CIRCLE('',#37461,0.3);
#12998=CIRCLE('',#37462,0.3);
#12999=CIRCLE('',#37464,0.6);
#13000=CIRCLE('',#37466,0.6);
#13001=CIRCLE('',#37468,0.6);
#13002=CIRCLE('',#37469,1.);
#13003=CIRCLE('',#37471,12.2256279976);
#13004=CIRCLE('',#37472,0.3);
#13005=CIRCLE('',#37473,12.5256279976);
#13006=CIRCLE('',#37477,14.6875296363);
#13007=CIRCLE('',#37478,0.3);
#13008=CIRCLE('',#37479,14.9875296363);
#13009=CIRCLE('',#37481,0.3);
#13010=CIRCLE('',#37482,0.3);
#13011=CIRCLE('',#37485,3.00001824423103);
#13012=CIRCLE('',#37487,16.1875296363);
#13013=CIRCLE('',#37489,16.1875296363);
#13014=CIRCLE('',#37490,16.1875296363);
#13015=CIRCLE('',#37491,16.1875296363);
#13016=CIRCLE('',#37493,0.3);
#13017=CIRCLE('',#37494,0.3);
#13018=CIRCLE('',#37498,0.3);
#13019=CIRCLE('',#37503,0.3);
#13020=CIRCLE('',#37506,0.3);
#13021=CIRCLE('',#37507,0.3);
#13022=CIRCLE('',#37509,0.3);
#13023=CIRCLE('',#37510,0.3);
#13024=CIRCLE('',#37512,15.6875296363);
#13025=CIRCLE('',#37513,0.300000000000001);
#13026=CIRCLE('',#37515,15.6875296363);
#13027=CIRCLE('',#37516,15.6875296363);
#13028=CIRCLE('',#37517,15.6875296363);
#13029=CIRCLE('',#37519,0.3);
#13030=CIRCLE('',#37521,0.599999999902816);
#13031=CIRCLE('',#37523,0.3);
#13032=CIRCLE('',#37524,0.3);
#13033=CIRCLE('',#37526,7.84541841273);
#13034=CIRCLE('',#37527,7.84541841273);
#13035=CIRCLE('',#37529,0.3);
#13036=CIRCLE('',#37530,0.3);
#13037=CIRCLE('',#37533,0.3);
#13038=CIRCLE('',#37535,0.3);
#13039=CIRCLE('',#37536,0.3);
#13040=CIRCLE('',#37538,14.6875296363);
#13041=CIRCLE('',#37539,14.6875296363);
#13042=CIRCLE('',#37541,0.3);
#13043=CIRCLE('',#37542,0.3);
#13044=CIRCLE('',#37544,0.3);
#13045=CIRCLE('',#37545,5.19295371933);
#13046=CIRCLE('',#37546,0.3);
#13047=CIRCLE('',#37547,4.89295371933);
#13048=CIRCLE('',#37549,0.3);
#13049=CIRCLE('',#37550,0.3);
#13050=CIRCLE('',#37551,0.6);
#13051=CIRCLE('',#37553,0.3);
#13052=CIRCLE('',#37555,0.299999999999999);
#13053=CIRCLE('',#37556,0.3);
#13054=CIRCLE('',#37557,0.6);
#13055=CIRCLE('',#37559,0.3);
#13056=CIRCLE('',#37560,6.34541841273);
#13057=CIRCLE('',#37561,6.64541841273);
#13058=CIRCLE('',#37563,0.3);
#13059=CIRCLE('',#37564,0.3);
#13060=CIRCLE('',#37565,0.6);
#13061=CIRCLE('',#37567,0.3);
#13062=CIRCLE('',#37568,0.3);
#13063=CIRCLE('',#37569,0.6);
#13064=CIRCLE('',#37572,0.3);
#13065=CIRCLE('',#37573,6.64541841273);
#13066=CIRCLE('',#37574,0.3);
#13067=CIRCLE('',#37575,6.34541841273);
#13068=CIRCLE('',#37579,0.3);
#13069=CIRCLE('',#37580,0.3);
#13070=CIRCLE('',#37581,0.6);
#13071=CIRCLE('',#37587,4.89295371933);
#13072=CIRCLE('',#37588,0.3);
#13073=CIRCLE('',#37589,5.19295371933);
#13074=CIRCLE('',#37591,0.300000000000002);
#13075=CIRCLE('',#37592,0.6);
#13076=CIRCLE('',#37593,0.3);
#13077=CIRCLE('',#37595,0.6);
#13078=CIRCLE('',#37596,0.300000000000002);
#13079=CIRCLE('',#37597,0.3);
#13080=CIRCLE('',#37606,4.89295371933);
#13081=CIRCLE('',#37607,0.3);
#13082=CIRCLE('',#37608,5.19295371933);
#13083=CIRCLE('',#37609,0.3);
#13084=CIRCLE('',#37610,4.89295371933);
#13085=CIRCLE('',#37612,0.3);
#13086=CIRCLE('',#37613,0.3);
#13087=CIRCLE('',#37614,0.6);
#13088=CIRCLE('',#37616,0.3);
#13089=CIRCLE('',#37618,0.3);
#13090=CIRCLE('',#37619,0.3);
#13091=CIRCLE('',#37620,0.6);
#13092=CIRCLE('',#37622,0.3);
#13093=CIRCLE('',#37623,6.34541841273);
#13094=CIRCLE('',#37624,6.64541841273);
#13095=CIRCLE('',#37626,0.3);
#13096=CIRCLE('',#37627,0.300000000000002);
#13097=CIRCLE('',#37628,0.6);
#13098=CIRCLE('',#37630,0.300000000000002);
#13099=CIRCLE('',#37631,0.3);
#13100=CIRCLE('',#37632,0.6);
#13101=CIRCLE('',#37636,0.300000000000002);
#13102=CIRCLE('',#37638,6.34541841273);
#13103=CIRCLE('',#37639,6.04541841273);
#13104=CIRCLE('',#37641,0.3);
#13105=CIRCLE('',#37642,0.3);
#13106=CIRCLE('',#37644,5.49295371933);
#13107=CIRCLE('',#37645,5.19295371933);
#13108=CIRCLE('',#37647,0.300000000000002);
#13109=CIRCLE('',#37648,0.3);
#13110=CIRCLE('',#37650,0.300000000000002);
#13111=CIRCLE('',#37651,0.3);
#13112=CIRCLE('',#37653,0.3);
#13113=CIRCLE('',#37654,0.3);
#13114=CIRCLE('',#37657,5.19295371933);
#13115=CIRCLE('',#37658,5.49295371933);
#13116=CIRCLE('',#37660,0.6);
#13117=CIRCLE('',#37661,0.3);
#13118=CIRCLE('',#37662,0.3);
#13119=CIRCLE('',#37664,7.54541841273);
#13120=CIRCLE('',#37665,0.3);
#13121=CIRCLE('',#37666,7.84541841273);
#13122=CIRCLE('',#37668,0.3);
#13123=CIRCLE('',#37669,0.6);
#13124=CIRCLE('',#37670,0.3);
#13125=CIRCLE('',#37672,0.6);
#13126=CIRCLE('',#37673,0.3);
#13127=CIRCLE('',#37674,0.3);
#13128=CIRCLE('',#37676,0.3);
#13129=CIRCLE('',#37677,0.3);
#13130=CIRCLE('',#37679,0.999999999999988);
#13131=CIRCLE('',#37681,12.5256279976);
#13132=CIRCLE('',#37683,0.3);
#13133=CIRCLE('',#37685,12.8256279976);
#13134=CIRCLE('',#37687,0.3);
#13135=CIRCLE('',#37688,0.3);
#13136=CIRCLE('',#37690,5.19295371933);
#13137=CIRCLE('',#37691,0.299999999999998);
#13138=CIRCLE('',#37692,5.49295371933);
#13139=CIRCLE('',#37694,0.385778366608001);
#13140=CIRCLE('',#37695,15.8875296363);
#13141=CIRCLE('',#37697,0.3);
#13142=CIRCLE('',#37698,0.299999999999999);
#13143=CIRCLE('',#37699,15.8875296363);
#13144=CIRCLE('',#37701,0.3);
#13145=CIRCLE('',#37702,0.3);
#13146=CIRCLE('',#37703,15.3875296363);
#13147=CIRCLE('',#37705,0.0999999999999999);
#13148=CIRCLE('',#37706,0.0999999999999999);
#13149=CIRCLE('',#37708,0.0999999999999999);
#13150=CIRCLE('',#37709,0.0999999999999999);
#13151=CIRCLE('',#37711,0.4);
#13152=CIRCLE('',#37712,0.0999999999999999);
#13153=CIRCLE('',#37714,0.0999999999999999);
#13154=CIRCLE('',#37716,0.4);
#13155=CIRCLE('',#37717,0.0999999999999999);
#13156=CIRCLE('',#37719,0.0999999999999999);
#13157=CIRCLE('',#37721,0.4);
#13158=CIRCLE('',#37723,0.4);
#13159=CIRCLE('',#37724,0.0999999999999999);
#13160=CIRCLE('',#37726,0.0999999999999999);
#13161=CIRCLE('',#37728,0.0999999999999999);
#13162=CIRCLE('',#37729,0.4);
#13163=CIRCLE('',#37731,0.0999999999999999);
#13164=CIRCLE('',#37733,0.0999999999999999);
#13165=CIRCLE('',#37734,0.4);
#13166=CIRCLE('',#37736,0.0999999999999999);
#13167=CIRCLE('',#37738,0.0999999999999999);
#13168=CIRCLE('',#37739,0.4);
#13169=CIRCLE('',#37741,0.0999999999999999);
#13170=CIRCLE('',#37743,0.4);
#13171=CIRCLE('',#37745,2.7);
#13172=CIRCLE('',#37746,0.6);
#13173=CIRCLE('',#37747,15.8875296363);
#13174=CIRCLE('',#37748,0.985778366608001);
#13175=CIRCLE('',#37751,0.3);
#13176=CIRCLE('',#37752,0.685778366608001);
#13177=CIRCLE('',#37753,0.3);
#13178=CIRCLE('',#37755,0.3);
#13179=CIRCLE('',#37756,0.300000000000006);
#13180=CIRCLE('',#37758,0.3);
#13181=CIRCLE('',#37760,3.);
#13182=CIRCLE('',#37762,3.);
#13183=CIRCLE('',#37770,0.3);
#13184=CIRCLE('',#37773,0.3);
#13185=CIRCLE('',#37775,0.300000000000002);
#13186=CIRCLE('',#37778,0.300000000000002);
#13187=CIRCLE('',#37780,15.3875296363);
#13188=CIRCLE('',#37781,0.300000000000003);
#13189=CIRCLE('',#37783,7.86257571140099);
#13190=CIRCLE('',#37784,0.282842712475);
#13191=CIRCLE('',#37785,0.282842712475);
#13192=CIRCLE('',#37786,14.6703723485088);
#13193=CIRCLE('',#37788,0.3);
#13194=CIRCLE('',#37789,0.3);
#13195=CIRCLE('',#37790,0.3);
#13196=CIRCLE('',#37792,0.3);
#13197=CIRCLE('',#37797,0.3);
#13198=CIRCLE('',#37799,0.3);
#13199=CIRCLE('',#37800,0.299999999999999);
#13200=CIRCLE('',#37802,0.3);
#13201=CIRCLE('',#37804,8.14541841273);
#13202=CIRCLE('',#37805,0.3);
#13203=CIRCLE('',#37807,0.3);
#13204=CIRCLE('',#37809,0.3);
#13205=CIRCLE('',#37811,0.3);
#13206=CIRCLE('',#37813,0.3);
#13207=CIRCLE('',#37815,14.3875296363);
#13208=CIRCLE('',#37821,0.3);
#13209=CIRCLE('',#37824,0.3);
#13210=CIRCLE('',#37826,6.34541841273);
#13211=CIRCLE('',#37840,0.3);
#13212=CIRCLE('',#37842,6.34541841273);
#13213=CIRCLE('',#37844,0.3);
#13214=CIRCLE('',#37846,0.3);
#13215=CIRCLE('',#37849,0.3);
#13216=CIRCLE('',#37851,6.04541841273);
#13217=CIRCLE('',#37853,0.300000000000002);
#13218=CIRCLE('',#37855,0.300000000000002);
#13219=CIRCLE('',#37858,6.04541841273);
#13220=CIRCLE('',#37861,0.3);
#13221=CIRCLE('',#37862,0.3);
#13222=CIRCLE('',#37863,0.3);
#13223=CIRCLE('',#37868,0.685778366608001);
#13224=CIRCLE('',#37870,0.3);
#13225=CIRCLE('',#37873,0.3);
#13226=CIRCLE('',#37880,0.3);
#13227=CIRCLE('',#37881,0.3);
#13228=CIRCLE('',#37882,0.3);
#13229=CIRCLE('',#37885,7.84541841273);
#13230=CIRCLE('',#37887,8.14541841273);
#13231=CIRCLE('',#37889,0.3);
#13232=CIRCLE('',#37890,0.3);
#13233=CIRCLE('',#37892,0.6);
#13234=CIRCLE('',#37893,0.3);
#13235=CIRCLE('',#37895,13.3462109523);
#13236=CIRCLE('',#37896,0.3);
#13237=CIRCLE('',#37898,0.6);
#13238=CIRCLE('',#37899,0.3);
#13239=CIRCLE('',#37901,0.3);
#13240=CIRCLE('',#37903,14.3875296363);
#13241=CIRCLE('',#37904,14.3875296363);
#13242=CIRCLE('',#37906,0.3);
#13243=CIRCLE('',#37907,0.3);
#13244=CIRCLE('',#37908,0.300000000000001);
#13245=CIRCLE('',#37910,14.6875296363);
#13246=CIRCLE('',#37912,0.3);
#13247=CIRCLE('',#37913,1.);
#13248=CIRCLE('',#37915,14.6875296363);
#13249=CIRCLE('',#37921,0.3);
#13250=CIRCLE('',#37923,0.3);
#13251=CIRCLE('',#37929,0.299999999999999);
#13252=CIRCLE('',#37931,0.6);
#13253=CIRCLE('',#37932,0.3);
#13254=CIRCLE('',#37934,7.54541841273);
#13255=CIRCLE('',#37935,0.3);
#13256=CIRCLE('',#37937,0.6);
#13257=CIRCLE('',#37938,0.3);
#13258=CIRCLE('',#37940,0.3);
#13259=CIRCLE('',#37941,0.3);
#13260=CIRCLE('',#37943,0.3);
#13261=CIRCLE('',#37944,0.6);
#13262=CIRCLE('',#37946,0.6);
#13263=CIRCLE('',#37947,0.3);
#13264=CIRCLE('',#37949,14.9875296363);
#13265=CIRCLE('',#37951,0.6);
#13266=CIRCLE('',#37952,0.299999999999999);
#13267=CIRCLE('',#37954,13.216744254);
#13268=CIRCLE('',#37966,15.8875296363);
#13269=CIRCLE('',#37968,15.3875296363);
#13270=CIRCLE('',#37970,0.0999999999999999);
#13271=CIRCLE('',#37971,0.0999999999999999);
#13272=CIRCLE('',#37973,0.0999999999999999);
#13273=CIRCLE('',#37976,0.0999999999999999);
#13274=CIRCLE('',#37978,0.4);
#13275=CIRCLE('',#37980,0.0999999999999999);
#13276=CIRCLE('',#37981,0.4);
#13277=CIRCLE('',#37983,0.0999999999999999);
#13278=CIRCLE('',#37985,0.4);
#13279=CIRCLE('',#37986,0.0999999999999999);
#13280=CIRCLE('',#37990,0.0999999999999999);
#13281=CIRCLE('',#37992,0.4);
#13282=CIRCLE('',#37994,0.6);
#13283=CIRCLE('',#37995,7.54541841273);
#13284=CIRCLE('',#37996,0.6);
#13285=CIRCLE('',#37997,0.6);
#13286=CIRCLE('',#37998,14.9875296363);
#13287=CIRCLE('',#38000,0.999999999999999);
#13288=CIRCLE('',#38002,0.825178907983792);
#13289=CIRCLE('',#38004,0.299999999999999);
#13290=CIRCLE('',#38005,14.6875296363);
#13291=CIRCLE('',#38007,0.300000000000002);
#13292=CIRCLE('',#38008,0.3);
#13293=CIRCLE('',#38010,0.300000000000002);
#13294=CIRCLE('',#38012,0.3);
#13295=CIRCLE('',#38013,0.3);
#13296=CIRCLE('',#38015,0.3);
#13297=CIRCLE('',#38016,7.84541841273);
#13298=CIRCLE('',#38018,0.299999999999999);
#13299=CIRCLE('',#38019,0.3);
#13300=CIRCLE('',#38024,14.6875296363);
#13301=CIRCLE('',#38026,0.999999999999999);
#13302=CIRCLE('',#38028,14.6875296363);
#13303=CIRCLE('',#38030,0.3);
#13304=CIRCLE('',#38032,14.6875296363);
#13305=CIRCLE('',#38034,0.3);
#13306=CIRCLE('',#38037,0.3);
#13307=CIRCLE('',#38039,7.84541841273);
#13308=CIRCLE('',#38041,0.3);
#13309=CIRCLE('',#38044,0.3);
#13310=CIRCLE('',#38046,0.3);
#13311=CIRCLE('',#38047,0.3);
#13312=CIRCLE('',#38049,0.3);
#13313=CIRCLE('',#38050,14.3875296363);
#13314=CIRCLE('',#38052,0.3);
#13315=CIRCLE('',#38053,0.699999999999999);
#13316=CIRCLE('',#38055,0.3);
#13317=CIRCLE('',#38056,0.300000000000001);
#13318=CIRCLE('',#38058,14.3875296363);
#13319=CIRCLE('',#38060,0.3);
#13320=CIRCLE('',#38061,0.3);
#13321=CIRCLE('',#38063,0.300000000000002);
#13322=CIRCLE('',#38064,14.3875296363);
#13323=CIRCLE('',#38066,0.300000000000002);
#13324=CIRCLE('',#38068,0.299999999999998);
#13325=CIRCLE('',#38070,0.3);
#13326=CIRCLE('',#38072,0.299999999999994);
#13327=CIRCLE('',#38073,8.14541841273);
#13328=CIRCLE('',#38075,0.299999999999999);
#13329=CIRCLE('',#38078,0.3);
#13330=CIRCLE('',#38080,0.299999999999999);
#13331=CIRCLE('',#38081,0.6);
#13332=CIRCLE('',#38083,0.299999999999999);
#13333=CIRCLE('',#38084,13.216744254);
#13334=CIRCLE('',#38086,0.6);
#15513=VERTEX_POINT('',#85189);
#15514=VERTEX_POINT('',#85190);
#15515=VERTEX_POINT('',#85209);
#15516=VERTEX_POINT('',#85211);
#15517=VERTEX_POINT('',#85213);
#15518=VERTEX_POINT('',#85217);
#15519=VERTEX_POINT('',#85218);
#15520=VERTEX_POINT('',#85221);
#15521=VERTEX_POINT('',#85225);
#15522=VERTEX_POINT('',#85275);
#15523=VERTEX_POINT('',#85279);
#15524=VERTEX_POINT('',#85280);
#15525=VERTEX_POINT('',#85282);
#15526=VERTEX_POINT('',#85284);
#15527=VERTEX_POINT('',#85302);
#15528=VERTEX_POINT('',#85303);
#15529=VERTEX_POINT('',#85305);
#15530=VERTEX_POINT('',#85307);
#15531=VERTEX_POINT('',#85311);
#15532=VERTEX_POINT('',#85312);
#15533=VERTEX_POINT('',#85317);
#15534=VERTEX_POINT('',#85319);
#15535=VERTEX_POINT('',#85323);
#15536=VERTEX_POINT('',#85324);
#15537=VERTEX_POINT('',#85329);
#15538=VERTEX_POINT('',#85331);
#15539=VERTEX_POINT('',#85333);
#15540=VERTEX_POINT('',#85389);
#15541=VERTEX_POINT('',#85393);
#15542=VERTEX_POINT('',#85394);
#15543=VERTEX_POINT('',#85397);
#15544=VERTEX_POINT('',#85401);
#15545=VERTEX_POINT('',#85402);
#15546=VERTEX_POINT('',#85456);
#15547=VERTEX_POINT('',#85462);
#15548=VERTEX_POINT('',#85468);
#15549=VERTEX_POINT('',#85470);
#15550=VERTEX_POINT('',#85474);
#15551=VERTEX_POINT('',#85476);
#15552=VERTEX_POINT('',#85480);
#15553=VERTEX_POINT('',#85485);
#15554=VERTEX_POINT('',#85489);
#15555=VERTEX_POINT('',#85494);
#15556=VERTEX_POINT('',#85498);
#15557=VERTEX_POINT('',#85504);
#15558=VERTEX_POINT('',#85510);
#15559=VERTEX_POINT('',#85556);
#15560=VERTEX_POINT('',#85560);
#15561=VERTEX_POINT('',#85561);
#15562=VERTEX_POINT('',#85563);
#15563=VERTEX_POINT('',#85565);
#15564=VERTEX_POINT('',#85567);
#15565=VERTEX_POINT('',#85569);
#15566=VERTEX_POINT('',#85613);
#15567=VERTEX_POINT('',#85617);
#15568=VERTEX_POINT('',#85619);
#15569=VERTEX_POINT('',#85623);
#15570=VERTEX_POINT('',#85624);
#15571=VERTEX_POINT('',#85629);
#15572=VERTEX_POINT('',#85631);
#15573=VERTEX_POINT('',#85635);
#15574=VERTEX_POINT('',#85637);
#15575=VERTEX_POINT('',#85641);
#15576=VERTEX_POINT('',#85642);
#15577=VERTEX_POINT('',#85683);
#15578=VERTEX_POINT('',#85685);
#15579=VERTEX_POINT('',#85689);
#15580=VERTEX_POINT('',#85690);
#15581=VERTEX_POINT('',#85697);
#15582=VERTEX_POINT('',#85703);
#15583=VERTEX_POINT('',#85707);
#15584=VERTEX_POINT('',#85711);
#15585=VERTEX_POINT('',#85712);
#15586=VERTEX_POINT('',#85724);
#15587=VERTEX_POINT('',#85725);
#15588=VERTEX_POINT('',#85823);
#15589=VERTEX_POINT('',#85824);
#15590=VERTEX_POINT('',#85826);
#15591=VERTEX_POINT('',#85903);
#15592=VERTEX_POINT('',#85961);
#15593=VERTEX_POINT('',#85963);
#15594=VERTEX_POINT('',#86022);
#15595=VERTEX_POINT('',#86026);
#15596=VERTEX_POINT('',#86028);
#15597=VERTEX_POINT('',#86075);
#15598=VERTEX_POINT('',#86079);
#15599=VERTEX_POINT('',#86080);
#15600=VERTEX_POINT('',#86196);
#15601=VERTEX_POINT('',#86197);
#15602=VERTEX_POINT('',#86204);
#15603=VERTEX_POINT('',#86205);
#15604=VERTEX_POINT('',#86212);
#15605=VERTEX_POINT('',#86214);
#15606=VERTEX_POINT('',#86220);
#15607=VERTEX_POINT('',#86222);
#15608=VERTEX_POINT('',#86228);
#15609=VERTEX_POINT('',#86230);
#15610=VERTEX_POINT('',#86236);
#15611=VERTEX_POINT('',#86238);
#15612=VERTEX_POINT('',#86244);
#15613=VERTEX_POINT('',#86246);
#15614=VERTEX_POINT('',#86252);
#15615=VERTEX_POINT('',#86254);
#15616=VERTEX_POINT('',#86260);
#15617=VERTEX_POINT('',#86261);
#15618=VERTEX_POINT('',#86263);
#15619=VERTEX_POINT('',#86273);
#15620=VERTEX_POINT('',#86274);
#15621=VERTEX_POINT('',#86281);
#15622=VERTEX_POINT('',#86283);
#15623=VERTEX_POINT('',#86341);
#15624=VERTEX_POINT('',#86348);
#15625=VERTEX_POINT('',#86427);
#15626=VERTEX_POINT('',#86429);
#15627=VERTEX_POINT('',#86433);
#15628=VERTEX_POINT('',#86434);
#15629=VERTEX_POINT('',#86436);
#15630=VERTEX_POINT('',#86438);
#15631=VERTEX_POINT('',#86442);
#15632=VERTEX_POINT('',#86443);
#15633=VERTEX_POINT('',#86445);
#15634=VERTEX_POINT('',#86447);
#15635=VERTEX_POINT('',#86506);
#15636=VERTEX_POINT('',#86508);
#15637=VERTEX_POINT('',#86567);
#15638=VERTEX_POINT('',#86569);
#15639=VERTEX_POINT('',#86571);
#15640=VERTEX_POINT('',#86573);
#15641=VERTEX_POINT('',#86575);
#15642=VERTEX_POINT('',#86619);
#15643=VERTEX_POINT('',#86620);
#15644=VERTEX_POINT('',#86622);
#15645=VERTEX_POINT('',#86624);
#15646=VERTEX_POINT('',#86626);
#15647=VERTEX_POINT('',#86630);
#15648=VERTEX_POINT('',#86632);
#15649=VERTEX_POINT('',#86675);
#15650=VERTEX_POINT('',#86677);
#15651=VERTEX_POINT('',#86679);
#15652=VERTEX_POINT('',#86681);
#15653=VERTEX_POINT('',#86685);
#15654=VERTEX_POINT('',#86687);
#15655=VERTEX_POINT('',#86730);
#15656=VERTEX_POINT('',#86732);
#15657=VERTEX_POINT('',#86734);
#15658=VERTEX_POINT('',#86736);
#15659=VERTEX_POINT('',#86748);
#15660=VERTEX_POINT('',#86752);
#15661=VERTEX_POINT('',#86756);
#15662=VERTEX_POINT('',#86758);
#15663=VERTEX_POINT('',#86762);
#15664=VERTEX_POINT('',#86764);
#15665=VERTEX_POINT('',#86766);
#15666=VERTEX_POINT('',#86768);
#15667=VERTEX_POINT('',#86770);
#15668=VERTEX_POINT('',#86774);
#15669=VERTEX_POINT('',#86776);
#15670=VERTEX_POINT('',#86780);
#15671=VERTEX_POINT('',#86782);
#15672=VERTEX_POINT('',#86786);
#15673=VERTEX_POINT('',#86788);
#15674=VERTEX_POINT('',#86792);
#15675=VERTEX_POINT('',#86794);
#15676=VERTEX_POINT('',#86798);
#15677=VERTEX_POINT('',#86799);
#15678=VERTEX_POINT('',#86809);
#15679=VERTEX_POINT('',#86811);
#15680=VERTEX_POINT('',#86818);
#15681=VERTEX_POINT('',#86819);
#15682=VERTEX_POINT('',#86821);
#15683=VERTEX_POINT('',#86826);
#15684=VERTEX_POINT('',#86827);
#15685=VERTEX_POINT('',#86829);
#15686=VERTEX_POINT('',#86831);
#15687=VERTEX_POINT('',#86835);
#15688=VERTEX_POINT('',#86837);
#15689=VERTEX_POINT('',#86841);
#15690=VERTEX_POINT('',#86843);
#15691=VERTEX_POINT('',#86847);
#15692=VERTEX_POINT('',#86849);
#15693=VERTEX_POINT('',#86853);
#15694=VERTEX_POINT('',#86855);
#15695=VERTEX_POINT('',#86859);
#15696=VERTEX_POINT('',#86861);
#15697=VERTEX_POINT('',#86865);
#15698=VERTEX_POINT('',#86867);
#15699=VERTEX_POINT('',#86874);
#15700=VERTEX_POINT('',#86875);
#15701=VERTEX_POINT('',#86877);
#15702=VERTEX_POINT('',#86879);
#15703=VERTEX_POINT('',#86918);
#15704=VERTEX_POINT('',#86920);
#15705=VERTEX_POINT('',#86928);
#15706=VERTEX_POINT('',#86967);
#15707=VERTEX_POINT('',#86969);
#15708=VERTEX_POINT('',#87008);
#15709=VERTEX_POINT('',#87070);
#15710=VERTEX_POINT('',#87072);
#15711=VERTEX_POINT('',#87076);
#15712=VERTEX_POINT('',#87078);
#15713=VERTEX_POINT('',#87082);
#15714=VERTEX_POINT('',#87084);
#15715=VERTEX_POINT('',#87126);
#15716=VERTEX_POINT('',#87128);
#15717=VERTEX_POINT('',#87167);
#15718=VERTEX_POINT('',#87233);
#15719=VERTEX_POINT('',#87237);
#15720=VERTEX_POINT('',#87239);
#15721=VERTEX_POINT('',#87241);
#15722=VERTEX_POINT('',#87243);
#15723=VERTEX_POINT('',#87247);
#15724=VERTEX_POINT('',#87249);
#15725=VERTEX_POINT('',#87253);
#15726=VERTEX_POINT('',#87255);
#15727=VERTEX_POINT('',#87259);
#15728=VERTEX_POINT('',#87261);
#15729=VERTEX_POINT('',#87265);
#15730=VERTEX_POINT('',#87267);
#15731=VERTEX_POINT('',#87271);
#15732=VERTEX_POINT('',#87273);
#15733=VERTEX_POINT('',#87277);
#15734=VERTEX_POINT('',#87279);
#15735=VERTEX_POINT('',#87286);
#15736=VERTEX_POINT('',#87287);
#15737=VERTEX_POINT('',#87289);
#15738=VERTEX_POINT('',#87291);
#15739=VERTEX_POINT('',#87373);
#15740=VERTEX_POINT('',#87375);
#15741=VERTEX_POINT('',#87439);
#15742=VERTEX_POINT('',#87440);
#15743=VERTEX_POINT('',#87442);
#15744=VERTEX_POINT('',#87543);
#15745=VERTEX_POINT('',#87547);
#15746=VERTEX_POINT('',#87551);
#15747=VERTEX_POINT('',#87553);
#15748=VERTEX_POINT('',#87629);
#15749=VERTEX_POINT('',#87633);
#15750=VERTEX_POINT('',#87637);
#15751=VERTEX_POINT('',#87644);
#15752=VERTEX_POINT('',#87646);
#15753=VERTEX_POINT('',#87650);
#15754=VERTEX_POINT('',#87652);
#15755=VERTEX_POINT('',#87656);
#15756=VERTEX_POINT('',#87658);
#15757=VERTEX_POINT('',#87662);
#15758=VERTEX_POINT('',#87664);
#15759=VERTEX_POINT('',#87668);
#15760=VERTEX_POINT('',#87670);
#15761=VERTEX_POINT('',#87674);
#15762=VERTEX_POINT('',#87678);
#15763=VERTEX_POINT('',#87679);
#15764=VERTEX_POINT('',#87686);
#15765=VERTEX_POINT('',#87687);
#15766=VERTEX_POINT('',#87726);
#15767=VERTEX_POINT('',#87727);
#15768=VERTEX_POINT('',#87729);
#15769=VERTEX_POINT('',#87731);
#15770=VERTEX_POINT('',#87735);
#15771=VERTEX_POINT('',#87737);
#15772=VERTEX_POINT('',#87798);
#15773=VERTEX_POINT('',#87799);
#15774=VERTEX_POINT('',#87803);
#15775=VERTEX_POINT('',#87804);
#15776=VERTEX_POINT('',#87809);
#15777=VERTEX_POINT('',#87810);
#15778=VERTEX_POINT('',#87812);
#15779=VERTEX_POINT('',#87814);
#15780=VERTEX_POINT('',#87818);
#15781=VERTEX_POINT('',#87910);
#15782=VERTEX_POINT('',#87914);
#15783=VERTEX_POINT('',#87973);
#15784=VERTEX_POINT('',#87978);
#15785=VERTEX_POINT('',#87980);
#15786=VERTEX_POINT('',#88080);
#15787=VERTEX_POINT('',#88182);
#15788=VERTEX_POINT('',#88232);
#15789=VERTEX_POINT('',#88235);
#15790=VERTEX_POINT('',#88238);
#15791=VERTEX_POINT('',#88243);
#15792=VERTEX_POINT('',#88245);
#15793=VERTEX_POINT('',#88304);
#15794=VERTEX_POINT('',#88314);
#15795=VERTEX_POINT('',#88357);
#15796=VERTEX_POINT('',#88359);
#15797=VERTEX_POINT('',#88361);
#15798=VERTEX_POINT('',#88363);
#15799=VERTEX_POINT('',#88389);
#15800=VERTEX_POINT('',#88391);
#15801=VERTEX_POINT('',#88397);
#15802=VERTEX_POINT('',#88400);
#15803=VERTEX_POINT('',#88417);
#15804=VERTEX_POINT('',#88430);
#15805=VERTEX_POINT('',#88434);
#15806=VERTEX_POINT('',#88440);
#15807=VERTEX_POINT('',#88450);
#15808=VERTEX_POINT('',#88452);
#15809=VERTEX_POINT('',#88459);
#15810=VERTEX_POINT('',#88463);
#15811=VERTEX_POINT('',#88467);
#15812=VERTEX_POINT('',#88498);
#15813=VERTEX_POINT('',#88502);
#15814=VERTEX_POINT('',#88506);
#15815=VERTEX_POINT('',#88510);
#15816=VERTEX_POINT('',#88518);
#15817=VERTEX_POINT('',#88585);
#15818=VERTEX_POINT('',#88590);
#15819=VERTEX_POINT('',#88592);
#15820=VERTEX_POINT('',#88828);
#15821=VERTEX_POINT('',#88832);
#15822=VERTEX_POINT('',#88833);
#15823=VERTEX_POINT('',#88835);
#15824=VERTEX_POINT('',#88846);
#15825=VERTEX_POINT('',#88848);
#15826=VERTEX_POINT('',#88852);
#15827=VERTEX_POINT('',#88856);
#15828=VERTEX_POINT('',#88860);
#15829=VERTEX_POINT('',#88864);
#15830=VERTEX_POINT('',#88868);
#15831=VERTEX_POINT('',#88871);
#15832=VERTEX_POINT('',#88874);
#15833=VERTEX_POINT('',#88876);
#15834=VERTEX_POINT('',#88957);
#15835=VERTEX_POINT('',#88959);
#15836=VERTEX_POINT('',#88973);
#15837=VERTEX_POINT('',#89093);
#15838=VERTEX_POINT('',#89160);
#15839=VERTEX_POINT('',#89164);
#15840=VERTEX_POINT('',#89168);
#15841=VERTEX_POINT('',#89172);
#15842=VERTEX_POINT('',#89176);
#15843=VERTEX_POINT('',#89233);
#15844=VERTEX_POINT('',#89315);
#15845=VERTEX_POINT('',#89319);
#15846=VERTEX_POINT('',#89325);
#15847=VERTEX_POINT('',#89329);
#15848=VERTEX_POINT('',#89368);
#15849=VERTEX_POINT('',#89369);
#15850=VERTEX_POINT('',#89437);
#15851=VERTEX_POINT('',#89494);
#15852=VERTEX_POINT('',#89543);
#15853=VERTEX_POINT('',#89575);
#15854=VERTEX_POINT('',#89628);
#15855=VERTEX_POINT('',#89639);
#15856=VERTEX_POINT('',#89705);
#15857=VERTEX_POINT('',#89707);
#15858=VERTEX_POINT('',#89786);
#15859=VERTEX_POINT('',#89788);
#15860=VERTEX_POINT('',#89792);
#15861=VERTEX_POINT('',#89794);
#15862=VERTEX_POINT('',#89798);
#15863=VERTEX_POINT('',#89800);
#15864=VERTEX_POINT('',#89804);
#15865=VERTEX_POINT('',#89806);
#15866=VERTEX_POINT('',#89810);
#15867=VERTEX_POINT('',#89812);
#15868=VERTEX_POINT('',#89816);
#15869=VERTEX_POINT('',#89818);
#15870=VERTEX_POINT('',#89857);
#15871=VERTEX_POINT('',#89964);
#15872=VERTEX_POINT('',#89966);
#15873=VERTEX_POINT('',#89970);
#15874=VERTEX_POINT('',#89976);
#15875=VERTEX_POINT('',#89980);
#15876=VERTEX_POINT('',#89984);
#15877=VERTEX_POINT('',#89988);
#15878=VERTEX_POINT('',#89992);
#15879=VERTEX_POINT('',#89996);
#15880=VERTEX_POINT('',#90000);
#15881=VERTEX_POINT('',#90004);
#15882=VERTEX_POINT('',#90010);
#15883=VERTEX_POINT('',#90014);
#15884=VERTEX_POINT('',#90018);
#15885=VERTEX_POINT('',#90022);
#15886=VERTEX_POINT('',#90028);
#15887=VERTEX_POINT('',#90032);
#15888=VERTEX_POINT('',#90092);
#15889=VERTEX_POINT('',#90152);
#15890=VERTEX_POINT('',#90214);
#15891=VERTEX_POINT('',#90218);
#15892=VERTEX_POINT('',#90222);
#15893=VERTEX_POINT('',#90229);
#15894=VERTEX_POINT('',#90230);
#15895=VERTEX_POINT('',#90232);
#15896=VERTEX_POINT('',#90234);
#15897=VERTEX_POINT('',#90236);
#15898=VERTEX_POINT('',#90303);
#15899=VERTEX_POINT('',#90304);
#15900=VERTEX_POINT('',#90307);
#15901=VERTEX_POINT('',#90311);
#15902=VERTEX_POINT('',#90313);
#15903=VERTEX_POINT('',#90389);
#15904=VERTEX_POINT('',#90390);
#15905=VERTEX_POINT('',#90406);
#15906=VERTEX_POINT('',#90408);
#15907=VERTEX_POINT('',#90412);
#15908=VERTEX_POINT('',#90413);
#15909=VERTEX_POINT('',#90448);
#15910=VERTEX_POINT('',#90450);
#15911=VERTEX_POINT('',#90454);
#15912=VERTEX_POINT('',#90456);
#15913=VERTEX_POINT('',#90460);
#15914=VERTEX_POINT('',#90462);
#15915=VERTEX_POINT('',#90466);
#15916=VERTEX_POINT('',#90468);
#15917=VERTEX_POINT('',#90472);
#15918=VERTEX_POINT('',#90474);
#15919=VERTEX_POINT('',#90476);
#15920=VERTEX_POINT('',#90486);
#15921=VERTEX_POINT('',#90490);
#15922=VERTEX_POINT('',#90491);
#15923=VERTEX_POINT('',#90494);
#15924=VERTEX_POINT('',#90498);
#15925=VERTEX_POINT('',#90499);
#15926=VERTEX_POINT('',#90502);
#15927=VERTEX_POINT('',#90508);
#15928=VERTEX_POINT('',#90514);
#15929=VERTEX_POINT('',#90515);
#15930=VERTEX_POINT('',#90520);
#15931=VERTEX_POINT('',#90521);
#15932=VERTEX_POINT('',#90526);
#15933=VERTEX_POINT('',#90531);
#15934=VERTEX_POINT('',#90535);
#15935=VERTEX_POINT('',#90540);
#15936=VERTEX_POINT('',#90544);
#15937=VERTEX_POINT('',#90550);
#15938=VERTEX_POINT('',#90556);
#15939=VERTEX_POINT('',#90560);
#15940=VERTEX_POINT('',#90564);
#15941=VERTEX_POINT('',#90565);
#15942=VERTEX_POINT('',#90567);
#15943=VERTEX_POINT('',#90569);
#15944=VERTEX_POINT('',#90613);
#15945=VERTEX_POINT('',#90615);
#15946=VERTEX_POINT('',#90617);
#15947=VERTEX_POINT('',#90621);
#15948=VERTEX_POINT('',#90623);
#15949=VERTEX_POINT('',#90627);
#15950=VERTEX_POINT('',#90629);
#15951=VERTEX_POINT('',#90633);
#15952=VERTEX_POINT('',#90635);
#15953=VERTEX_POINT('',#90639);
#15954=VERTEX_POINT('',#90641);
#15955=VERTEX_POINT('',#90645);
#15956=VERTEX_POINT('',#90647);
#15957=VERTEX_POINT('',#90651);
#15958=VERTEX_POINT('',#90652);
#15959=VERTEX_POINT('',#90657);
#15960=VERTEX_POINT('',#90659);
#15961=VERTEX_POINT('',#90665);
#15962=VERTEX_POINT('',#90671);
#15963=VERTEX_POINT('',#90675);
#15964=VERTEX_POINT('',#90714);
#15965=VERTEX_POINT('',#90848);
#15966=VERTEX_POINT('',#90913);
#15967=VERTEX_POINT('',#90914);
#15968=VERTEX_POINT('',#90916);
#15969=VERTEX_POINT('',#90918);
#15970=VERTEX_POINT('',#91060);
#15971=VERTEX_POINT('',#91116);
#15972=VERTEX_POINT('',#91118);
#15973=VERTEX_POINT('',#91122);
#15974=VERTEX_POINT('',#91181);
#15975=VERTEX_POINT('',#91183);
#15976=VERTEX_POINT('',#91253);
#15977=VERTEX_POINT('',#91313);
#15978=VERTEX_POINT('',#91319);
#15979=VERTEX_POINT('',#91321);
#15980=VERTEX_POINT('',#91327);
#15981=VERTEX_POINT('',#91329);
#15982=VERTEX_POINT('',#91335);
#15983=VERTEX_POINT('',#91336);
#15984=VERTEX_POINT('',#91343);
#15985=VERTEX_POINT('',#91344);
#15986=VERTEX_POINT('',#91351);
#15987=VERTEX_POINT('',#91353);
#15988=VERTEX_POINT('',#91359);
#15989=VERTEX_POINT('',#91361);
#15990=VERTEX_POINT('',#91367);
#15991=VERTEX_POINT('',#91369);
#15992=VERTEX_POINT('',#91375);
#15993=VERTEX_POINT('',#91377);
#15994=VERTEX_POINT('',#91383);
#15995=VERTEX_POINT('',#91384);
#15996=VERTEX_POINT('',#91386);
#15997=VERTEX_POINT('',#91431);
#15998=VERTEX_POINT('',#91489);
#15999=VERTEX_POINT('',#91491);
#16000=VERTEX_POINT('',#91549);
#16001=VERTEX_POINT('',#91550);
#16002=VERTEX_POINT('',#91599);
#16003=VERTEX_POINT('',#91601);
#16004=VERTEX_POINT('',#91605);
#16005=VERTEX_POINT('',#91607);
#16006=VERTEX_POINT('',#91611);
#16007=VERTEX_POINT('',#91612);
#16008=VERTEX_POINT('',#91617);
#16009=VERTEX_POINT('',#91621);
#16010=VERTEX_POINT('',#91662);
#16011=VERTEX_POINT('',#91664);
#16012=VERTEX_POINT('',#91666);
#16013=VERTEX_POINT('',#91668);
#16014=VERTEX_POINT('',#91670);
#16015=VERTEX_POINT('',#91672);
#16016=VERTEX_POINT('',#91731);
#16017=VERTEX_POINT('',#91733);
#16018=VERTEX_POINT('',#91792);
#16019=VERTEX_POINT('',#91796);
#16020=VERTEX_POINT('',#91798);
#16021=VERTEX_POINT('',#91802);
#16022=VERTEX_POINT('',#91804);
#16023=VERTEX_POINT('',#91806);
#16024=VERTEX_POINT('',#91810);
#16025=VERTEX_POINT('',#91812);
#16026=VERTEX_POINT('',#91852);
#16027=VERTEX_POINT('',#91854);
#16028=VERTEX_POINT('',#91856);
#16029=VERTEX_POINT('',#91858);
#16030=VERTEX_POINT('',#91862);
#16031=VERTEX_POINT('',#91864);
#16032=VERTEX_POINT('',#91904);
#16033=VERTEX_POINT('',#91909);
#16034=VERTEX_POINT('',#91914);
#16035=VERTEX_POINT('',#91916);
#16036=VERTEX_POINT('',#91923);
#16037=VERTEX_POINT('',#91927);
#16038=VERTEX_POINT('',#91931);
#16039=VERTEX_POINT('',#91932);
#16040=VERTEX_POINT('',#91935);
#16041=VERTEX_POINT('',#91937);
#16042=VERTEX_POINT('',#91945);
#16043=VERTEX_POINT('',#91947);
#16044=VERTEX_POINT('',#91990);
#16045=VERTEX_POINT('',#91994);
#16046=VERTEX_POINT('',#91996);
#16047=VERTEX_POINT('',#91998);
#16048=VERTEX_POINT('',#92000);
#16049=VERTEX_POINT('',#92002);
#16050=VERTEX_POINT('',#92006);
#16051=VERTEX_POINT('',#92008);
#16052=VERTEX_POINT('',#92012);
#16053=VERTEX_POINT('',#92013);
#16054=VERTEX_POINT('',#92018);
#16055=VERTEX_POINT('',#92020);
#16056=VERTEX_POINT('',#92024);
#16057=VERTEX_POINT('',#92025);
#16058=VERTEX_POINT('',#92030);
#16059=VERTEX_POINT('',#92062);
#16060=VERTEX_POINT('',#92066);
#16061=VERTEX_POINT('',#92068);
#16062=VERTEX_POINT('',#92075);
#16063=VERTEX_POINT('',#92077);
#16064=VERTEX_POINT('',#92079);
#16065=VERTEX_POINT('',#92083);
#16066=VERTEX_POINT('',#92084);
#16067=VERTEX_POINT('',#92086);
#16068=VERTEX_POINT('',#92088);
#16069=VERTEX_POINT('',#92092);
#16070=VERTEX_POINT('',#92093);
#16071=VERTEX_POINT('',#92098);
#16072=VERTEX_POINT('',#92099);
#16073=VERTEX_POINT('',#92104);
#16074=VERTEX_POINT('',#92105);
#16075=VERTEX_POINT('',#92110);
#16076=VERTEX_POINT('',#92111);
#16077=VERTEX_POINT('',#92116);
#16078=VERTEX_POINT('',#92118);
#16079=VERTEX_POINT('',#92122);
#16080=VERTEX_POINT('',#92123);
#16081=VERTEX_POINT('',#92131);
#16082=VERTEX_POINT('',#92132);
#16083=VERTEX_POINT('',#92134);
#16084=VERTEX_POINT('',#92136);
#16085=VERTEX_POINT('',#92169);
#16086=VERTEX_POINT('',#92171);
#16087=VERTEX_POINT('',#92178);
#16088=VERTEX_POINT('',#92218);
#16089=VERTEX_POINT('',#92220);
#16090=VERTEX_POINT('',#92259);
#16091=VERTEX_POINT('',#92318);
#16092=VERTEX_POINT('',#92320);
#16093=VERTEX_POINT('',#92324);
#16094=VERTEX_POINT('',#92325);
#16095=VERTEX_POINT('',#92330);
#16096=VERTEX_POINT('',#92332);
#16097=VERTEX_POINT('',#92374);
#16098=VERTEX_POINT('',#92376);
#16099=VERTEX_POINT('',#92415);
#16100=VERTEX_POINT('',#92481);
#16101=VERTEX_POINT('',#92485);
#16102=VERTEX_POINT('',#92487);
#16103=VERTEX_POINT('',#92489);
#16104=VERTEX_POINT('',#92491);
#16105=VERTEX_POINT('',#92495);
#16106=VERTEX_POINT('',#92496);
#16107=VERTEX_POINT('',#92501);
#16108=VERTEX_POINT('',#92502);
#16109=VERTEX_POINT('',#92507);
#16110=VERTEX_POINT('',#92508);
#16111=VERTEX_POINT('',#92513);
#16112=VERTEX_POINT('',#92514);
#16113=VERTEX_POINT('',#92519);
#16114=VERTEX_POINT('',#92521);
#16115=VERTEX_POINT('',#92525);
#16116=VERTEX_POINT('',#92526);
#16117=VERTEX_POINT('',#92534);
#16118=VERTEX_POINT('',#92535);
#16119=VERTEX_POINT('',#92612);
#16120=VERTEX_POINT('',#92614);
#16121=VERTEX_POINT('',#92675);
#16122=VERTEX_POINT('',#92677);
#16123=VERTEX_POINT('',#92681);
#16124=VERTEX_POINT('',#92682);
#16125=VERTEX_POINT('',#92756);
#16126=VERTEX_POINT('',#92758);
#16127=VERTEX_POINT('',#92828);
#16128=VERTEX_POINT('',#92832);
#16129=VERTEX_POINT('',#92833);
#16130=VERTEX_POINT('',#92949);
#16131=VERTEX_POINT('',#92953);
#16132=VERTEX_POINT('',#92957);
#16133=VERTEX_POINT('',#92964);
#16134=VERTEX_POINT('',#92965);
#16135=VERTEX_POINT('',#93027);
#16136=VERTEX_POINT('',#93029);
#16137=VERTEX_POINT('',#93033);
#16138=VERTEX_POINT('',#93035);
#16139=VERTEX_POINT('',#93039);
#16140=VERTEX_POINT('',#93040);
#16141=VERTEX_POINT('',#93045);
#16142=VERTEX_POINT('',#93047);
#16143=VERTEX_POINT('',#93051);
#16144=VERTEX_POINT('',#93055);
#16145=VERTEX_POINT('',#93059);
#16146=VERTEX_POINT('',#93165);
#16147=VERTEX_POINT('',#93217);
#16148=VERTEX_POINT('',#93218);
#16149=VERTEX_POINT('',#93220);
#16150=VERTEX_POINT('',#93222);
#16151=VERTEX_POINT('',#93226);
#16152=VERTEX_POINT('',#93228);
#16153=VERTEX_POINT('',#93232);
#16154=VERTEX_POINT('',#93233);
#16155=VERTEX_POINT('',#93237);
#16156=VERTEX_POINT('',#93239);
#16157=VERTEX_POINT('',#93243);
#16158=VERTEX_POINT('',#93245);
#16159=VERTEX_POINT('',#93249);
#16160=VERTEX_POINT('',#93251);
#16161=VERTEX_POINT('',#93255);
#16162=VERTEX_POINT('',#93257);
#16163=VERTEX_POINT('',#93261);
#16164=VERTEX_POINT('',#93265);
#16165=VERTEX_POINT('',#93269);
#16166=VERTEX_POINT('',#93273);
#16167=VERTEX_POINT('',#93279);
#16168=VERTEX_POINT('',#93283);
#16169=VERTEX_POINT('',#93287);
#16170=VERTEX_POINT('',#93291);
#16171=VERTEX_POINT('',#93295);
#16172=VERTEX_POINT('',#93299);
#16173=VERTEX_POINT('',#93303);
#16174=VERTEX_POINT('',#93307);
#16175=VERTEX_POINT('',#93314);
#16176=VERTEX_POINT('',#93316);
#16177=VERTEX_POINT('',#93319);
#16178=VERTEX_POINT('',#93524);
#16179=VERTEX_POINT('',#93526);
#16180=VERTEX_POINT('',#93530);
#16181=VERTEX_POINT('',#93532);
#16182=VERTEX_POINT('',#93630);
#16183=VERTEX_POINT('',#93750);
#16184=VERTEX_POINT('',#93823);
#16185=VERTEX_POINT('',#93825);
#16186=VERTEX_POINT('',#93840);
#16187=VERTEX_POINT('',#93844);
#16188=VERTEX_POINT('',#93846);
#16189=VERTEX_POINT('',#93848);
#16190=VERTEX_POINT('',#93850);
#16191=VERTEX_POINT('',#93852);
#16192=VERTEX_POINT('',#93856);
#16193=VERTEX_POINT('',#93859);
#16194=VERTEX_POINT('',#93865);
#16195=VERTEX_POINT('',#93994);
#16196=VERTEX_POINT('',#94018);
#16197=VERTEX_POINT('',#94020);
#16198=VERTEX_POINT('',#94024);
#16199=VERTEX_POINT('',#94025);
#16200=VERTEX_POINT('',#94063);
#16201=VERTEX_POINT('',#94065);
#16202=VERTEX_POINT('',#94072);
#16203=VERTEX_POINT('',#94076);
#16204=VERTEX_POINT('',#94080);
#16205=VERTEX_POINT('',#94111);
#16206=VERTEX_POINT('',#94115);
#16207=VERTEX_POINT('',#94119);
#16208=VERTEX_POINT('',#94123);
#16209=VERTEX_POINT('',#94131);
#16210=VERTEX_POINT('',#94213);
#16211=VERTEX_POINT('',#94218);
#16212=VERTEX_POINT('',#94219);
#16213=VERTEX_POINT('',#94409);
#16214=VERTEX_POINT('',#94410);
#16215=VERTEX_POINT('',#94412);
#16216=VERTEX_POINT('',#94423);
#16217=VERTEX_POINT('',#94424);
#16218=VERTEX_POINT('',#94429);
#16219=VERTEX_POINT('',#94433);
#16220=VERTEX_POINT('',#94437);
#16221=VERTEX_POINT('',#94441);
#16222=VERTEX_POINT('',#94446);
#16223=VERTEX_POINT('',#94450);
#16224=VERTEX_POINT('',#94453);
#16225=VERTEX_POINT('',#94456);
#16226=VERTEX_POINT('',#94623);
#16227=VERTEX_POINT('',#94690);
#16228=VERTEX_POINT('',#94809);
#16229=VERTEX_POINT('',#94830);
#16230=VERTEX_POINT('',#94834);
#16231=VERTEX_POINT('',#94838);
#16232=VERTEX_POINT('',#94842);
#16233=VERTEX_POINT('',#94846);
#16234=VERTEX_POINT('',#94903);
#16235=VERTEX_POINT('',#94915);
#16236=VERTEX_POINT('',#94919);
#16237=VERTEX_POINT('',#94925);
#16238=VERTEX_POINT('',#94929);
#16239=VERTEX_POINT('',#94968);
#16240=VERTEX_POINT('',#94970);
#16241=VERTEX_POINT('',#95056);
#16242=VERTEX_POINT('',#95113);
#16243=VERTEX_POINT('',#95196);
#16244=VERTEX_POINT('',#95248);
#16245=VERTEX_POINT('',#95250);
#16246=VERTEX_POINT('',#95254);
#16247=VERTEX_POINT('',#95260);
#16248=VERTEX_POINT('',#95266);
#16249=VERTEX_POINT('',#95270);
#16250=VERTEX_POINT('',#95274);
#16251=VERTEX_POINT('',#95282);
#16252=VERTEX_POINT('',#95288);
#16253=VERTEX_POINT('',#95290);
#16254=VERTEX_POINT('',#95292);
#16255=VERTEX_POINT('',#95294);
#16256=VERTEX_POINT('',#95296);
#16257=VERTEX_POINT('',#95298);
#16258=VERTEX_POINT('',#95302);
#16259=VERTEX_POINT('',#95303);
#16260=VERTEX_POINT('',#95379);
#16261=VERTEX_POINT('',#95411);
#16262=VERTEX_POINT('',#95542);
#16263=VERTEX_POINT('',#95546);
#16264=VERTEX_POINT('',#95550);
#16265=VERTEX_POINT('',#95554);
#16266=VERTEX_POINT('',#95558);
#16267=VERTEX_POINT('',#95562);
#16268=VERTEX_POINT('',#95601);
#16269=VERTEX_POINT('',#95692);
#16270=VERTEX_POINT('',#95694);
#16271=VERTEX_POINT('',#95698);
#16272=VERTEX_POINT('',#95704);
#16273=VERTEX_POINT('',#95708);
#16274=VERTEX_POINT('',#95712);
#16275=VERTEX_POINT('',#95716);
#16276=VERTEX_POINT('',#95720);
#16277=VERTEX_POINT('',#95724);
#16278=VERTEX_POINT('',#95728);
#16279=VERTEX_POINT('',#95732);
#16280=VERTEX_POINT('',#95738);
#16281=VERTEX_POINT('',#95742);
#16282=VERTEX_POINT('',#95746);
#16283=VERTEX_POINT('',#95750);
#16284=VERTEX_POINT('',#95756);
#16285=VERTEX_POINT('',#95760);
#16286=VERTEX_POINT('',#95766);
#16287=VERTEX_POINT('',#95772);
#16288=VERTEX_POINT('',#95780);
#16289=VERTEX_POINT('',#95784);
#16290=VERTEX_POINT('',#95788);
#19768=EDGE_CURVE('',#15513,#15514,#1874,.T.);
#19769=EDGE_CURVE('',#15515,#15513,#12518,.T.);
#19770=EDGE_CURVE('',#15515,#15516,#8812,.T.);
#19771=EDGE_CURVE('',#15516,#15517,#12519,.T.);
#19772=EDGE_CURVE('',#15514,#15517,#8813,.T.);
#19773=EDGE_CURVE('',#15518,#15519,#8814,.T.);
#19774=EDGE_CURVE('',#15519,#15516,#12520,.T.);
#19775=EDGE_CURVE('',#15520,#15515,#12521,.T.);
#19776=EDGE_CURVE('',#15518,#15520,#636,.T.);
#19777=EDGE_CURVE('',#15521,#15518,#1875,.T.);
#19778=EDGE_CURVE('',#15521,#15522,#8815,.T.);
#19779=EDGE_CURVE('',#15522,#15519,#12522,.T.);
#19780=EDGE_CURVE('',#15523,#15524,#8816,.T.);
#19781=EDGE_CURVE('',#15523,#15525,#12523,.T.);
#19782=EDGE_CURVE('',#15525,#15526,#8817,.T.);
#19783=EDGE_CURVE('',#15526,#15524,#1876,.T.);
#19784=EDGE_CURVE('',#15527,#15528,#8818,.T.);
#19785=EDGE_CURVE('',#15527,#15529,#12524,.T.);
#19786=EDGE_CURVE('',#15529,#15530,#8819,.T.);
#19787=EDGE_CURVE('',#15530,#15528,#12525,.T.);
#19788=EDGE_CURVE('',#15531,#15532,#8820,.T.);
#19789=EDGE_CURVE('',#15532,#15527,#8821,.T.);
#19790=EDGE_CURVE('',#15528,#15531,#8822,.T.);
#19791=EDGE_CURVE('',#15531,#15533,#12526,.T.);
#19792=EDGE_CURVE('',#15533,#15534,#8823,.T.);
#19793=EDGE_CURVE('',#15534,#15532,#12527,.T.);
#19794=EDGE_CURVE('',#15535,#15536,#8824,.T.);
#19795=EDGE_CURVE('',#15536,#15534,#12528,.T.);
#19796=EDGE_CURVE('',#15533,#15535,#12529,.T.);
#19797=EDGE_CURVE('',#15535,#15537,#12530,.T.);
#19798=EDGE_CURVE('',#15537,#15538,#8825,.T.);
#19799=EDGE_CURVE('',#15538,#15539,#1877,.T.);
#19800=EDGE_CURVE('',#15539,#15540,#8826,.T.);
#19801=EDGE_CURVE('',#15540,#15536,#12531,.T.);
#19802=EDGE_CURVE('',#15541,#15542,#8827,.T.);
#19803=EDGE_CURVE('',#15541,#15540,#8828,.T.);
#19804=EDGE_CURVE('',#15539,#15543,#12532,.T.);
#19805=EDGE_CURVE('',#15543,#15542,#8829,.T.);
#19806=EDGE_CURVE('',#15544,#15545,#1878,.T.);
#19807=EDGE_CURVE('',#15517,#15544,#8830,.T.);
#19808=EDGE_CURVE('',#15546,#15517,#12533,.T.);
#19809=EDGE_CURVE('',#15546,#15545,#8831,.T.);
#19810=EDGE_CURVE('',#15546,#15516,#12534,.T.);
#19811=EDGE_CURVE('',#15547,#15546,#12535,.T.);
#19812=EDGE_CURVE('',#15547,#15519,#12536,.T.);
#19813=EDGE_CURVE('',#15547,#15522,#12537,.T.);
#19814=EDGE_CURVE('',#15548,#15547,#8832,.T.);
#19815=EDGE_CURVE('',#15549,#15522,#8833,.T.);
#19816=EDGE_CURVE('',#15548,#15549,#12538,.T.);
#19817=EDGE_CURVE('',#15550,#15548,#12539,.T.);
#19818=EDGE_CURVE('',#15551,#15549,#12540,.T.);
#19819=EDGE_CURVE('',#15550,#15551,#12541,.T.);
#19820=EDGE_CURVE('',#15552,#15550,#12542,.T.);
#19821=EDGE_CURVE('',#15525,#15551,#12543,.T.);
#19822=EDGE_CURVE('',#15552,#15525,#12544,.T.);
#19823=EDGE_CURVE('',#15553,#15552,#12545,.T.);
#19824=EDGE_CURVE('',#15553,#15523,#12546,.T.);
#19825=EDGE_CURVE('',#15554,#15553,#12547,.T.);
#19826=EDGE_CURVE('',#15529,#15523,#12548,.T.);
#19827=EDGE_CURVE('',#15554,#15529,#12549,.T.);
#19828=EDGE_CURVE('',#15555,#15554,#12550,.T.);
#19829=EDGE_CURVE('',#15555,#15527,#12551,.T.);
#19830=EDGE_CURVE('',#15556,#15555,#8834,.T.);
#19831=EDGE_CURVE('',#15556,#15532,#12552,.T.);
#19832=EDGE_CURVE('',#15556,#15534,#12553,.T.);
#19833=EDGE_CURVE('',#15557,#15556,#12554,.T.);
#19834=EDGE_CURVE('',#15557,#15536,#12555,.T.);
#19835=EDGE_CURVE('',#15557,#15540,#12556,.T.);
#19836=EDGE_CURVE('',#15558,#15541,#1879,.T.);
#19837=EDGE_CURVE('',#15558,#15557,#8835,.T.);
#19838=EDGE_CURVE('',#15559,#15558,#12557,.T.);
#19839=EDGE_CURVE('',#15545,#15559,#12558,.T.);
#19840=EDGE_CURVE('',#15560,#15561,#8836,.T.);
#19841=EDGE_CURVE('',#15561,#15562,#8837,.T.);
#19842=EDGE_CURVE('',#15563,#15562,#8838,.T.);
#19843=EDGE_CURVE('',#15564,#15563,#8839,.T.);
#19844=EDGE_CURVE('',#15565,#15564,#1880,.T.);
#19845=EDGE_CURVE('',#15566,#15565,#8840,.T.);
#19846=EDGE_CURVE('',#15560,#15566,#8841,.T.);
#19847=EDGE_CURVE('',#15567,#15560,#12559,.T.);
#19848=EDGE_CURVE('',#15567,#15568,#8842,.T.);
#19849=EDGE_CURVE('',#15568,#15561,#12560,.T.);
#19850=EDGE_CURVE('',#15569,#15570,#8843,.T.);
#19851=EDGE_CURVE('',#15570,#15568,#12561,.T.);
#19852=EDGE_CURVE('',#15569,#15567,#12562,.T.);
#19853=EDGE_CURVE('',#15571,#15569,#12563,.T.);
#19854=EDGE_CURVE('',#15571,#15572,#8844,.T.);
#19855=EDGE_CURVE('',#15572,#15570,#12564,.T.);
#19856=EDGE_CURVE('',#15573,#15571,#8845,.T.);
#19857=EDGE_CURVE('',#15574,#15573,#8846,.T.);
#19858=EDGE_CURVE('',#15574,#15572,#8847,.T.);
#19859=EDGE_CURVE('',#15575,#15576,#8848,.T.);
#19860=EDGE_CURVE('',#15575,#15574,#12565,.T.);
#19861=EDGE_CURVE('',#15576,#15573,#1881,.T.);
#19862=EDGE_CURVE('',#15577,#15563,#12566,.T.);
#19863=EDGE_CURVE('',#15562,#15578,#12567,.T.);
#19864=EDGE_CURVE('',#15577,#15578,#8849,.T.);
#19865=EDGE_CURVE('',#15579,#15580,#8850,.T.);
#19866=EDGE_CURVE('',#15580,#15562,#12568,.T.);
#19867=EDGE_CURVE('',#15579,#15561,#12569,.T.);
#19868=EDGE_CURVE('',#15579,#15568,#12570,.T.);
#19869=EDGE_CURVE('',#15581,#15579,#12571,.T.);
#19870=EDGE_CURVE('',#15581,#15570,#12572,.T.);
#19871=EDGE_CURVE('',#15581,#15572,#12573,.T.);
#19872=EDGE_CURVE('',#15582,#15581,#8851,.T.);
#19873=EDGE_CURVE('',#15582,#15574,#12574,.T.);
#19874=EDGE_CURVE('',#15583,#15582,#12575,.T.);
#19875=EDGE_CURVE('',#15583,#15575,#12576,.T.);
#19876=EDGE_CURVE('',#15584,#15585,#1882,.T.);
#19877=EDGE_CURVE('',#15584,#15583,#12577,.T.);
#19878=EDGE_CURVE('',#15585,#15575,#12578,.T.);
#19879=EDGE_CURVE('',#15580,#15578,#12579,.T.);
#19880=EDGE_CURVE('',#15586,#15587,#1883,.T.);
#19881=EDGE_CURVE('',#15578,#15587,#12580,.T.);
#19882=EDGE_CURVE('',#15580,#15586,#12581,.T.);
#19883=EDGE_CURVE('',#15588,#15589,#8852,.T.);
#19884=EDGE_CURVE('',#15590,#15588,#1884,.T.);
#19885=EDGE_CURVE('',#15590,#15591,#8853,.T.);
#19886=EDGE_CURVE('',#15589,#15591,#1885,.T.);
#19887=EDGE_CURVE('',#15591,#15592,#12582,.T.);
#19888=EDGE_CURVE('',#15593,#15592,#1886,.T.);
#19889=EDGE_CURVE('',#15594,#15593,#12583,.T.);
#19890=EDGE_CURVE('',#15594,#15591,#12584,.T.);
#19891=EDGE_CURVE('',#15592,#15595,#8854,.T.);
#19892=EDGE_CURVE('',#15595,#15596,#1887,.T.);
#19893=EDGE_CURVE('',#15597,#15596,#8855,.T.);
#19894=EDGE_CURVE('',#15597,#15592,#12585,.T.);
#19895=EDGE_CURVE('',#15598,#15599,#12586,.T.);
#19896=EDGE_CURVE('',#15595,#15598,#1888,.T.);
#19897=EDGE_CURVE('',#15595,#15590,#12587,.T.);
#19898=EDGE_CURVE('',#15590,#15599,#12588,.T.);
#19899=EDGE_CURVE('',#15599,#15588,#12589,.T.);
#19900=EDGE_CURVE('',#15600,#15601,#8856,.T.);
#19901=EDGE_CURVE('',#15588,#15600,#8857,.T.);
#19902=EDGE_CURVE('',#15601,#15589,#8858,.T.);
#19903=EDGE_CURVE('',#15594,#15589,#12590,.T.);
#19904=EDGE_CURVE('',#15602,#15603,#12591,.T.);
#19905=EDGE_CURVE('',#15602,#15594,#8859,.T.);
#19906=EDGE_CURVE('',#15603,#15593,#8860,.T.);
#19907=EDGE_CURVE('',#15597,#15593,#12592,.T.);
#19908=EDGE_CURVE('',#15604,#15597,#8861,.T.);
#19909=EDGE_CURVE('',#15596,#15605,#8862,.T.);
#19910=EDGE_CURVE('',#15604,#15605,#8863,.T.);
#19911=EDGE_CURVE('',#15596,#15598,#12593,.T.);
#19912=EDGE_CURVE('',#15598,#15606,#8864,.T.);
#19913=EDGE_CURVE('',#15599,#15607,#8865,.T.);
#19914=EDGE_CURVE('',#15606,#15607,#12594,.T.);
#19915=EDGE_CURVE('',#15607,#15600,#12595,.T.);
#19916=EDGE_CURVE('',#15601,#15608,#12596,.T.);
#19917=EDGE_CURVE('',#15609,#15608,#8866,.T.);
#19918=EDGE_CURVE('',#15600,#15609,#12597,.T.);
#19919=EDGE_CURVE('',#15601,#15602,#12598,.T.);
#19920=EDGE_CURVE('',#15603,#15610,#12599,.T.);
#19921=EDGE_CURVE('',#15611,#15610,#12600,.T.);
#19922=EDGE_CURVE('',#15602,#15611,#12601,.T.);
#19923=EDGE_CURVE('',#15603,#15604,#12602,.T.);
#19924=EDGE_CURVE('',#15605,#15612,#12603,.T.);
#19925=EDGE_CURVE('',#15613,#15612,#8867,.T.);
#19926=EDGE_CURVE('',#15604,#15613,#12604,.T.);
#19927=EDGE_CURVE('',#15605,#15606,#12605,.T.);
#19928=EDGE_CURVE('',#15607,#15614,#12606,.T.);
#19929=EDGE_CURVE('',#15615,#15614,#12607,.T.);
#19930=EDGE_CURVE('',#15606,#15615,#12608,.T.);
#19931=EDGE_CURVE('',#15614,#15609,#12609,.T.);
#19932=EDGE_CURVE('',#15616,#15617,#12610,.T.);
#19933=EDGE_CURVE('',#15617,#15618,#12611,.T.);
#19934=EDGE_CURVE('',#15616,#15618,#12612,.T.);
#19935=EDGE_CURVE('',#15608,#15611,#12613,.T.);
#19936=EDGE_CURVE('',#15610,#15613,#12614,.T.);
#19937=EDGE_CURVE('',#15612,#15615,#12615,.T.);
#19938=EDGE_CURVE('',#15619,#15620,#1889,.T.);
#19939=EDGE_CURVE('',#15621,#15619,#12616,.T.);
#19940=EDGE_CURVE('',#15621,#15622,#12617,.T.);
#19941=EDGE_CURVE('',#15622,#15620,#12618,.T.);
#19942=EDGE_CURVE('',#15623,#15565,#1890,.T.);
#19943=EDGE_CURVE('',#15624,#15564,#637,.T.);
#19944=EDGE_CURVE('',#15623,#15624,#1891,.T.);
#19945=EDGE_CURVE('',#15625,#15624,#12619,.T.);
#19946=EDGE_CURVE('',#15626,#15625,#12620,.T.);
#19947=EDGE_CURVE('',#15626,#15623,#12621,.T.);
#19948=EDGE_CURVE('',#15627,#15628,#8868,.T.);
#19949=EDGE_CURVE('',#15628,#15629,#8869,.T.);
#19950=EDGE_CURVE('',#15629,#15630,#8870,.T.);
#19951=EDGE_CURVE('',#15627,#15630,#8871,.T.);
#19952=EDGE_CURVE('',#15631,#15632,#12622,.T.);
#19953=EDGE_CURVE('',#15632,#15633,#8872,.T.);
#19954=EDGE_CURVE('',#15633,#15634,#1892,.T.);
#19955=EDGE_CURVE('',#15634,#15635,#12623,.T.);
#19956=EDGE_CURVE('',#15635,#15636,#1893,.T.);
#19957=EDGE_CURVE('',#15636,#15637,#8873,.T.);
#19958=EDGE_CURVE('',#15637,#15638,#12624,.T.);
#19959=EDGE_CURVE('',#15638,#15639,#8874,.T.);
#19960=EDGE_CURVE('',#15639,#15640,#638,.T.);
#19961=EDGE_CURVE('',#15640,#15641,#12625,.T.);
#19962=EDGE_CURVE('',#15641,#15577,#1894,.T.);
#19963=EDGE_CURVE('',#15587,#15631,#8875,.T.);
#19964=EDGE_CURVE('',#15642,#15643,#8876,.T.);
#19965=EDGE_CURVE('',#15643,#15644,#8877,.T.);
#19966=EDGE_CURVE('',#15644,#15645,#639,.T.);
#19967=EDGE_CURVE('',#15645,#15646,#8878,.T.);
#19968=EDGE_CURVE('',#15642,#15646,#8879,.T.);
#19969=EDGE_CURVE('',#15643,#15647,#12626,.T.);
#19970=EDGE_CURVE('',#15647,#15648,#8880,.T.);
#19971=EDGE_CURVE('',#15648,#15644,#1895,.T.);
#19972=EDGE_CURVE('',#15647,#15649,#8881,.T.);
#19973=EDGE_CURVE('',#15649,#15650,#8882,.T.);
#19974=EDGE_CURVE('',#15650,#15651,#640,.T.);
#19975=EDGE_CURVE('',#15651,#15652,#8883,.T.);
#19976=EDGE_CURVE('',#15652,#15648,#641,.T.);
#19977=EDGE_CURVE('',#15649,#15653,#12627,.T.);
#19978=EDGE_CURVE('',#15653,#15654,#8884,.T.);
#19979=EDGE_CURVE('',#15654,#15650,#1896,.T.);
#19980=EDGE_CURVE('',#15653,#15655,#8885,.T.);
#19981=EDGE_CURVE('',#15655,#15656,#8886,.T.);
#19982=EDGE_CURVE('',#15656,#15657,#8887,.T.);
#19983=EDGE_CURVE('',#15657,#15658,#1897,.T.);
#19984=EDGE_CURVE('',#15658,#15654,#642,.T.);
#19985=EDGE_CURVE('',#15655,#15627,#12628,.T.);
#19986=EDGE_CURVE('',#15630,#15656,#12629,.T.);
#19987=EDGE_CURVE('',#15545,#15659,#12630,.T.);
#19988=EDGE_CURVE('',#15544,#15659,#12631,.T.);
#19989=EDGE_CURVE('',#15559,#15660,#12632,.T.);
#19990=EDGE_CURVE('',#15659,#15660,#12633,.T.);
#19991=EDGE_CURVE('',#15661,#15544,#8888,.T.);
#19992=EDGE_CURVE('',#15662,#15659,#8889,.T.);
#19993=EDGE_CURVE('',#15661,#15662,#643,.T.);
#19994=EDGE_CURVE('',#15663,#15661,#8890,.T.);
#19995=EDGE_CURVE('',#15664,#15663,#12634,.T.);
#19996=EDGE_CURVE('',#15665,#15664,#8891,.T.);
#19997=EDGE_CURVE('',#15666,#15665,#8892,.T.);
#19998=EDGE_CURVE('',#15666,#15667,#8893,.T.);
#19999=EDGE_CURVE('',#15514,#15667,#8894,.T.);
#20000=EDGE_CURVE('',#15668,#15666,#12635,.T.);
#20001=EDGE_CURVE('',#15668,#15669,#8895,.T.);
#20002=EDGE_CURVE('',#15667,#15669,#12636,.T.);
#20003=EDGE_CURVE('',#15669,#15670,#12637,.T.);
#20004=EDGE_CURVE('',#15671,#15668,#12638,.T.);
#20005=EDGE_CURVE('',#15671,#15670,#8896,.T.);
#20006=EDGE_CURVE('',#15672,#15671,#12639,.T.);
#20007=EDGE_CURVE('',#15672,#15673,#8897,.T.);
#20008=EDGE_CURVE('',#15670,#15673,#12640,.T.);
#20009=EDGE_CURVE('',#15673,#15674,#8898,.T.);
#20010=EDGE_CURVE('',#15675,#15672,#8899,.T.);
#20011=EDGE_CURVE('',#15675,#15674,#8900,.T.);
#20012=EDGE_CURVE('',#15676,#15677,#8901,.T.);
#20013=EDGE_CURVE('',#15665,#15676,#12641,.T.);
#20014=EDGE_CURVE('',#15677,#15664,#1898,.T.);
#20015=EDGE_CURVE('',#15678,#15675,#12642,.T.);
#20016=EDGE_CURVE('',#15678,#15679,#8902,.T.);
#20017=EDGE_CURVE('',#15674,#15679,#12643,.T.);
#20018=EDGE_CURVE('',#15676,#15678,#12644,.T.);
#20019=EDGE_CURVE('',#15679,#15677,#12645,.T.);
#20020=EDGE_CURVE('',#15680,#15681,#8903,.T.);
#20021=EDGE_CURVE('',#15681,#15682,#12646,.T.);
#20022=EDGE_CURVE('',#15622,#15682,#8904,.T.);
#20023=EDGE_CURVE('',#15680,#15622,#12647,.T.);
#20024=EDGE_CURVE('',#15683,#15684,#12648,.T.);
#20025=EDGE_CURVE('',#15684,#15685,#12649,.T.);
#20026=EDGE_CURVE('',#15686,#15685,#12650,.T.);
#20027=EDGE_CURVE('',#15683,#15686,#12651,.T.);
#20028=EDGE_CURVE('',#15687,#15683,#12652,.T.);
#20029=EDGE_CURVE('',#15688,#15686,#12653,.T.);
#20030=EDGE_CURVE('',#15687,#15688,#12654,.T.);
#20031=EDGE_CURVE('',#15689,#15687,#8905,.T.);
#20032=EDGE_CURVE('',#15690,#15688,#8906,.T.);
#20033=EDGE_CURVE('',#15689,#15690,#12655,.T.);
#20034=EDGE_CURVE('',#15691,#15689,#12656,.T.);
#20035=EDGE_CURVE('',#15692,#15690,#12657,.T.);
#20036=EDGE_CURVE('',#15691,#15692,#12658,.T.);
#20037=EDGE_CURVE('',#15693,#15691,#12659,.T.);
#20038=EDGE_CURVE('',#15694,#15692,#12660,.T.);
#20039=EDGE_CURVE('',#15693,#15694,#12661,.T.);
#20040=EDGE_CURVE('',#15684,#15695,#12662,.T.);
#20041=EDGE_CURVE('',#15695,#15696,#12663,.T.);
#20042=EDGE_CURVE('',#15685,#15696,#12664,.T.);
#20043=EDGE_CURVE('',#15697,#15693,#12665,.T.);
#20044=EDGE_CURVE('',#15698,#15694,#12666,.T.);
#20045=EDGE_CURVE('',#15697,#15698,#12667,.T.);
#20046=EDGE_CURVE('',#15695,#15697,#8907,.T.);
#20047=EDGE_CURVE('',#15696,#15698,#8908,.T.);
#20048=EDGE_CURVE('',#15699,#15700,#12668,.T.);
#20049=EDGE_CURVE('',#15700,#15701,#12669,.T.);
#20050=EDGE_CURVE('',#15702,#15701,#12670,.T.);
#20051=EDGE_CURVE('',#15699,#15702,#12671,.T.);
#20052=EDGE_CURVE('',#15657,#15703,#644,.T.);
#20053=EDGE_CURVE('',#15703,#15704,#1899,.T.);
#20054=EDGE_CURVE('',#15658,#15704,#645,.T.);
#20055=EDGE_CURVE('',#15701,#15703,#12672,.T.);
#20056=EDGE_CURVE('',#15700,#15705,#12673,.T.);
#20057=EDGE_CURVE('',#15705,#15704,#12674,.T.);
#20058=EDGE_CURVE('',#15650,#15706,#646,.T.);
#20059=EDGE_CURVE('',#15706,#15707,#647,.T.);
#20060=EDGE_CURVE('',#15651,#15707,#648,.T.);
#20061=EDGE_CURVE('',#15654,#15708,#649,.T.);
#20062=EDGE_CURVE('',#15708,#15706,#1900,.T.);
#20063=EDGE_CURVE('',#15704,#15708,#650,.T.);
#20064=EDGE_CURVE('',#15705,#15709,#12675,.T.);
#20065=EDGE_CURVE('',#15709,#15710,#12676,.T.);
#20066=EDGE_CURVE('',#15707,#15710,#12677,.T.);
#20067=EDGE_CURVE('',#15711,#15699,#12678,.T.);
#20068=EDGE_CURVE('',#15712,#15702,#12679,.T.);
#20069=EDGE_CURVE('',#15711,#15712,#12680,.T.);
#20070=EDGE_CURVE('',#15709,#15713,#12681,.T.);
#20071=EDGE_CURVE('',#15713,#15714,#12682,.T.);
#20072=EDGE_CURVE('',#15710,#15714,#12683,.T.);
#20073=EDGE_CURVE('',#15713,#15711,#8909,.T.);
#20074=EDGE_CURVE('',#15714,#15712,#8910,.T.);
#20075=EDGE_CURVE('',#15644,#15715,#651,.T.);
#20076=EDGE_CURVE('',#15715,#15716,#652,.T.);
#20077=EDGE_CURVE('',#15645,#15716,#653,.T.);
#20078=EDGE_CURVE('',#15648,#15717,#654,.T.);
#20079=EDGE_CURVE('',#15717,#15715,#1901,.T.);
#20080=EDGE_CURVE('',#15652,#15718,#655,.T.);
#20081=EDGE_CURVE('',#15718,#15717,#656,.T.);
#20082=EDGE_CURVE('',#15718,#15719,#12684,.T.);
#20083=EDGE_CURVE('',#15719,#15720,#12685,.T.);
#20084=EDGE_CURVE('',#15721,#15720,#12686,.T.);
#20085=EDGE_CURVE('',#15722,#15721,#12687,.T.);
#20086=EDGE_CURVE('',#15722,#15716,#12688,.T.);
#20087=EDGE_CURVE('',#15723,#15722,#12689,.T.);
#20088=EDGE_CURVE('',#15724,#15721,#12690,.T.);
#20089=EDGE_CURVE('',#15723,#15724,#12691,.T.);
#20090=EDGE_CURVE('',#15725,#15723,#8911,.T.);
#20091=EDGE_CURVE('',#15726,#15724,#8912,.T.);
#20092=EDGE_CURVE('',#15725,#15726,#12692,.T.);
#20093=EDGE_CURVE('',#15727,#15725,#12693,.T.);
#20094=EDGE_CURVE('',#15728,#15726,#12694,.T.);
#20095=EDGE_CURVE('',#15727,#15728,#12695,.T.);
#20096=EDGE_CURVE('',#15729,#15727,#12696,.T.);
#20097=EDGE_CURVE('',#15730,#15728,#12697,.T.);
#20098=EDGE_CURVE('',#15729,#15730,#12698,.T.);
#20099=EDGE_CURVE('',#15719,#15731,#12699,.T.);
#20100=EDGE_CURVE('',#15731,#15732,#12700,.T.);
#20101=EDGE_CURVE('',#15720,#15732,#12701,.T.);
#20102=EDGE_CURVE('',#15733,#15729,#12702,.T.);
#20103=EDGE_CURVE('',#15734,#15730,#12703,.T.);
#20104=EDGE_CURVE('',#15733,#15734,#12704,.T.);
#20105=EDGE_CURVE('',#15731,#15733,#8913,.T.);
#20106=EDGE_CURVE('',#15732,#15734,#8914,.T.);
#20107=EDGE_CURVE('',#15735,#15736,#8915,.T.);
#20108=EDGE_CURVE('',#15736,#15737,#12705,.T.);
#20109=EDGE_CURVE('',#15738,#15737,#8916,.T.);
#20110=EDGE_CURVE('',#15735,#15738,#1902,.T.);
#20111=EDGE_CURVE('',#15618,#15739,#8917,.T.);
#20112=EDGE_CURVE('',#15740,#15739,#1903,.T.);
#20113=EDGE_CURVE('',#15616,#15740,#8918,.T.);
#20114=EDGE_CURVE('',#15741,#15742,#12706,.T.);
#20115=EDGE_CURVE('',#15743,#15741,#1904,.T.);
#20116=EDGE_CURVE('',#15743,#15744,#12707,.T.);
#20117=EDGE_CURVE('',#15744,#15742,#12708,.T.);
#20118=EDGE_CURVE('',#15745,#15743,#12709,.T.);
#20119=EDGE_CURVE('',#15745,#15741,#12710,.T.);
#20120=EDGE_CURVE('',#15746,#15745,#12711,.T.);
#20121=EDGE_CURVE('',#15747,#15741,#12712,.T.);
#20122=EDGE_CURVE('',#15746,#15747,#1905,.T.);
#20123=EDGE_CURVE('',#15744,#15748,#12713,.T.);
#20124=EDGE_CURVE('',#15748,#15742,#12714,.T.);
#20125=EDGE_CURVE('',#15749,#15746,#12715,.T.);
#20126=EDGE_CURVE('',#15749,#15747,#12716,.T.);
#20127=EDGE_CURVE('',#15750,#15738,#12717,.T.);
#20128=EDGE_CURVE('',#15735,#15750,#12718,.T.);
#20129=EDGE_CURVE('',#15748,#15749,#8919,.T.);
#20130=EDGE_CURVE('',#15742,#15747,#8920,.T.);
#20131=EDGE_CURVE('',#15751,#15735,#12719,.T.);
#20132=EDGE_CURVE('',#15752,#15750,#12720,.T.);
#20133=EDGE_CURVE('',#15752,#15751,#12721,.T.);
#20134=EDGE_CURVE('',#15681,#15753,#12722,.T.);
#20135=EDGE_CURVE('',#15753,#15754,#12723,.T.);
#20136=EDGE_CURVE('',#15682,#15754,#12724,.T.);
#20137=EDGE_CURVE('',#15753,#15755,#12725,.T.);
#20138=EDGE_CURVE('',#15755,#15756,#12726,.T.);
#20139=EDGE_CURVE('',#15754,#15756,#12727,.T.);
#20140=EDGE_CURVE('',#15757,#15626,#12728,.T.);
#20141=EDGE_CURVE('',#15758,#15625,#12729,.T.);
#20142=EDGE_CURVE('',#15757,#15758,#12730,.T.);
#20143=EDGE_CURVE('',#15755,#15759,#12731,.T.);
#20144=EDGE_CURVE('',#15759,#15760,#12732,.T.);
#20145=EDGE_CURVE('',#15756,#15760,#12733,.T.);
#20146=EDGE_CURVE('',#15761,#15740,#12734,.T.);
#20147=EDGE_CURVE('',#15761,#15739,#12735,.T.);
#20148=EDGE_CURVE('',#15762,#15763,#12736,.T.);
#20149=EDGE_CURVE('',#15763,#15621,#8921,.T.);
#20150=EDGE_CURVE('',#15762,#15619,#8922,.T.);
#20151=EDGE_CURVE('',#15621,#15680,#12737,.T.);
#20152=EDGE_CURVE('',#15764,#15765,#12738,.T.);
#20153=EDGE_CURVE('',#15765,#15763,#1906,.T.);
#20154=EDGE_CURVE('',#15764,#15762,#1907,.T.);
#20155=EDGE_CURVE('',#15766,#15767,#8923,.T.);
#20156=EDGE_CURVE('',#15768,#15766,#12739,.T.);
#20157=EDGE_CURVE('',#15768,#15769,#8924,.T.);
#20158=EDGE_CURVE('',#15767,#15769,#12740,.T.);
#20159=EDGE_CURVE('',#15739,#15770,#12741,.T.);
#20160=EDGE_CURVE('',#15771,#15770,#1908,.T.);
#20161=EDGE_CURVE('',#15761,#15771,#12742,.T.);
#20162=EDGE_CURVE('',#15772,#15773,#12743,.T.);
#20163=EDGE_CURVE('',#15772,#15773,#12744,.T.);
#20164=EDGE_CURVE('',#15774,#15775,#12745,.T.);
#20165=EDGE_CURVE('',#15775,#15638,#12746,.T.);
#20166=EDGE_CURVE('',#15774,#15637,#12747,.T.);
#20167=EDGE_CURVE('',#15776,#15777,#12748,.T.);
#20168=EDGE_CURVE('',#15777,#15778,#12749,.T.);
#20169=EDGE_CURVE('',#15779,#15778,#12750,.T.);
#20170=EDGE_CURVE('',#15776,#15779,#12751,.T.);
#20171=EDGE_CURVE('',#15631,#15780,#1909,.T.);
#20172=EDGE_CURVE('',#15780,#15781,#12752,.T.);
#20173=EDGE_CURVE('',#15781,#15632,#12753,.T.);
#20174=EDGE_CURVE('',#15782,#15774,#1910,.T.);
#20175=EDGE_CURVE('',#15782,#15783,#12754,.T.);
#20176=EDGE_CURVE('',#15783,#15781,#12755,.T.);
#20177=EDGE_CURVE('',#15774,#15781,#12756,.T.);
#20178=EDGE_CURVE('',#15542,#15784,#12757,.T.);
#20179=EDGE_CURVE('',#15785,#15784,#8925,.T.);
#20180=EDGE_CURVE('',#15541,#15785,#12758,.T.);
#20181=EDGE_CURVE('',#15558,#15785,#12759,.T.);
#20182=EDGE_CURVE('',#15660,#15785,#12760,.T.);
#20183=EDGE_CURVE('',#15775,#15776,#12761,.T.);
#20184=EDGE_CURVE('',#15638,#15779,#12762,.T.);
#20185=EDGE_CURVE('',#15779,#15660,#8926,.T.);
#20186=EDGE_CURVE('',#15784,#15639,#1911,.T.);
#20187=EDGE_CURVE('',#15786,#15772,#1912,.T.);
#20188=EDGE_CURVE('',#15772,#15634,#657,.T.);
#20189=EDGE_CURVE('',#15786,#15633,#658,.T.);
#20190=EDGE_CURVE('',#15773,#15635,#12763,.T.);
#20191=EDGE_CURVE('',#15773,#15787,#1913,.T.);
#20192=EDGE_CURVE('',#15787,#15636,#659,.T.);
#20193=EDGE_CURVE('',#15782,#15637,#12764,.T.);
#20194=EDGE_CURVE('',#15787,#15782,#8927,.T.);
#20195=EDGE_CURVE('',#15783,#15786,#8928,.T.);
#20196=EDGE_CURVE('',#15783,#15632,#12765,.T.);
#20197=EDGE_CURVE('',#15777,#15788,#12766,.T.);
#20198=EDGE_CURVE('',#15788,#15778,#12767,.T.);
#20199=EDGE_CURVE('',#15789,#15777,#12768,.T.);
#20200=EDGE_CURVE('',#15790,#15777,#8929,.T.);
#20201=EDGE_CURVE('',#15769,#15790,#12769,.T.);
#20202=EDGE_CURVE('',#15769,#15788,#8930,.T.);
#20203=EDGE_CURVE('',#15788,#15791,#8931,.T.);
#20204=EDGE_CURVE('',#15791,#15792,#12770,.T.);
#20205=EDGE_CURVE('',#15778,#15792,#8932,.T.);
#20206=EDGE_CURVE('',#15791,#15768,#8933,.T.);
#20207=EDGE_CURVE('',#15791,#15793,#1914,.T.);
#20208=EDGE_CURVE('',#15793,#15794,#660,.T.);
#20209=EDGE_CURVE('',#15792,#15794,#1915,.T.);
#20210=EDGE_CURVE('',#15795,#15768,#12771,.T.);
#20211=EDGE_CURVE('',#15796,#15795,#661,.T.);
#20212=EDGE_CURVE('',#15796,#15797,#8934,.T.);
#20213=EDGE_CURVE('',#15798,#15797,#1916,.T.);
#20214=EDGE_CURVE('',#15798,#15793,#8935,.T.);
#20215=EDGE_CURVE('',#15799,#15666,#12772,.T.);
#20216=EDGE_CURVE('',#15800,#15665,#12773,.T.);
#20217=EDGE_CURVE('',#15799,#15800,#8936,.T.);
#20218=EDGE_CURVE('',#15799,#15668,#12774,.T.);
#20219=EDGE_CURVE('',#15801,#15671,#12775,.T.);
#20220=EDGE_CURVE('',#15796,#15799,#12776,.T.);
#20221=EDGE_CURVE('',#15795,#15802,#1917,.T.);
#20222=EDGE_CURVE('',#15802,#15803,#1918,.T.);
#20223=EDGE_CURVE('',#15803,#15801,#12777,.T.);
#20224=EDGE_CURVE('',#15801,#15804,#12778,.T.);
#20225=EDGE_CURVE('',#15804,#15672,#12779,.T.);
#20226=EDGE_CURVE('',#15804,#15805,#8937,.T.);
#20227=EDGE_CURVE('',#15805,#15675,#12780,.T.);
#20228=EDGE_CURVE('',#15800,#15676,#12781,.T.);
#20229=EDGE_CURVE('',#15805,#15806,#12782,.T.);
#20230=EDGE_CURVE('',#15806,#15678,#12783,.T.);
#20231=EDGE_CURVE('',#15800,#15797,#12784,.T.);
#20232=EDGE_CURVE('',#15806,#15798,#12785,.T.);
#20233=EDGE_CURVE('',#15766,#15802,#12786,.T.);
#20234=EDGE_CURVE('',#15807,#15680,#8938,.T.);
#20235=EDGE_CURVE('',#15807,#15808,#8939,.T.);
#20236=EDGE_CURVE('',#15681,#15808,#8940,.T.);
#20237=EDGE_CURVE('',#15685,#15761,#8941,.T.);
#20238=EDGE_CURVE('',#15686,#15771,#8942,.T.);
#20239=EDGE_CURVE('',#15809,#15771,#12787,.T.);
#20240=EDGE_CURVE('',#15688,#15809,#8943,.T.);
#20241=EDGE_CURVE('',#15809,#15810,#8944,.T.);
#20242=EDGE_CURVE('',#15810,#15690,#8945,.T.);
#20243=EDGE_CURVE('',#15810,#15811,#12788,.T.);
#20244=EDGE_CURVE('',#15811,#15692,#8946,.T.);
#20245=EDGE_CURVE('',#15811,#15617,#12789,.T.);
#20246=EDGE_CURVE('',#15694,#15617,#8947,.T.);
#20247=EDGE_CURVE('',#15696,#15740,#8948,.T.);
#20248=EDGE_CURVE('',#15698,#15616,#8949,.T.);
#20249=EDGE_CURVE('',#15699,#15744,#8950,.T.);
#20250=EDGE_CURVE('',#15700,#15743,#8951,.T.);
#20251=EDGE_CURVE('',#15705,#15745,#8952,.T.);
#20252=EDGE_CURVE('',#15709,#15746,#8953,.T.);
#20253=EDGE_CURVE('',#15711,#15748,#8954,.T.);
#20254=EDGE_CURVE('',#15713,#15749,#8955,.T.);
#20255=EDGE_CURVE('',#15720,#15752,#8956,.T.);
#20256=EDGE_CURVE('',#15750,#15721,#8957,.T.);
#20257=EDGE_CURVE('',#15738,#15724,#8958,.T.);
#20258=EDGE_CURVE('',#15737,#15726,#8959,.T.);
#20259=EDGE_CURVE('',#15737,#15812,#12790,.T.);
#20260=EDGE_CURVE('',#15812,#15728,#8960,.T.);
#20261=EDGE_CURVE('',#15812,#15813,#12791,.T.);
#20262=EDGE_CURVE('',#15813,#15730,#8961,.T.);
#20263=EDGE_CURVE('',#15732,#15814,#8962,.T.);
#20264=EDGE_CURVE('',#15752,#15814,#12792,.T.);
#20265=EDGE_CURVE('',#15813,#15815,#12793,.T.);
#20266=EDGE_CURVE('',#15815,#15734,#8963,.T.);
#20267=EDGE_CURVE('',#15815,#15814,#8964,.T.);
#20268=EDGE_CURVE('',#15736,#15812,#12794,.T.);
#20269=EDGE_CURVE('',#15736,#15816,#12795,.T.);
#20270=EDGE_CURVE('',#15816,#15813,#1919,.T.);
#20271=EDGE_CURVE('',#15814,#15751,#12796,.T.);
#20272=EDGE_CURVE('',#15816,#15815,#12797,.T.);
#20273=EDGE_CURVE('',#15816,#15751,#8965,.T.);
#20274=EDGE_CURVE('',#15770,#15817,#8966,.T.);
#20275=EDGE_CURVE('',#15817,#15618,#12798,.T.);
#20276=EDGE_CURVE('',#15818,#15808,#12799,.T.);
#20277=EDGE_CURVE('',#15808,#15819,#12800,.T.);
#20278=EDGE_CURVE('',#15818,#15819,#12801,.T.);
#20279=EDGE_CURVE('',#15753,#15818,#8967,.T.);
#20280=EDGE_CURVE('',#15786,#15787,#12802,.T.);
#20281=EDGE_CURVE('',#15809,#15770,#12803,.T.);
#20282=EDGE_CURVE('',#15817,#15811,#1920,.T.);
#20283=EDGE_CURVE('',#15807,#15763,#662,.T.);
#20284=EDGE_CURVE('',#15765,#15807,#1921,.T.);
#20285=EDGE_CURVE('',#15817,#15810,#1922,.T.);
#20286=EDGE_CURVE('',#15765,#15819,#8968,.T.);
#20287=EDGE_CURVE('',#15820,#15790,#12804,.T.);
#20288=EDGE_CURVE('',#15767,#15820,#12805,.T.);
#20289=EDGE_CURVE('',#15821,#15822,#12806,.T.);
#20290=EDGE_CURVE('',#15822,#15823,#12807,.T.);
#20291=EDGE_CURVE('',#15821,#15823,#12808,.T.);
#20292=EDGE_CURVE('',#15755,#15822,#8969,.T.);
#20293=EDGE_CURVE('',#15759,#15821,#8970,.T.);
#20294=EDGE_CURVE('',#15818,#15822,#12809,.T.);
#20295=EDGE_CURVE('',#15819,#15823,#12810,.T.);
#20296=EDGE_CURVE('',#15824,#15560,#12811,.T.);
#20297=EDGE_CURVE('',#15825,#15566,#12812,.T.);
#20298=EDGE_CURVE('',#15824,#15825,#8971,.T.);
#20299=EDGE_CURVE('',#15826,#15567,#12813,.T.);
#20300=EDGE_CURVE('',#15826,#15824,#12814,.T.);
#20301=EDGE_CURVE('',#15827,#15569,#12815,.T.);
#20302=EDGE_CURVE('',#15827,#15826,#12816,.T.);
#20303=EDGE_CURVE('',#15828,#15571,#12817,.T.);
#20304=EDGE_CURVE('',#15828,#15827,#12818,.T.);
#20305=EDGE_CURVE('',#15829,#15573,#12819,.T.);
#20306=EDGE_CURVE('',#15829,#15828,#8972,.T.);
#20307=EDGE_CURVE('',#15830,#15566,#12820,.T.);
#20308=EDGE_CURVE('',#15825,#15830,#12821,.T.);
#20309=EDGE_CURVE('',#15825,#15831,#12822,.T.);
#20310=EDGE_CURVE('',#15830,#15832,#12823,.T.);
#20311=EDGE_CURVE('',#15833,#15832,#1923,.T.);
#20312=EDGE_CURVE('',#15825,#15833,#12824,.T.);
#20313=EDGE_CURVE('',#15576,#15829,#12825,.T.);
#20314=EDGE_CURVE('',#15834,#15576,#12826,.T.);
#20315=EDGE_CURVE('',#15835,#15829,#12827,.T.);
#20316=EDGE_CURVE('',#15834,#15835,#1924,.T.);
#20317=EDGE_CURVE('',#15830,#15623,#8973,.T.);
#20318=EDGE_CURVE('',#15832,#15626,#8974,.T.);
#20319=EDGE_CURVE('',#15585,#15834,#8975,.T.);
#20320=EDGE_CURVE('',#15836,#15757,#8976,.T.);
#20321=EDGE_CURVE('',#15836,#15832,#12828,.T.);
#20322=EDGE_CURVE('',#15833,#15836,#12829,.T.);
#20323=EDGE_CURVE('',#15821,#15836,#8977,.T.);
#20324=EDGE_CURVE('',#15823,#15833,#8978,.T.);
#20325=EDGE_CURVE('',#15759,#15757,#8979,.T.);
#20326=EDGE_CURVE('',#15760,#15758,#8980,.T.);
#20327=EDGE_CURVE('',#15837,#15513,#663,.T.);
#20328=EDGE_CURVE('',#15837,#15514,#1925,.T.);
#20329=EDGE_CURVE('',#15667,#15838,#12830,.T.);
#20330=EDGE_CURVE('',#15837,#15838,#8981,.T.);
#20331=EDGE_CURVE('',#15669,#15839,#12831,.T.);
#20332=EDGE_CURVE('',#15838,#15839,#12832,.T.);
#20333=EDGE_CURVE('',#15670,#15840,#12833,.T.);
#20334=EDGE_CURVE('',#15839,#15840,#12834,.T.);
#20335=EDGE_CURVE('',#15673,#15841,#12835,.T.);
#20336=EDGE_CURVE('',#15840,#15841,#12836,.T.);
#20337=EDGE_CURVE('',#15674,#15842,#12837,.T.);
#20338=EDGE_CURVE('',#15841,#15842,#8982,.T.);
#20339=EDGE_CURVE('',#15843,#15663,#12838,.T.);
#20340=EDGE_CURVE('',#15677,#15843,#1926,.T.);
#20341=EDGE_CURVE('',#15844,#15843,#12839,.T.);
#20342=EDGE_CURVE('',#15677,#15844,#12840,.T.);
#20343=EDGE_CURVE('',#15679,#15845,#12841,.T.);
#20344=EDGE_CURVE('',#15842,#15845,#12842,.T.);
#20345=EDGE_CURVE('',#15845,#15844,#12843,.T.);
#20346=EDGE_CURVE('',#15846,#15515,#12844,.T.);
#20347=EDGE_CURVE('',#15846,#15837,#12845,.T.);
#20348=EDGE_CURVE('',#15847,#15520,#12846,.T.);
#20349=EDGE_CURVE('',#15847,#15846,#12847,.T.);
#20350=EDGE_CURVE('',#15848,#15849,#664,.T.);
#20351=EDGE_CURVE('',#15849,#15640,#665,.T.);
#20352=EDGE_CURVE('',#15848,#15639,#666,.T.);
#20353=EDGE_CURVE('',#15542,#15848,#1927,.T.);
#20354=EDGE_CURVE('',#15543,#15850,#12848,.T.);
#20355=EDGE_CURVE('',#15850,#15849,#8983,.T.);
#20356=EDGE_CURVE('',#15851,#15563,#1928,.T.);
#20357=EDGE_CURVE('',#15851,#15641,#667,.T.);
#20358=EDGE_CURVE('',#15624,#15851,#8984,.T.);
#20359=EDGE_CURVE('',#15852,#15661,#1929,.T.);
#20360=EDGE_CURVE('',#15853,#15662,#1930,.T.);
#20361=EDGE_CURVE('',#15852,#15853,#668,.T.);
#20362=EDGE_CURVE('',#15843,#15852,#8985,.T.);
#20363=EDGE_CURVE('',#15849,#15851,#12849,.T.);
#20364=EDGE_CURVE('',#15854,#15524,#1931,.T.);
#20365=EDGE_CURVE('',#15855,#15526,#1932,.T.);
#20366=EDGE_CURVE('',#15855,#15854,#12850,.T.);
#20367=EDGE_CURVE('',#15538,#15856,#669,.T.);
#20368=EDGE_CURVE('',#15856,#15857,#1933,.T.);
#20369=EDGE_CURVE('',#15539,#15857,#1934,.T.);
#20370=EDGE_CURVE('',#15857,#15850,#12851,.T.);
#20371=EDGE_CURVE('',#15856,#15858,#12852,.T.);
#20372=EDGE_CURVE('',#15858,#15859,#12853,.T.);
#20373=EDGE_CURVE('',#15850,#15859,#12854,.T.);
#20374=EDGE_CURVE('',#15858,#15860,#12855,.T.);
#20375=EDGE_CURVE('',#15860,#15861,#12856,.T.);
#20376=EDGE_CURVE('',#15859,#15861,#12857,.T.);
#20377=EDGE_CURVE('',#15860,#15862,#8986,.T.);
#20378=EDGE_CURVE('',#15862,#15863,#12858,.T.);
#20379=EDGE_CURVE('',#15861,#15863,#8987,.T.);
#20380=EDGE_CURVE('',#15862,#15864,#12859,.T.);
#20381=EDGE_CURVE('',#15864,#15865,#12860,.T.);
#20382=EDGE_CURVE('',#15863,#15865,#12861,.T.);
#20383=EDGE_CURVE('',#15864,#15866,#12862,.T.);
#20384=EDGE_CURVE('',#15866,#15867,#12863,.T.);
#20385=EDGE_CURVE('',#15865,#15867,#12864,.T.);
#20386=EDGE_CURVE('',#15866,#15868,#12865,.T.);
#20387=EDGE_CURVE('',#15868,#15869,#12866,.T.);
#20388=EDGE_CURVE('',#15867,#15869,#12867,.T.);
#20389=EDGE_CURVE('',#15870,#15518,#670,.T.);
#20390=EDGE_CURVE('',#15870,#15847,#671,.T.);
#20391=EDGE_CURVE('',#15521,#15870,#1935,.T.);
#20392=EDGE_CURVE('',#15869,#15847,#8988,.T.);
#20393=EDGE_CURVE('',#15868,#15521,#8989,.T.);
#20394=EDGE_CURVE('',#15551,#15871,#8990,.T.);
#20395=EDGE_CURVE('',#15871,#15872,#12868,.T.);
#20396=EDGE_CURVE('',#15872,#15855,#8991,.T.);
#20397=EDGE_CURVE('',#15872,#15873,#12869,.T.);
#20398=EDGE_CURVE('',#15873,#15854,#8992,.T.);
#20399=EDGE_CURVE('',#15873,#15530,#12870,.T.);
#20400=EDGE_CURVE('',#15537,#15874,#12871,.T.);
#20401=EDGE_CURVE('',#15874,#15856,#8993,.T.);
#20402=EDGE_CURVE('',#15874,#15875,#12872,.T.);
#20403=EDGE_CURVE('',#15858,#15875,#8994,.T.);
#20404=EDGE_CURVE('',#15876,#15875,#12873,.T.);
#20405=EDGE_CURVE('',#15860,#15876,#8995,.T.);
#20406=EDGE_CURVE('',#15876,#15877,#8996,.T.);
#20407=EDGE_CURVE('',#15862,#15877,#8997,.T.);
#20408=EDGE_CURVE('',#15878,#15877,#12874,.T.);
#20409=EDGE_CURVE('',#15864,#15878,#8998,.T.);
#20410=EDGE_CURVE('',#15878,#15879,#12875,.T.);
#20411=EDGE_CURVE('',#15866,#15879,#8999,.T.);
#20412=EDGE_CURVE('',#15880,#15879,#12876,.T.);
#20413=EDGE_CURVE('',#15868,#15880,#9000,.T.);
#20414=EDGE_CURVE('',#15880,#15881,#9001,.T.);
#20415=EDGE_CURVE('',#15549,#15881,#9002,.T.);
#20416=EDGE_CURVE('',#15881,#15871,#12877,.T.);
#20417=EDGE_CURVE('',#15882,#15871,#12878,.T.);
#20418=EDGE_CURVE('',#15882,#15881,#12879,.T.);
#20419=EDGE_CURVE('',#15882,#15883,#12880,.T.);
#20420=EDGE_CURVE('',#15872,#15883,#12881,.T.);
#20421=EDGE_CURVE('',#15883,#15884,#12882,.T.);
#20422=EDGE_CURVE('',#15873,#15884,#12883,.T.);
#20423=EDGE_CURVE('',#15530,#15885,#12884,.T.);
#20424=EDGE_CURVE('',#15528,#15885,#12885,.T.);
#20425=EDGE_CURVE('',#15884,#15885,#12886,.T.);
#20426=EDGE_CURVE('',#15537,#15886,#12887,.T.);
#20427=EDGE_CURVE('',#15886,#15874,#12888,.T.);
#20428=EDGE_CURVE('',#15886,#15887,#12889,.T.);
#20429=EDGE_CURVE('',#15875,#15887,#1936,.T.);
#20430=EDGE_CURVE('',#15876,#15887,#12890,.T.);
#20431=EDGE_CURVE('',#15887,#15888,#9003,.T.);
#20432=EDGE_CURVE('',#15877,#15888,#1937,.T.);
#20433=EDGE_CURVE('',#15878,#15888,#12891,.T.);
#20434=EDGE_CURVE('',#15888,#15889,#12892,.T.);
#20435=EDGE_CURVE('',#15879,#15889,#1938,.T.);
#20436=EDGE_CURVE('',#15880,#15889,#12893,.T.);
#20437=EDGE_CURVE('',#15889,#15882,#9004,.T.);
#20438=EDGE_CURVE('',#15885,#15890,#9005,.T.);
#20439=EDGE_CURVE('',#15531,#15890,#12894,.T.);
#20440=EDGE_CURVE('',#15890,#15891,#12895,.T.);
#20441=EDGE_CURVE('',#15533,#15891,#12896,.T.);
#20442=EDGE_CURVE('',#15891,#15892,#12897,.T.);
#20443=EDGE_CURVE('',#15535,#15892,#12898,.T.);
#20444=EDGE_CURVE('',#15892,#15886,#12899,.T.);
#20445=EDGE_CURVE('',#15893,#15894,#9006,.T.);
#20446=EDGE_CURVE('',#15895,#15894,#12900,.T.);
#20447=EDGE_CURVE('',#15896,#15895,#9007,.T.);
#20448=EDGE_CURVE('',#15896,#15897,#12901,.T.);
#20449=EDGE_CURVE('',#15897,#15893,#1939,.T.);
#20450=EDGE_CURVE('',#15898,#15899,#672,.T.);
#20451=EDGE_CURVE('',#15899,#15896,#12902,.T.);
#20452=EDGE_CURVE('',#15900,#15895,#12903,.T.);
#20453=EDGE_CURVE('',#15898,#15900,#9008,.T.);
#20454=EDGE_CURVE('',#15901,#15900,#12904,.T.);
#20455=EDGE_CURVE('',#15902,#15901,#9009,.T.);
#20456=EDGE_CURVE('',#15902,#15898,#1940,.T.);
#20457=EDGE_CURVE('',#15903,#15904,#1941,.T.);
#20458=EDGE_CURVE('',#15905,#15903,#9010,.T.);
#20459=EDGE_CURVE('',#15906,#15905,#12905,.T.);
#20460=EDGE_CURVE('',#15906,#15904,#9011,.T.);
#20461=EDGE_CURVE('',#15907,#15908,#1942,.T.);
#20462=EDGE_CURVE('',#15909,#15907,#9012,.T.);
#20463=EDGE_CURVE('',#15910,#15909,#12906,.T.);
#20464=EDGE_CURVE('',#15910,#15908,#9013,.T.);
#20465=EDGE_CURVE('',#15908,#15911,#9014,.T.);
#20466=EDGE_CURVE('',#15912,#15910,#9015,.T.);
#20467=EDGE_CURVE('',#15911,#15912,#9016,.T.);
#20468=EDGE_CURVE('',#15913,#15912,#12907,.T.);
#20469=EDGE_CURVE('',#15914,#15913,#9017,.T.);
#20470=EDGE_CURVE('',#15911,#15914,#12908,.T.);
#20471=EDGE_CURVE('',#15914,#15915,#12909,.T.);
#20472=EDGE_CURVE('',#15916,#15913,#12910,.T.);
#20473=EDGE_CURVE('',#15915,#15916,#9018,.T.);
#20474=EDGE_CURVE('',#15917,#15916,#12911,.T.);
#20475=EDGE_CURVE('',#15918,#15917,#9019,.T.);
#20476=EDGE_CURVE('',#15919,#15918,#1943,.T.);
#20477=EDGE_CURVE('',#15920,#15919,#9020,.T.);
#20478=EDGE_CURVE('',#15915,#15920,#12912,.T.);
#20479=EDGE_CURVE('',#15921,#15922,#9021,.T.);
#20480=EDGE_CURVE('',#15918,#15921,#12913,.T.);
#20481=EDGE_CURVE('',#15923,#15917,#9022,.T.);
#20482=EDGE_CURVE('',#15923,#15922,#9023,.T.);
#20483=EDGE_CURVE('',#15924,#15925,#9024,.T.);
#20484=EDGE_CURVE('',#15924,#15894,#12914,.T.);
#20485=EDGE_CURVE('',#15894,#15926,#9025,.T.);
#20486=EDGE_CURVE('',#15926,#15925,#12915,.T.);
#20487=EDGE_CURVE('',#15924,#15895,#12916,.T.);
#20488=EDGE_CURVE('',#15927,#15900,#12917,.T.);
#20489=EDGE_CURVE('',#15927,#15924,#12918,.T.);
#20490=EDGE_CURVE('',#15927,#15901,#12919,.T.);
#20491=EDGE_CURVE('',#15928,#15929,#12920,.T.);
#20492=EDGE_CURVE('',#15929,#15901,#9026,.T.);
#20493=EDGE_CURVE('',#15928,#15927,#9027,.T.);
#20494=EDGE_CURVE('',#15930,#15931,#12921,.T.);
#20495=EDGE_CURVE('',#15931,#15929,#12922,.T.);
#20496=EDGE_CURVE('',#15930,#15928,#12923,.T.);
#20497=EDGE_CURVE('',#15932,#15905,#12924,.T.);
#20498=EDGE_CURVE('',#15905,#15931,#12925,.T.);
#20499=EDGE_CURVE('',#15932,#15930,#12926,.T.);
#20500=EDGE_CURVE('',#15933,#15906,#12927,.T.);
#20501=EDGE_CURVE('',#15933,#15932,#12928,.T.);
#20502=EDGE_CURVE('',#15934,#15909,#12929,.T.);
#20503=EDGE_CURVE('',#15909,#15906,#12930,.T.);
#20504=EDGE_CURVE('',#15934,#15933,#12931,.T.);
#20505=EDGE_CURVE('',#15935,#15910,#12932,.T.);
#20506=EDGE_CURVE('',#15935,#15934,#12933,.T.);
#20507=EDGE_CURVE('',#15936,#15912,#12934,.T.);
#20508=EDGE_CURVE('',#15936,#15935,#9028,.T.);
#20509=EDGE_CURVE('',#15936,#15913,#12935,.T.);
#20510=EDGE_CURVE('',#15937,#15916,#12936,.T.);
#20511=EDGE_CURVE('',#15937,#15936,#12937,.T.);
#20512=EDGE_CURVE('',#15937,#15917,#12938,.T.);
#20513=EDGE_CURVE('',#15938,#15937,#9029,.T.);
#20514=EDGE_CURVE('',#15938,#15923,#12939,.T.);
#20515=EDGE_CURVE('',#15925,#15939,#12940,.T.);
#20516=EDGE_CURVE('',#15939,#15938,#12941,.T.);
#20517=EDGE_CURVE('',#15940,#15941,#9030,.T.);
#20518=EDGE_CURVE('',#15941,#15942,#9031,.T.);
#20519=EDGE_CURVE('',#15942,#15943,#1944,.T.);
#20520=EDGE_CURVE('',#15943,#15944,#9032,.T.);
#20521=EDGE_CURVE('',#15944,#15945,#9033,.T.);
#20522=EDGE_CURVE('',#15946,#15945,#9034,.T.);
#20523=EDGE_CURVE('',#15940,#15946,#9035,.T.);
#20524=EDGE_CURVE('',#15947,#15946,#12942,.T.);
#20525=EDGE_CURVE('',#15948,#15947,#9036,.T.);
#20526=EDGE_CURVE('',#15948,#15940,#12943,.T.);
#20527=EDGE_CURVE('',#15949,#15948,#12944,.T.);
#20528=EDGE_CURVE('',#15950,#15947,#12945,.T.);
#20529=EDGE_CURVE('',#15949,#15950,#9037,.T.);
#20530=EDGE_CURVE('',#15951,#15950,#12946,.T.);
#20531=EDGE_CURVE('',#15952,#15951,#9038,.T.);
#20532=EDGE_CURVE('',#15952,#15949,#12947,.T.);
#20533=EDGE_CURVE('',#15953,#15951,#9039,.T.);
#20534=EDGE_CURVE('',#15953,#15954,#9040,.T.);
#20535=EDGE_CURVE('',#15954,#15952,#9041,.T.);
#20536=EDGE_CURVE('',#15955,#15954,#12948,.T.);
#20537=EDGE_CURVE('',#15956,#15953,#12949,.T.);
#20538=EDGE_CURVE('',#15956,#15955,#9042,.T.);
#20539=EDGE_CURVE('',#15957,#15958,#9043,.T.);
#20540=EDGE_CURVE('',#15945,#15958,#12950,.T.);
#20541=EDGE_CURVE('',#15957,#15944,#12951,.T.);
#20542=EDGE_CURVE('',#15959,#15946,#12952,.T.);
#20543=EDGE_CURVE('',#15960,#15945,#12953,.T.);
#20544=EDGE_CURVE('',#15959,#15960,#9044,.T.);
#20545=EDGE_CURVE('',#15959,#15947,#12954,.T.);
#20546=EDGE_CURVE('',#15961,#15950,#12955,.T.);
#20547=EDGE_CURVE('',#15961,#15959,#12956,.T.);
#20548=EDGE_CURVE('',#15961,#15951,#12957,.T.);
#20549=EDGE_CURVE('',#15962,#15953,#12958,.T.);
#20550=EDGE_CURVE('',#15962,#15961,#9045,.T.);
#20551=EDGE_CURVE('',#15963,#15956,#12959,.T.);
#20552=EDGE_CURVE('',#15963,#15962,#12960,.T.);
#20553=EDGE_CURVE('',#15585,#15964,#12961,.T.);
#20554=EDGE_CURVE('',#15584,#15964,#1945,.T.);
#20555=EDGE_CURVE('',#15964,#15956,#12962,.T.);
#20556=EDGE_CURVE('',#15584,#15963,#12963,.T.);
#20557=EDGE_CURVE('',#15960,#15958,#12964,.T.);
#20558=EDGE_CURVE('',#15586,#15965,#1946,.T.);
#20559=EDGE_CURVE('',#15587,#15965,#12965,.T.);
#20560=EDGE_CURVE('',#15960,#15586,#12966,.T.);
#20561=EDGE_CURVE('',#15958,#15965,#12967,.T.);
#20562=EDGE_CURVE('',#15966,#15967,#12968,.T.);
#20563=EDGE_CURVE('',#15968,#15967,#9046,.T.);
#20564=EDGE_CURVE('',#15968,#15969,#1947,.T.);
#20565=EDGE_CURVE('',#15969,#15966,#9047,.T.);
#20566=EDGE_CURVE('',#15970,#15967,#1948,.T.);
#20567=EDGE_CURVE('',#15970,#15971,#12969,.T.);
#20568=EDGE_CURVE('',#15971,#15972,#12970,.T.);
#20569=EDGE_CURVE('',#15967,#15972,#12971,.T.);
#20570=EDGE_CURVE('',#15973,#15972,#1949,.T.);
#20571=EDGE_CURVE('',#15973,#15974,#9048,.T.);
#20572=EDGE_CURVE('',#15975,#15974,#1950,.T.);
#20573=EDGE_CURVE('',#15972,#15975,#9049,.T.);
#20574=EDGE_CURVE('',#15968,#15976,#1951,.T.);
#20575=EDGE_CURVE('',#15975,#15968,#12972,.T.);
#20576=EDGE_CURVE('',#15975,#15977,#12973,.T.);
#20577=EDGE_CURVE('',#15977,#15976,#12974,.T.);
#20578=EDGE_CURVE('',#15976,#15969,#12975,.T.);
#20579=EDGE_CURVE('',#15978,#15966,#9050,.T.);
#20580=EDGE_CURVE('',#15969,#15979,#9051,.T.);
#20581=EDGE_CURVE('',#15979,#15978,#9052,.T.);
#20582=EDGE_CURVE('',#15970,#15966,#12976,.T.);
#20583=EDGE_CURVE('',#15980,#15971,#9053,.T.);
#20584=EDGE_CURVE('',#15981,#15970,#9054,.T.);
#20585=EDGE_CURVE('',#15981,#15980,#12977,.T.);
#20586=EDGE_CURVE('',#15973,#15971,#12978,.T.);
#20587=EDGE_CURVE('',#15982,#15983,#9055,.T.);
#20588=EDGE_CURVE('',#15974,#15983,#9056,.T.);
#20589=EDGE_CURVE('',#15982,#15973,#9057,.T.);
#20590=EDGE_CURVE('',#15974,#15977,#12979,.T.);
#20591=EDGE_CURVE('',#15984,#15985,#12980,.T.);
#20592=EDGE_CURVE('',#15976,#15985,#9058,.T.);
#20593=EDGE_CURVE('',#15977,#15984,#9059,.T.);
#20594=EDGE_CURVE('',#15985,#15979,#12981,.T.);
#20595=EDGE_CURVE('',#15979,#15986,#12982,.T.);
#20596=EDGE_CURVE('',#15986,#15987,#9060,.T.);
#20597=EDGE_CURVE('',#15978,#15987,#12983,.T.);
#20598=EDGE_CURVE('',#15978,#15981,#12984,.T.);
#20599=EDGE_CURVE('',#15981,#15988,#12985,.T.);
#20600=EDGE_CURVE('',#15988,#15989,#12986,.T.);
#20601=EDGE_CURVE('',#15980,#15989,#12987,.T.);
#20602=EDGE_CURVE('',#15980,#15982,#12988,.T.);
#20603=EDGE_CURVE('',#15982,#15990,#12989,.T.);
#20604=EDGE_CURVE('',#15990,#15991,#9061,.T.);
#20605=EDGE_CURVE('',#15983,#15991,#12990,.T.);
#20606=EDGE_CURVE('',#15983,#15984,#12991,.T.);
#20607=EDGE_CURVE('',#15984,#15992,#12992,.T.);
#20608=EDGE_CURVE('',#15992,#15993,#12993,.T.);
#20609=EDGE_CURVE('',#15985,#15993,#12994,.T.);
#20610=EDGE_CURVE('',#15993,#15986,#12995,.T.);
#20611=EDGE_CURVE('',#15994,#15995,#12996,.T.);
#20612=EDGE_CURVE('',#15996,#15995,#12997,.T.);
#20613=EDGE_CURVE('',#15994,#15996,#12998,.T.);
#20614=EDGE_CURVE('',#15987,#15988,#12999,.T.);
#20615=EDGE_CURVE('',#15989,#15990,#13000,.T.);
#20616=EDGE_CURVE('',#15991,#15992,#13001,.T.);
#20617=EDGE_CURVE('',#15997,#15619,#13002,.T.);
#20618=EDGE_CURVE('',#15997,#15620,#1952,.T.);
#20619=EDGE_CURVE('',#15998,#15620,#13003,.T.);
#20620=EDGE_CURVE('',#15999,#15998,#13004,.T.);
#20621=EDGE_CURVE('',#15999,#15997,#13005,.T.);
#20622=EDGE_CURVE('',#16000,#16001,#1953,.T.);
#20623=EDGE_CURVE('',#16001,#15943,#673,.T.);
#20624=EDGE_CURVE('',#16000,#15942,#1954,.T.);
#20625=EDGE_CURVE('',#16002,#16000,#13006,.T.);
#20626=EDGE_CURVE('',#16002,#16003,#13007,.T.);
#20627=EDGE_CURVE('',#16003,#16001,#13008,.T.);
#20628=EDGE_CURVE('',#15628,#16004,#13009,.T.);
#20629=EDGE_CURVE('',#16004,#16005,#9062,.T.);
#20630=EDGE_CURVE('',#16005,#15629,#13010,.T.);
#20631=EDGE_CURVE('',#16006,#16007,#9063,.T.);
#20632=EDGE_CURVE('',#16007,#16005,#9064,.T.);
#20633=EDGE_CURVE('',#16004,#16006,#9065,.T.);
#20634=EDGE_CURVE('',#15965,#16008,#9066,.T.);
#20635=EDGE_CURVE('',#15631,#16008,#13011,.T.);
#20636=EDGE_CURVE('',#16009,#15957,#1955,.T.);
#20637=EDGE_CURVE('',#16010,#16009,#13012,.T.);
#20638=EDGE_CURVE('',#16011,#16010,#674,.T.);
#20639=EDGE_CURVE('',#16012,#16011,#9067,.T.);
#20640=EDGE_CURVE('',#16013,#16012,#13013,.T.);
#20641=EDGE_CURVE('',#16014,#16013,#9068,.T.);
#20642=EDGE_CURVE('',#16015,#16014,#1956,.T.);
#20643=EDGE_CURVE('',#16016,#16015,#13014,.T.);
#20644=EDGE_CURVE('',#16017,#16016,#1957,.T.);
#20645=EDGE_CURVE('',#16018,#16017,#9069,.T.);
#20646=EDGE_CURVE('',#16008,#16018,#13015,.T.);
#20647=EDGE_CURVE('',#16019,#15642,#13016,.T.);
#20648=EDGE_CURVE('',#15646,#16020,#13017,.T.);
#20649=EDGE_CURVE('',#16019,#16020,#9070,.T.);
#20650=EDGE_CURVE('',#16020,#16021,#9071,.T.);
#20651=EDGE_CURVE('',#16021,#16022,#675,.T.);
#20652=EDGE_CURVE('',#16023,#16022,#9072,.T.);
#20653=EDGE_CURVE('',#16023,#16019,#9073,.T.);
#20654=EDGE_CURVE('',#16024,#16023,#13018,.T.);
#20655=EDGE_CURVE('',#16022,#16025,#1958,.T.);
#20656=EDGE_CURVE('',#16024,#16025,#9074,.T.);
#20657=EDGE_CURVE('',#16025,#16026,#676,.T.);
#20658=EDGE_CURVE('',#16026,#16027,#9075,.T.);
#20659=EDGE_CURVE('',#16027,#16028,#677,.T.);
#20660=EDGE_CURVE('',#16029,#16028,#9076,.T.);
#20661=EDGE_CURVE('',#16029,#16024,#9077,.T.);
#20662=EDGE_CURVE('',#16030,#16029,#13019,.T.);
#20663=EDGE_CURVE('',#16028,#16031,#1959,.T.);
#20664=EDGE_CURVE('',#16030,#16031,#9078,.T.);
#20665=EDGE_CURVE('',#16031,#16032,#1960,.T.);
#20666=EDGE_CURVE('',#16032,#16033,#1961,.T.);
#20667=EDGE_CURVE('',#16033,#16034,#9079,.T.);
#20668=EDGE_CURVE('',#16035,#16034,#9080,.T.);
#20669=EDGE_CURVE('',#16035,#16030,#9081,.T.);
#20670=EDGE_CURVE('',#16006,#16035,#13020,.T.);
#20671=EDGE_CURVE('',#16034,#16007,#13021,.T.);
#20672=EDGE_CURVE('',#15926,#16036,#13022,.T.);
#20673=EDGE_CURVE('',#15925,#16036,#13023,.T.);
#20674=EDGE_CURVE('',#16036,#16037,#13024,.T.);
#20675=EDGE_CURVE('',#15939,#16037,#13025,.T.);
#20676=EDGE_CURVE('',#16038,#16039,#13026,.T.);
#20677=EDGE_CURVE('',#16038,#16037,#9082,.T.);
#20678=EDGE_CURVE('',#16040,#16036,#9083,.T.);
#20679=EDGE_CURVE('',#16041,#16040,#1962,.T.);
#20680=EDGE_CURVE('',#16041,#15853,#13027,.T.);
#20681=EDGE_CURVE('',#15794,#16042,#13028,.T.);
#20682=EDGE_CURVE('',#16043,#16042,#1963,.T.);
#20683=EDGE_CURVE('',#16039,#16043,#9084,.T.);
#20684=EDGE_CURVE('',#16044,#16040,#13029,.T.);
#20685=EDGE_CURVE('',#16044,#15926,#9085,.T.);
#20686=EDGE_CURVE('',#15893,#16045,#9086,.T.);
#20687=EDGE_CURVE('',#16046,#16045,#9087,.T.);
#20688=EDGE_CURVE('',#16046,#16047,#9088,.T.);
#20689=EDGE_CURVE('',#16047,#16048,#9089,.T.);
#20690=EDGE_CURVE('',#16048,#16049,#13030,.T.);
#20691=EDGE_CURVE('',#16049,#16044,#9090,.T.);
#20692=EDGE_CURVE('',#16045,#16050,#13031,.T.);
#20693=EDGE_CURVE('',#16051,#16050,#9091,.T.);
#20694=EDGE_CURVE('',#16051,#16046,#13032,.T.);
#20695=EDGE_CURVE('',#16052,#16053,#9092,.T.);
#20696=EDGE_CURVE('',#16052,#16051,#13033,.T.);
#20697=EDGE_CURVE('',#16050,#16053,#13034,.T.);
#20698=EDGE_CURVE('',#16053,#16054,#13035,.T.);
#20699=EDGE_CURVE('',#16055,#16054,#9093,.T.);
#20700=EDGE_CURVE('',#16055,#16052,#13036,.T.);
#20701=EDGE_CURVE('',#16056,#16057,#9094,.T.);
#20702=EDGE_CURVE('',#16056,#16055,#9095,.T.);
#20703=EDGE_CURVE('',#16054,#16057,#9096,.T.);
#20704=EDGE_CURVE('',#16058,#16048,#1964,.T.);
#20705=EDGE_CURVE('',#16047,#16059,#13037,.T.);
#20706=EDGE_CURVE('',#16059,#16058,#9097,.T.);
#20707=EDGE_CURVE('',#16057,#16060,#13038,.T.);
#20708=EDGE_CURVE('',#16061,#16060,#9098,.T.);
#20709=EDGE_CURVE('',#16061,#16056,#13039,.T.);
#20710=EDGE_CURVE('',#16060,#16058,#13040,.T.);
#20711=EDGE_CURVE('',#16059,#16061,#13041,.T.);
#20712=EDGE_CURVE('',#16062,#15998,#13042,.T.);
#20713=EDGE_CURVE('',#15998,#16063,#9099,.T.);
#20714=EDGE_CURVE('',#16064,#16063,#13043,.T.);
#20715=EDGE_CURVE('',#16062,#16064,#9100,.T.);
#20716=EDGE_CURVE('',#16065,#16066,#13044,.T.);
#20717=EDGE_CURVE('',#16066,#16067,#13045,.T.);
#20718=EDGE_CURVE('',#16068,#16067,#13046,.T.);
#20719=EDGE_CURVE('',#16065,#16068,#13047,.T.);
#20720=EDGE_CURVE('',#16069,#16070,#13048,.T.);
#20721=EDGE_CURVE('',#16070,#16066,#13049,.T.);
#20722=EDGE_CURVE('',#16069,#16065,#13050,.T.);
#20723=EDGE_CURVE('',#16071,#16072,#13051,.T.);
#20724=EDGE_CURVE('',#16072,#16070,#9101,.T.);
#20725=EDGE_CURVE('',#16071,#16069,#9102,.T.);
#20726=EDGE_CURVE('',#16073,#16074,#13052,.T.);
#20727=EDGE_CURVE('',#16074,#16072,#13053,.T.);
#20728=EDGE_CURVE('',#16073,#16071,#13054,.T.);
#20729=EDGE_CURVE('',#16075,#16076,#13055,.T.);
#20730=EDGE_CURVE('',#16076,#16074,#13056,.T.);
#20731=EDGE_CURVE('',#16075,#16073,#13057,.T.);
#20732=EDGE_CURVE('',#16067,#16077,#13058,.T.);
#20733=EDGE_CURVE('',#16078,#16077,#13059,.T.);
#20734=EDGE_CURVE('',#16068,#16078,#13060,.T.);
#20735=EDGE_CURVE('',#16079,#16080,#13061,.T.);
#20736=EDGE_CURVE('',#16080,#16076,#13062,.T.);
#20737=EDGE_CURVE('',#16079,#16075,#13063,.T.);
#20738=EDGE_CURVE('',#16077,#16080,#9103,.T.);
#20739=EDGE_CURVE('',#16078,#16079,#9104,.T.);
#20740=EDGE_CURVE('',#16081,#16082,#13064,.T.);
#20741=EDGE_CURVE('',#16082,#16083,#13065,.T.);
#20742=EDGE_CURVE('',#16084,#16083,#13066,.T.);
#20743=EDGE_CURVE('',#16081,#16084,#13067,.T.);
#20744=EDGE_CURVE('',#16032,#16085,#678,.T.);
#20745=EDGE_CURVE('',#16085,#16086,#1965,.T.);
#20746=EDGE_CURVE('',#16033,#16086,#679,.T.);
#20747=EDGE_CURVE('',#16087,#16085,#13068,.T.);
#20748=EDGE_CURVE('',#16084,#16087,#13069,.T.);
#20749=EDGE_CURVE('',#16083,#16086,#13070,.T.);
#20750=EDGE_CURVE('',#16027,#16088,#680,.T.);
#20751=EDGE_CURVE('',#16088,#16089,#681,.T.);
#20752=EDGE_CURVE('',#16028,#16089,#682,.T.);
#20753=EDGE_CURVE('',#16089,#16090,#1966,.T.);
#20754=EDGE_CURVE('',#16031,#16090,#683,.T.);
#20755=EDGE_CURVE('',#16090,#16085,#1967,.T.);
#20756=EDGE_CURVE('',#16088,#16091,#13071,.T.);
#20757=EDGE_CURVE('',#16092,#16091,#13072,.T.);
#20758=EDGE_CURVE('',#16087,#16092,#13073,.T.);
#20759=EDGE_CURVE('',#16093,#16094,#13074,.T.);
#20760=EDGE_CURVE('',#16094,#16082,#13075,.T.);
#20761=EDGE_CURVE('',#16093,#16081,#13076,.T.);
#20762=EDGE_CURVE('',#16091,#16095,#13077,.T.);
#20763=EDGE_CURVE('',#16096,#16095,#13078,.T.);
#20764=EDGE_CURVE('',#16092,#16096,#13079,.T.);
#20765=EDGE_CURVE('',#16095,#16094,#9105,.T.);
#20766=EDGE_CURVE('',#16096,#16093,#9106,.T.);
#20767=EDGE_CURVE('',#16021,#16097,#684,.T.);
#20768=EDGE_CURVE('',#16097,#16098,#685,.T.);
#20769=EDGE_CURVE('',#16022,#16098,#686,.T.);
#20770=EDGE_CURVE('',#16098,#16099,#1968,.T.);
#20771=EDGE_CURVE('',#16025,#16099,#687,.T.);
#20772=EDGE_CURVE('',#16099,#16100,#688,.T.);
#20773=EDGE_CURVE('',#16026,#16100,#689,.T.);
#20774=EDGE_CURVE('',#16101,#16097,#13080,.T.);
#20775=EDGE_CURVE('',#16101,#16102,#13081,.T.);
#20776=EDGE_CURVE('',#16102,#16103,#13082,.T.);
#20777=EDGE_CURVE('',#16104,#16103,#13083,.T.);
#20778=EDGE_CURVE('',#16100,#16104,#13084,.T.);
#20779=EDGE_CURVE('',#16105,#16106,#13085,.T.);
#20780=EDGE_CURVE('',#16106,#16102,#13086,.T.);
#20781=EDGE_CURVE('',#16105,#16101,#13087,.T.);
#20782=EDGE_CURVE('',#16107,#16108,#13088,.T.);
#20783=EDGE_CURVE('',#16108,#16106,#9107,.T.);
#20784=EDGE_CURVE('',#16107,#16105,#9108,.T.);
#20785=EDGE_CURVE('',#16109,#16110,#13089,.T.);
#20786=EDGE_CURVE('',#16110,#16108,#13090,.T.);
#20787=EDGE_CURVE('',#16109,#16107,#13091,.T.);
#20788=EDGE_CURVE('',#16111,#16112,#13092,.T.);
#20789=EDGE_CURVE('',#16112,#16110,#13093,.T.);
#20790=EDGE_CURVE('',#16111,#16109,#13094,.T.);
#20791=EDGE_CURVE('',#16103,#16113,#13095,.T.);
#20792=EDGE_CURVE('',#16114,#16113,#13096,.T.);
#20793=EDGE_CURVE('',#16104,#16114,#13097,.T.);
#20794=EDGE_CURVE('',#16115,#16116,#13098,.T.);
#20795=EDGE_CURVE('',#16116,#16112,#13099,.T.);
#20796=EDGE_CURVE('',#16115,#16111,#13100,.T.);
#20797=EDGE_CURVE('',#16113,#16116,#9109,.T.);
#20798=EDGE_CURVE('',#16114,#16115,#9110,.T.);
#20799=EDGE_CURVE('',#16117,#16118,#1969,.T.);
#20800=EDGE_CURVE('',#16118,#16119,#9111,.T.);
#20801=EDGE_CURVE('',#16120,#16119,#1970,.T.);
#20802=EDGE_CURVE('',#16117,#16120,#9112,.T.);
#20803=EDGE_CURVE('',#15994,#16121,#9113,.T.);
#20804=EDGE_CURVE('',#16121,#16122,#13101,.T.);
#20805=EDGE_CURVE('',#15995,#16122,#9114,.T.);
#20806=EDGE_CURVE('',#16123,#16124,#1971,.T.);
#20807=EDGE_CURVE('',#16125,#16123,#13102,.T.);
#20808=EDGE_CURVE('',#16125,#16126,#1972,.T.);
#20809=EDGE_CURVE('',#16126,#16124,#13103,.T.);
#20810=EDGE_CURVE('',#16127,#16126,#13104,.T.);
#20811=EDGE_CURVE('',#16127,#16125,#13105,.T.);
#20812=EDGE_CURVE('',#16128,#16129,#1973,.T.);
#20813=EDGE_CURVE('',#16129,#16126,#13106,.T.);
#20814=EDGE_CURVE('',#16128,#16127,#13107,.T.);
#20815=EDGE_CURVE('',#16130,#16124,#13108,.T.);
#20816=EDGE_CURVE('',#16123,#16130,#13109,.T.);
#20817=EDGE_CURVE('',#16131,#16129,#13110,.T.);
#20818=EDGE_CURVE('',#16131,#16128,#13111,.T.);
#20819=EDGE_CURVE('',#16117,#16132,#13112,.T.);
#20820=EDGE_CURVE('',#16132,#16118,#13113,.T.);
#20821=EDGE_CURVE('',#16124,#16129,#9115,.T.);
#20822=EDGE_CURVE('',#16130,#16131,#9116,.T.);
#20823=EDGE_CURVE('',#16133,#16134,#1974,.T.);
#20824=EDGE_CURVE('',#16133,#16132,#13114,.T.);
#20825=EDGE_CURVE('',#16134,#16117,#13115,.T.);
#20826=EDGE_CURVE('',#16063,#16135,#13116,.T.);
#20827=EDGE_CURVE('',#16136,#16135,#13117,.T.);
#20828=EDGE_CURVE('',#16064,#16136,#13118,.T.);
#20829=EDGE_CURVE('',#16135,#16137,#13119,.T.);
#20830=EDGE_CURVE('',#16138,#16137,#13120,.T.);
#20831=EDGE_CURVE('',#16136,#16138,#13121,.T.);
#20832=EDGE_CURVE('',#16139,#16140,#13122,.T.);
#20833=EDGE_CURVE('',#16140,#16003,#13123,.T.);
#20834=EDGE_CURVE('',#16139,#16002,#13124,.T.);
#20835=EDGE_CURVE('',#16137,#16141,#13125,.T.);
#20836=EDGE_CURVE('',#16142,#16141,#13126,.T.);
#20837=EDGE_CURVE('',#16138,#16142,#13127,.T.);
#20838=EDGE_CURVE('',#16143,#16122,#13128,.T.);
#20839=EDGE_CURVE('',#16143,#16121,#13129,.T.);
#20840=EDGE_CURVE('',#16144,#15762,#13130,.T.);
#20841=EDGE_CURVE('',#16144,#15997,#9117,.T.);
#20842=EDGE_CURVE('',#16145,#15999,#9118,.T.);
#20843=EDGE_CURVE('',#16144,#16145,#13131,.T.);
#20844=EDGE_CURVE('',#15999,#16062,#13132,.T.);
#20845=EDGE_CURVE('',#15764,#16144,#1975,.T.);
#20846=EDGE_CURVE('',#16146,#16145,#1976,.T.);
#20847=EDGE_CURVE('',#15764,#16146,#13133,.T.);
#20848=EDGE_CURVE('',#16147,#16148,#13134,.T.);
#20849=EDGE_CURVE('',#16149,#16148,#9119,.T.);
#20850=EDGE_CURVE('',#16149,#16150,#13135,.T.);
#20851=EDGE_CURVE('',#16150,#16147,#9120,.T.);
#20852=EDGE_CURVE('',#16143,#16151,#13136,.T.);
#20853=EDGE_CURVE('',#16151,#16152,#13137,.T.);
#20854=EDGE_CURVE('',#16122,#16152,#13138,.T.);
#20855=EDGE_CURVE('',#16153,#16154,#13139,.T.);
#20856=EDGE_CURVE('',#16153,#16154,#13140,.T.);
#20857=EDGE_CURVE('',#16155,#16013,#13141,.T.);
#20858=EDGE_CURVE('',#16156,#16012,#13142,.T.);
#20859=EDGE_CURVE('',#16155,#16156,#13143,.T.);
#20860=EDGE_CURVE('',#16157,#16038,#13144,.T.);
#20861=EDGE_CURVE('',#16158,#16039,#13145,.T.);
#20862=EDGE_CURVE('',#16157,#16158,#13146,.T.);
#20863=EDGE_CURVE('',#15627,#16159,#13147,.T.);
#20864=EDGE_CURVE('',#16159,#16160,#9121,.T.);
#20865=EDGE_CURVE('',#15628,#16160,#13148,.T.);
#20866=EDGE_CURVE('',#15642,#16161,#13149,.T.);
#20867=EDGE_CURVE('',#16161,#16162,#9122,.T.);
#20868=EDGE_CURVE('',#15643,#16162,#13150,.T.);
#20869=EDGE_CURVE('',#16162,#16163,#13151,.T.);
#20870=EDGE_CURVE('',#15647,#16163,#13152,.T.);
#20871=EDGE_CURVE('',#16163,#16164,#9123,.T.);
#20872=EDGE_CURVE('',#15649,#16164,#13153,.T.);
#20873=EDGE_CURVE('',#16164,#16165,#13154,.T.);
#20874=EDGE_CURVE('',#15653,#16165,#13155,.T.);
#20875=EDGE_CURVE('',#16165,#16166,#9124,.T.);
#20876=EDGE_CURVE('',#15655,#16166,#13156,.T.);
#20877=EDGE_CURVE('',#16166,#16159,#13157,.T.);
#20878=EDGE_CURVE('',#16160,#16167,#13158,.T.);
#20879=EDGE_CURVE('',#16004,#16167,#13159,.T.);
#20880=EDGE_CURVE('',#16167,#16168,#9125,.T.);
#20881=EDGE_CURVE('',#16006,#16168,#13160,.T.);
#20882=EDGE_CURVE('',#16019,#16169,#13161,.T.);
#20883=EDGE_CURVE('',#16169,#16161,#13162,.T.);
#20884=EDGE_CURVE('',#16023,#16170,#13163,.T.);
#20885=EDGE_CURVE('',#16170,#16169,#9126,.T.);
#20886=EDGE_CURVE('',#16024,#16171,#13164,.T.);
#20887=EDGE_CURVE('',#16171,#16170,#13165,.T.);
#20888=EDGE_CURVE('',#16029,#16172,#13166,.T.);
#20889=EDGE_CURVE('',#16172,#16171,#9127,.T.);
#20890=EDGE_CURVE('',#16030,#16173,#13167,.T.);
#20891=EDGE_CURVE('',#16173,#16172,#13168,.T.);
#20892=EDGE_CURVE('',#16035,#16174,#13169,.T.);
#20893=EDGE_CURVE('',#16174,#16173,#9128,.T.);
#20894=EDGE_CURVE('',#16168,#16174,#13170,.T.);
#20895=EDGE_CURVE('',#16156,#16157,#13171,.T.);
#20896=EDGE_CURVE('',#16175,#16158,#9129,.T.);
#20897=EDGE_CURVE('',#16176,#16175,#13172,.T.);
#20898=EDGE_CURVE('',#16176,#15820,#9130,.T.);
#20899=EDGE_CURVE('',#15780,#16177,#13173,.T.);
#20900=EDGE_CURVE('',#16155,#16177,#13174,.T.);
#20901=EDGE_CURVE('',#16008,#15780,#1977,.T.);
#20902=EDGE_CURVE('',#16177,#16018,#1978,.T.);
#20903=EDGE_CURVE('',#16178,#16177,#13175,.T.);
#20904=EDGE_CURVE('',#16179,#16178,#13176,.T.);
#20905=EDGE_CURVE('',#16179,#16155,#13177,.T.);
#20906=EDGE_CURVE('',#15923,#16180,#13178,.T.);
#20907=EDGE_CURVE('',#16180,#16181,#9131,.T.);
#20908=EDGE_CURVE('',#15922,#16181,#13179,.T.);
#20909=EDGE_CURVE('',#15938,#16180,#13180,.T.);
#20910=EDGE_CURVE('',#16037,#16180,#13181,.T.);
#20911=EDGE_CURVE('',#16012,#16038,#13182,.T.);
#20912=EDGE_CURVE('',#16181,#16011,#1979,.T.);
#20913=EDGE_CURVE('',#16182,#16017,#690,.T.);
#20914=EDGE_CURVE('',#16153,#16016,#691,.T.);
#20915=EDGE_CURVE('',#16182,#16153,#1980,.T.);
#20916=EDGE_CURVE('',#16154,#16015,#692,.T.);
#20917=EDGE_CURVE('',#16183,#16014,#693,.T.);
#20918=EDGE_CURVE('',#16154,#16183,#1981,.T.);
#20919=EDGE_CURVE('',#16179,#16013,#13183,.T.);
#20920=EDGE_CURVE('',#16183,#16179,#9132,.T.);
#20921=EDGE_CURVE('',#16178,#16018,#13184,.T.);
#20922=EDGE_CURVE('',#16178,#16182,#9133,.T.);
#20923=EDGE_CURVE('',#16147,#16176,#13185,.T.);
#20924=EDGE_CURVE('',#16147,#15767,#9134,.T.);
#20925=EDGE_CURVE('',#15766,#16150,#9135,.T.);
#20926=EDGE_CURVE('',#16150,#16184,#13186,.T.);
#20927=EDGE_CURVE('',#16184,#16185,#1982,.T.);
#20928=EDGE_CURVE('',#16185,#15803,#9136,.T.);
#20929=EDGE_CURVE('',#16186,#15793,#13187,.T.);
#20930=EDGE_CURVE('',#16186,#16042,#13188,.T.);
#20931=EDGE_CURVE('',#16185,#16187,#13189,.T.);
#20932=EDGE_CURVE('',#16187,#16188,#13190,.T.);
#20933=EDGE_CURVE('',#16188,#16189,#9137,.T.);
#20934=EDGE_CURVE('',#16189,#16190,#13191,.T.);
#20935=EDGE_CURVE('',#16190,#16191,#13192,.T.);
#20936=EDGE_CURVE('',#16191,#16186,#9138,.T.);
#20937=EDGE_CURVE('',#16192,#16039,#13193,.T.);
#20938=EDGE_CURVE('',#16158,#16192,#13194,.T.);
#20939=EDGE_CURVE('',#16193,#16158,#13195,.T.);
#20940=EDGE_CURVE('',#16148,#16192,#9139,.T.);
#20941=EDGE_CURVE('',#16148,#16175,#13196,.T.);
#20942=EDGE_CURVE('',#16194,#16043,#1983,.T.);
#20943=EDGE_CURVE('',#16192,#16194,#9140,.T.);
#20944=EDGE_CURVE('',#16194,#16149,#9141,.T.);
#20945=EDGE_CURVE('',#16194,#16186,#1984,.T.);
#20946=EDGE_CURVE('',#16191,#16195,#1985,.T.);
#20947=EDGE_CURVE('',#16196,#16195,#9142,.T.);
#20948=EDGE_CURVE('',#16196,#16197,#694,.T.);
#20949=EDGE_CURVE('',#16197,#16149,#13197,.T.);
#20950=EDGE_CURVE('',#16198,#16199,#9143,.T.);
#20951=EDGE_CURVE('',#16199,#16047,#13198,.T.);
#20952=EDGE_CURVE('',#16198,#16046,#13199,.T.);
#20953=EDGE_CURVE('',#16198,#16051,#13200,.T.);
#20954=EDGE_CURVE('',#16197,#16184,#1986,.T.);
#20955=EDGE_CURVE('',#16196,#16198,#13201,.T.);
#20956=EDGE_CURVE('',#16187,#16052,#13202,.T.);
#20957=EDGE_CURVE('',#16188,#16055,#13203,.T.);
#20958=EDGE_CURVE('',#16189,#16056,#13204,.T.);
#20959=EDGE_CURVE('',#16199,#16059,#13205,.T.);
#20960=EDGE_CURVE('',#16190,#16061,#13206,.T.);
#20961=EDGE_CURVE('',#16199,#16195,#13207,.T.);
#20962=EDGE_CURVE('',#16064,#16200,#9144,.T.);
#20963=EDGE_CURVE('',#16201,#16200,#9145,.T.);
#20964=EDGE_CURVE('',#16201,#16062,#9146,.T.);
#20965=EDGE_CURVE('',#16066,#16151,#9147,.T.);
#20966=EDGE_CURVE('',#16067,#16143,#9148,.T.);
#20967=EDGE_CURVE('',#16070,#16202,#9149,.T.);
#20968=EDGE_CURVE('',#16202,#16151,#13208,.T.);
#20969=EDGE_CURVE('',#16203,#16072,#9150,.T.);
#20970=EDGE_CURVE('',#16202,#16203,#9151,.T.);
#20971=EDGE_CURVE('',#16204,#16074,#9152,.T.);
#20972=EDGE_CURVE('',#16203,#16204,#13209,.T.);
#20973=EDGE_CURVE('',#16076,#15996,#9153,.T.);
#20974=EDGE_CURVE('',#16204,#15996,#13210,.T.);
#20975=EDGE_CURVE('',#16077,#16121,#9154,.T.);
#20976=EDGE_CURVE('',#16080,#15994,#9155,.T.);
#20977=EDGE_CURVE('',#16084,#16125,#9156,.T.);
#20978=EDGE_CURVE('',#16081,#16123,#9157,.T.);
#20979=EDGE_CURVE('',#16087,#16127,#9158,.T.);
#20980=EDGE_CURVE('',#16092,#16128,#9159,.T.);
#20981=EDGE_CURVE('',#16093,#16130,#9160,.T.);
#20982=EDGE_CURVE('',#16096,#16131,#9161,.T.);
#20983=EDGE_CURVE('',#16132,#16102,#9162,.T.);
#20984=EDGE_CURVE('',#16103,#16133,#9163,.T.);
#20985=EDGE_CURVE('',#16118,#16106,#9164,.T.);
#20986=EDGE_CURVE('',#16119,#16108,#9165,.T.);
#20987=EDGE_CURVE('',#16205,#16110,#9166,.T.);
#20988=EDGE_CURVE('',#16119,#16205,#13211,.T.);
#20989=EDGE_CURVE('',#16206,#16112,#9167,.T.);
#20990=EDGE_CURVE('',#16205,#16206,#13212,.T.);
#20991=EDGE_CURVE('',#16133,#16207,#13213,.T.);
#20992=EDGE_CURVE('',#16113,#16207,#9168,.T.);
#20993=EDGE_CURVE('',#16208,#16116,#9169,.T.);
#20994=EDGE_CURVE('',#16206,#16208,#13214,.T.);
#20995=EDGE_CURVE('',#16208,#16207,#9170,.T.);
#20996=EDGE_CURVE('',#16120,#16205,#13215,.T.);
#20997=EDGE_CURVE('',#16209,#16206,#1987,.T.);
#20998=EDGE_CURVE('',#16120,#16209,#13216,.T.);
#20999=EDGE_CURVE('',#16207,#16134,#13217,.T.);
#21000=EDGE_CURVE('',#16209,#16208,#13218,.T.);
#21001=EDGE_CURVE('',#16209,#16134,#9171,.T.);
#21002=EDGE_CURVE('',#16210,#15995,#13219,.T.);
#21003=EDGE_CURVE('',#16152,#16210,#9172,.T.);
#21004=EDGE_CURVE('',#16211,#16212,#13220,.T.);
#21005=EDGE_CURVE('',#16200,#16212,#13221,.T.);
#21006=EDGE_CURVE('',#16211,#16200,#13222,.T.);
#21007=EDGE_CURVE('',#16136,#16211,#9173,.T.);
#21008=EDGE_CURVE('',#16182,#16183,#13223,.T.);
#21009=EDGE_CURVE('',#16202,#16152,#13224,.T.);
#21010=EDGE_CURVE('',#16210,#16204,#1988,.T.);
#21011=EDGE_CURVE('',#16201,#16145,#13225,.T.);
#21012=EDGE_CURVE('',#16146,#16201,#1989,.T.);
#21013=EDGE_CURVE('',#16210,#16203,#1990,.T.);
#21014=EDGE_CURVE('',#16146,#16212,#9174,.T.);
#21015=EDGE_CURVE('',#16213,#16214,#13226,.T.);
#21016=EDGE_CURVE('',#16215,#16214,#13227,.T.);
#21017=EDGE_CURVE('',#16213,#16215,#13228,.T.);
#21018=EDGE_CURVE('',#16142,#16213,#9175,.T.);
#21019=EDGE_CURVE('',#16138,#16215,#9176,.T.);
#21020=EDGE_CURVE('',#16211,#16215,#13229,.T.);
#21021=EDGE_CURVE('',#16212,#16214,#13230,.T.);
#21022=EDGE_CURVE('',#16216,#16217,#9177,.T.);
#21023=EDGE_CURVE('',#16217,#15941,#13231,.T.);
#21024=EDGE_CURVE('',#16216,#15940,#13232,.T.);
#21025=EDGE_CURVE('',#16218,#16216,#13233,.T.);
#21026=EDGE_CURVE('',#16218,#15948,#13234,.T.);
#21027=EDGE_CURVE('',#16219,#16218,#13235,.T.);
#21028=EDGE_CURVE('',#16219,#15949,#13236,.T.);
#21029=EDGE_CURVE('',#16220,#16219,#13237,.T.);
#21030=EDGE_CURVE('',#16220,#15952,#13238,.T.);
#21031=EDGE_CURVE('',#16221,#16220,#9178,.T.);
#21032=EDGE_CURVE('',#16221,#15954,#13239,.T.);
#21033=EDGE_CURVE('',#15835,#16221,#13240,.T.);
#21034=EDGE_CURVE('',#16214,#16222,#9179,.T.);
#21035=EDGE_CURVE('',#16217,#16222,#13241,.T.);
#21036=EDGE_CURVE('',#16217,#16223,#13242,.T.);
#21037=EDGE_CURVE('',#16223,#15941,#13243,.T.);
#21038=EDGE_CURVE('',#16217,#16224,#13244,.T.);
#21039=EDGE_CURVE('',#16222,#16225,#1991,.T.);
#21040=EDGE_CURVE('',#16223,#16225,#13245,.T.);
#21041=EDGE_CURVE('',#15955,#16221,#13246,.T.);
#21042=EDGE_CURVE('',#16226,#15835,#1992,.T.);
#21043=EDGE_CURVE('',#15834,#16226,#13247,.T.);
#21044=EDGE_CURVE('',#16226,#15955,#13248,.T.);
#21045=EDGE_CURVE('',#16223,#16000,#9180,.T.);
#21046=EDGE_CURVE('',#16225,#16002,#9181,.T.);
#21047=EDGE_CURVE('',#15964,#16226,#9182,.T.);
#21048=EDGE_CURVE('',#16227,#16225,#13249,.T.);
#21049=EDGE_CURVE('',#16227,#16139,#9183,.T.);
#21050=EDGE_CURVE('',#16222,#16227,#13250,.T.);
#21051=EDGE_CURVE('',#16213,#16227,#9184,.T.);
#21052=EDGE_CURVE('',#16142,#16139,#9185,.T.);
#21053=EDGE_CURVE('',#16141,#16140,#9186,.T.);
#21054=EDGE_CURVE('',#16228,#15893,#1993,.T.);
#21055=EDGE_CURVE('',#16228,#15897,#695,.T.);
#21056=EDGE_CURVE('',#16228,#16229,#9187,.T.);
#21057=EDGE_CURVE('',#16045,#16229,#13251,.T.);
#21058=EDGE_CURVE('',#16229,#16230,#13252,.T.);
#21059=EDGE_CURVE('',#16050,#16230,#13253,.T.);
#21060=EDGE_CURVE('',#16230,#16231,#13254,.T.);
#21061=EDGE_CURVE('',#16053,#16231,#13255,.T.);
#21062=EDGE_CURVE('',#16231,#16232,#13256,.T.);
#21063=EDGE_CURVE('',#16054,#16232,#13257,.T.);
#21064=EDGE_CURVE('',#16232,#16233,#9188,.T.);
#21065=EDGE_CURVE('',#16057,#16233,#13258,.T.);
#21066=EDGE_CURVE('',#16058,#16234,#1994,.T.);
#21067=EDGE_CURVE('',#16234,#16049,#13259,.T.);
#21068=EDGE_CURVE('',#16058,#16235,#13260,.T.);
#21069=EDGE_CURVE('',#16235,#16234,#13261,.T.);
#21070=EDGE_CURVE('',#16233,#16236,#13262,.T.);
#21071=EDGE_CURVE('',#16060,#16236,#13263,.T.);
#21072=EDGE_CURVE('',#16236,#16235,#13264,.T.);
#21073=EDGE_CURVE('',#16237,#16228,#13265,.T.);
#21074=EDGE_CURVE('',#16237,#15896,#13266,.T.);
#21075=EDGE_CURVE('',#16238,#16237,#13267,.T.);
#21076=EDGE_CURVE('',#16238,#15899,#696,.T.);
#21077=EDGE_CURVE('',#16239,#16011,#697,.T.);
#21078=EDGE_CURVE('',#16240,#16010,#698,.T.);
#21079=EDGE_CURVE('',#16239,#16240,#699,.T.);
#21080=EDGE_CURVE('',#15922,#16239,#1995,.T.);
#21081=EDGE_CURVE('',#16241,#16240,#9189,.T.);
#21082=EDGE_CURVE('',#15921,#16241,#700,.T.);
#21083=EDGE_CURVE('',#16242,#16009,#701,.T.);
#21084=EDGE_CURVE('',#16242,#15944,#1996,.T.);
#21085=EDGE_CURVE('',#16001,#16242,#9190,.T.);
#21086=EDGE_CURVE('',#16243,#16041,#702,.T.);
#21087=EDGE_CURVE('',#16243,#16044,#1997,.T.);
#21088=EDGE_CURVE('',#16234,#16243,#9191,.T.);
#21089=EDGE_CURVE('',#16240,#16242,#13268,.T.);
#21090=EDGE_CURVE('',#16243,#15852,#13269,.T.);
#21091=EDGE_CURVE('',#15629,#16244,#13270,.T.);
#21092=EDGE_CURVE('',#16244,#16245,#9192,.T.);
#21093=EDGE_CURVE('',#15630,#16245,#13271,.T.);
#21094=EDGE_CURVE('',#15716,#16246,#9193,.T.);
#21095=EDGE_CURVE('',#15646,#16246,#13272,.T.);
#21096=EDGE_CURVE('',#15707,#15718,#9194,.T.);
#21097=EDGE_CURVE('',#15656,#16247,#13273,.T.);
#21098=EDGE_CURVE('',#16247,#15703,#9195,.T.);
#21099=EDGE_CURVE('',#16245,#16247,#13274,.T.);
#21100=EDGE_CURVE('',#16005,#16248,#13275,.T.);
#21101=EDGE_CURVE('',#16248,#16244,#13276,.T.);
#21102=EDGE_CURVE('',#16007,#16249,#13277,.T.);
#21103=EDGE_CURVE('',#16249,#16248,#9196,.T.);
#21104=EDGE_CURVE('',#16246,#16250,#13278,.T.);
#21105=EDGE_CURVE('',#16020,#16250,#13279,.T.);
#21106=EDGE_CURVE('',#16250,#16097,#9197,.T.);
#21107=EDGE_CURVE('',#16100,#16088,#9198,.T.);
#21108=EDGE_CURVE('',#16086,#16251,#9199,.T.);
#21109=EDGE_CURVE('',#16034,#16251,#13280,.T.);
#21110=EDGE_CURVE('',#16251,#16249,#13281,.T.);
#21111=EDGE_CURVE('',#16252,#16238,#9200,.T.);
#21112=EDGE_CURVE('',#16253,#16252,#13282,.T.);
#21113=EDGE_CURVE('',#16254,#16253,#13283,.T.);
#21114=EDGE_CURVE('',#16255,#16254,#13284,.T.);
#21115=EDGE_CURVE('',#16256,#16255,#9201,.T.);
#21116=EDGE_CURVE('',#16257,#16256,#13285,.T.);
#21117=EDGE_CURVE('',#16241,#16257,#13286,.T.);
#21118=EDGE_CURVE('',#16258,#16259,#13287,.T.);
#21119=EDGE_CURVE('',#16258,#15903,#1998,.T.);
#21120=EDGE_CURVE('',#16259,#15904,#1999,.T.);
#21121=EDGE_CURVE('',#15918,#16260,#2000,.T.);
#21122=EDGE_CURVE('',#16261,#16260,#2001,.T.);
#21123=EDGE_CURVE('',#15919,#16261,#703,.T.);
#21124=EDGE_CURVE('',#16260,#16241,#13288,.T.);
#21125=EDGE_CURVE('',#16262,#16257,#13289,.T.);
#21126=EDGE_CURVE('',#16261,#16262,#13290,.T.);
#21127=EDGE_CURVE('',#16263,#16256,#13291,.T.);
#21128=EDGE_CURVE('',#16262,#16263,#13292,.T.);
#21129=EDGE_CURVE('',#16264,#16255,#13293,.T.);
#21130=EDGE_CURVE('',#16263,#16264,#9202,.T.);
#21131=EDGE_CURVE('',#16265,#16254,#13294,.T.);
#21132=EDGE_CURVE('',#16264,#16265,#13295,.T.);
#21133=EDGE_CURVE('',#16266,#16253,#13296,.T.);
#21134=EDGE_CURVE('',#16265,#16266,#13297,.T.);
#21135=EDGE_CURVE('',#16267,#16252,#13298,.T.);
#21136=EDGE_CURVE('',#16266,#16267,#13299,.T.);
#21137=EDGE_CURVE('',#16268,#16238,#704,.T.);
#21138=EDGE_CURVE('',#16268,#15898,#705,.T.);
#21139=EDGE_CURVE('',#15902,#16268,#2002,.T.);
#21140=EDGE_CURVE('',#16267,#15902,#9203,.T.);
#21141=EDGE_CURVE('',#16269,#16258,#9204,.T.);
#21142=EDGE_CURVE('',#16270,#16269,#13300,.T.);
#21143=EDGE_CURVE('',#15931,#16270,#9205,.T.);
#21144=EDGE_CURVE('',#16271,#16259,#9206,.T.);
#21145=EDGE_CURVE('',#16269,#16271,#13301,.T.);
#21146=EDGE_CURVE('',#16271,#15907,#13302,.T.);
#21147=EDGE_CURVE('',#16272,#16261,#9207,.T.);
#21148=EDGE_CURVE('',#15920,#16272,#13303,.T.);
#21149=EDGE_CURVE('',#16262,#16273,#9208,.T.);
#21150=EDGE_CURVE('',#16272,#16273,#13304,.T.);
#21151=EDGE_CURVE('',#16263,#16274,#9209,.T.);
#21152=EDGE_CURVE('',#16274,#16273,#13305,.T.);
#21153=EDGE_CURVE('',#16264,#16275,#9210,.T.);
#21154=EDGE_CURVE('',#16274,#16275,#9211,.T.);
#21155=EDGE_CURVE('',#16265,#16276,#9212,.T.);
#21156=EDGE_CURVE('',#16276,#16275,#13306,.T.);
#21157=EDGE_CURVE('',#16266,#16277,#9213,.T.);
#21158=EDGE_CURVE('',#16276,#16277,#13307,.T.);
#21159=EDGE_CURVE('',#16267,#16278,#9214,.T.);
#21160=EDGE_CURVE('',#16278,#16277,#13308,.T.);
#21161=EDGE_CURVE('',#15929,#16279,#9215,.T.);
#21162=EDGE_CURVE('',#16278,#16279,#9216,.T.);
#21163=EDGE_CURVE('',#16279,#16270,#13309,.T.);
#21164=EDGE_CURVE('',#16280,#16279,#13310,.T.);
#21165=EDGE_CURVE('',#16280,#16270,#13311,.T.);
#21166=EDGE_CURVE('',#16269,#16281,#13312,.T.);
#21167=EDGE_CURVE('',#16280,#16281,#13313,.T.);
#21168=EDGE_CURVE('',#16271,#16282,#13314,.T.);
#21169=EDGE_CURVE('',#16281,#16282,#13315,.T.);
#21170=EDGE_CURVE('',#15908,#16283,#13316,.T.);
#21171=EDGE_CURVE('',#15907,#16283,#13317,.T.);
#21172=EDGE_CURVE('',#16282,#16283,#13318,.T.);
#21173=EDGE_CURVE('',#16284,#16272,#13319,.T.);
#21174=EDGE_CURVE('',#15920,#16284,#13320,.T.);
#21175=EDGE_CURVE('',#16273,#16285,#13321,.T.);
#21176=EDGE_CURVE('',#16284,#16285,#13322,.T.);
#21177=EDGE_CURVE('',#16274,#16285,#13323,.T.);
#21178=EDGE_CURVE('',#16275,#16286,#13324,.T.);
#21179=EDGE_CURVE('',#16285,#16286,#9217,.T.);
#21180=EDGE_CURVE('',#16276,#16286,#13325,.T.);
#21181=EDGE_CURVE('',#16277,#16287,#13326,.T.);
#21182=EDGE_CURVE('',#16286,#16287,#13327,.T.);
#21183=EDGE_CURVE('',#16278,#16287,#13328,.T.);
#21184=EDGE_CURVE('',#16287,#16280,#9218,.T.);
#21185=EDGE_CURVE('',#15911,#16288,#13329,.T.);
#21186=EDGE_CURVE('',#16283,#16288,#9219,.T.);
#21187=EDGE_CURVE('',#15914,#16289,#13330,.T.);
#21188=EDGE_CURVE('',#16288,#16289,#13331,.T.);
#21189=EDGE_CURVE('',#15915,#16290,#13332,.T.);
#21190=EDGE_CURVE('',#16289,#16290,#13333,.T.);
#21191=EDGE_CURVE('',#16290,#16284,#13334,.T.);
#27993=ORIENTED_EDGE('',*,*,#19768,.F.);
#27994=ORIENTED_EDGE('',*,*,#19769,.F.);
#27995=ORIENTED_EDGE('',*,*,#19770,.T.);
#27996=ORIENTED_EDGE('',*,*,#19771,.T.);
#27997=ORIENTED_EDGE('',*,*,#19772,.F.);
#27998=ORIENTED_EDGE('',*,*,#19773,.T.);
#27999=ORIENTED_EDGE('',*,*,#19774,.T.);
#28000=ORIENTED_EDGE('',*,*,#19770,.F.);
#28001=ORIENTED_EDGE('',*,*,#19775,.F.);
#28002=ORIENTED_EDGE('',*,*,#19776,.F.);
#28003=ORIENTED_EDGE('',*,*,#19777,.F.);
#28004=ORIENTED_EDGE('',*,*,#19778,.T.);
#28005=ORIENTED_EDGE('',*,*,#19779,.T.);
#28006=ORIENTED_EDGE('',*,*,#19773,.F.);
#28007=ORIENTED_EDGE('',*,*,#19780,.F.);
#28008=ORIENTED_EDGE('',*,*,#19781,.T.);
#28009=ORIENTED_EDGE('',*,*,#19782,.T.);
#28010=ORIENTED_EDGE('',*,*,#19783,.T.);
#28011=ORIENTED_EDGE('',*,*,#19784,.F.);
#28012=ORIENTED_EDGE('',*,*,#19785,.T.);
#28013=ORIENTED_EDGE('',*,*,#19786,.T.);
#28014=ORIENTED_EDGE('',*,*,#19787,.T.);
#28015=ORIENTED_EDGE('',*,*,#19788,.T.);
#28016=ORIENTED_EDGE('',*,*,#19789,.T.);
#28017=ORIENTED_EDGE('',*,*,#19784,.T.);
#28018=ORIENTED_EDGE('',*,*,#19790,.T.);
#28019=ORIENTED_EDGE('',*,*,#19791,.T.);
#28020=ORIENTED_EDGE('',*,*,#19792,.T.);
#28021=ORIENTED_EDGE('',*,*,#19793,.T.);
#28022=ORIENTED_EDGE('',*,*,#19788,.F.);
#28023=ORIENTED_EDGE('',*,*,#19794,.T.);
#28024=ORIENTED_EDGE('',*,*,#19795,.T.);
#28025=ORIENTED_EDGE('',*,*,#19792,.F.);
#28026=ORIENTED_EDGE('',*,*,#19796,.T.);
#28027=ORIENTED_EDGE('',*,*,#19797,.T.);
#28028=ORIENTED_EDGE('',*,*,#19798,.T.);
#28029=ORIENTED_EDGE('',*,*,#19799,.T.);
#28030=ORIENTED_EDGE('',*,*,#19800,.T.);
#28031=ORIENTED_EDGE('',*,*,#19801,.T.);
#28032=ORIENTED_EDGE('',*,*,#19794,.F.);
#28033=ORIENTED_EDGE('',*,*,#19802,.F.);
#28034=ORIENTED_EDGE('',*,*,#19803,.T.);
#28035=ORIENTED_EDGE('',*,*,#19800,.F.);
#28036=ORIENTED_EDGE('',*,*,#19804,.T.);
#28037=ORIENTED_EDGE('',*,*,#19805,.T.);
#28038=ORIENTED_EDGE('',*,*,#19806,.F.);
#28039=ORIENTED_EDGE('',*,*,#19807,.F.);
#28040=ORIENTED_EDGE('',*,*,#19808,.F.);
#28041=ORIENTED_EDGE('',*,*,#19809,.T.);
#28042=ORIENTED_EDGE('',*,*,#19808,.T.);
#28043=ORIENTED_EDGE('',*,*,#19771,.F.);
#28044=ORIENTED_EDGE('',*,*,#19810,.F.);
#28045=ORIENTED_EDGE('',*,*,#19811,.T.);
#28046=ORIENTED_EDGE('',*,*,#19810,.T.);
#28047=ORIENTED_EDGE('',*,*,#19774,.F.);
#28048=ORIENTED_EDGE('',*,*,#19812,.F.);
#28049=ORIENTED_EDGE('',*,*,#19812,.T.);
#28050=ORIENTED_EDGE('',*,*,#19779,.F.);
#28051=ORIENTED_EDGE('',*,*,#19813,.F.);
#28052=ORIENTED_EDGE('',*,*,#19814,.T.);
#28053=ORIENTED_EDGE('',*,*,#19813,.T.);
#28054=ORIENTED_EDGE('',*,*,#19815,.F.);
#28055=ORIENTED_EDGE('',*,*,#19816,.F.);
#28056=ORIENTED_EDGE('',*,*,#19817,.T.);
#28057=ORIENTED_EDGE('',*,*,#19816,.T.);
#28058=ORIENTED_EDGE('',*,*,#19818,.F.);
#28059=ORIENTED_EDGE('',*,*,#19819,.F.);
#28060=ORIENTED_EDGE('',*,*,#19820,.T.);
#28061=ORIENTED_EDGE('',*,*,#19819,.T.);
#28062=ORIENTED_EDGE('',*,*,#19821,.F.);
#28063=ORIENTED_EDGE('',*,*,#19822,.F.);
#28064=ORIENTED_EDGE('',*,*,#19823,.T.);
#28065=ORIENTED_EDGE('',*,*,#19822,.T.);
#28066=ORIENTED_EDGE('',*,*,#19781,.F.);
#28067=ORIENTED_EDGE('',*,*,#19824,.F.);
#28068=ORIENTED_EDGE('',*,*,#19825,.T.);
#28069=ORIENTED_EDGE('',*,*,#19824,.T.);
#28070=ORIENTED_EDGE('',*,*,#19826,.F.);
#28071=ORIENTED_EDGE('',*,*,#19827,.F.);
#28072=ORIENTED_EDGE('',*,*,#19828,.T.);
#28073=ORIENTED_EDGE('',*,*,#19827,.T.);
#28074=ORIENTED_EDGE('',*,*,#19785,.F.);
#28075=ORIENTED_EDGE('',*,*,#19829,.F.);
#28076=ORIENTED_EDGE('',*,*,#19830,.T.);
#28077=ORIENTED_EDGE('',*,*,#19829,.T.);
#28078=ORIENTED_EDGE('',*,*,#19789,.F.);
#28079=ORIENTED_EDGE('',*,*,#19831,.F.);
#28080=ORIENTED_EDGE('',*,*,#19831,.T.);
#28081=ORIENTED_EDGE('',*,*,#19793,.F.);
#28082=ORIENTED_EDGE('',*,*,#19832,.F.);
#28083=ORIENTED_EDGE('',*,*,#19833,.T.);
#28084=ORIENTED_EDGE('',*,*,#19832,.T.);
#28085=ORIENTED_EDGE('',*,*,#19795,.F.);
#28086=ORIENTED_EDGE('',*,*,#19834,.F.);
#28087=ORIENTED_EDGE('',*,*,#19834,.T.);
#28088=ORIENTED_EDGE('',*,*,#19801,.F.);
#28089=ORIENTED_EDGE('',*,*,#19835,.F.);
#28090=ORIENTED_EDGE('',*,*,#19836,.F.);
#28091=ORIENTED_EDGE('',*,*,#19837,.T.);
#28092=ORIENTED_EDGE('',*,*,#19835,.T.);
#28093=ORIENTED_EDGE('',*,*,#19803,.F.);
#28094=ORIENTED_EDGE('',*,*,#19838,.F.);
#28095=ORIENTED_EDGE('',*,*,#19839,.F.);
#28096=ORIENTED_EDGE('',*,*,#19809,.F.);
#28097=ORIENTED_EDGE('',*,*,#19811,.F.);
#28098=ORIENTED_EDGE('',*,*,#19814,.F.);
#28099=ORIENTED_EDGE('',*,*,#19817,.F.);
#28100=ORIENTED_EDGE('',*,*,#19820,.F.);
#28101=ORIENTED_EDGE('',*,*,#19823,.F.);
#28102=ORIENTED_EDGE('',*,*,#19825,.F.);
#28103=ORIENTED_EDGE('',*,*,#19828,.F.);
#28104=ORIENTED_EDGE('',*,*,#19830,.F.);
#28105=ORIENTED_EDGE('',*,*,#19833,.F.);
#28106=ORIENTED_EDGE('',*,*,#19837,.F.);
#28107=ORIENTED_EDGE('',*,*,#19840,.T.);
#28108=ORIENTED_EDGE('',*,*,#19841,.T.);
#28109=ORIENTED_EDGE('',*,*,#19842,.F.);
#28110=ORIENTED_EDGE('',*,*,#19843,.F.);
#28111=ORIENTED_EDGE('',*,*,#19844,.F.);
#28112=ORIENTED_EDGE('',*,*,#19845,.F.);
#28113=ORIENTED_EDGE('',*,*,#19846,.F.);
#28114=ORIENTED_EDGE('',*,*,#19847,.F.);
#28115=ORIENTED_EDGE('',*,*,#19848,.T.);
#28116=ORIENTED_EDGE('',*,*,#19849,.T.);
#28117=ORIENTED_EDGE('',*,*,#19840,.F.);
#28118=ORIENTED_EDGE('',*,*,#19850,.T.);
#28119=ORIENTED_EDGE('',*,*,#19851,.T.);
#28120=ORIENTED_EDGE('',*,*,#19848,.F.);
#28121=ORIENTED_EDGE('',*,*,#19852,.F.);
#28122=ORIENTED_EDGE('',*,*,#19853,.F.);
#28123=ORIENTED_EDGE('',*,*,#19854,.T.);
#28124=ORIENTED_EDGE('',*,*,#19855,.T.);
#28125=ORIENTED_EDGE('',*,*,#19850,.F.);
#28126=ORIENTED_EDGE('',*,*,#19856,.F.);
#28127=ORIENTED_EDGE('',*,*,#19857,.F.);
#28128=ORIENTED_EDGE('',*,*,#19858,.T.);
#28129=ORIENTED_EDGE('',*,*,#19854,.F.);
#28130=ORIENTED_EDGE('',*,*,#19859,.F.);
#28131=ORIENTED_EDGE('',*,*,#19860,.T.);
#28132=ORIENTED_EDGE('',*,*,#19857,.T.);
#28133=ORIENTED_EDGE('',*,*,#19861,.F.);
#28134=ORIENTED_EDGE('',*,*,#19862,.T.);
#28135=ORIENTED_EDGE('',*,*,#19842,.T.);
#28136=ORIENTED_EDGE('',*,*,#19863,.T.);
#28137=ORIENTED_EDGE('',*,*,#19864,.F.);
#28138=ORIENTED_EDGE('',*,*,#19865,.T.);
#28139=ORIENTED_EDGE('',*,*,#19866,.T.);
#28140=ORIENTED_EDGE('',*,*,#19841,.F.);
#28141=ORIENTED_EDGE('',*,*,#19867,.F.);
#28142=ORIENTED_EDGE('',*,*,#19867,.T.);
#28143=ORIENTED_EDGE('',*,*,#19849,.F.);
#28144=ORIENTED_EDGE('',*,*,#19868,.F.);
#28145=ORIENTED_EDGE('',*,*,#19869,.T.);
#28146=ORIENTED_EDGE('',*,*,#19868,.T.);
#28147=ORIENTED_EDGE('',*,*,#19851,.F.);
#28148=ORIENTED_EDGE('',*,*,#19870,.F.);
#28149=ORIENTED_EDGE('',*,*,#19870,.T.);
#28150=ORIENTED_EDGE('',*,*,#19855,.F.);
#28151=ORIENTED_EDGE('',*,*,#19871,.F.);
#28152=ORIENTED_EDGE('',*,*,#19872,.T.);
#28153=ORIENTED_EDGE('',*,*,#19871,.T.);
#28154=ORIENTED_EDGE('',*,*,#19858,.F.);
#28155=ORIENTED_EDGE('',*,*,#19873,.F.);
#28156=ORIENTED_EDGE('',*,*,#19874,.T.);
#28157=ORIENTED_EDGE('',*,*,#19873,.T.);
#28158=ORIENTED_EDGE('',*,*,#19860,.F.);
#28159=ORIENTED_EDGE('',*,*,#19875,.F.);
#28160=ORIENTED_EDGE('',*,*,#19876,.F.);
#28161=ORIENTED_EDGE('',*,*,#19877,.T.);
#28162=ORIENTED_EDGE('',*,*,#19875,.T.);
#28163=ORIENTED_EDGE('',*,*,#19878,.F.);
#28164=ORIENTED_EDGE('',*,*,#19879,.T.);
#28165=ORIENTED_EDGE('',*,*,#19863,.F.);
#28166=ORIENTED_EDGE('',*,*,#19866,.F.);
#28167=ORIENTED_EDGE('',*,*,#19880,.T.);
#28168=ORIENTED_EDGE('',*,*,#19881,.F.);
#28169=ORIENTED_EDGE('',*,*,#19879,.F.);
#28170=ORIENTED_EDGE('',*,*,#19882,.T.);
#28171=ORIENTED_EDGE('',*,*,#19883,.F.);
#28172=ORIENTED_EDGE('',*,*,#19884,.F.);
#28173=ORIENTED_EDGE('',*,*,#19885,.T.);
#28174=ORIENTED_EDGE('',*,*,#19886,.F.);
#28175=ORIENTED_EDGE('',*,*,#19887,.T.);
#28176=ORIENTED_EDGE('',*,*,#19888,.F.);
#28177=ORIENTED_EDGE('',*,*,#19889,.F.);
#28178=ORIENTED_EDGE('',*,*,#19890,.T.);
#28179=ORIENTED_EDGE('',*,*,#19891,.T.);
#28180=ORIENTED_EDGE('',*,*,#19892,.T.);
#28181=ORIENTED_EDGE('',*,*,#19893,.F.);
#28182=ORIENTED_EDGE('',*,*,#19894,.T.);
#28183=ORIENTED_EDGE('',*,*,#19895,.F.);
#28184=ORIENTED_EDGE('',*,*,#19896,.F.);
#28185=ORIENTED_EDGE('',*,*,#19897,.T.);
#28186=ORIENTED_EDGE('',*,*,#19898,.T.);
#28187=ORIENTED_EDGE('',*,*,#19884,.T.);
#28188=ORIENTED_EDGE('',*,*,#19899,.F.);
#28189=ORIENTED_EDGE('',*,*,#19898,.F.);
#28190=ORIENTED_EDGE('',*,*,#19900,.F.);
#28191=ORIENTED_EDGE('',*,*,#19901,.F.);
#28192=ORIENTED_EDGE('',*,*,#19883,.T.);
#28193=ORIENTED_EDGE('',*,*,#19902,.F.);
#28194=ORIENTED_EDGE('',*,*,#19903,.T.);
#28195=ORIENTED_EDGE('',*,*,#19886,.T.);
#28196=ORIENTED_EDGE('',*,*,#19890,.F.);
#28197=ORIENTED_EDGE('',*,*,#19904,.F.);
#28198=ORIENTED_EDGE('',*,*,#19905,.T.);
#28199=ORIENTED_EDGE('',*,*,#19889,.T.);
#28200=ORIENTED_EDGE('',*,*,#19906,.F.);
#28201=ORIENTED_EDGE('',*,*,#19907,.T.);
#28202=ORIENTED_EDGE('',*,*,#19888,.T.);
#28203=ORIENTED_EDGE('',*,*,#19894,.F.);
#28204=ORIENTED_EDGE('',*,*,#19908,.T.);
#28205=ORIENTED_EDGE('',*,*,#19893,.T.);
#28206=ORIENTED_EDGE('',*,*,#19909,.T.);
#28207=ORIENTED_EDGE('',*,*,#19910,.F.);
#28208=ORIENTED_EDGE('',*,*,#19896,.T.);
#28209=ORIENTED_EDGE('',*,*,#19911,.F.);
#28210=ORIENTED_EDGE('',*,*,#19892,.F.);
#28211=ORIENTED_EDGE('',*,*,#19912,.F.);
#28212=ORIENTED_EDGE('',*,*,#19895,.T.);
#28213=ORIENTED_EDGE('',*,*,#19913,.T.);
#28214=ORIENTED_EDGE('',*,*,#19914,.F.);
#28215=ORIENTED_EDGE('',*,*,#19913,.F.);
#28216=ORIENTED_EDGE('',*,*,#19899,.T.);
#28217=ORIENTED_EDGE('',*,*,#19901,.T.);
#28218=ORIENTED_EDGE('',*,*,#19915,.F.);
#28219=ORIENTED_EDGE('',*,*,#19900,.T.);
#28220=ORIENTED_EDGE('',*,*,#19916,.T.);
#28221=ORIENTED_EDGE('',*,*,#19917,.F.);
#28222=ORIENTED_EDGE('',*,*,#19918,.F.);
#28223=ORIENTED_EDGE('',*,*,#19902,.T.);
#28224=ORIENTED_EDGE('',*,*,#19903,.F.);
#28225=ORIENTED_EDGE('',*,*,#19905,.F.);
#28226=ORIENTED_EDGE('',*,*,#19919,.F.);
#28227=ORIENTED_EDGE('',*,*,#19904,.T.);
#28228=ORIENTED_EDGE('',*,*,#19920,.T.);
#28229=ORIENTED_EDGE('',*,*,#19921,.F.);
#28230=ORIENTED_EDGE('',*,*,#19922,.F.);
#28231=ORIENTED_EDGE('',*,*,#19906,.T.);
#28232=ORIENTED_EDGE('',*,*,#19907,.F.);
#28233=ORIENTED_EDGE('',*,*,#19908,.F.);
#28234=ORIENTED_EDGE('',*,*,#19923,.F.);
#28235=ORIENTED_EDGE('',*,*,#19910,.T.);
#28236=ORIENTED_EDGE('',*,*,#19924,.T.);
#28237=ORIENTED_EDGE('',*,*,#19925,.F.);
#28238=ORIENTED_EDGE('',*,*,#19926,.F.);
#28239=ORIENTED_EDGE('',*,*,#19909,.F.);
#28240=ORIENTED_EDGE('',*,*,#19911,.T.);
#28241=ORIENTED_EDGE('',*,*,#19912,.T.);
#28242=ORIENTED_EDGE('',*,*,#19927,.F.);
#28243=ORIENTED_EDGE('',*,*,#19914,.T.);
#28244=ORIENTED_EDGE('',*,*,#19928,.T.);
#28245=ORIENTED_EDGE('',*,*,#19929,.F.);
#28246=ORIENTED_EDGE('',*,*,#19930,.F.);
#28247=ORIENTED_EDGE('',*,*,#19915,.T.);
#28248=ORIENTED_EDGE('',*,*,#19918,.T.);
#28249=ORIENTED_EDGE('',*,*,#19931,.F.);
#28250=ORIENTED_EDGE('',*,*,#19928,.F.);
#28251=ORIENTED_EDGE('',*,*,#19932,.T.);
#28252=ORIENTED_EDGE('',*,*,#19933,.T.);
#28253=ORIENTED_EDGE('',*,*,#19934,.F.);
#28254=ORIENTED_EDGE('',*,*,#19919,.T.);
#28255=ORIENTED_EDGE('',*,*,#19922,.T.);
#28256=ORIENTED_EDGE('',*,*,#19935,.F.);
#28257=ORIENTED_EDGE('',*,*,#19916,.F.);
#28258=ORIENTED_EDGE('',*,*,#19923,.T.);
#28259=ORIENTED_EDGE('',*,*,#19926,.T.);
#28260=ORIENTED_EDGE('',*,*,#19936,.F.);
#28261=ORIENTED_EDGE('',*,*,#19920,.F.);
#28262=ORIENTED_EDGE('',*,*,#19927,.T.);
#28263=ORIENTED_EDGE('',*,*,#19930,.T.);
#28264=ORIENTED_EDGE('',*,*,#19937,.F.);
#28265=ORIENTED_EDGE('',*,*,#19924,.F.);
#28266=ORIENTED_EDGE('',*,*,#19938,.F.);
#28267=ORIENTED_EDGE('',*,*,#19939,.F.);
#28268=ORIENTED_EDGE('',*,*,#19940,.T.);
#28269=ORIENTED_EDGE('',*,*,#19941,.T.);
#28270=ORIENTED_EDGE('',*,*,#19897,.F.);
#28271=ORIENTED_EDGE('',*,*,#19891,.F.);
#28272=ORIENTED_EDGE('',*,*,#19887,.F.);
#28273=ORIENTED_EDGE('',*,*,#19885,.F.);
#28274=ORIENTED_EDGE('',*,*,#19942,.T.);
#28275=ORIENTED_EDGE('',*,*,#19844,.T.);
#28276=ORIENTED_EDGE('',*,*,#19943,.F.);
#28277=ORIENTED_EDGE('',*,*,#19944,.F.);
#28278=ORIENTED_EDGE('',*,*,#19944,.T.);
#28279=ORIENTED_EDGE('',*,*,#19945,.F.);
#28280=ORIENTED_EDGE('',*,*,#19946,.F.);
#28281=ORIENTED_EDGE('',*,*,#19947,.T.);
#28282=ORIENTED_EDGE('',*,*,#19948,.T.);
#28283=ORIENTED_EDGE('',*,*,#19949,.T.);
#28284=ORIENTED_EDGE('',*,*,#19950,.T.);
#28285=ORIENTED_EDGE('',*,*,#19951,.F.);
#28286=ORIENTED_EDGE('',*,*,#19952,.T.);
#28287=ORIENTED_EDGE('',*,*,#19953,.T.);
#28288=ORIENTED_EDGE('',*,*,#19954,.T.);
#28289=ORIENTED_EDGE('',*,*,#19955,.T.);
#28290=ORIENTED_EDGE('',*,*,#19956,.T.);
#28291=ORIENTED_EDGE('',*,*,#19957,.T.);
#28292=ORIENTED_EDGE('',*,*,#19958,.T.);
#28293=ORIENTED_EDGE('',*,*,#19959,.T.);
#28294=ORIENTED_EDGE('',*,*,#19960,.T.);
#28295=ORIENTED_EDGE('',*,*,#19961,.T.);
#28296=ORIENTED_EDGE('',*,*,#19962,.T.);
#28297=ORIENTED_EDGE('',*,*,#19864,.T.);
#28298=ORIENTED_EDGE('',*,*,#19881,.T.);
#28299=ORIENTED_EDGE('',*,*,#19963,.T.);
#28300=ORIENTED_EDGE('',*,*,#19964,.T.);
#28301=ORIENTED_EDGE('',*,*,#19965,.T.);
#28302=ORIENTED_EDGE('',*,*,#19966,.T.);
#28303=ORIENTED_EDGE('',*,*,#19967,.T.);
#28304=ORIENTED_EDGE('',*,*,#19968,.F.);
#28305=ORIENTED_EDGE('',*,*,#19969,.T.);
#28306=ORIENTED_EDGE('',*,*,#19970,.T.);
#28307=ORIENTED_EDGE('',*,*,#19971,.T.);
#28308=ORIENTED_EDGE('',*,*,#19965,.F.);
#28309=ORIENTED_EDGE('',*,*,#19972,.T.);
#28310=ORIENTED_EDGE('',*,*,#19973,.T.);
#28311=ORIENTED_EDGE('',*,*,#19974,.T.);
#28312=ORIENTED_EDGE('',*,*,#19975,.T.);
#28313=ORIENTED_EDGE('',*,*,#19976,.T.);
#28314=ORIENTED_EDGE('',*,*,#19970,.F.);
#28315=ORIENTED_EDGE('',*,*,#19977,.T.);
#28316=ORIENTED_EDGE('',*,*,#19978,.T.);
#28317=ORIENTED_EDGE('',*,*,#19979,.T.);
#28318=ORIENTED_EDGE('',*,*,#19973,.F.);
#28319=ORIENTED_EDGE('',*,*,#19980,.T.);
#28320=ORIENTED_EDGE('',*,*,#19981,.T.);
#28321=ORIENTED_EDGE('',*,*,#19982,.T.);
#28322=ORIENTED_EDGE('',*,*,#19983,.T.);
#28323=ORIENTED_EDGE('',*,*,#19984,.T.);
#28324=ORIENTED_EDGE('',*,*,#19978,.F.);
#28325=ORIENTED_EDGE('',*,*,#19985,.T.);
#28326=ORIENTED_EDGE('',*,*,#19951,.T.);
#28327=ORIENTED_EDGE('',*,*,#19986,.T.);
#28328=ORIENTED_EDGE('',*,*,#19981,.F.);
#28329=ORIENTED_EDGE('',*,*,#19806,.T.);
#28330=ORIENTED_EDGE('',*,*,#19987,.T.);
#28331=ORIENTED_EDGE('',*,*,#19988,.F.);
#28332=ORIENTED_EDGE('',*,*,#19839,.T.);
#28333=ORIENTED_EDGE('',*,*,#19989,.T.);
#28334=ORIENTED_EDGE('',*,*,#19990,.F.);
#28335=ORIENTED_EDGE('',*,*,#19987,.F.);
#28336=ORIENTED_EDGE('',*,*,#19991,.T.);
#28337=ORIENTED_EDGE('',*,*,#19988,.T.);
#28338=ORIENTED_EDGE('',*,*,#19992,.F.);
#28339=ORIENTED_EDGE('',*,*,#19993,.F.);
#28340=ORIENTED_EDGE('',*,*,#19991,.F.);
#28341=ORIENTED_EDGE('',*,*,#19994,.F.);
#28342=ORIENTED_EDGE('',*,*,#19995,.F.);
#28343=ORIENTED_EDGE('',*,*,#19996,.F.);
#28344=ORIENTED_EDGE('',*,*,#19997,.F.);
#28345=ORIENTED_EDGE('',*,*,#19998,.T.);
#28346=ORIENTED_EDGE('',*,*,#19999,.F.);
#28347=ORIENTED_EDGE('',*,*,#19772,.T.);
#28348=ORIENTED_EDGE('',*,*,#19807,.T.);
#28349=ORIENTED_EDGE('',*,*,#19998,.F.);
#28350=ORIENTED_EDGE('',*,*,#20000,.F.);
#28351=ORIENTED_EDGE('',*,*,#20001,.T.);
#28352=ORIENTED_EDGE('',*,*,#20002,.F.);
#28353=ORIENTED_EDGE('',*,*,#20003,.F.);
#28354=ORIENTED_EDGE('',*,*,#20001,.F.);
#28355=ORIENTED_EDGE('',*,*,#20004,.F.);
#28356=ORIENTED_EDGE('',*,*,#20005,.T.);
#28357=ORIENTED_EDGE('',*,*,#20005,.F.);
#28358=ORIENTED_EDGE('',*,*,#20006,.F.);
#28359=ORIENTED_EDGE('',*,*,#20007,.T.);
#28360=ORIENTED_EDGE('',*,*,#20008,.F.);
#28361=ORIENTED_EDGE('',*,*,#20009,.F.);
#28362=ORIENTED_EDGE('',*,*,#20007,.F.);
#28363=ORIENTED_EDGE('',*,*,#20010,.F.);
#28364=ORIENTED_EDGE('',*,*,#20011,.T.);
#28365=ORIENTED_EDGE('',*,*,#20012,.F.);
#28366=ORIENTED_EDGE('',*,*,#20013,.F.);
#28367=ORIENTED_EDGE('',*,*,#19996,.T.);
#28368=ORIENTED_EDGE('',*,*,#20014,.F.);
#28369=ORIENTED_EDGE('',*,*,#20011,.F.);
#28370=ORIENTED_EDGE('',*,*,#20015,.F.);
#28371=ORIENTED_EDGE('',*,*,#20016,.T.);
#28372=ORIENTED_EDGE('',*,*,#20017,.F.);
#28373=ORIENTED_EDGE('',*,*,#20016,.F.);
#28374=ORIENTED_EDGE('',*,*,#20018,.F.);
#28375=ORIENTED_EDGE('',*,*,#20012,.T.);
#28376=ORIENTED_EDGE('',*,*,#20019,.F.);
#28377=ORIENTED_EDGE('',*,*,#20020,.T.);
#28378=ORIENTED_EDGE('',*,*,#20021,.T.);
#28379=ORIENTED_EDGE('',*,*,#20022,.F.);
#28380=ORIENTED_EDGE('',*,*,#20023,.F.);
#28381=ORIENTED_EDGE('',*,*,#20024,.T.);
#28382=ORIENTED_EDGE('',*,*,#20025,.T.);
#28383=ORIENTED_EDGE('',*,*,#20026,.F.);
#28384=ORIENTED_EDGE('',*,*,#20027,.F.);
#28385=ORIENTED_EDGE('',*,*,#20028,.T.);
#28386=ORIENTED_EDGE('',*,*,#20027,.T.);
#28387=ORIENTED_EDGE('',*,*,#20029,.F.);
#28388=ORIENTED_EDGE('',*,*,#20030,.F.);
#28389=ORIENTED_EDGE('',*,*,#20031,.T.);
#28390=ORIENTED_EDGE('',*,*,#20030,.T.);
#28391=ORIENTED_EDGE('',*,*,#20032,.F.);
#28392=ORIENTED_EDGE('',*,*,#20033,.F.);
#28393=ORIENTED_EDGE('',*,*,#20034,.T.);
#28394=ORIENTED_EDGE('',*,*,#20033,.T.);
#28395=ORIENTED_EDGE('',*,*,#20035,.F.);
#28396=ORIENTED_EDGE('',*,*,#20036,.F.);
#28397=ORIENTED_EDGE('',*,*,#20037,.T.);
#28398=ORIENTED_EDGE('',*,*,#20036,.T.);
#28399=ORIENTED_EDGE('',*,*,#20038,.F.);
#28400=ORIENTED_EDGE('',*,*,#20039,.F.);
#28401=ORIENTED_EDGE('',*,*,#20040,.T.);
#28402=ORIENTED_EDGE('',*,*,#20041,.T.);
#28403=ORIENTED_EDGE('',*,*,#20042,.F.);
#28404=ORIENTED_EDGE('',*,*,#20025,.F.);
#28405=ORIENTED_EDGE('',*,*,#20043,.T.);
#28406=ORIENTED_EDGE('',*,*,#20039,.T.);
#28407=ORIENTED_EDGE('',*,*,#20044,.F.);
#28408=ORIENTED_EDGE('',*,*,#20045,.F.);
#28409=ORIENTED_EDGE('',*,*,#20046,.T.);
#28410=ORIENTED_EDGE('',*,*,#20045,.T.);
#28411=ORIENTED_EDGE('',*,*,#20047,.F.);
#28412=ORIENTED_EDGE('',*,*,#20041,.F.);
#28413=ORIENTED_EDGE('',*,*,#20048,.T.);
#28414=ORIENTED_EDGE('',*,*,#20049,.T.);
#28415=ORIENTED_EDGE('',*,*,#20050,.F.);
#28416=ORIENTED_EDGE('',*,*,#20051,.F.);
#28417=ORIENTED_EDGE('',*,*,#20052,.T.);
#28418=ORIENTED_EDGE('',*,*,#20053,.T.);
#28419=ORIENTED_EDGE('',*,*,#20054,.F.);
#28420=ORIENTED_EDGE('',*,*,#19983,.F.);
#28421=ORIENTED_EDGE('',*,*,#20053,.F.);
#28422=ORIENTED_EDGE('',*,*,#20055,.F.);
#28423=ORIENTED_EDGE('',*,*,#20049,.F.);
#28424=ORIENTED_EDGE('',*,*,#20056,.T.);
#28425=ORIENTED_EDGE('',*,*,#20057,.T.);
#28426=ORIENTED_EDGE('',*,*,#20058,.T.);
#28427=ORIENTED_EDGE('',*,*,#20059,.T.);
#28428=ORIENTED_EDGE('',*,*,#20060,.F.);
#28429=ORIENTED_EDGE('',*,*,#19974,.F.);
#28430=ORIENTED_EDGE('',*,*,#20061,.T.);
#28431=ORIENTED_EDGE('',*,*,#20062,.T.);
#28432=ORIENTED_EDGE('',*,*,#20058,.F.);
#28433=ORIENTED_EDGE('',*,*,#19979,.F.);
#28434=ORIENTED_EDGE('',*,*,#20054,.T.);
#28435=ORIENTED_EDGE('',*,*,#20063,.T.);
#28436=ORIENTED_EDGE('',*,*,#20061,.F.);
#28437=ORIENTED_EDGE('',*,*,#19984,.F.);
#28438=ORIENTED_EDGE('',*,*,#20059,.F.);
#28439=ORIENTED_EDGE('',*,*,#20062,.F.);
#28440=ORIENTED_EDGE('',*,*,#20063,.F.);
#28441=ORIENTED_EDGE('',*,*,#20057,.F.);
#28442=ORIENTED_EDGE('',*,*,#20064,.T.);
#28443=ORIENTED_EDGE('',*,*,#20065,.T.);
#28444=ORIENTED_EDGE('',*,*,#20066,.F.);
#28445=ORIENTED_EDGE('',*,*,#20067,.T.);
#28446=ORIENTED_EDGE('',*,*,#20051,.T.);
#28447=ORIENTED_EDGE('',*,*,#20068,.F.);
#28448=ORIENTED_EDGE('',*,*,#20069,.F.);
#28449=ORIENTED_EDGE('',*,*,#20070,.T.);
#28450=ORIENTED_EDGE('',*,*,#20071,.T.);
#28451=ORIENTED_EDGE('',*,*,#20072,.F.);
#28452=ORIENTED_EDGE('',*,*,#20065,.F.);
#28453=ORIENTED_EDGE('',*,*,#20073,.T.);
#28454=ORIENTED_EDGE('',*,*,#20069,.T.);
#28455=ORIENTED_EDGE('',*,*,#20074,.F.);
#28456=ORIENTED_EDGE('',*,*,#20071,.F.);
#28457=ORIENTED_EDGE('',*,*,#20075,.T.);
#28458=ORIENTED_EDGE('',*,*,#20076,.T.);
#28459=ORIENTED_EDGE('',*,*,#20077,.F.);
#28460=ORIENTED_EDGE('',*,*,#19966,.F.);
#28461=ORIENTED_EDGE('',*,*,#20078,.T.);
#28462=ORIENTED_EDGE('',*,*,#20079,.T.);
#28463=ORIENTED_EDGE('',*,*,#20075,.F.);
#28464=ORIENTED_EDGE('',*,*,#19971,.F.);
#28465=ORIENTED_EDGE('',*,*,#20080,.T.);
#28466=ORIENTED_EDGE('',*,*,#20081,.T.);
#28467=ORIENTED_EDGE('',*,*,#20078,.F.);
#28468=ORIENTED_EDGE('',*,*,#19976,.F.);
#28469=ORIENTED_EDGE('',*,*,#20076,.F.);
#28470=ORIENTED_EDGE('',*,*,#20079,.F.);
#28471=ORIENTED_EDGE('',*,*,#20081,.F.);
#28472=ORIENTED_EDGE('',*,*,#20082,.T.);
#28473=ORIENTED_EDGE('',*,*,#20083,.T.);
#28474=ORIENTED_EDGE('',*,*,#20084,.F.);
#28475=ORIENTED_EDGE('',*,*,#20085,.F.);
#28476=ORIENTED_EDGE('',*,*,#20086,.T.);
#28477=ORIENTED_EDGE('',*,*,#20087,.T.);
#28478=ORIENTED_EDGE('',*,*,#20085,.T.);
#28479=ORIENTED_EDGE('',*,*,#20088,.F.);
#28480=ORIENTED_EDGE('',*,*,#20089,.F.);
#28481=ORIENTED_EDGE('',*,*,#20090,.T.);
#28482=ORIENTED_EDGE('',*,*,#20089,.T.);
#28483=ORIENTED_EDGE('',*,*,#20091,.F.);
#28484=ORIENTED_EDGE('',*,*,#20092,.F.);
#28485=ORIENTED_EDGE('',*,*,#20093,.T.);
#28486=ORIENTED_EDGE('',*,*,#20092,.T.);
#28487=ORIENTED_EDGE('',*,*,#20094,.F.);
#28488=ORIENTED_EDGE('',*,*,#20095,.F.);
#28489=ORIENTED_EDGE('',*,*,#20096,.T.);
#28490=ORIENTED_EDGE('',*,*,#20095,.T.);
#28491=ORIENTED_EDGE('',*,*,#20097,.F.);
#28492=ORIENTED_EDGE('',*,*,#20098,.F.);
#28493=ORIENTED_EDGE('',*,*,#20099,.T.);
#28494=ORIENTED_EDGE('',*,*,#20100,.T.);
#28495=ORIENTED_EDGE('',*,*,#20101,.F.);
#28496=ORIENTED_EDGE('',*,*,#20083,.F.);
#28497=ORIENTED_EDGE('',*,*,#20102,.T.);
#28498=ORIENTED_EDGE('',*,*,#20098,.T.);
#28499=ORIENTED_EDGE('',*,*,#20103,.F.);
#28500=ORIENTED_EDGE('',*,*,#20104,.F.);
#28501=ORIENTED_EDGE('',*,*,#20105,.T.);
#28502=ORIENTED_EDGE('',*,*,#20104,.T.);
#28503=ORIENTED_EDGE('',*,*,#20106,.F.);
#28504=ORIENTED_EDGE('',*,*,#20100,.F.);
#28505=ORIENTED_EDGE('',*,*,#20107,.T.);
#28506=ORIENTED_EDGE('',*,*,#20108,.T.);
#28507=ORIENTED_EDGE('',*,*,#20109,.F.);
#28508=ORIENTED_EDGE('',*,*,#20110,.F.);
#28509=ORIENTED_EDGE('',*,*,#20111,.T.);
#28510=ORIENTED_EDGE('',*,*,#20112,.F.);
#28511=ORIENTED_EDGE('',*,*,#20113,.F.);
#28512=ORIENTED_EDGE('',*,*,#19934,.T.);
#28513=ORIENTED_EDGE('',*,*,#20114,.F.);
#28514=ORIENTED_EDGE('',*,*,#20115,.F.);
#28515=ORIENTED_EDGE('',*,*,#20116,.T.);
#28516=ORIENTED_EDGE('',*,*,#20117,.T.);
#28517=ORIENTED_EDGE('',*,*,#20118,.T.);
#28518=ORIENTED_EDGE('',*,*,#20115,.T.);
#28519=ORIENTED_EDGE('',*,*,#20119,.F.);
#28520=ORIENTED_EDGE('',*,*,#20120,.T.);
#28521=ORIENTED_EDGE('',*,*,#20119,.T.);
#28522=ORIENTED_EDGE('',*,*,#20121,.F.);
#28523=ORIENTED_EDGE('',*,*,#20122,.F.);
#28524=ORIENTED_EDGE('',*,*,#20123,.T.);
#28525=ORIENTED_EDGE('',*,*,#20124,.T.);
#28526=ORIENTED_EDGE('',*,*,#20117,.F.);
#28527=ORIENTED_EDGE('',*,*,#20125,.T.);
#28528=ORIENTED_EDGE('',*,*,#20122,.T.);
#28529=ORIENTED_EDGE('',*,*,#20126,.F.);
#28530=ORIENTED_EDGE('',*,*,#20110,.T.);
#28531=ORIENTED_EDGE('',*,*,#20127,.F.);
#28532=ORIENTED_EDGE('',*,*,#20128,.F.);
#28533=ORIENTED_EDGE('',*,*,#20129,.T.);
#28534=ORIENTED_EDGE('',*,*,#20126,.T.);
#28535=ORIENTED_EDGE('',*,*,#20130,.F.);
#28536=ORIENTED_EDGE('',*,*,#20124,.F.);
#28537=ORIENTED_EDGE('',*,*,#20131,.T.);
#28538=ORIENTED_EDGE('',*,*,#20128,.T.);
#28539=ORIENTED_EDGE('',*,*,#20132,.F.);
#28540=ORIENTED_EDGE('',*,*,#20133,.T.);
#28541=ORIENTED_EDGE('',*,*,#20134,.T.);
#28542=ORIENTED_EDGE('',*,*,#20135,.T.);
#28543=ORIENTED_EDGE('',*,*,#20136,.F.);
#28544=ORIENTED_EDGE('',*,*,#20021,.F.);
#28545=ORIENTED_EDGE('',*,*,#20137,.T.);
#28546=ORIENTED_EDGE('',*,*,#20138,.T.);
#28547=ORIENTED_EDGE('',*,*,#20139,.F.);
#28548=ORIENTED_EDGE('',*,*,#20135,.F.);
#28549=ORIENTED_EDGE('',*,*,#20140,.T.);
#28550=ORIENTED_EDGE('',*,*,#19946,.T.);
#28551=ORIENTED_EDGE('',*,*,#20141,.F.);
#28552=ORIENTED_EDGE('',*,*,#20142,.F.);
#28553=ORIENTED_EDGE('',*,*,#20143,.T.);
#28554=ORIENTED_EDGE('',*,*,#20144,.T.);
#28555=ORIENTED_EDGE('',*,*,#20145,.F.);
#28556=ORIENTED_EDGE('',*,*,#20138,.F.);
#28557=ORIENTED_EDGE('',*,*,#20146,.T.);
#28558=ORIENTED_EDGE('',*,*,#20112,.T.);
#28559=ORIENTED_EDGE('',*,*,#20147,.F.);
#28560=ORIENTED_EDGE('',*,*,#20148,.T.);
#28561=ORIENTED_EDGE('',*,*,#20149,.T.);
#28562=ORIENTED_EDGE('',*,*,#19939,.T.);
#28563=ORIENTED_EDGE('',*,*,#20150,.F.);
#28564=ORIENTED_EDGE('',*,*,#20151,.T.);
#28565=ORIENTED_EDGE('',*,*,#20023,.T.);
#28566=ORIENTED_EDGE('',*,*,#19940,.F.);
#28567=ORIENTED_EDGE('',*,*,#20152,.T.);
#28568=ORIENTED_EDGE('',*,*,#20153,.T.);
#28569=ORIENTED_EDGE('',*,*,#20148,.F.);
#28570=ORIENTED_EDGE('',*,*,#20154,.F.);
#28571=ORIENTED_EDGE('',*,*,#20155,.F.);
#28572=ORIENTED_EDGE('',*,*,#20156,.F.);
#28573=ORIENTED_EDGE('',*,*,#20157,.T.);
#28574=ORIENTED_EDGE('',*,*,#20158,.F.);
#28575=ORIENTED_EDGE('',*,*,#20159,.T.);
#28576=ORIENTED_EDGE('',*,*,#20160,.F.);
#28577=ORIENTED_EDGE('',*,*,#20161,.F.);
#28578=ORIENTED_EDGE('',*,*,#20147,.T.);
#28579=ORIENTED_EDGE('',*,*,#20162,.F.);
#28580=ORIENTED_EDGE('',*,*,#20163,.T.);
#28581=ORIENTED_EDGE('',*,*,#20164,.T.);
#28582=ORIENTED_EDGE('',*,*,#20165,.T.);
#28583=ORIENTED_EDGE('',*,*,#19958,.F.);
#28584=ORIENTED_EDGE('',*,*,#20166,.F.);
#28585=ORIENTED_EDGE('',*,*,#20167,.T.);
#28586=ORIENTED_EDGE('',*,*,#20168,.T.);
#28587=ORIENTED_EDGE('',*,*,#20169,.F.);
#28588=ORIENTED_EDGE('',*,*,#20170,.F.);
#28589=ORIENTED_EDGE('',*,*,#20171,.T.);
#28590=ORIENTED_EDGE('',*,*,#20172,.T.);
#28591=ORIENTED_EDGE('',*,*,#20173,.T.);
#28592=ORIENTED_EDGE('',*,*,#19952,.F.);
#28593=ORIENTED_EDGE('',*,*,#20174,.F.);
#28594=ORIENTED_EDGE('',*,*,#20175,.T.);
#28595=ORIENTED_EDGE('',*,*,#20176,.T.);
#28596=ORIENTED_EDGE('',*,*,#20177,.F.);
#28597=ORIENTED_EDGE('',*,*,#19802,.T.);
#28598=ORIENTED_EDGE('',*,*,#20178,.T.);
#28599=ORIENTED_EDGE('',*,*,#20179,.F.);
#28600=ORIENTED_EDGE('',*,*,#20180,.F.);
#28601=ORIENTED_EDGE('',*,*,#19836,.T.);
#28602=ORIENTED_EDGE('',*,*,#20180,.T.);
#28603=ORIENTED_EDGE('',*,*,#20181,.F.);
#28604=ORIENTED_EDGE('',*,*,#19838,.T.);
#28605=ORIENTED_EDGE('',*,*,#20181,.T.);
#28606=ORIENTED_EDGE('',*,*,#20182,.F.);
#28607=ORIENTED_EDGE('',*,*,#19989,.F.);
#28608=ORIENTED_EDGE('',*,*,#20183,.T.);
#28609=ORIENTED_EDGE('',*,*,#20170,.T.);
#28610=ORIENTED_EDGE('',*,*,#20184,.F.);
#28611=ORIENTED_EDGE('',*,*,#20165,.F.);
#28612=ORIENTED_EDGE('',*,*,#20184,.T.);
#28613=ORIENTED_EDGE('',*,*,#20185,.T.);
#28614=ORIENTED_EDGE('',*,*,#20182,.T.);
#28615=ORIENTED_EDGE('',*,*,#20179,.T.);
#28616=ORIENTED_EDGE('',*,*,#20186,.T.);
#28617=ORIENTED_EDGE('',*,*,#19959,.F.);
#28618=ORIENTED_EDGE('',*,*,#20187,.T.);
#28619=ORIENTED_EDGE('',*,*,#20188,.T.);
#28620=ORIENTED_EDGE('',*,*,#19954,.F.);
#28621=ORIENTED_EDGE('',*,*,#20189,.F.);
#28622=ORIENTED_EDGE('',*,*,#20162,.T.);
#28623=ORIENTED_EDGE('',*,*,#20190,.T.);
#28624=ORIENTED_EDGE('',*,*,#19955,.F.);
#28625=ORIENTED_EDGE('',*,*,#20188,.F.);
#28626=ORIENTED_EDGE('',*,*,#20191,.T.);
#28627=ORIENTED_EDGE('',*,*,#20192,.T.);
#28628=ORIENTED_EDGE('',*,*,#19956,.F.);
#28629=ORIENTED_EDGE('',*,*,#20190,.F.);
#28630=ORIENTED_EDGE('',*,*,#20174,.T.);
#28631=ORIENTED_EDGE('',*,*,#20166,.T.);
#28632=ORIENTED_EDGE('',*,*,#20193,.F.);
#28633=ORIENTED_EDGE('',*,*,#20193,.T.);
#28634=ORIENTED_EDGE('',*,*,#19957,.F.);
#28635=ORIENTED_EDGE('',*,*,#20192,.F.);
#28636=ORIENTED_EDGE('',*,*,#20194,.T.);
#28637=ORIENTED_EDGE('',*,*,#20195,.T.);
#28638=ORIENTED_EDGE('',*,*,#20189,.T.);
#28639=ORIENTED_EDGE('',*,*,#19953,.F.);
#28640=ORIENTED_EDGE('',*,*,#20196,.F.);
#28641=ORIENTED_EDGE('',*,*,#20197,.T.);
#28642=ORIENTED_EDGE('',*,*,#20198,.T.);
#28643=ORIENTED_EDGE('',*,*,#20168,.F.);
#28644=ORIENTED_EDGE('',*,*,#20199,.F.);
#28645=ORIENTED_EDGE('',*,*,#20199,.T.);
#28646=ORIENTED_EDGE('',*,*,#20197,.F.);
#28647=ORIENTED_EDGE('',*,*,#20200,.F.);
#28648=ORIENTED_EDGE('',*,*,#20201,.F.);
#28649=ORIENTED_EDGE('',*,*,#20202,.T.);
#28650=ORIENTED_EDGE('',*,*,#20203,.T.);
#28651=ORIENTED_EDGE('',*,*,#20204,.T.);
#28652=ORIENTED_EDGE('',*,*,#20205,.F.);
#28653=ORIENTED_EDGE('',*,*,#20198,.F.);
#28654=ORIENTED_EDGE('',*,*,#20203,.F.);
#28655=ORIENTED_EDGE('',*,*,#20202,.F.);
#28656=ORIENTED_EDGE('',*,*,#20157,.F.);
#28657=ORIENTED_EDGE('',*,*,#20206,.F.);
#28658=ORIENTED_EDGE('',*,*,#20207,.T.);
#28659=ORIENTED_EDGE('',*,*,#20208,.T.);
#28660=ORIENTED_EDGE('',*,*,#20209,.F.);
#28661=ORIENTED_EDGE('',*,*,#20204,.F.);
#28662=ORIENTED_EDGE('',*,*,#20206,.T.);
#28663=ORIENTED_EDGE('',*,*,#20210,.F.);
#28664=ORIENTED_EDGE('',*,*,#20211,.F.);
#28665=ORIENTED_EDGE('',*,*,#20212,.T.);
#28666=ORIENTED_EDGE('',*,*,#20213,.F.);
#28667=ORIENTED_EDGE('',*,*,#20214,.T.);
#28668=ORIENTED_EDGE('',*,*,#20207,.F.);
#28669=ORIENTED_EDGE('',*,*,#20215,.T.);
#28670=ORIENTED_EDGE('',*,*,#19997,.T.);
#28671=ORIENTED_EDGE('',*,*,#20216,.F.);
#28672=ORIENTED_EDGE('',*,*,#20217,.F.);
#28673=ORIENTED_EDGE('',*,*,#20218,.T.);
#28674=ORIENTED_EDGE('',*,*,#20000,.T.);
#28675=ORIENTED_EDGE('',*,*,#20215,.F.);
#28676=ORIENTED_EDGE('',*,*,#20219,.T.);
#28677=ORIENTED_EDGE('',*,*,#20004,.T.);
#28678=ORIENTED_EDGE('',*,*,#20218,.F.);
#28679=ORIENTED_EDGE('',*,*,#20220,.F.);
#28680=ORIENTED_EDGE('',*,*,#20211,.T.);
#28681=ORIENTED_EDGE('',*,*,#20221,.T.);
#28682=ORIENTED_EDGE('',*,*,#20222,.T.);
#28683=ORIENTED_EDGE('',*,*,#20223,.T.);
#28684=ORIENTED_EDGE('',*,*,#20224,.T.);
#28685=ORIENTED_EDGE('',*,*,#20225,.T.);
#28686=ORIENTED_EDGE('',*,*,#20006,.T.);
#28687=ORIENTED_EDGE('',*,*,#20219,.F.);
#28688=ORIENTED_EDGE('',*,*,#20226,.T.);
#28689=ORIENTED_EDGE('',*,*,#20227,.T.);
#28690=ORIENTED_EDGE('',*,*,#20010,.T.);
#28691=ORIENTED_EDGE('',*,*,#20225,.F.);
#28692=ORIENTED_EDGE('',*,*,#20216,.T.);
#28693=ORIENTED_EDGE('',*,*,#20013,.T.);
#28694=ORIENTED_EDGE('',*,*,#20228,.F.);
#28695=ORIENTED_EDGE('',*,*,#20229,.T.);
#28696=ORIENTED_EDGE('',*,*,#20230,.T.);
#28697=ORIENTED_EDGE('',*,*,#20015,.T.);
#28698=ORIENTED_EDGE('',*,*,#20227,.F.);
#28699=ORIENTED_EDGE('',*,*,#20231,.F.);
#28700=ORIENTED_EDGE('',*,*,#20228,.T.);
#28701=ORIENTED_EDGE('',*,*,#20018,.T.);
#28702=ORIENTED_EDGE('',*,*,#20230,.F.);
#28703=ORIENTED_EDGE('',*,*,#20232,.T.);
#28704=ORIENTED_EDGE('',*,*,#20213,.T.);
#28705=ORIENTED_EDGE('',*,*,#20212,.F.);
#28706=ORIENTED_EDGE('',*,*,#20220,.T.);
#28707=ORIENTED_EDGE('',*,*,#20217,.T.);
#28708=ORIENTED_EDGE('',*,*,#20231,.T.);
#28709=ORIENTED_EDGE('',*,*,#20210,.T.);
#28710=ORIENTED_EDGE('',*,*,#20156,.T.);
#28711=ORIENTED_EDGE('',*,*,#20233,.T.);
#28712=ORIENTED_EDGE('',*,*,#20221,.F.);
#28713=ORIENTED_EDGE('',*,*,#20020,.F.);
#28714=ORIENTED_EDGE('',*,*,#20234,.F.);
#28715=ORIENTED_EDGE('',*,*,#20235,.T.);
#28716=ORIENTED_EDGE('',*,*,#20236,.F.);
#28717=ORIENTED_EDGE('',*,*,#20026,.T.);
#28718=ORIENTED_EDGE('',*,*,#20237,.T.);
#28719=ORIENTED_EDGE('',*,*,#20161,.T.);
#28720=ORIENTED_EDGE('',*,*,#20238,.F.);
#28721=ORIENTED_EDGE('',*,*,#20238,.T.);
#28722=ORIENTED_EDGE('',*,*,#20239,.F.);
#28723=ORIENTED_EDGE('',*,*,#20240,.F.);
#28724=ORIENTED_EDGE('',*,*,#20029,.T.);
#28725=ORIENTED_EDGE('',*,*,#20032,.T.);
#28726=ORIENTED_EDGE('',*,*,#20240,.T.);
#28727=ORIENTED_EDGE('',*,*,#20241,.T.);
#28728=ORIENTED_EDGE('',*,*,#20242,.T.);
#28729=ORIENTED_EDGE('',*,*,#20242,.F.);
#28730=ORIENTED_EDGE('',*,*,#20243,.T.);
#28731=ORIENTED_EDGE('',*,*,#20244,.T.);
#28732=ORIENTED_EDGE('',*,*,#20035,.T.);
#28733=ORIENTED_EDGE('',*,*,#20244,.F.);
#28734=ORIENTED_EDGE('',*,*,#20245,.T.);
#28735=ORIENTED_EDGE('',*,*,#20246,.F.);
#28736=ORIENTED_EDGE('',*,*,#20038,.T.);
#28737=ORIENTED_EDGE('',*,*,#20247,.T.);
#28738=ORIENTED_EDGE('',*,*,#20146,.F.);
#28739=ORIENTED_EDGE('',*,*,#20237,.F.);
#28740=ORIENTED_EDGE('',*,*,#20042,.T.);
#28741=ORIENTED_EDGE('',*,*,#20246,.T.);
#28742=ORIENTED_EDGE('',*,*,#19932,.F.);
#28743=ORIENTED_EDGE('',*,*,#20248,.F.);
#28744=ORIENTED_EDGE('',*,*,#20044,.T.);
#28745=ORIENTED_EDGE('',*,*,#20047,.T.);
#28746=ORIENTED_EDGE('',*,*,#20248,.T.);
#28747=ORIENTED_EDGE('',*,*,#20113,.T.);
#28748=ORIENTED_EDGE('',*,*,#20247,.F.);
#28749=ORIENTED_EDGE('',*,*,#20249,.T.);
#28750=ORIENTED_EDGE('',*,*,#20116,.F.);
#28751=ORIENTED_EDGE('',*,*,#20250,.F.);
#28752=ORIENTED_EDGE('',*,*,#20048,.F.);
#28753=ORIENTED_EDGE('',*,*,#20250,.T.);
#28754=ORIENTED_EDGE('',*,*,#20118,.F.);
#28755=ORIENTED_EDGE('',*,*,#20251,.F.);
#28756=ORIENTED_EDGE('',*,*,#20056,.F.);
#28757=ORIENTED_EDGE('',*,*,#20064,.F.);
#28758=ORIENTED_EDGE('',*,*,#20251,.T.);
#28759=ORIENTED_EDGE('',*,*,#20120,.F.);
#28760=ORIENTED_EDGE('',*,*,#20252,.F.);
#28761=ORIENTED_EDGE('',*,*,#20253,.T.);
#28762=ORIENTED_EDGE('',*,*,#20123,.F.);
#28763=ORIENTED_EDGE('',*,*,#20249,.F.);
#28764=ORIENTED_EDGE('',*,*,#20067,.F.);
#28765=ORIENTED_EDGE('',*,*,#20252,.T.);
#28766=ORIENTED_EDGE('',*,*,#20125,.F.);
#28767=ORIENTED_EDGE('',*,*,#20254,.F.);
#28768=ORIENTED_EDGE('',*,*,#20070,.F.);
#28769=ORIENTED_EDGE('',*,*,#20254,.T.);
#28770=ORIENTED_EDGE('',*,*,#20129,.F.);
#28771=ORIENTED_EDGE('',*,*,#20253,.F.);
#28772=ORIENTED_EDGE('',*,*,#20073,.F.);
#28773=ORIENTED_EDGE('',*,*,#20084,.T.);
#28774=ORIENTED_EDGE('',*,*,#20255,.T.);
#28775=ORIENTED_EDGE('',*,*,#20132,.T.);
#28776=ORIENTED_EDGE('',*,*,#20256,.T.);
#28777=ORIENTED_EDGE('',*,*,#20256,.F.);
#28778=ORIENTED_EDGE('',*,*,#20127,.T.);
#28779=ORIENTED_EDGE('',*,*,#20257,.T.);
#28780=ORIENTED_EDGE('',*,*,#20088,.T.);
#28781=ORIENTED_EDGE('',*,*,#20257,.F.);
#28782=ORIENTED_EDGE('',*,*,#20109,.T.);
#28783=ORIENTED_EDGE('',*,*,#20258,.T.);
#28784=ORIENTED_EDGE('',*,*,#20091,.T.);
#28785=ORIENTED_EDGE('',*,*,#20258,.F.);
#28786=ORIENTED_EDGE('',*,*,#20259,.T.);
#28787=ORIENTED_EDGE('',*,*,#20260,.T.);
#28788=ORIENTED_EDGE('',*,*,#20094,.T.);
#28789=ORIENTED_EDGE('',*,*,#20260,.F.);
#28790=ORIENTED_EDGE('',*,*,#20261,.T.);
#28791=ORIENTED_EDGE('',*,*,#20262,.T.);
#28792=ORIENTED_EDGE('',*,*,#20097,.T.);
#28793=ORIENTED_EDGE('',*,*,#20263,.T.);
#28794=ORIENTED_EDGE('',*,*,#20264,.F.);
#28795=ORIENTED_EDGE('',*,*,#20255,.F.);
#28796=ORIENTED_EDGE('',*,*,#20101,.T.);
#28797=ORIENTED_EDGE('',*,*,#20262,.F.);
#28798=ORIENTED_EDGE('',*,*,#20265,.T.);
#28799=ORIENTED_EDGE('',*,*,#20266,.T.);
#28800=ORIENTED_EDGE('',*,*,#20103,.T.);
#28801=ORIENTED_EDGE('',*,*,#20106,.T.);
#28802=ORIENTED_EDGE('',*,*,#20266,.F.);
#28803=ORIENTED_EDGE('',*,*,#20267,.T.);
#28804=ORIENTED_EDGE('',*,*,#20263,.F.);
#28805=ORIENTED_EDGE('',*,*,#20268,.T.);
#28806=ORIENTED_EDGE('',*,*,#20259,.F.);
#28807=ORIENTED_EDGE('',*,*,#20108,.F.);
#28808=ORIENTED_EDGE('',*,*,#20261,.F.);
#28809=ORIENTED_EDGE('',*,*,#20268,.F.);
#28810=ORIENTED_EDGE('',*,*,#20269,.T.);
#28811=ORIENTED_EDGE('',*,*,#20270,.T.);
#28812=ORIENTED_EDGE('',*,*,#20264,.T.);
#28813=ORIENTED_EDGE('',*,*,#20271,.T.);
#28814=ORIENTED_EDGE('',*,*,#20133,.F.);
#28815=ORIENTED_EDGE('',*,*,#20272,.T.);
#28816=ORIENTED_EDGE('',*,*,#20265,.F.);
#28817=ORIENTED_EDGE('',*,*,#20270,.F.);
#28818=ORIENTED_EDGE('',*,*,#20267,.F.);
#28819=ORIENTED_EDGE('',*,*,#20272,.F.);
#28820=ORIENTED_EDGE('',*,*,#20273,.T.);
#28821=ORIENTED_EDGE('',*,*,#20271,.F.);
#28822=ORIENTED_EDGE('',*,*,#20274,.F.);
#28823=ORIENTED_EDGE('',*,*,#20159,.F.);
#28824=ORIENTED_EDGE('',*,*,#20111,.F.);
#28825=ORIENTED_EDGE('',*,*,#20275,.F.);
#28826=ORIENTED_EDGE('',*,*,#20196,.T.);
#28827=ORIENTED_EDGE('',*,*,#20173,.F.);
#28828=ORIENTED_EDGE('',*,*,#20176,.F.);
#28829=ORIENTED_EDGE('',*,*,#20276,.T.);
#28830=ORIENTED_EDGE('',*,*,#20277,.T.);
#28831=ORIENTED_EDGE('',*,*,#20278,.F.);
#28832=ORIENTED_EDGE('',*,*,#20121,.T.);
#28833=ORIENTED_EDGE('',*,*,#20114,.T.);
#28834=ORIENTED_EDGE('',*,*,#20130,.T.);
#28835=ORIENTED_EDGE('',*,*,#20269,.F.);
#28836=ORIENTED_EDGE('',*,*,#20107,.F.);
#28837=ORIENTED_EDGE('',*,*,#20131,.F.);
#28838=ORIENTED_EDGE('',*,*,#20273,.F.);
#28839=ORIENTED_EDGE('',*,*,#20236,.T.);
#28840=ORIENTED_EDGE('',*,*,#20276,.F.);
#28841=ORIENTED_EDGE('',*,*,#20279,.F.);
#28842=ORIENTED_EDGE('',*,*,#20134,.F.);
#28843=ORIENTED_EDGE('',*,*,#20280,.F.);
#28844=ORIENTED_EDGE('',*,*,#20195,.F.);
#28845=ORIENTED_EDGE('',*,*,#20175,.F.);
#28846=ORIENTED_EDGE('',*,*,#20194,.F.);
#28847=ORIENTED_EDGE('',*,*,#20239,.T.);
#28848=ORIENTED_EDGE('',*,*,#20160,.T.);
#28849=ORIENTED_EDGE('',*,*,#20281,.F.);
#28850=ORIENTED_EDGE('',*,*,#20245,.F.);
#28851=ORIENTED_EDGE('',*,*,#20282,.F.);
#28852=ORIENTED_EDGE('',*,*,#20275,.T.);
#28853=ORIENTED_EDGE('',*,*,#19933,.F.);
#28854=ORIENTED_EDGE('',*,*,#20151,.F.);
#28855=ORIENTED_EDGE('',*,*,#20149,.F.);
#28856=ORIENTED_EDGE('',*,*,#20283,.F.);
#28857=ORIENTED_EDGE('',*,*,#20234,.T.);
#28858=ORIENTED_EDGE('',*,*,#20284,.T.);
#28859=ORIENTED_EDGE('',*,*,#20283,.T.);
#28860=ORIENTED_EDGE('',*,*,#20153,.F.);
#28861=ORIENTED_EDGE('',*,*,#20241,.F.);
#28862=ORIENTED_EDGE('',*,*,#20281,.T.);
#28863=ORIENTED_EDGE('',*,*,#20274,.T.);
#28864=ORIENTED_EDGE('',*,*,#20285,.T.);
#28865=ORIENTED_EDGE('',*,*,#20235,.F.);
#28866=ORIENTED_EDGE('',*,*,#20284,.F.);
#28867=ORIENTED_EDGE('',*,*,#20286,.T.);
#28868=ORIENTED_EDGE('',*,*,#20277,.F.);
#28869=ORIENTED_EDGE('',*,*,#20282,.T.);
#28870=ORIENTED_EDGE('',*,*,#20243,.F.);
#28871=ORIENTED_EDGE('',*,*,#20285,.F.);
#28872=ORIENTED_EDGE('',*,*,#20187,.F.);
#28873=ORIENTED_EDGE('',*,*,#20280,.T.);
#28874=ORIENTED_EDGE('',*,*,#20191,.F.);
#28875=ORIENTED_EDGE('',*,*,#20163,.F.);
#28876=ORIENTED_EDGE('',*,*,#20158,.T.);
#28877=ORIENTED_EDGE('',*,*,#20201,.T.);
#28878=ORIENTED_EDGE('',*,*,#20287,.F.);
#28879=ORIENTED_EDGE('',*,*,#20288,.F.);
#28880=ORIENTED_EDGE('',*,*,#20289,.T.);
#28881=ORIENTED_EDGE('',*,*,#20290,.T.);
#28882=ORIENTED_EDGE('',*,*,#20291,.F.);
#28883=ORIENTED_EDGE('',*,*,#20292,.T.);
#28884=ORIENTED_EDGE('',*,*,#20289,.F.);
#28885=ORIENTED_EDGE('',*,*,#20293,.F.);
#28886=ORIENTED_EDGE('',*,*,#20143,.F.);
#28887=ORIENTED_EDGE('',*,*,#20137,.F.);
#28888=ORIENTED_EDGE('',*,*,#20279,.T.);
#28889=ORIENTED_EDGE('',*,*,#20294,.T.);
#28890=ORIENTED_EDGE('',*,*,#20292,.F.);
#28891=ORIENTED_EDGE('',*,*,#20294,.F.);
#28892=ORIENTED_EDGE('',*,*,#20278,.T.);
#28893=ORIENTED_EDGE('',*,*,#20295,.T.);
#28894=ORIENTED_EDGE('',*,*,#20290,.F.);
#28895=ORIENTED_EDGE('',*,*,#20296,.T.);
#28896=ORIENTED_EDGE('',*,*,#19846,.T.);
#28897=ORIENTED_EDGE('',*,*,#20297,.F.);
#28898=ORIENTED_EDGE('',*,*,#20298,.F.);
#28899=ORIENTED_EDGE('',*,*,#20299,.T.);
#28900=ORIENTED_EDGE('',*,*,#19847,.T.);
#28901=ORIENTED_EDGE('',*,*,#20296,.F.);
#28902=ORIENTED_EDGE('',*,*,#20300,.F.);
#28903=ORIENTED_EDGE('',*,*,#20301,.T.);
#28904=ORIENTED_EDGE('',*,*,#19852,.T.);
#28905=ORIENTED_EDGE('',*,*,#20299,.F.);
#28906=ORIENTED_EDGE('',*,*,#20302,.F.);
#28907=ORIENTED_EDGE('',*,*,#20303,.T.);
#28908=ORIENTED_EDGE('',*,*,#19853,.T.);
#28909=ORIENTED_EDGE('',*,*,#20301,.F.);
#28910=ORIENTED_EDGE('',*,*,#20304,.F.);
#28911=ORIENTED_EDGE('',*,*,#20305,.T.);
#28912=ORIENTED_EDGE('',*,*,#19856,.T.);
#28913=ORIENTED_EDGE('',*,*,#20303,.F.);
#28914=ORIENTED_EDGE('',*,*,#20306,.F.);
#28915=ORIENTED_EDGE('',*,*,#20297,.T.);
#28916=ORIENTED_EDGE('',*,*,#20307,.F.);
#28917=ORIENTED_EDGE('',*,*,#20308,.F.);
#28918=ORIENTED_EDGE('',*,*,#20309,.T.);
#28919=ORIENTED_EDGE('',*,*,#20309,.F.);
#28920=ORIENTED_EDGE('',*,*,#20310,.T.);
#28921=ORIENTED_EDGE('',*,*,#20311,.F.);
#28922=ORIENTED_EDGE('',*,*,#20312,.F.);
#28923=ORIENTED_EDGE('',*,*,#20308,.T.);
#28924=ORIENTED_EDGE('',*,*,#19861,.T.);
#28925=ORIENTED_EDGE('',*,*,#20305,.F.);
#28926=ORIENTED_EDGE('',*,*,#20313,.F.);
#28927=ORIENTED_EDGE('',*,*,#20314,.T.);
#28928=ORIENTED_EDGE('',*,*,#20313,.T.);
#28929=ORIENTED_EDGE('',*,*,#20315,.F.);
#28930=ORIENTED_EDGE('',*,*,#20316,.F.);
#28931=ORIENTED_EDGE('',*,*,#20307,.T.);
#28932=ORIENTED_EDGE('',*,*,#19845,.T.);
#28933=ORIENTED_EDGE('',*,*,#19942,.F.);
#28934=ORIENTED_EDGE('',*,*,#20317,.F.);
#28935=ORIENTED_EDGE('',*,*,#19947,.F.);
#28936=ORIENTED_EDGE('',*,*,#20318,.F.);
#28937=ORIENTED_EDGE('',*,*,#20310,.F.);
#28938=ORIENTED_EDGE('',*,*,#20317,.T.);
#28939=ORIENTED_EDGE('',*,*,#20319,.F.);
#28940=ORIENTED_EDGE('',*,*,#19878,.T.);
#28941=ORIENTED_EDGE('',*,*,#19859,.T.);
#28942=ORIENTED_EDGE('',*,*,#20314,.F.);
#28943=ORIENTED_EDGE('',*,*,#20320,.F.);
#28944=ORIENTED_EDGE('',*,*,#20321,.T.);
#28945=ORIENTED_EDGE('',*,*,#20318,.T.);
#28946=ORIENTED_EDGE('',*,*,#20140,.F.);
#28947=ORIENTED_EDGE('',*,*,#20311,.T.);
#28948=ORIENTED_EDGE('',*,*,#20321,.F.);
#28949=ORIENTED_EDGE('',*,*,#20322,.F.);
#28950=ORIENTED_EDGE('',*,*,#20323,.F.);
#28951=ORIENTED_EDGE('',*,*,#20291,.T.);
#28952=ORIENTED_EDGE('',*,*,#20324,.T.);
#28953=ORIENTED_EDGE('',*,*,#20322,.T.);
#28954=ORIENTED_EDGE('',*,*,#20293,.T.);
#28955=ORIENTED_EDGE('',*,*,#20323,.T.);
#28956=ORIENTED_EDGE('',*,*,#20320,.T.);
#28957=ORIENTED_EDGE('',*,*,#20325,.F.);
#28958=ORIENTED_EDGE('',*,*,#20325,.T.);
#28959=ORIENTED_EDGE('',*,*,#20142,.T.);
#28960=ORIENTED_EDGE('',*,*,#20326,.F.);
#28961=ORIENTED_EDGE('',*,*,#20144,.F.);
#28962=ORIENTED_EDGE('',*,*,#20327,.T.);
#28963=ORIENTED_EDGE('',*,*,#19768,.T.);
#28964=ORIENTED_EDGE('',*,*,#20328,.F.);
#28965=ORIENTED_EDGE('',*,*,#20328,.T.);
#28966=ORIENTED_EDGE('',*,*,#19999,.T.);
#28967=ORIENTED_EDGE('',*,*,#20329,.T.);
#28968=ORIENTED_EDGE('',*,*,#20330,.F.);
#28969=ORIENTED_EDGE('',*,*,#20002,.T.);
#28970=ORIENTED_EDGE('',*,*,#20331,.T.);
#28971=ORIENTED_EDGE('',*,*,#20332,.F.);
#28972=ORIENTED_EDGE('',*,*,#20329,.F.);
#28973=ORIENTED_EDGE('',*,*,#20003,.T.);
#28974=ORIENTED_EDGE('',*,*,#20333,.T.);
#28975=ORIENTED_EDGE('',*,*,#20334,.F.);
#28976=ORIENTED_EDGE('',*,*,#20331,.F.);
#28977=ORIENTED_EDGE('',*,*,#20008,.T.);
#28978=ORIENTED_EDGE('',*,*,#20335,.T.);
#28979=ORIENTED_EDGE('',*,*,#20336,.F.);
#28980=ORIENTED_EDGE('',*,*,#20333,.F.);
#28981=ORIENTED_EDGE('',*,*,#20009,.T.);
#28982=ORIENTED_EDGE('',*,*,#20337,.T.);
#28983=ORIENTED_EDGE('',*,*,#20338,.F.);
#28984=ORIENTED_EDGE('',*,*,#20335,.F.);
#28985=ORIENTED_EDGE('',*,*,#20339,.F.);
#28986=ORIENTED_EDGE('',*,*,#20340,.F.);
#28987=ORIENTED_EDGE('',*,*,#20014,.T.);
#28988=ORIENTED_EDGE('',*,*,#19995,.T.);
#28989=ORIENTED_EDGE('',*,*,#20340,.T.);
#28990=ORIENTED_EDGE('',*,*,#20341,.F.);
#28991=ORIENTED_EDGE('',*,*,#20342,.F.);
#28992=ORIENTED_EDGE('',*,*,#20017,.T.);
#28993=ORIENTED_EDGE('',*,*,#20343,.T.);
#28994=ORIENTED_EDGE('',*,*,#20344,.F.);
#28995=ORIENTED_EDGE('',*,*,#20337,.F.);
#28996=ORIENTED_EDGE('',*,*,#20019,.T.);
#28997=ORIENTED_EDGE('',*,*,#20342,.T.);
#28998=ORIENTED_EDGE('',*,*,#20345,.F.);
#28999=ORIENTED_EDGE('',*,*,#20343,.F.);
#29000=ORIENTED_EDGE('',*,*,#20346,.T.);
#29001=ORIENTED_EDGE('',*,*,#19769,.T.);
#29002=ORIENTED_EDGE('',*,*,#20327,.F.);
#29003=ORIENTED_EDGE('',*,*,#20347,.F.);
#29004=ORIENTED_EDGE('',*,*,#20348,.T.);
#29005=ORIENTED_EDGE('',*,*,#19775,.T.);
#29006=ORIENTED_EDGE('',*,*,#20346,.F.);
#29007=ORIENTED_EDGE('',*,*,#20349,.F.);
#29008=ORIENTED_EDGE('',*,*,#20350,.T.);
#29009=ORIENTED_EDGE('',*,*,#20351,.T.);
#29010=ORIENTED_EDGE('',*,*,#19960,.F.);
#29011=ORIENTED_EDGE('',*,*,#20352,.F.);
#29012=ORIENTED_EDGE('',*,*,#20353,.T.);
#29013=ORIENTED_EDGE('',*,*,#20352,.T.);
#29014=ORIENTED_EDGE('',*,*,#20186,.F.);
#29015=ORIENTED_EDGE('',*,*,#20178,.F.);
#29016=ORIENTED_EDGE('',*,*,#19805,.F.);
#29017=ORIENTED_EDGE('',*,*,#20354,.T.);
#29018=ORIENTED_EDGE('',*,*,#20355,.T.);
#29019=ORIENTED_EDGE('',*,*,#20350,.F.);
#29020=ORIENTED_EDGE('',*,*,#20353,.F.);
#29021=ORIENTED_EDGE('',*,*,#20356,.T.);
#29022=ORIENTED_EDGE('',*,*,#19862,.F.);
#29023=ORIENTED_EDGE('',*,*,#19962,.F.);
#29024=ORIENTED_EDGE('',*,*,#20357,.F.);
#29025=ORIENTED_EDGE('',*,*,#20358,.F.);
#29026=ORIENTED_EDGE('',*,*,#19943,.T.);
#29027=ORIENTED_EDGE('',*,*,#19843,.T.);
#29028=ORIENTED_EDGE('',*,*,#20356,.F.);
#29029=ORIENTED_EDGE('',*,*,#20359,.T.);
#29030=ORIENTED_EDGE('',*,*,#19993,.T.);
#29031=ORIENTED_EDGE('',*,*,#20360,.F.);
#29032=ORIENTED_EDGE('',*,*,#20361,.F.);
#29033=ORIENTED_EDGE('',*,*,#20362,.F.);
#29034=ORIENTED_EDGE('',*,*,#20339,.T.);
#29035=ORIENTED_EDGE('',*,*,#19994,.T.);
#29036=ORIENTED_EDGE('',*,*,#20359,.F.);
#29037=ORIENTED_EDGE('',*,*,#20363,.T.);
#29038=ORIENTED_EDGE('',*,*,#20357,.T.);
#29039=ORIENTED_EDGE('',*,*,#19961,.F.);
#29040=ORIENTED_EDGE('',*,*,#20351,.F.);
#29041=ORIENTED_EDGE('',*,*,#20364,.T.);
#29042=ORIENTED_EDGE('',*,*,#19783,.F.);
#29043=ORIENTED_EDGE('',*,*,#20365,.F.);
#29044=ORIENTED_EDGE('',*,*,#20366,.T.);
#29045=ORIENTED_EDGE('',*,*,#20367,.T.);
#29046=ORIENTED_EDGE('',*,*,#20368,.T.);
#29047=ORIENTED_EDGE('',*,*,#20369,.F.);
#29048=ORIENTED_EDGE('',*,*,#19799,.F.);
#29049=ORIENTED_EDGE('',*,*,#20369,.T.);
#29050=ORIENTED_EDGE('',*,*,#20370,.T.);
#29051=ORIENTED_EDGE('',*,*,#20354,.F.);
#29052=ORIENTED_EDGE('',*,*,#19804,.F.);
#29053=ORIENTED_EDGE('',*,*,#20370,.F.);
#29054=ORIENTED_EDGE('',*,*,#20368,.F.);
#29055=ORIENTED_EDGE('',*,*,#20371,.T.);
#29056=ORIENTED_EDGE('',*,*,#20372,.T.);
#29057=ORIENTED_EDGE('',*,*,#20373,.F.);
#29058=ORIENTED_EDGE('',*,*,#20374,.T.);
#29059=ORIENTED_EDGE('',*,*,#20375,.T.);
#29060=ORIENTED_EDGE('',*,*,#20376,.F.);
#29061=ORIENTED_EDGE('',*,*,#20372,.F.);
#29062=ORIENTED_EDGE('',*,*,#20377,.T.);
#29063=ORIENTED_EDGE('',*,*,#20378,.T.);
#29064=ORIENTED_EDGE('',*,*,#20379,.F.);
#29065=ORIENTED_EDGE('',*,*,#20375,.F.);
#29066=ORIENTED_EDGE('',*,*,#20380,.T.);
#29067=ORIENTED_EDGE('',*,*,#20381,.T.);
#29068=ORIENTED_EDGE('',*,*,#20382,.F.);
#29069=ORIENTED_EDGE('',*,*,#20378,.F.);
#29070=ORIENTED_EDGE('',*,*,#20383,.T.);
#29071=ORIENTED_EDGE('',*,*,#20384,.T.);
#29072=ORIENTED_EDGE('',*,*,#20385,.F.);
#29073=ORIENTED_EDGE('',*,*,#20381,.F.);
#29074=ORIENTED_EDGE('',*,*,#20386,.T.);
#29075=ORIENTED_EDGE('',*,*,#20387,.T.);
#29076=ORIENTED_EDGE('',*,*,#20388,.F.);
#29077=ORIENTED_EDGE('',*,*,#20384,.F.);
#29078=ORIENTED_EDGE('',*,*,#20389,.T.);
#29079=ORIENTED_EDGE('',*,*,#19776,.T.);
#29080=ORIENTED_EDGE('',*,*,#20348,.F.);
#29081=ORIENTED_EDGE('',*,*,#20390,.F.);
#29082=ORIENTED_EDGE('',*,*,#19777,.T.);
#29083=ORIENTED_EDGE('',*,*,#20389,.F.);
#29084=ORIENTED_EDGE('',*,*,#20391,.F.);
#29085=ORIENTED_EDGE('',*,*,#20391,.T.);
#29086=ORIENTED_EDGE('',*,*,#20390,.T.);
#29087=ORIENTED_EDGE('',*,*,#20392,.F.);
#29088=ORIENTED_EDGE('',*,*,#20387,.F.);
#29089=ORIENTED_EDGE('',*,*,#20393,.T.);
#29090=ORIENTED_EDGE('',*,*,#19782,.F.);
#29091=ORIENTED_EDGE('',*,*,#19821,.T.);
#29092=ORIENTED_EDGE('',*,*,#20394,.T.);
#29093=ORIENTED_EDGE('',*,*,#20395,.T.);
#29094=ORIENTED_EDGE('',*,*,#20396,.T.);
#29095=ORIENTED_EDGE('',*,*,#20365,.T.);
#29096=ORIENTED_EDGE('',*,*,#20396,.F.);
#29097=ORIENTED_EDGE('',*,*,#20397,.T.);
#29098=ORIENTED_EDGE('',*,*,#20398,.T.);
#29099=ORIENTED_EDGE('',*,*,#20366,.F.);
#29100=ORIENTED_EDGE('',*,*,#20398,.F.);
#29101=ORIENTED_EDGE('',*,*,#20399,.T.);
#29102=ORIENTED_EDGE('',*,*,#19786,.F.);
#29103=ORIENTED_EDGE('',*,*,#19826,.T.);
#29104=ORIENTED_EDGE('',*,*,#19780,.T.);
#29105=ORIENTED_EDGE('',*,*,#20364,.F.);
#29106=ORIENTED_EDGE('',*,*,#20400,.T.);
#29107=ORIENTED_EDGE('',*,*,#20401,.T.);
#29108=ORIENTED_EDGE('',*,*,#20367,.F.);
#29109=ORIENTED_EDGE('',*,*,#19798,.F.);
#29110=ORIENTED_EDGE('',*,*,#20402,.T.);
#29111=ORIENTED_EDGE('',*,*,#20403,.F.);
#29112=ORIENTED_EDGE('',*,*,#20371,.F.);
#29113=ORIENTED_EDGE('',*,*,#20401,.F.);
#29114=ORIENTED_EDGE('',*,*,#20403,.T.);
#29115=ORIENTED_EDGE('',*,*,#20404,.F.);
#29116=ORIENTED_EDGE('',*,*,#20405,.F.);
#29117=ORIENTED_EDGE('',*,*,#20374,.F.);
#29118=ORIENTED_EDGE('',*,*,#20377,.F.);
#29119=ORIENTED_EDGE('',*,*,#20405,.T.);
#29120=ORIENTED_EDGE('',*,*,#20406,.T.);
#29121=ORIENTED_EDGE('',*,*,#20407,.F.);
#29122=ORIENTED_EDGE('',*,*,#20407,.T.);
#29123=ORIENTED_EDGE('',*,*,#20408,.F.);
#29124=ORIENTED_EDGE('',*,*,#20409,.F.);
#29125=ORIENTED_EDGE('',*,*,#20380,.F.);
#29126=ORIENTED_EDGE('',*,*,#20383,.F.);
#29127=ORIENTED_EDGE('',*,*,#20409,.T.);
#29128=ORIENTED_EDGE('',*,*,#20410,.T.);
#29129=ORIENTED_EDGE('',*,*,#20411,.F.);
#29130=ORIENTED_EDGE('',*,*,#20411,.T.);
#29131=ORIENTED_EDGE('',*,*,#20412,.F.);
#29132=ORIENTED_EDGE('',*,*,#20413,.F.);
#29133=ORIENTED_EDGE('',*,*,#20386,.F.);
#29134=ORIENTED_EDGE('',*,*,#20414,.T.);
#29135=ORIENTED_EDGE('',*,*,#20415,.F.);
#29136=ORIENTED_EDGE('',*,*,#19815,.T.);
#29137=ORIENTED_EDGE('',*,*,#19778,.F.);
#29138=ORIENTED_EDGE('',*,*,#20393,.F.);
#29139=ORIENTED_EDGE('',*,*,#20413,.T.);
#29140=ORIENTED_EDGE('',*,*,#20394,.F.);
#29141=ORIENTED_EDGE('',*,*,#19818,.T.);
#29142=ORIENTED_EDGE('',*,*,#20415,.T.);
#29143=ORIENTED_EDGE('',*,*,#20416,.T.);
#29144=ORIENTED_EDGE('',*,*,#20417,.T.);
#29145=ORIENTED_EDGE('',*,*,#20416,.F.);
#29146=ORIENTED_EDGE('',*,*,#20418,.F.);
#29147=ORIENTED_EDGE('',*,*,#20419,.T.);
#29148=ORIENTED_EDGE('',*,*,#20420,.F.);
#29149=ORIENTED_EDGE('',*,*,#20395,.F.);
#29150=ORIENTED_EDGE('',*,*,#20417,.F.);
#29151=ORIENTED_EDGE('',*,*,#20420,.T.);
#29152=ORIENTED_EDGE('',*,*,#20421,.T.);
#29153=ORIENTED_EDGE('',*,*,#20422,.F.);
#29154=ORIENTED_EDGE('',*,*,#20397,.F.);
#29155=ORIENTED_EDGE('',*,*,#20423,.T.);
#29156=ORIENTED_EDGE('',*,*,#20424,.F.);
#29157=ORIENTED_EDGE('',*,*,#19787,.F.);
#29158=ORIENTED_EDGE('',*,*,#20399,.F.);
#29159=ORIENTED_EDGE('',*,*,#20422,.T.);
#29160=ORIENTED_EDGE('',*,*,#20425,.T.);
#29161=ORIENTED_EDGE('',*,*,#20423,.F.);
#29162=ORIENTED_EDGE('',*,*,#20426,.T.);
#29163=ORIENTED_EDGE('',*,*,#20427,.T.);
#29164=ORIENTED_EDGE('',*,*,#20400,.F.);
#29165=ORIENTED_EDGE('',*,*,#20428,.T.);
#29166=ORIENTED_EDGE('',*,*,#20429,.F.);
#29167=ORIENTED_EDGE('',*,*,#20402,.F.);
#29168=ORIENTED_EDGE('',*,*,#20427,.F.);
#29169=ORIENTED_EDGE('',*,*,#20404,.T.);
#29170=ORIENTED_EDGE('',*,*,#20429,.T.);
#29171=ORIENTED_EDGE('',*,*,#20430,.F.);
#29172=ORIENTED_EDGE('',*,*,#20406,.F.);
#29173=ORIENTED_EDGE('',*,*,#20430,.T.);
#29174=ORIENTED_EDGE('',*,*,#20431,.T.);
#29175=ORIENTED_EDGE('',*,*,#20432,.F.);
#29176=ORIENTED_EDGE('',*,*,#20408,.T.);
#29177=ORIENTED_EDGE('',*,*,#20432,.T.);
#29178=ORIENTED_EDGE('',*,*,#20433,.F.);
#29179=ORIENTED_EDGE('',*,*,#20434,.T.);
#29180=ORIENTED_EDGE('',*,*,#20435,.F.);
#29181=ORIENTED_EDGE('',*,*,#20410,.F.);
#29182=ORIENTED_EDGE('',*,*,#20433,.T.);
#29183=ORIENTED_EDGE('',*,*,#20412,.T.);
#29184=ORIENTED_EDGE('',*,*,#20435,.T.);
#29185=ORIENTED_EDGE('',*,*,#20436,.F.);
#29186=ORIENTED_EDGE('',*,*,#20437,.T.);
#29187=ORIENTED_EDGE('',*,*,#20418,.T.);
#29188=ORIENTED_EDGE('',*,*,#20414,.F.);
#29189=ORIENTED_EDGE('',*,*,#20436,.T.);
#29190=ORIENTED_EDGE('',*,*,#20424,.T.);
#29191=ORIENTED_EDGE('',*,*,#20438,.T.);
#29192=ORIENTED_EDGE('',*,*,#20439,.F.);
#29193=ORIENTED_EDGE('',*,*,#19790,.F.);
#29194=ORIENTED_EDGE('',*,*,#20439,.T.);
#29195=ORIENTED_EDGE('',*,*,#20440,.T.);
#29196=ORIENTED_EDGE('',*,*,#20441,.F.);
#29197=ORIENTED_EDGE('',*,*,#19791,.F.);
#29198=ORIENTED_EDGE('',*,*,#20441,.T.);
#29199=ORIENTED_EDGE('',*,*,#20442,.T.);
#29200=ORIENTED_EDGE('',*,*,#20443,.F.);
#29201=ORIENTED_EDGE('',*,*,#19796,.F.);
#29202=ORIENTED_EDGE('',*,*,#20443,.T.);
#29203=ORIENTED_EDGE('',*,*,#20444,.T.);
#29204=ORIENTED_EDGE('',*,*,#20426,.F.);
#29205=ORIENTED_EDGE('',*,*,#19797,.F.);
#29206=ORIENTED_EDGE('',*,*,#20425,.F.);
#29207=ORIENTED_EDGE('',*,*,#20421,.F.);
#29208=ORIENTED_EDGE('',*,*,#20419,.F.);
#29209=ORIENTED_EDGE('',*,*,#20437,.F.);
#29210=ORIENTED_EDGE('',*,*,#20434,.F.);
#29211=ORIENTED_EDGE('',*,*,#20431,.F.);
#29212=ORIENTED_EDGE('',*,*,#20428,.F.);
#29213=ORIENTED_EDGE('',*,*,#20444,.F.);
#29214=ORIENTED_EDGE('',*,*,#20442,.F.);
#29215=ORIENTED_EDGE('',*,*,#20440,.F.);
#29216=ORIENTED_EDGE('',*,*,#20438,.F.);
#29217=ORIENTED_EDGE('',*,*,#20445,.T.);
#29218=ORIENTED_EDGE('',*,*,#20446,.F.);
#29219=ORIENTED_EDGE('',*,*,#20447,.F.);
#29220=ORIENTED_EDGE('',*,*,#20448,.T.);
#29221=ORIENTED_EDGE('',*,*,#20449,.T.);
#29222=ORIENTED_EDGE('',*,*,#20450,.T.);
#29223=ORIENTED_EDGE('',*,*,#20451,.T.);
#29224=ORIENTED_EDGE('',*,*,#20447,.T.);
#29225=ORIENTED_EDGE('',*,*,#20452,.F.);
#29226=ORIENTED_EDGE('',*,*,#20453,.F.);
#29227=ORIENTED_EDGE('',*,*,#20453,.T.);
#29228=ORIENTED_EDGE('',*,*,#20454,.F.);
#29229=ORIENTED_EDGE('',*,*,#20455,.F.);
#29230=ORIENTED_EDGE('',*,*,#20456,.T.);
#29231=ORIENTED_EDGE('',*,*,#20457,.F.);
#29232=ORIENTED_EDGE('',*,*,#20458,.F.);
#29233=ORIENTED_EDGE('',*,*,#20459,.F.);
#29234=ORIENTED_EDGE('',*,*,#20460,.T.);
#29235=ORIENTED_EDGE('',*,*,#20461,.F.);
#29236=ORIENTED_EDGE('',*,*,#20462,.F.);
#29237=ORIENTED_EDGE('',*,*,#20463,.F.);
#29238=ORIENTED_EDGE('',*,*,#20464,.T.);
#29239=ORIENTED_EDGE('',*,*,#20465,.F.);
#29240=ORIENTED_EDGE('',*,*,#20464,.F.);
#29241=ORIENTED_EDGE('',*,*,#20466,.F.);
#29242=ORIENTED_EDGE('',*,*,#20467,.F.);
#29243=ORIENTED_EDGE('',*,*,#20467,.T.);
#29244=ORIENTED_EDGE('',*,*,#20468,.F.);
#29245=ORIENTED_EDGE('',*,*,#20469,.F.);
#29246=ORIENTED_EDGE('',*,*,#20470,.F.);
#29247=ORIENTED_EDGE('',*,*,#20471,.F.);
#29248=ORIENTED_EDGE('',*,*,#20469,.T.);
#29249=ORIENTED_EDGE('',*,*,#20472,.F.);
#29250=ORIENTED_EDGE('',*,*,#20473,.F.);
#29251=ORIENTED_EDGE('',*,*,#20473,.T.);
#29252=ORIENTED_EDGE('',*,*,#20474,.F.);
#29253=ORIENTED_EDGE('',*,*,#20475,.F.);
#29254=ORIENTED_EDGE('',*,*,#20476,.F.);
#29255=ORIENTED_EDGE('',*,*,#20477,.F.);
#29256=ORIENTED_EDGE('',*,*,#20478,.F.);
#29257=ORIENTED_EDGE('',*,*,#20479,.F.);
#29258=ORIENTED_EDGE('',*,*,#20480,.F.);
#29259=ORIENTED_EDGE('',*,*,#20475,.T.);
#29260=ORIENTED_EDGE('',*,*,#20481,.F.);
#29261=ORIENTED_EDGE('',*,*,#20482,.T.);
#29262=ORIENTED_EDGE('',*,*,#20483,.F.);
#29263=ORIENTED_EDGE('',*,*,#20484,.T.);
#29264=ORIENTED_EDGE('',*,*,#20485,.T.);
#29265=ORIENTED_EDGE('',*,*,#20486,.T.);
#29266=ORIENTED_EDGE('',*,*,#20487,.T.);
#29267=ORIENTED_EDGE('',*,*,#20446,.T.);
#29268=ORIENTED_EDGE('',*,*,#20484,.F.);
#29269=ORIENTED_EDGE('',*,*,#20488,.T.);
#29270=ORIENTED_EDGE('',*,*,#20452,.T.);
#29271=ORIENTED_EDGE('',*,*,#20487,.F.);
#29272=ORIENTED_EDGE('',*,*,#20489,.F.);
#29273=ORIENTED_EDGE('',*,*,#20490,.T.);
#29274=ORIENTED_EDGE('',*,*,#20454,.T.);
#29275=ORIENTED_EDGE('',*,*,#20488,.F.);
#29276=ORIENTED_EDGE('',*,*,#20491,.T.);
#29277=ORIENTED_EDGE('',*,*,#20492,.T.);
#29278=ORIENTED_EDGE('',*,*,#20490,.F.);
#29279=ORIENTED_EDGE('',*,*,#20493,.F.);
#29280=ORIENTED_EDGE('',*,*,#20494,.T.);
#29281=ORIENTED_EDGE('',*,*,#20495,.T.);
#29282=ORIENTED_EDGE('',*,*,#20491,.F.);
#29283=ORIENTED_EDGE('',*,*,#20496,.F.);
#29284=ORIENTED_EDGE('',*,*,#20497,.T.);
#29285=ORIENTED_EDGE('',*,*,#20498,.T.);
#29286=ORIENTED_EDGE('',*,*,#20494,.F.);
#29287=ORIENTED_EDGE('',*,*,#20499,.F.);
#29288=ORIENTED_EDGE('',*,*,#20500,.T.);
#29289=ORIENTED_EDGE('',*,*,#20459,.T.);
#29290=ORIENTED_EDGE('',*,*,#20497,.F.);
#29291=ORIENTED_EDGE('',*,*,#20501,.F.);
#29292=ORIENTED_EDGE('',*,*,#20502,.T.);
#29293=ORIENTED_EDGE('',*,*,#20503,.T.);
#29294=ORIENTED_EDGE('',*,*,#20500,.F.);
#29295=ORIENTED_EDGE('',*,*,#20504,.F.);
#29296=ORIENTED_EDGE('',*,*,#20505,.T.);
#29297=ORIENTED_EDGE('',*,*,#20463,.T.);
#29298=ORIENTED_EDGE('',*,*,#20502,.F.);
#29299=ORIENTED_EDGE('',*,*,#20506,.F.);
#29300=ORIENTED_EDGE('',*,*,#20507,.T.);
#29301=ORIENTED_EDGE('',*,*,#20466,.T.);
#29302=ORIENTED_EDGE('',*,*,#20505,.F.);
#29303=ORIENTED_EDGE('',*,*,#20508,.F.);
#29304=ORIENTED_EDGE('',*,*,#20509,.T.);
#29305=ORIENTED_EDGE('',*,*,#20468,.T.);
#29306=ORIENTED_EDGE('',*,*,#20507,.F.);
#29307=ORIENTED_EDGE('',*,*,#20510,.T.);
#29308=ORIENTED_EDGE('',*,*,#20472,.T.);
#29309=ORIENTED_EDGE('',*,*,#20509,.F.);
#29310=ORIENTED_EDGE('',*,*,#20511,.F.);
#29311=ORIENTED_EDGE('',*,*,#20512,.T.);
#29312=ORIENTED_EDGE('',*,*,#20474,.T.);
#29313=ORIENTED_EDGE('',*,*,#20510,.F.);
#29314=ORIENTED_EDGE('',*,*,#20481,.T.);
#29315=ORIENTED_EDGE('',*,*,#20512,.F.);
#29316=ORIENTED_EDGE('',*,*,#20513,.F.);
#29317=ORIENTED_EDGE('',*,*,#20514,.T.);
#29318=ORIENTED_EDGE('',*,*,#20513,.T.);
#29319=ORIENTED_EDGE('',*,*,#20511,.T.);
#29320=ORIENTED_EDGE('',*,*,#20508,.T.);
#29321=ORIENTED_EDGE('',*,*,#20506,.T.);
#29322=ORIENTED_EDGE('',*,*,#20504,.T.);
#29323=ORIENTED_EDGE('',*,*,#20501,.T.);
#29324=ORIENTED_EDGE('',*,*,#20499,.T.);
#29325=ORIENTED_EDGE('',*,*,#20496,.T.);
#29326=ORIENTED_EDGE('',*,*,#20493,.T.);
#29327=ORIENTED_EDGE('',*,*,#20489,.T.);
#29328=ORIENTED_EDGE('',*,*,#20483,.T.);
#29329=ORIENTED_EDGE('',*,*,#20515,.T.);
#29330=ORIENTED_EDGE('',*,*,#20516,.T.);
#29331=ORIENTED_EDGE('',*,*,#20517,.T.);
#29332=ORIENTED_EDGE('',*,*,#20518,.T.);
#29333=ORIENTED_EDGE('',*,*,#20519,.T.);
#29334=ORIENTED_EDGE('',*,*,#20520,.T.);
#29335=ORIENTED_EDGE('',*,*,#20521,.T.);
#29336=ORIENTED_EDGE('',*,*,#20522,.F.);
#29337=ORIENTED_EDGE('',*,*,#20523,.F.);
#29338=ORIENTED_EDGE('',*,*,#20523,.T.);
#29339=ORIENTED_EDGE('',*,*,#20524,.F.);
#29340=ORIENTED_EDGE('',*,*,#20525,.F.);
#29341=ORIENTED_EDGE('',*,*,#20526,.T.);
#29342=ORIENTED_EDGE('',*,*,#20527,.T.);
#29343=ORIENTED_EDGE('',*,*,#20525,.T.);
#29344=ORIENTED_EDGE('',*,*,#20528,.F.);
#29345=ORIENTED_EDGE('',*,*,#20529,.F.);
#29346=ORIENTED_EDGE('',*,*,#20529,.T.);
#29347=ORIENTED_EDGE('',*,*,#20530,.F.);
#29348=ORIENTED_EDGE('',*,*,#20531,.F.);
#29349=ORIENTED_EDGE('',*,*,#20532,.T.);
#29350=ORIENTED_EDGE('',*,*,#20531,.T.);
#29351=ORIENTED_EDGE('',*,*,#20533,.F.);
#29352=ORIENTED_EDGE('',*,*,#20534,.T.);
#29353=ORIENTED_EDGE('',*,*,#20535,.T.);
#29354=ORIENTED_EDGE('',*,*,#20536,.T.);
#29355=ORIENTED_EDGE('',*,*,#20534,.F.);
#29356=ORIENTED_EDGE('',*,*,#20537,.F.);
#29357=ORIENTED_EDGE('',*,*,#20538,.T.);
#29358=ORIENTED_EDGE('',*,*,#20539,.T.);
#29359=ORIENTED_EDGE('',*,*,#20540,.F.);
#29360=ORIENTED_EDGE('',*,*,#20521,.F.);
#29361=ORIENTED_EDGE('',*,*,#20541,.F.);
#29362=ORIENTED_EDGE('',*,*,#20542,.T.);
#29363=ORIENTED_EDGE('',*,*,#20522,.T.);
#29364=ORIENTED_EDGE('',*,*,#20543,.F.);
#29365=ORIENTED_EDGE('',*,*,#20544,.F.);
#29366=ORIENTED_EDGE('',*,*,#20545,.T.);
#29367=ORIENTED_EDGE('',*,*,#20524,.T.);
#29368=ORIENTED_EDGE('',*,*,#20542,.F.);
#29369=ORIENTED_EDGE('',*,*,#20546,.T.);
#29370=ORIENTED_EDGE('',*,*,#20528,.T.);
#29371=ORIENTED_EDGE('',*,*,#20545,.F.);
#29372=ORIENTED_EDGE('',*,*,#20547,.F.);
#29373=ORIENTED_EDGE('',*,*,#20548,.T.);
#29374=ORIENTED_EDGE('',*,*,#20530,.T.);
#29375=ORIENTED_EDGE('',*,*,#20546,.F.);
#29376=ORIENTED_EDGE('',*,*,#20549,.T.);
#29377=ORIENTED_EDGE('',*,*,#20533,.T.);
#29378=ORIENTED_EDGE('',*,*,#20548,.F.);
#29379=ORIENTED_EDGE('',*,*,#20550,.F.);
#29380=ORIENTED_EDGE('',*,*,#20551,.T.);
#29381=ORIENTED_EDGE('',*,*,#20537,.T.);
#29382=ORIENTED_EDGE('',*,*,#20549,.F.);
#29383=ORIENTED_EDGE('',*,*,#20552,.F.);
#29384=ORIENTED_EDGE('',*,*,#19876,.T.);
#29385=ORIENTED_EDGE('',*,*,#20553,.T.);
#29386=ORIENTED_EDGE('',*,*,#20554,.F.);
#29387=ORIENTED_EDGE('',*,*,#20555,.T.);
#29388=ORIENTED_EDGE('',*,*,#20551,.F.);
#29389=ORIENTED_EDGE('',*,*,#20556,.F.);
#29390=ORIENTED_EDGE('',*,*,#20554,.T.);
#29391=ORIENTED_EDGE('',*,*,#20543,.T.);
#29392=ORIENTED_EDGE('',*,*,#20540,.T.);
#29393=ORIENTED_EDGE('',*,*,#20557,.F.);
#29394=ORIENTED_EDGE('',*,*,#20558,.T.);
#29395=ORIENTED_EDGE('',*,*,#20559,.F.);
#29396=ORIENTED_EDGE('',*,*,#19880,.F.);
#29397=ORIENTED_EDGE('',*,*,#20560,.F.);
#29398=ORIENTED_EDGE('',*,*,#20557,.T.);
#29399=ORIENTED_EDGE('',*,*,#20561,.T.);
#29400=ORIENTED_EDGE('',*,*,#20558,.F.);
#29401=ORIENTED_EDGE('',*,*,#20556,.T.);
#29402=ORIENTED_EDGE('',*,*,#20552,.T.);
#29403=ORIENTED_EDGE('',*,*,#20550,.T.);
#29404=ORIENTED_EDGE('',*,*,#20547,.T.);
#29405=ORIENTED_EDGE('',*,*,#20544,.T.);
#29406=ORIENTED_EDGE('',*,*,#20560,.T.);
#29407=ORIENTED_EDGE('',*,*,#19882,.F.);
#29408=ORIENTED_EDGE('',*,*,#19865,.F.);
#29409=ORIENTED_EDGE('',*,*,#19869,.F.);
#29410=ORIENTED_EDGE('',*,*,#19872,.F.);
#29411=ORIENTED_EDGE('',*,*,#19874,.F.);
#29412=ORIENTED_EDGE('',*,*,#19877,.F.);
#29413=ORIENTED_EDGE('',*,*,#20562,.T.);
#29414=ORIENTED_EDGE('',*,*,#20563,.F.);
#29415=ORIENTED_EDGE('',*,*,#20564,.T.);
#29416=ORIENTED_EDGE('',*,*,#20565,.T.);
#29417=ORIENTED_EDGE('',*,*,#20566,.F.);
#29418=ORIENTED_EDGE('',*,*,#20567,.T.);
#29419=ORIENTED_EDGE('',*,*,#20568,.T.);
#29420=ORIENTED_EDGE('',*,*,#20569,.F.);
#29421=ORIENTED_EDGE('',*,*,#20570,.F.);
#29422=ORIENTED_EDGE('',*,*,#20571,.T.);
#29423=ORIENTED_EDGE('',*,*,#20572,.F.);
#29424=ORIENTED_EDGE('',*,*,#20573,.F.);
#29425=ORIENTED_EDGE('',*,*,#20574,.F.);
#29426=ORIENTED_EDGE('',*,*,#20575,.F.);
#29427=ORIENTED_EDGE('',*,*,#20576,.T.);
#29428=ORIENTED_EDGE('',*,*,#20577,.T.);
#29429=ORIENTED_EDGE('',*,*,#20574,.T.);
#29430=ORIENTED_EDGE('',*,*,#20578,.T.);
#29431=ORIENTED_EDGE('',*,*,#20564,.F.);
#29432=ORIENTED_EDGE('',*,*,#20579,.T.);
#29433=ORIENTED_EDGE('',*,*,#20565,.F.);
#29434=ORIENTED_EDGE('',*,*,#20580,.T.);
#29435=ORIENTED_EDGE('',*,*,#20581,.T.);
#29436=ORIENTED_EDGE('',*,*,#20566,.T.);
#29437=ORIENTED_EDGE('',*,*,#20562,.F.);
#29438=ORIENTED_EDGE('',*,*,#20582,.F.);
#29439=ORIENTED_EDGE('',*,*,#20583,.T.);
#29440=ORIENTED_EDGE('',*,*,#20567,.F.);
#29441=ORIENTED_EDGE('',*,*,#20584,.F.);
#29442=ORIENTED_EDGE('',*,*,#20585,.T.);
#29443=ORIENTED_EDGE('',*,*,#20570,.T.);
#29444=ORIENTED_EDGE('',*,*,#20568,.F.);
#29445=ORIENTED_EDGE('',*,*,#20586,.F.);
#29446=ORIENTED_EDGE('',*,*,#20587,.T.);
#29447=ORIENTED_EDGE('',*,*,#20588,.F.);
#29448=ORIENTED_EDGE('',*,*,#20571,.F.);
#29449=ORIENTED_EDGE('',*,*,#20589,.F.);
#29450=ORIENTED_EDGE('',*,*,#20572,.T.);
#29451=ORIENTED_EDGE('',*,*,#20590,.T.);
#29452=ORIENTED_EDGE('',*,*,#20576,.F.);
#29453=ORIENTED_EDGE('',*,*,#20591,.T.);
#29454=ORIENTED_EDGE('',*,*,#20592,.F.);
#29455=ORIENTED_EDGE('',*,*,#20577,.F.);
#29456=ORIENTED_EDGE('',*,*,#20593,.T.);
#29457=ORIENTED_EDGE('',*,*,#20594,.T.);
#29458=ORIENTED_EDGE('',*,*,#20580,.F.);
#29459=ORIENTED_EDGE('',*,*,#20578,.F.);
#29460=ORIENTED_EDGE('',*,*,#20592,.T.);
#29461=ORIENTED_EDGE('',*,*,#20595,.T.);
#29462=ORIENTED_EDGE('',*,*,#20596,.T.);
#29463=ORIENTED_EDGE('',*,*,#20597,.F.);
#29464=ORIENTED_EDGE('',*,*,#20581,.F.);
#29465=ORIENTED_EDGE('',*,*,#20598,.T.);
#29466=ORIENTED_EDGE('',*,*,#20584,.T.);
#29467=ORIENTED_EDGE('',*,*,#20582,.T.);
#29468=ORIENTED_EDGE('',*,*,#20579,.F.);
#29469=ORIENTED_EDGE('',*,*,#20599,.T.);
#29470=ORIENTED_EDGE('',*,*,#20600,.T.);
#29471=ORIENTED_EDGE('',*,*,#20601,.F.);
#29472=ORIENTED_EDGE('',*,*,#20585,.F.);
#29473=ORIENTED_EDGE('',*,*,#20602,.T.);
#29474=ORIENTED_EDGE('',*,*,#20589,.T.);
#29475=ORIENTED_EDGE('',*,*,#20586,.T.);
#29476=ORIENTED_EDGE('',*,*,#20583,.F.);
#29477=ORIENTED_EDGE('',*,*,#20603,.T.);
#29478=ORIENTED_EDGE('',*,*,#20604,.T.);
#29479=ORIENTED_EDGE('',*,*,#20605,.F.);
#29480=ORIENTED_EDGE('',*,*,#20587,.F.);
#29481=ORIENTED_EDGE('',*,*,#20606,.T.);
#29482=ORIENTED_EDGE('',*,*,#20593,.F.);
#29483=ORIENTED_EDGE('',*,*,#20590,.F.);
#29484=ORIENTED_EDGE('',*,*,#20588,.T.);
#29485=ORIENTED_EDGE('',*,*,#20607,.T.);
#29486=ORIENTED_EDGE('',*,*,#20608,.T.);
#29487=ORIENTED_EDGE('',*,*,#20609,.F.);
#29488=ORIENTED_EDGE('',*,*,#20591,.F.);
#29489=ORIENTED_EDGE('',*,*,#20609,.T.);
#29490=ORIENTED_EDGE('',*,*,#20610,.T.);
#29491=ORIENTED_EDGE('',*,*,#20595,.F.);
#29492=ORIENTED_EDGE('',*,*,#20594,.F.);
#29493=ORIENTED_EDGE('',*,*,#20611,.T.);
#29494=ORIENTED_EDGE('',*,*,#20612,.F.);
#29495=ORIENTED_EDGE('',*,*,#20613,.F.);
#29496=ORIENTED_EDGE('',*,*,#20597,.T.);
#29497=ORIENTED_EDGE('',*,*,#20614,.T.);
#29498=ORIENTED_EDGE('',*,*,#20599,.F.);
#29499=ORIENTED_EDGE('',*,*,#20598,.F.);
#29500=ORIENTED_EDGE('',*,*,#20601,.T.);
#29501=ORIENTED_EDGE('',*,*,#20615,.T.);
#29502=ORIENTED_EDGE('',*,*,#20603,.F.);
#29503=ORIENTED_EDGE('',*,*,#20602,.F.);
#29504=ORIENTED_EDGE('',*,*,#20605,.T.);
#29505=ORIENTED_EDGE('',*,*,#20616,.T.);
#29506=ORIENTED_EDGE('',*,*,#20607,.F.);
#29507=ORIENTED_EDGE('',*,*,#20606,.F.);
#29508=ORIENTED_EDGE('',*,*,#20617,.T.);
#29509=ORIENTED_EDGE('',*,*,#19938,.T.);
#29510=ORIENTED_EDGE('',*,*,#20618,.F.);
#29511=ORIENTED_EDGE('',*,*,#20619,.F.);
#29512=ORIENTED_EDGE('',*,*,#20620,.F.);
#29513=ORIENTED_EDGE('',*,*,#20621,.T.);
#29514=ORIENTED_EDGE('',*,*,#20618,.T.);
#29515=ORIENTED_EDGE('',*,*,#20563,.T.);
#29516=ORIENTED_EDGE('',*,*,#20569,.T.);
#29517=ORIENTED_EDGE('',*,*,#20573,.T.);
#29518=ORIENTED_EDGE('',*,*,#20575,.T.);
#29519=ORIENTED_EDGE('',*,*,#20622,.T.);
#29520=ORIENTED_EDGE('',*,*,#20623,.T.);
#29521=ORIENTED_EDGE('',*,*,#20519,.F.);
#29522=ORIENTED_EDGE('',*,*,#20624,.F.);
#29523=ORIENTED_EDGE('',*,*,#20625,.F.);
#29524=ORIENTED_EDGE('',*,*,#20626,.T.);
#29525=ORIENTED_EDGE('',*,*,#20627,.T.);
#29526=ORIENTED_EDGE('',*,*,#20622,.F.);
#29527=ORIENTED_EDGE('',*,*,#20628,.T.);
#29528=ORIENTED_EDGE('',*,*,#20629,.T.);
#29529=ORIENTED_EDGE('',*,*,#20630,.T.);
#29530=ORIENTED_EDGE('',*,*,#19949,.F.);
#29531=ORIENTED_EDGE('',*,*,#20631,.T.);
#29532=ORIENTED_EDGE('',*,*,#20632,.T.);
#29533=ORIENTED_EDGE('',*,*,#20629,.F.);
#29534=ORIENTED_EDGE('',*,*,#20633,.T.);
#29535=ORIENTED_EDGE('',*,*,#20559,.T.);
#29536=ORIENTED_EDGE('',*,*,#20634,.T.);
#29537=ORIENTED_EDGE('',*,*,#20635,.F.);
#29538=ORIENTED_EDGE('',*,*,#19963,.F.);
#29539=ORIENTED_EDGE('',*,*,#20561,.F.);
#29540=ORIENTED_EDGE('',*,*,#20539,.F.);
#29541=ORIENTED_EDGE('',*,*,#20636,.F.);
#29542=ORIENTED_EDGE('',*,*,#20637,.F.);
#29543=ORIENTED_EDGE('',*,*,#20638,.F.);
#29544=ORIENTED_EDGE('',*,*,#20639,.F.);
#29545=ORIENTED_EDGE('',*,*,#20640,.F.);
#29546=ORIENTED_EDGE('',*,*,#20641,.F.);
#29547=ORIENTED_EDGE('',*,*,#20642,.F.);
#29548=ORIENTED_EDGE('',*,*,#20643,.F.);
#29549=ORIENTED_EDGE('',*,*,#20644,.F.);
#29550=ORIENTED_EDGE('',*,*,#20645,.F.);
#29551=ORIENTED_EDGE('',*,*,#20646,.F.);
#29552=ORIENTED_EDGE('',*,*,#20634,.F.);
#29553=ORIENTED_EDGE('',*,*,#20647,.T.);
#29554=ORIENTED_EDGE('',*,*,#19968,.T.);
#29555=ORIENTED_EDGE('',*,*,#20648,.T.);
#29556=ORIENTED_EDGE('',*,*,#20649,.F.);
#29557=ORIENTED_EDGE('',*,*,#20649,.T.);
#29558=ORIENTED_EDGE('',*,*,#20650,.T.);
#29559=ORIENTED_EDGE('',*,*,#20651,.T.);
#29560=ORIENTED_EDGE('',*,*,#20652,.F.);
#29561=ORIENTED_EDGE('',*,*,#20653,.T.);
#29562=ORIENTED_EDGE('',*,*,#20654,.T.);
#29563=ORIENTED_EDGE('',*,*,#20652,.T.);
#29564=ORIENTED_EDGE('',*,*,#20655,.T.);
#29565=ORIENTED_EDGE('',*,*,#20656,.F.);
#29566=ORIENTED_EDGE('',*,*,#20656,.T.);
#29567=ORIENTED_EDGE('',*,*,#20657,.T.);
#29568=ORIENTED_EDGE('',*,*,#20658,.T.);
#29569=ORIENTED_EDGE('',*,*,#20659,.T.);
#29570=ORIENTED_EDGE('',*,*,#20660,.F.);
#29571=ORIENTED_EDGE('',*,*,#20661,.T.);
#29572=ORIENTED_EDGE('',*,*,#20662,.T.);
#29573=ORIENTED_EDGE('',*,*,#20660,.T.);
#29574=ORIENTED_EDGE('',*,*,#20663,.T.);
#29575=ORIENTED_EDGE('',*,*,#20664,.F.);
#29576=ORIENTED_EDGE('',*,*,#20664,.T.);
#29577=ORIENTED_EDGE('',*,*,#20665,.T.);
#29578=ORIENTED_EDGE('',*,*,#20666,.T.);
#29579=ORIENTED_EDGE('',*,*,#20667,.T.);
#29580=ORIENTED_EDGE('',*,*,#20668,.F.);
#29581=ORIENTED_EDGE('',*,*,#20669,.T.);
#29582=ORIENTED_EDGE('',*,*,#20670,.T.);
#29583=ORIENTED_EDGE('',*,*,#20668,.T.);
#29584=ORIENTED_EDGE('',*,*,#20671,.T.);
#29585=ORIENTED_EDGE('',*,*,#20631,.F.);
#29586=ORIENTED_EDGE('',*,*,#20672,.T.);
#29587=ORIENTED_EDGE('',*,*,#20673,.F.);
#29588=ORIENTED_EDGE('',*,*,#20486,.F.);
#29589=ORIENTED_EDGE('',*,*,#20673,.T.);
#29590=ORIENTED_EDGE('',*,*,#20674,.T.);
#29591=ORIENTED_EDGE('',*,*,#20675,.F.);
#29592=ORIENTED_EDGE('',*,*,#20515,.F.);
#29593=ORIENTED_EDGE('',*,*,#20676,.F.);
#29594=ORIENTED_EDGE('',*,*,#20677,.T.);
#29595=ORIENTED_EDGE('',*,*,#20674,.F.);
#29596=ORIENTED_EDGE('',*,*,#20678,.F.);
#29597=ORIENTED_EDGE('',*,*,#20679,.F.);
#29598=ORIENTED_EDGE('',*,*,#20680,.T.);
#29599=ORIENTED_EDGE('',*,*,#20360,.T.);
#29600=ORIENTED_EDGE('',*,*,#19992,.T.);
#29601=ORIENTED_EDGE('',*,*,#19990,.T.);
#29602=ORIENTED_EDGE('',*,*,#20185,.F.);
#29603=ORIENTED_EDGE('',*,*,#20169,.T.);
#29604=ORIENTED_EDGE('',*,*,#20205,.T.);
#29605=ORIENTED_EDGE('',*,*,#20209,.T.);
#29606=ORIENTED_EDGE('',*,*,#20681,.T.);
#29607=ORIENTED_EDGE('',*,*,#20682,.F.);
#29608=ORIENTED_EDGE('',*,*,#20683,.F.);
#29609=ORIENTED_EDGE('',*,*,#20684,.T.);
#29610=ORIENTED_EDGE('',*,*,#20678,.T.);
#29611=ORIENTED_EDGE('',*,*,#20672,.F.);
#29612=ORIENTED_EDGE('',*,*,#20685,.F.);
#29613=ORIENTED_EDGE('',*,*,#20485,.F.);
#29614=ORIENTED_EDGE('',*,*,#20445,.F.);
#29615=ORIENTED_EDGE('',*,*,#20686,.T.);
#29616=ORIENTED_EDGE('',*,*,#20687,.F.);
#29617=ORIENTED_EDGE('',*,*,#20688,.T.);
#29618=ORIENTED_EDGE('',*,*,#20689,.T.);
#29619=ORIENTED_EDGE('',*,*,#20690,.T.);
#29620=ORIENTED_EDGE('',*,*,#20691,.T.);
#29621=ORIENTED_EDGE('',*,*,#20685,.T.);
#29622=ORIENTED_EDGE('',*,*,#20692,.T.);
#29623=ORIENTED_EDGE('',*,*,#20693,.F.);
#29624=ORIENTED_EDGE('',*,*,#20694,.T.);
#29625=ORIENTED_EDGE('',*,*,#20687,.T.);
#29626=ORIENTED_EDGE('',*,*,#20695,.F.);
#29627=ORIENTED_EDGE('',*,*,#20696,.T.);
#29628=ORIENTED_EDGE('',*,*,#20693,.T.);
#29629=ORIENTED_EDGE('',*,*,#20697,.T.);
#29630=ORIENTED_EDGE('',*,*,#20698,.T.);
#29631=ORIENTED_EDGE('',*,*,#20699,.F.);
#29632=ORIENTED_EDGE('',*,*,#20700,.T.);
#29633=ORIENTED_EDGE('',*,*,#20695,.T.);
#29634=ORIENTED_EDGE('',*,*,#20701,.F.);
#29635=ORIENTED_EDGE('',*,*,#20702,.T.);
#29636=ORIENTED_EDGE('',*,*,#20699,.T.);
#29637=ORIENTED_EDGE('',*,*,#20703,.T.);
#29638=ORIENTED_EDGE('',*,*,#20704,.T.);
#29639=ORIENTED_EDGE('',*,*,#20689,.F.);
#29640=ORIENTED_EDGE('',*,*,#20705,.T.);
#29641=ORIENTED_EDGE('',*,*,#20706,.T.);
#29642=ORIENTED_EDGE('',*,*,#20707,.T.);
#29643=ORIENTED_EDGE('',*,*,#20708,.F.);
#29644=ORIENTED_EDGE('',*,*,#20709,.T.);
#29645=ORIENTED_EDGE('',*,*,#20701,.T.);
#29646=ORIENTED_EDGE('',*,*,#20710,.T.);
#29647=ORIENTED_EDGE('',*,*,#20706,.F.);
#29648=ORIENTED_EDGE('',*,*,#20711,.T.);
#29649=ORIENTED_EDGE('',*,*,#20708,.T.);
#29650=ORIENTED_EDGE('',*,*,#20712,.T.);
#29651=ORIENTED_EDGE('',*,*,#20713,.T.);
#29652=ORIENTED_EDGE('',*,*,#20714,.F.);
#29653=ORIENTED_EDGE('',*,*,#20715,.F.);
#29654=ORIENTED_EDGE('',*,*,#20716,.T.);
#29655=ORIENTED_EDGE('',*,*,#20717,.T.);
#29656=ORIENTED_EDGE('',*,*,#20718,.F.);
#29657=ORIENTED_EDGE('',*,*,#20719,.F.);
#29658=ORIENTED_EDGE('',*,*,#20720,.T.);
#29659=ORIENTED_EDGE('',*,*,#20721,.T.);
#29660=ORIENTED_EDGE('',*,*,#20716,.F.);
#29661=ORIENTED_EDGE('',*,*,#20722,.F.);
#29662=ORIENTED_EDGE('',*,*,#20723,.T.);
#29663=ORIENTED_EDGE('',*,*,#20724,.T.);
#29664=ORIENTED_EDGE('',*,*,#20720,.F.);
#29665=ORIENTED_EDGE('',*,*,#20725,.F.);
#29666=ORIENTED_EDGE('',*,*,#20726,.T.);
#29667=ORIENTED_EDGE('',*,*,#20727,.T.);
#29668=ORIENTED_EDGE('',*,*,#20723,.F.);
#29669=ORIENTED_EDGE('',*,*,#20728,.F.);
#29670=ORIENTED_EDGE('',*,*,#20729,.T.);
#29671=ORIENTED_EDGE('',*,*,#20730,.T.);
#29672=ORIENTED_EDGE('',*,*,#20726,.F.);
#29673=ORIENTED_EDGE('',*,*,#20731,.F.);
#29674=ORIENTED_EDGE('',*,*,#20718,.T.);
#29675=ORIENTED_EDGE('',*,*,#20732,.T.);
#29676=ORIENTED_EDGE('',*,*,#20733,.F.);
#29677=ORIENTED_EDGE('',*,*,#20734,.F.);
#29678=ORIENTED_EDGE('',*,*,#20735,.T.);
#29679=ORIENTED_EDGE('',*,*,#20736,.T.);
#29680=ORIENTED_EDGE('',*,*,#20729,.F.);
#29681=ORIENTED_EDGE('',*,*,#20737,.F.);
#29682=ORIENTED_EDGE('',*,*,#20733,.T.);
#29683=ORIENTED_EDGE('',*,*,#20738,.T.);
#29684=ORIENTED_EDGE('',*,*,#20735,.F.);
#29685=ORIENTED_EDGE('',*,*,#20739,.F.);
#29686=ORIENTED_EDGE('',*,*,#20740,.T.);
#29687=ORIENTED_EDGE('',*,*,#20741,.T.);
#29688=ORIENTED_EDGE('',*,*,#20742,.F.);
#29689=ORIENTED_EDGE('',*,*,#20743,.F.);
#29690=ORIENTED_EDGE('',*,*,#20744,.T.);
#29691=ORIENTED_EDGE('',*,*,#20745,.T.);
#29692=ORIENTED_EDGE('',*,*,#20746,.F.);
#29693=ORIENTED_EDGE('',*,*,#20666,.F.);
#29694=ORIENTED_EDGE('',*,*,#20747,.F.);
#29695=ORIENTED_EDGE('',*,*,#20748,.F.);
#29696=ORIENTED_EDGE('',*,*,#20742,.T.);
#29697=ORIENTED_EDGE('',*,*,#20749,.T.);
#29698=ORIENTED_EDGE('',*,*,#20745,.F.);
#29699=ORIENTED_EDGE('',*,*,#20750,.T.);
#29700=ORIENTED_EDGE('',*,*,#20751,.T.);
#29701=ORIENTED_EDGE('',*,*,#20752,.F.);
#29702=ORIENTED_EDGE('',*,*,#20659,.F.);
#29703=ORIENTED_EDGE('',*,*,#20752,.T.);
#29704=ORIENTED_EDGE('',*,*,#20753,.T.);
#29705=ORIENTED_EDGE('',*,*,#20754,.F.);
#29706=ORIENTED_EDGE('',*,*,#20663,.F.);
#29707=ORIENTED_EDGE('',*,*,#20754,.T.);
#29708=ORIENTED_EDGE('',*,*,#20755,.T.);
#29709=ORIENTED_EDGE('',*,*,#20744,.F.);
#29710=ORIENTED_EDGE('',*,*,#20665,.F.);
#29711=ORIENTED_EDGE('',*,*,#20756,.T.);
#29712=ORIENTED_EDGE('',*,*,#20757,.F.);
#29713=ORIENTED_EDGE('',*,*,#20758,.F.);
#29714=ORIENTED_EDGE('',*,*,#20747,.T.);
#29715=ORIENTED_EDGE('',*,*,#20755,.F.);
#29716=ORIENTED_EDGE('',*,*,#20753,.F.);
#29717=ORIENTED_EDGE('',*,*,#20751,.F.);
#29718=ORIENTED_EDGE('',*,*,#20759,.T.);
#29719=ORIENTED_EDGE('',*,*,#20760,.T.);
#29720=ORIENTED_EDGE('',*,*,#20740,.F.);
#29721=ORIENTED_EDGE('',*,*,#20761,.F.);
#29722=ORIENTED_EDGE('',*,*,#20757,.T.);
#29723=ORIENTED_EDGE('',*,*,#20762,.T.);
#29724=ORIENTED_EDGE('',*,*,#20763,.F.);
#29725=ORIENTED_EDGE('',*,*,#20764,.F.);
#29726=ORIENTED_EDGE('',*,*,#20763,.T.);
#29727=ORIENTED_EDGE('',*,*,#20765,.T.);
#29728=ORIENTED_EDGE('',*,*,#20759,.F.);
#29729=ORIENTED_EDGE('',*,*,#20766,.F.);
#29730=ORIENTED_EDGE('',*,*,#20767,.T.);
#29731=ORIENTED_EDGE('',*,*,#20768,.T.);
#29732=ORIENTED_EDGE('',*,*,#20769,.F.);
#29733=ORIENTED_EDGE('',*,*,#20651,.F.);
#29734=ORIENTED_EDGE('',*,*,#20769,.T.);
#29735=ORIENTED_EDGE('',*,*,#20770,.T.);
#29736=ORIENTED_EDGE('',*,*,#20771,.F.);
#29737=ORIENTED_EDGE('',*,*,#20655,.F.);
#29738=ORIENTED_EDGE('',*,*,#20771,.T.);
#29739=ORIENTED_EDGE('',*,*,#20772,.T.);
#29740=ORIENTED_EDGE('',*,*,#20773,.F.);
#29741=ORIENTED_EDGE('',*,*,#20657,.F.);
#29742=ORIENTED_EDGE('',*,*,#20774,.F.);
#29743=ORIENTED_EDGE('',*,*,#20775,.T.);
#29744=ORIENTED_EDGE('',*,*,#20776,.T.);
#29745=ORIENTED_EDGE('',*,*,#20777,.F.);
#29746=ORIENTED_EDGE('',*,*,#20778,.F.);
#29747=ORIENTED_EDGE('',*,*,#20772,.F.);
#29748=ORIENTED_EDGE('',*,*,#20770,.F.);
#29749=ORIENTED_EDGE('',*,*,#20768,.F.);
#29750=ORIENTED_EDGE('',*,*,#20779,.T.);
#29751=ORIENTED_EDGE('',*,*,#20780,.T.);
#29752=ORIENTED_EDGE('',*,*,#20775,.F.);
#29753=ORIENTED_EDGE('',*,*,#20781,.F.);
#29754=ORIENTED_EDGE('',*,*,#20782,.T.);
#29755=ORIENTED_EDGE('',*,*,#20783,.T.);
#29756=ORIENTED_EDGE('',*,*,#20779,.F.);
#29757=ORIENTED_EDGE('',*,*,#20784,.F.);
#29758=ORIENTED_EDGE('',*,*,#20785,.T.);
#29759=ORIENTED_EDGE('',*,*,#20786,.T.);
#29760=ORIENTED_EDGE('',*,*,#20782,.F.);
#29761=ORIENTED_EDGE('',*,*,#20787,.F.);
#29762=ORIENTED_EDGE('',*,*,#20788,.T.);
#29763=ORIENTED_EDGE('',*,*,#20789,.T.);
#29764=ORIENTED_EDGE('',*,*,#20785,.F.);
#29765=ORIENTED_EDGE('',*,*,#20790,.F.);
#29766=ORIENTED_EDGE('',*,*,#20777,.T.);
#29767=ORIENTED_EDGE('',*,*,#20791,.T.);
#29768=ORIENTED_EDGE('',*,*,#20792,.F.);
#29769=ORIENTED_EDGE('',*,*,#20793,.F.);
#29770=ORIENTED_EDGE('',*,*,#20794,.T.);
#29771=ORIENTED_EDGE('',*,*,#20795,.T.);
#29772=ORIENTED_EDGE('',*,*,#20788,.F.);
#29773=ORIENTED_EDGE('',*,*,#20796,.F.);
#29774=ORIENTED_EDGE('',*,*,#20792,.T.);
#29775=ORIENTED_EDGE('',*,*,#20797,.T.);
#29776=ORIENTED_EDGE('',*,*,#20794,.F.);
#29777=ORIENTED_EDGE('',*,*,#20798,.F.);
#29778=ORIENTED_EDGE('',*,*,#20799,.T.);
#29779=ORIENTED_EDGE('',*,*,#20800,.T.);
#29780=ORIENTED_EDGE('',*,*,#20801,.F.);
#29781=ORIENTED_EDGE('',*,*,#20802,.F.);
#29782=ORIENTED_EDGE('',*,*,#20611,.F.);
#29783=ORIENTED_EDGE('',*,*,#20803,.T.);
#29784=ORIENTED_EDGE('',*,*,#20804,.T.);
#29785=ORIENTED_EDGE('',*,*,#20805,.F.);
#29786=ORIENTED_EDGE('',*,*,#20806,.F.);
#29787=ORIENTED_EDGE('',*,*,#20807,.F.);
#29788=ORIENTED_EDGE('',*,*,#20808,.T.);
#29789=ORIENTED_EDGE('',*,*,#20809,.T.);
#29790=ORIENTED_EDGE('',*,*,#20810,.T.);
#29791=ORIENTED_EDGE('',*,*,#20808,.F.);
#29792=ORIENTED_EDGE('',*,*,#20811,.F.);
#29793=ORIENTED_EDGE('',*,*,#20812,.T.);
#29794=ORIENTED_EDGE('',*,*,#20813,.T.);
#29795=ORIENTED_EDGE('',*,*,#20810,.F.);
#29796=ORIENTED_EDGE('',*,*,#20814,.F.);
#29797=ORIENTED_EDGE('',*,*,#20806,.T.);
#29798=ORIENTED_EDGE('',*,*,#20815,.F.);
#29799=ORIENTED_EDGE('',*,*,#20816,.F.);
#29800=ORIENTED_EDGE('',*,*,#20817,.T.);
#29801=ORIENTED_EDGE('',*,*,#20812,.F.);
#29802=ORIENTED_EDGE('',*,*,#20818,.F.);
#29803=ORIENTED_EDGE('',*,*,#20819,.T.);
#29804=ORIENTED_EDGE('',*,*,#20820,.T.);
#29805=ORIENTED_EDGE('',*,*,#20799,.F.);
#29806=ORIENTED_EDGE('',*,*,#20815,.T.);
#29807=ORIENTED_EDGE('',*,*,#20821,.T.);
#29808=ORIENTED_EDGE('',*,*,#20817,.F.);
#29809=ORIENTED_EDGE('',*,*,#20822,.F.);
#29810=ORIENTED_EDGE('',*,*,#20823,.F.);
#29811=ORIENTED_EDGE('',*,*,#20824,.T.);
#29812=ORIENTED_EDGE('',*,*,#20819,.F.);
#29813=ORIENTED_EDGE('',*,*,#20825,.F.);
#29814=ORIENTED_EDGE('',*,*,#20714,.T.);
#29815=ORIENTED_EDGE('',*,*,#20826,.T.);
#29816=ORIENTED_EDGE('',*,*,#20827,.F.);
#29817=ORIENTED_EDGE('',*,*,#20828,.F.);
#29818=ORIENTED_EDGE('',*,*,#20827,.T.);
#29819=ORIENTED_EDGE('',*,*,#20829,.T.);
#29820=ORIENTED_EDGE('',*,*,#20830,.F.);
#29821=ORIENTED_EDGE('',*,*,#20831,.F.);
#29822=ORIENTED_EDGE('',*,*,#20832,.T.);
#29823=ORIENTED_EDGE('',*,*,#20833,.T.);
#29824=ORIENTED_EDGE('',*,*,#20626,.F.);
#29825=ORIENTED_EDGE('',*,*,#20834,.F.);
#29826=ORIENTED_EDGE('',*,*,#20830,.T.);
#29827=ORIENTED_EDGE('',*,*,#20835,.T.);
#29828=ORIENTED_EDGE('',*,*,#20836,.F.);
#29829=ORIENTED_EDGE('',*,*,#20837,.F.);
#29830=ORIENTED_EDGE('',*,*,#20838,.T.);
#29831=ORIENTED_EDGE('',*,*,#20804,.F.);
#29832=ORIENTED_EDGE('',*,*,#20839,.F.);
#29833=ORIENTED_EDGE('',*,*,#20840,.T.);
#29834=ORIENTED_EDGE('',*,*,#20150,.T.);
#29835=ORIENTED_EDGE('',*,*,#20617,.F.);
#29836=ORIENTED_EDGE('',*,*,#20841,.F.);
#29837=ORIENTED_EDGE('',*,*,#20621,.F.);
#29838=ORIENTED_EDGE('',*,*,#20842,.F.);
#29839=ORIENTED_EDGE('',*,*,#20843,.F.);
#29840=ORIENTED_EDGE('',*,*,#20841,.T.);
#29841=ORIENTED_EDGE('',*,*,#20620,.T.);
#29842=ORIENTED_EDGE('',*,*,#20712,.F.);
#29843=ORIENTED_EDGE('',*,*,#20844,.F.);
#29844=ORIENTED_EDGE('',*,*,#20154,.T.);
#29845=ORIENTED_EDGE('',*,*,#20840,.F.);
#29846=ORIENTED_EDGE('',*,*,#20845,.F.);
#29847=ORIENTED_EDGE('',*,*,#20845,.T.);
#29848=ORIENTED_EDGE('',*,*,#20843,.T.);
#29849=ORIENTED_EDGE('',*,*,#20846,.F.);
#29850=ORIENTED_EDGE('',*,*,#20847,.F.);
#29851=ORIENTED_EDGE('',*,*,#20848,.T.);
#29852=ORIENTED_EDGE('',*,*,#20849,.F.);
#29853=ORIENTED_EDGE('',*,*,#20850,.T.);
#29854=ORIENTED_EDGE('',*,*,#20851,.T.);
#29855=ORIENTED_EDGE('',*,*,#20838,.F.);
#29856=ORIENTED_EDGE('',*,*,#20852,.T.);
#29857=ORIENTED_EDGE('',*,*,#20853,.T.);
#29858=ORIENTED_EDGE('',*,*,#20854,.F.);
#29859=ORIENTED_EDGE('',*,*,#20855,.F.);
#29860=ORIENTED_EDGE('',*,*,#20856,.T.);
#29861=ORIENTED_EDGE('',*,*,#20857,.T.);
#29862=ORIENTED_EDGE('',*,*,#20640,.T.);
#29863=ORIENTED_EDGE('',*,*,#20858,.F.);
#29864=ORIENTED_EDGE('',*,*,#20859,.F.);
#29865=ORIENTED_EDGE('',*,*,#20860,.T.);
#29866=ORIENTED_EDGE('',*,*,#20676,.T.);
#29867=ORIENTED_EDGE('',*,*,#20861,.F.);
#29868=ORIENTED_EDGE('',*,*,#20862,.F.);
#29869=ORIENTED_EDGE('',*,*,#20863,.T.);
#29870=ORIENTED_EDGE('',*,*,#20864,.T.);
#29871=ORIENTED_EDGE('',*,*,#20865,.F.);
#29872=ORIENTED_EDGE('',*,*,#19948,.F.);
#29873=ORIENTED_EDGE('',*,*,#20866,.T.);
#29874=ORIENTED_EDGE('',*,*,#20867,.T.);
#29875=ORIENTED_EDGE('',*,*,#20868,.F.);
#29876=ORIENTED_EDGE('',*,*,#19964,.F.);
#29877=ORIENTED_EDGE('',*,*,#20868,.T.);
#29878=ORIENTED_EDGE('',*,*,#20869,.T.);
#29879=ORIENTED_EDGE('',*,*,#20870,.F.);
#29880=ORIENTED_EDGE('',*,*,#19969,.F.);
#29881=ORIENTED_EDGE('',*,*,#20870,.T.);
#29882=ORIENTED_EDGE('',*,*,#20871,.T.);
#29883=ORIENTED_EDGE('',*,*,#20872,.F.);
#29884=ORIENTED_EDGE('',*,*,#19972,.F.);
#29885=ORIENTED_EDGE('',*,*,#20872,.T.);
#29886=ORIENTED_EDGE('',*,*,#20873,.T.);
#29887=ORIENTED_EDGE('',*,*,#20874,.F.);
#29888=ORIENTED_EDGE('',*,*,#19977,.F.);
#29889=ORIENTED_EDGE('',*,*,#20874,.T.);
#29890=ORIENTED_EDGE('',*,*,#20875,.T.);
#29891=ORIENTED_EDGE('',*,*,#20876,.F.);
#29892=ORIENTED_EDGE('',*,*,#19980,.F.);
#29893=ORIENTED_EDGE('',*,*,#20876,.T.);
#29894=ORIENTED_EDGE('',*,*,#20877,.T.);
#29895=ORIENTED_EDGE('',*,*,#20863,.F.);
#29896=ORIENTED_EDGE('',*,*,#19985,.F.);
#29897=ORIENTED_EDGE('',*,*,#20865,.T.);
#29898=ORIENTED_EDGE('',*,*,#20878,.T.);
#29899=ORIENTED_EDGE('',*,*,#20879,.F.);
#29900=ORIENTED_EDGE('',*,*,#20628,.F.);
#29901=ORIENTED_EDGE('',*,*,#20879,.T.);
#29902=ORIENTED_EDGE('',*,*,#20880,.T.);
#29903=ORIENTED_EDGE('',*,*,#20881,.F.);
#29904=ORIENTED_EDGE('',*,*,#20633,.F.);
#29905=ORIENTED_EDGE('',*,*,#20882,.T.);
#29906=ORIENTED_EDGE('',*,*,#20883,.T.);
#29907=ORIENTED_EDGE('',*,*,#20866,.F.);
#29908=ORIENTED_EDGE('',*,*,#20647,.F.);
#29909=ORIENTED_EDGE('',*,*,#20884,.T.);
#29910=ORIENTED_EDGE('',*,*,#20885,.T.);
#29911=ORIENTED_EDGE('',*,*,#20882,.F.);
#29912=ORIENTED_EDGE('',*,*,#20653,.F.);
#29913=ORIENTED_EDGE('',*,*,#20886,.T.);
#29914=ORIENTED_EDGE('',*,*,#20887,.T.);
#29915=ORIENTED_EDGE('',*,*,#20884,.F.);
#29916=ORIENTED_EDGE('',*,*,#20654,.F.);
#29917=ORIENTED_EDGE('',*,*,#20888,.T.);
#29918=ORIENTED_EDGE('',*,*,#20889,.T.);
#29919=ORIENTED_EDGE('',*,*,#20886,.F.);
#29920=ORIENTED_EDGE('',*,*,#20661,.F.);
#29921=ORIENTED_EDGE('',*,*,#20890,.T.);
#29922=ORIENTED_EDGE('',*,*,#20891,.T.);
#29923=ORIENTED_EDGE('',*,*,#20888,.F.);
#29924=ORIENTED_EDGE('',*,*,#20662,.F.);
#29925=ORIENTED_EDGE('',*,*,#20892,.T.);
#29926=ORIENTED_EDGE('',*,*,#20893,.T.);
#29927=ORIENTED_EDGE('',*,*,#20890,.F.);
#29928=ORIENTED_EDGE('',*,*,#20669,.F.);
#29929=ORIENTED_EDGE('',*,*,#20881,.T.);
#29930=ORIENTED_EDGE('',*,*,#20894,.T.);
#29931=ORIENTED_EDGE('',*,*,#20892,.F.);
#29932=ORIENTED_EDGE('',*,*,#20670,.F.);
#29933=ORIENTED_EDGE('',*,*,#20859,.T.);
#29934=ORIENTED_EDGE('',*,*,#20895,.T.);
#29935=ORIENTED_EDGE('',*,*,#20862,.T.);
#29936=ORIENTED_EDGE('',*,*,#20896,.F.);
#29937=ORIENTED_EDGE('',*,*,#20897,.F.);
#29938=ORIENTED_EDGE('',*,*,#20898,.T.);
#29939=ORIENTED_EDGE('',*,*,#20287,.T.);
#29940=ORIENTED_EDGE('',*,*,#20200,.T.);
#29941=ORIENTED_EDGE('',*,*,#20167,.F.);
#29942=ORIENTED_EDGE('',*,*,#20183,.F.);
#29943=ORIENTED_EDGE('',*,*,#20164,.F.);
#29944=ORIENTED_EDGE('',*,*,#20177,.T.);
#29945=ORIENTED_EDGE('',*,*,#20172,.F.);
#29946=ORIENTED_EDGE('',*,*,#20899,.T.);
#29947=ORIENTED_EDGE('',*,*,#20900,.F.);
#29948=ORIENTED_EDGE('',*,*,#20869,.F.);
#29949=ORIENTED_EDGE('',*,*,#20867,.F.);
#29950=ORIENTED_EDGE('',*,*,#20883,.F.);
#29951=ORIENTED_EDGE('',*,*,#20885,.F.);
#29952=ORIENTED_EDGE('',*,*,#20887,.F.);
#29953=ORIENTED_EDGE('',*,*,#20889,.F.);
#29954=ORIENTED_EDGE('',*,*,#20891,.F.);
#29955=ORIENTED_EDGE('',*,*,#20893,.F.);
#29956=ORIENTED_EDGE('',*,*,#20894,.F.);
#29957=ORIENTED_EDGE('',*,*,#20880,.F.);
#29958=ORIENTED_EDGE('',*,*,#20878,.F.);
#29959=ORIENTED_EDGE('',*,*,#20864,.F.);
#29960=ORIENTED_EDGE('',*,*,#20877,.F.);
#29961=ORIENTED_EDGE('',*,*,#20875,.F.);
#29962=ORIENTED_EDGE('',*,*,#20873,.F.);
#29963=ORIENTED_EDGE('',*,*,#20871,.F.);
#29964=ORIENTED_EDGE('',*,*,#20635,.T.);
#29965=ORIENTED_EDGE('',*,*,#20901,.T.);
#29966=ORIENTED_EDGE('',*,*,#20171,.F.);
#29967=ORIENTED_EDGE('',*,*,#20646,.T.);
#29968=ORIENTED_EDGE('',*,*,#20902,.F.);
#29969=ORIENTED_EDGE('',*,*,#20899,.F.);
#29970=ORIENTED_EDGE('',*,*,#20901,.F.);
#29971=ORIENTED_EDGE('',*,*,#20900,.T.);
#29972=ORIENTED_EDGE('',*,*,#20903,.F.);
#29973=ORIENTED_EDGE('',*,*,#20904,.F.);
#29974=ORIENTED_EDGE('',*,*,#20905,.T.);
#29975=ORIENTED_EDGE('',*,*,#20906,.T.);
#29976=ORIENTED_EDGE('',*,*,#20907,.T.);
#29977=ORIENTED_EDGE('',*,*,#20908,.F.);
#29978=ORIENTED_EDGE('',*,*,#20482,.F.);
#29979=ORIENTED_EDGE('',*,*,#20909,.T.);
#29980=ORIENTED_EDGE('',*,*,#20906,.F.);
#29981=ORIENTED_EDGE('',*,*,#20514,.F.);
#29982=ORIENTED_EDGE('',*,*,#20675,.T.);
#29983=ORIENTED_EDGE('',*,*,#20910,.T.);
#29984=ORIENTED_EDGE('',*,*,#20909,.F.);
#29985=ORIENTED_EDGE('',*,*,#20516,.F.);
#29986=ORIENTED_EDGE('',*,*,#20858,.T.);
#29987=ORIENTED_EDGE('',*,*,#20911,.T.);
#29988=ORIENTED_EDGE('',*,*,#20860,.F.);
#29989=ORIENTED_EDGE('',*,*,#20895,.F.);
#29990=ORIENTED_EDGE('',*,*,#20639,.T.);
#29991=ORIENTED_EDGE('',*,*,#20912,.F.);
#29992=ORIENTED_EDGE('',*,*,#20907,.F.);
#29993=ORIENTED_EDGE('',*,*,#20910,.F.);
#29994=ORIENTED_EDGE('',*,*,#20677,.F.);
#29995=ORIENTED_EDGE('',*,*,#20911,.F.);
#29996=ORIENTED_EDGE('',*,*,#20913,.T.);
#29997=ORIENTED_EDGE('',*,*,#20644,.T.);
#29998=ORIENTED_EDGE('',*,*,#20914,.F.);
#29999=ORIENTED_EDGE('',*,*,#20915,.F.);
#30000=ORIENTED_EDGE('',*,*,#20914,.T.);
#30001=ORIENTED_EDGE('',*,*,#20643,.T.);
#30002=ORIENTED_EDGE('',*,*,#20916,.F.);
#30003=ORIENTED_EDGE('',*,*,#20856,.F.);
#30004=ORIENTED_EDGE('',*,*,#20916,.T.);
#30005=ORIENTED_EDGE('',*,*,#20642,.T.);
#30006=ORIENTED_EDGE('',*,*,#20917,.F.);
#30007=ORIENTED_EDGE('',*,*,#20918,.F.);
#30008=ORIENTED_EDGE('',*,*,#20919,.T.);
#30009=ORIENTED_EDGE('',*,*,#20857,.F.);
#30010=ORIENTED_EDGE('',*,*,#20905,.F.);
#30011=ORIENTED_EDGE('',*,*,#20920,.F.);
#30012=ORIENTED_EDGE('',*,*,#20917,.T.);
#30013=ORIENTED_EDGE('',*,*,#20641,.T.);
#30014=ORIENTED_EDGE('',*,*,#20919,.F.);
#30015=ORIENTED_EDGE('',*,*,#20921,.T.);
#30016=ORIENTED_EDGE('',*,*,#20645,.T.);
#30017=ORIENTED_EDGE('',*,*,#20913,.F.);
#30018=ORIENTED_EDGE('',*,*,#20922,.F.);
#30019=ORIENTED_EDGE('',*,*,#20898,.F.);
#30020=ORIENTED_EDGE('',*,*,#20923,.F.);
#30021=ORIENTED_EDGE('',*,*,#20924,.T.);
#30022=ORIENTED_EDGE('',*,*,#20288,.T.);
#30023=ORIENTED_EDGE('',*,*,#20924,.F.);
#30024=ORIENTED_EDGE('',*,*,#20851,.F.);
#30025=ORIENTED_EDGE('',*,*,#20925,.F.);
#30026=ORIENTED_EDGE('',*,*,#20155,.T.);
#30027=ORIENTED_EDGE('',*,*,#20222,.F.);
#30028=ORIENTED_EDGE('',*,*,#20233,.F.);
#30029=ORIENTED_EDGE('',*,*,#20925,.T.);
#30030=ORIENTED_EDGE('',*,*,#20926,.T.);
#30031=ORIENTED_EDGE('',*,*,#20927,.T.);
#30032=ORIENTED_EDGE('',*,*,#20928,.T.);
#30033=ORIENTED_EDGE('',*,*,#20929,.F.);
#30034=ORIENTED_EDGE('',*,*,#20930,.T.);
#30035=ORIENTED_EDGE('',*,*,#20681,.F.);
#30036=ORIENTED_EDGE('',*,*,#20208,.F.);
#30037=ORIENTED_EDGE('',*,*,#20928,.F.);
#30038=ORIENTED_EDGE('',*,*,#20931,.T.);
#30039=ORIENTED_EDGE('',*,*,#20932,.T.);
#30040=ORIENTED_EDGE('',*,*,#20933,.T.);
#30041=ORIENTED_EDGE('',*,*,#20934,.T.);
#30042=ORIENTED_EDGE('',*,*,#20935,.T.);
#30043=ORIENTED_EDGE('',*,*,#20936,.T.);
#30044=ORIENTED_EDGE('',*,*,#20929,.T.);
#30045=ORIENTED_EDGE('',*,*,#20214,.F.);
#30046=ORIENTED_EDGE('',*,*,#20232,.F.);
#30047=ORIENTED_EDGE('',*,*,#20229,.F.);
#30048=ORIENTED_EDGE('',*,*,#20226,.F.);
#30049=ORIENTED_EDGE('',*,*,#20224,.F.);
#30050=ORIENTED_EDGE('',*,*,#20223,.F.);
#30051=ORIENTED_EDGE('',*,*,#20861,.T.);
#30052=ORIENTED_EDGE('',*,*,#20937,.F.);
#30053=ORIENTED_EDGE('',*,*,#20938,.F.);
#30054=ORIENTED_EDGE('',*,*,#20939,.F.);
#30055=ORIENTED_EDGE('',*,*,#20939,.T.);
#30056=ORIENTED_EDGE('',*,*,#20940,.F.);
#30057=ORIENTED_EDGE('',*,*,#20941,.T.);
#30058=ORIENTED_EDGE('',*,*,#20896,.T.);
#30059=ORIENTED_EDGE('',*,*,#20938,.T.);
#30060=ORIENTED_EDGE('',*,*,#20937,.T.);
#30061=ORIENTED_EDGE('',*,*,#20683,.T.);
#30062=ORIENTED_EDGE('',*,*,#20942,.F.);
#30063=ORIENTED_EDGE('',*,*,#20943,.F.);
#30064=ORIENTED_EDGE('',*,*,#20944,.T.);
#30065=ORIENTED_EDGE('',*,*,#20849,.T.);
#30066=ORIENTED_EDGE('',*,*,#20940,.T.);
#30067=ORIENTED_EDGE('',*,*,#20943,.T.);
#30068=ORIENTED_EDGE('',*,*,#20942,.T.);
#30069=ORIENTED_EDGE('',*,*,#20682,.T.);
#30070=ORIENTED_EDGE('',*,*,#20930,.F.);
#30071=ORIENTED_EDGE('',*,*,#20945,.F.);
#30072=ORIENTED_EDGE('',*,*,#20945,.T.);
#30073=ORIENTED_EDGE('',*,*,#20936,.F.);
#30074=ORIENTED_EDGE('',*,*,#20946,.T.);
#30075=ORIENTED_EDGE('',*,*,#20947,.F.);
#30076=ORIENTED_EDGE('',*,*,#20948,.T.);
#30077=ORIENTED_EDGE('',*,*,#20949,.T.);
#30078=ORIENTED_EDGE('',*,*,#20944,.F.);
#30079=ORIENTED_EDGE('',*,*,#20950,.T.);
#30080=ORIENTED_EDGE('',*,*,#20951,.T.);
#30081=ORIENTED_EDGE('',*,*,#20688,.F.);
#30082=ORIENTED_EDGE('',*,*,#20952,.F.);
#30083=ORIENTED_EDGE('',*,*,#20952,.T.);
#30084=ORIENTED_EDGE('',*,*,#20694,.F.);
#30085=ORIENTED_EDGE('',*,*,#20953,.F.);
#30086=ORIENTED_EDGE('',*,*,#20931,.F.);
#30087=ORIENTED_EDGE('',*,*,#20927,.F.);
#30088=ORIENTED_EDGE('',*,*,#20954,.F.);
#30089=ORIENTED_EDGE('',*,*,#20948,.F.);
#30090=ORIENTED_EDGE('',*,*,#20955,.T.);
#30091=ORIENTED_EDGE('',*,*,#20953,.T.);
#30092=ORIENTED_EDGE('',*,*,#20696,.F.);
#30093=ORIENTED_EDGE('',*,*,#20956,.F.);
#30094=ORIENTED_EDGE('',*,*,#20956,.T.);
#30095=ORIENTED_EDGE('',*,*,#20700,.F.);
#30096=ORIENTED_EDGE('',*,*,#20957,.F.);
#30097=ORIENTED_EDGE('',*,*,#20932,.F.);
#30098=ORIENTED_EDGE('',*,*,#20957,.T.);
#30099=ORIENTED_EDGE('',*,*,#20702,.F.);
#30100=ORIENTED_EDGE('',*,*,#20958,.F.);
#30101=ORIENTED_EDGE('',*,*,#20933,.F.);
#30102=ORIENTED_EDGE('',*,*,#20959,.T.);
#30103=ORIENTED_EDGE('',*,*,#20705,.F.);
#30104=ORIENTED_EDGE('',*,*,#20951,.F.);
#30105=ORIENTED_EDGE('',*,*,#20958,.T.);
#30106=ORIENTED_EDGE('',*,*,#20709,.F.);
#30107=ORIENTED_EDGE('',*,*,#20960,.F.);
#30108=ORIENTED_EDGE('',*,*,#20934,.F.);
#30109=ORIENTED_EDGE('',*,*,#20946,.F.);
#30110=ORIENTED_EDGE('',*,*,#20935,.F.);
#30111=ORIENTED_EDGE('',*,*,#20960,.T.);
#30112=ORIENTED_EDGE('',*,*,#20711,.F.);
#30113=ORIENTED_EDGE('',*,*,#20959,.F.);
#30114=ORIENTED_EDGE('',*,*,#20961,.T.);
#30115=ORIENTED_EDGE('',*,*,#20961,.F.);
#30116=ORIENTED_EDGE('',*,*,#20950,.F.);
#30117=ORIENTED_EDGE('',*,*,#20955,.F.);
#30118=ORIENTED_EDGE('',*,*,#20947,.T.);
#30119=ORIENTED_EDGE('',*,*,#20954,.T.);
#30120=ORIENTED_EDGE('',*,*,#20926,.F.);
#30121=ORIENTED_EDGE('',*,*,#20850,.F.);
#30122=ORIENTED_EDGE('',*,*,#20949,.F.);
#30123=ORIENTED_EDGE('',*,*,#20962,.T.);
#30124=ORIENTED_EDGE('',*,*,#20963,.F.);
#30125=ORIENTED_EDGE('',*,*,#20964,.T.);
#30126=ORIENTED_EDGE('',*,*,#20715,.T.);
#30127=ORIENTED_EDGE('',*,*,#20965,.T.);
#30128=ORIENTED_EDGE('',*,*,#20852,.F.);
#30129=ORIENTED_EDGE('',*,*,#20966,.F.);
#30130=ORIENTED_EDGE('',*,*,#20717,.F.);
#30131=ORIENTED_EDGE('',*,*,#20721,.F.);
#30132=ORIENTED_EDGE('',*,*,#20967,.T.);
#30133=ORIENTED_EDGE('',*,*,#20968,.T.);
#30134=ORIENTED_EDGE('',*,*,#20965,.F.);
#30135=ORIENTED_EDGE('',*,*,#20969,.F.);
#30136=ORIENTED_EDGE('',*,*,#20970,.F.);
#30137=ORIENTED_EDGE('',*,*,#20967,.F.);
#30138=ORIENTED_EDGE('',*,*,#20724,.F.);
#30139=ORIENTED_EDGE('',*,*,#20727,.F.);
#30140=ORIENTED_EDGE('',*,*,#20971,.F.);
#30141=ORIENTED_EDGE('',*,*,#20972,.F.);
#30142=ORIENTED_EDGE('',*,*,#20969,.T.);
#30143=ORIENTED_EDGE('',*,*,#20730,.F.);
#30144=ORIENTED_EDGE('',*,*,#20973,.T.);
#30145=ORIENTED_EDGE('',*,*,#20974,.F.);
#30146=ORIENTED_EDGE('',*,*,#20971,.T.);
#30147=ORIENTED_EDGE('',*,*,#20732,.F.);
#30148=ORIENTED_EDGE('',*,*,#20966,.T.);
#30149=ORIENTED_EDGE('',*,*,#20839,.T.);
#30150=ORIENTED_EDGE('',*,*,#20975,.F.);
#30151=ORIENTED_EDGE('',*,*,#20736,.F.);
#30152=ORIENTED_EDGE('',*,*,#20976,.T.);
#30153=ORIENTED_EDGE('',*,*,#20613,.T.);
#30154=ORIENTED_EDGE('',*,*,#20973,.F.);
#30155=ORIENTED_EDGE('',*,*,#20975,.T.);
#30156=ORIENTED_EDGE('',*,*,#20803,.F.);
#30157=ORIENTED_EDGE('',*,*,#20976,.F.);
#30158=ORIENTED_EDGE('',*,*,#20738,.F.);
#30159=ORIENTED_EDGE('',*,*,#20743,.T.);
#30160=ORIENTED_EDGE('',*,*,#20977,.T.);
#30161=ORIENTED_EDGE('',*,*,#20807,.T.);
#30162=ORIENTED_EDGE('',*,*,#20978,.F.);
#30163=ORIENTED_EDGE('',*,*,#20748,.T.);
#30164=ORIENTED_EDGE('',*,*,#20979,.T.);
#30165=ORIENTED_EDGE('',*,*,#20811,.T.);
#30166=ORIENTED_EDGE('',*,*,#20977,.F.);
#30167=ORIENTED_EDGE('',*,*,#20980,.T.);
#30168=ORIENTED_EDGE('',*,*,#20814,.T.);
#30169=ORIENTED_EDGE('',*,*,#20979,.F.);
#30170=ORIENTED_EDGE('',*,*,#20758,.T.);
#30171=ORIENTED_EDGE('',*,*,#20761,.T.);
#30172=ORIENTED_EDGE('',*,*,#20978,.T.);
#30173=ORIENTED_EDGE('',*,*,#20816,.T.);
#30174=ORIENTED_EDGE('',*,*,#20981,.F.);
#30175=ORIENTED_EDGE('',*,*,#20764,.T.);
#30176=ORIENTED_EDGE('',*,*,#20982,.T.);
#30177=ORIENTED_EDGE('',*,*,#20818,.T.);
#30178=ORIENTED_EDGE('',*,*,#20980,.F.);
#30179=ORIENTED_EDGE('',*,*,#20766,.T.);
#30180=ORIENTED_EDGE('',*,*,#20981,.T.);
#30181=ORIENTED_EDGE('',*,*,#20822,.T.);
#30182=ORIENTED_EDGE('',*,*,#20982,.F.);
#30183=ORIENTED_EDGE('',*,*,#20983,.F.);
#30184=ORIENTED_EDGE('',*,*,#20824,.F.);
#30185=ORIENTED_EDGE('',*,*,#20984,.F.);
#30186=ORIENTED_EDGE('',*,*,#20776,.F.);
#30187=ORIENTED_EDGE('',*,*,#20780,.F.);
#30188=ORIENTED_EDGE('',*,*,#20985,.F.);
#30189=ORIENTED_EDGE('',*,*,#20820,.F.);
#30190=ORIENTED_EDGE('',*,*,#20983,.T.);
#30191=ORIENTED_EDGE('',*,*,#20783,.F.);
#30192=ORIENTED_EDGE('',*,*,#20986,.F.);
#30193=ORIENTED_EDGE('',*,*,#20800,.F.);
#30194=ORIENTED_EDGE('',*,*,#20985,.T.);
#30195=ORIENTED_EDGE('',*,*,#20786,.F.);
#30196=ORIENTED_EDGE('',*,*,#20987,.F.);
#30197=ORIENTED_EDGE('',*,*,#20988,.F.);
#30198=ORIENTED_EDGE('',*,*,#20986,.T.);
#30199=ORIENTED_EDGE('',*,*,#20789,.F.);
#30200=ORIENTED_EDGE('',*,*,#20989,.F.);
#30201=ORIENTED_EDGE('',*,*,#20990,.F.);
#30202=ORIENTED_EDGE('',*,*,#20987,.T.);
#30203=ORIENTED_EDGE('',*,*,#20791,.F.);
#30204=ORIENTED_EDGE('',*,*,#20984,.T.);
#30205=ORIENTED_EDGE('',*,*,#20991,.T.);
#30206=ORIENTED_EDGE('',*,*,#20992,.F.);
#30207=ORIENTED_EDGE('',*,*,#20795,.F.);
#30208=ORIENTED_EDGE('',*,*,#20993,.F.);
#30209=ORIENTED_EDGE('',*,*,#20994,.F.);
#30210=ORIENTED_EDGE('',*,*,#20989,.T.);
#30211=ORIENTED_EDGE('',*,*,#20992,.T.);
#30212=ORIENTED_EDGE('',*,*,#20995,.F.);
#30213=ORIENTED_EDGE('',*,*,#20993,.T.);
#30214=ORIENTED_EDGE('',*,*,#20797,.F.);
#30215=ORIENTED_EDGE('',*,*,#20801,.T.);
#30216=ORIENTED_EDGE('',*,*,#20988,.T.);
#30217=ORIENTED_EDGE('',*,*,#20996,.F.);
#30218=ORIENTED_EDGE('',*,*,#20997,.F.);
#30219=ORIENTED_EDGE('',*,*,#20998,.F.);
#30220=ORIENTED_EDGE('',*,*,#20996,.T.);
#30221=ORIENTED_EDGE('',*,*,#20990,.T.);
#30222=ORIENTED_EDGE('',*,*,#20823,.T.);
#30223=ORIENTED_EDGE('',*,*,#20999,.F.);
#30224=ORIENTED_EDGE('',*,*,#20991,.F.);
#30225=ORIENTED_EDGE('',*,*,#20997,.T.);
#30226=ORIENTED_EDGE('',*,*,#20994,.T.);
#30227=ORIENTED_EDGE('',*,*,#21000,.F.);
#30228=ORIENTED_EDGE('',*,*,#20999,.T.);
#30229=ORIENTED_EDGE('',*,*,#21001,.F.);
#30230=ORIENTED_EDGE('',*,*,#21000,.T.);
#30231=ORIENTED_EDGE('',*,*,#20995,.T.);
#30232=ORIENTED_EDGE('',*,*,#21002,.T.);
#30233=ORIENTED_EDGE('',*,*,#20805,.T.);
#30234=ORIENTED_EDGE('',*,*,#20854,.T.);
#30235=ORIENTED_EDGE('',*,*,#21003,.T.);
#30236=ORIENTED_EDGE('',*,*,#20903,.T.);
#30237=ORIENTED_EDGE('',*,*,#20902,.T.);
#30238=ORIENTED_EDGE('',*,*,#20921,.F.);
#30239=ORIENTED_EDGE('',*,*,#21004,.T.);
#30240=ORIENTED_EDGE('',*,*,#21005,.F.);
#30241=ORIENTED_EDGE('',*,*,#21006,.F.);
#30242=ORIENTED_EDGE('',*,*,#20821,.F.);
#30243=ORIENTED_EDGE('',*,*,#20809,.F.);
#30244=ORIENTED_EDGE('',*,*,#20813,.F.);
#30245=ORIENTED_EDGE('',*,*,#21001,.T.);
#30246=ORIENTED_EDGE('',*,*,#20825,.T.);
#30247=ORIENTED_EDGE('',*,*,#20802,.T.);
#30248=ORIENTED_EDGE('',*,*,#20998,.T.);
#30249=ORIENTED_EDGE('',*,*,#20828,.T.);
#30250=ORIENTED_EDGE('',*,*,#21007,.T.);
#30251=ORIENTED_EDGE('',*,*,#21006,.T.);
#30252=ORIENTED_EDGE('',*,*,#20962,.F.);
#30253=ORIENTED_EDGE('',*,*,#20904,.T.);
#30254=ORIENTED_EDGE('',*,*,#20922,.T.);
#30255=ORIENTED_EDGE('',*,*,#21008,.T.);
#30256=ORIENTED_EDGE('',*,*,#20920,.T.);
#30257=ORIENTED_EDGE('',*,*,#21009,.T.);
#30258=ORIENTED_EDGE('',*,*,#20853,.F.);
#30259=ORIENTED_EDGE('',*,*,#20968,.F.);
#30260=ORIENTED_EDGE('',*,*,#20612,.T.);
#30261=ORIENTED_EDGE('',*,*,#21002,.F.);
#30262=ORIENTED_EDGE('',*,*,#21010,.T.);
#30263=ORIENTED_EDGE('',*,*,#20974,.T.);
#30264=ORIENTED_EDGE('',*,*,#20964,.F.);
#30265=ORIENTED_EDGE('',*,*,#21011,.T.);
#30266=ORIENTED_EDGE('',*,*,#20842,.T.);
#30267=ORIENTED_EDGE('',*,*,#20844,.T.);
#30268=ORIENTED_EDGE('',*,*,#20846,.T.);
#30269=ORIENTED_EDGE('',*,*,#21011,.F.);
#30270=ORIENTED_EDGE('',*,*,#21012,.F.);
#30271=ORIENTED_EDGE('',*,*,#21013,.F.);
#30272=ORIENTED_EDGE('',*,*,#21003,.F.);
#30273=ORIENTED_EDGE('',*,*,#21009,.F.);
#30274=ORIENTED_EDGE('',*,*,#20970,.T.);
#30275=ORIENTED_EDGE('',*,*,#21005,.T.);
#30276=ORIENTED_EDGE('',*,*,#21014,.F.);
#30277=ORIENTED_EDGE('',*,*,#21012,.T.);
#30278=ORIENTED_EDGE('',*,*,#20963,.T.);
#30279=ORIENTED_EDGE('',*,*,#21013,.T.);
#30280=ORIENTED_EDGE('',*,*,#20972,.T.);
#30281=ORIENTED_EDGE('',*,*,#21010,.F.);
#30282=ORIENTED_EDGE('',*,*,#20855,.T.);
#30283=ORIENTED_EDGE('',*,*,#20918,.T.);
#30284=ORIENTED_EDGE('',*,*,#21008,.F.);
#30285=ORIENTED_EDGE('',*,*,#20915,.T.);
#30286=ORIENTED_EDGE('',*,*,#20923,.T.);
#30287=ORIENTED_EDGE('',*,*,#20897,.T.);
#30288=ORIENTED_EDGE('',*,*,#20941,.F.);
#30289=ORIENTED_EDGE('',*,*,#20848,.F.);
#30290=ORIENTED_EDGE('',*,*,#21015,.T.);
#30291=ORIENTED_EDGE('',*,*,#21016,.F.);
#30292=ORIENTED_EDGE('',*,*,#21017,.F.);
#30293=ORIENTED_EDGE('',*,*,#20837,.T.);
#30294=ORIENTED_EDGE('',*,*,#21018,.T.);
#30295=ORIENTED_EDGE('',*,*,#21017,.T.);
#30296=ORIENTED_EDGE('',*,*,#21019,.F.);
#30297=ORIENTED_EDGE('',*,*,#21019,.T.);
#30298=ORIENTED_EDGE('',*,*,#21020,.F.);
#30299=ORIENTED_EDGE('',*,*,#21007,.F.);
#30300=ORIENTED_EDGE('',*,*,#20831,.T.);
#30301=ORIENTED_EDGE('',*,*,#21016,.T.);
#30302=ORIENTED_EDGE('',*,*,#21021,.F.);
#30303=ORIENTED_EDGE('',*,*,#21004,.F.);
#30304=ORIENTED_EDGE('',*,*,#21020,.T.);
#30305=ORIENTED_EDGE('',*,*,#21022,.T.);
#30306=ORIENTED_EDGE('',*,*,#21023,.T.);
#30307=ORIENTED_EDGE('',*,*,#20517,.F.);
#30308=ORIENTED_EDGE('',*,*,#21024,.F.);
#30309=ORIENTED_EDGE('',*,*,#21025,.T.);
#30310=ORIENTED_EDGE('',*,*,#21024,.T.);
#30311=ORIENTED_EDGE('',*,*,#20526,.F.);
#30312=ORIENTED_EDGE('',*,*,#21026,.F.);
#30313=ORIENTED_EDGE('',*,*,#21027,.T.);
#30314=ORIENTED_EDGE('',*,*,#21026,.T.);
#30315=ORIENTED_EDGE('',*,*,#20527,.F.);
#30316=ORIENTED_EDGE('',*,*,#21028,.F.);
#30317=ORIENTED_EDGE('',*,*,#21029,.T.);
#30318=ORIENTED_EDGE('',*,*,#21028,.T.);
#30319=ORIENTED_EDGE('',*,*,#20532,.F.);
#30320=ORIENTED_EDGE('',*,*,#21030,.F.);
#30321=ORIENTED_EDGE('',*,*,#21031,.T.);
#30322=ORIENTED_EDGE('',*,*,#21030,.T.);
#30323=ORIENTED_EDGE('',*,*,#20535,.F.);
#30324=ORIENTED_EDGE('',*,*,#21032,.F.);
#30325=ORIENTED_EDGE('',*,*,#21022,.F.);
#30326=ORIENTED_EDGE('',*,*,#21025,.F.);
#30327=ORIENTED_EDGE('',*,*,#21027,.F.);
#30328=ORIENTED_EDGE('',*,*,#21029,.F.);
#30329=ORIENTED_EDGE('',*,*,#21031,.F.);
#30330=ORIENTED_EDGE('',*,*,#21033,.F.);
#30331=ORIENTED_EDGE('',*,*,#20315,.T.);
#30332=ORIENTED_EDGE('',*,*,#20306,.T.);
#30333=ORIENTED_EDGE('',*,*,#20304,.T.);
#30334=ORIENTED_EDGE('',*,*,#20302,.T.);
#30335=ORIENTED_EDGE('',*,*,#20300,.T.);
#30336=ORIENTED_EDGE('',*,*,#20298,.T.);
#30337=ORIENTED_EDGE('',*,*,#20312,.T.);
#30338=ORIENTED_EDGE('',*,*,#20324,.F.);
#30339=ORIENTED_EDGE('',*,*,#20295,.F.);
#30340=ORIENTED_EDGE('',*,*,#20286,.F.);
#30341=ORIENTED_EDGE('',*,*,#20152,.F.);
#30342=ORIENTED_EDGE('',*,*,#20847,.T.);
#30343=ORIENTED_EDGE('',*,*,#21014,.T.);
#30344=ORIENTED_EDGE('',*,*,#21021,.T.);
#30345=ORIENTED_EDGE('',*,*,#21034,.T.);
#30346=ORIENTED_EDGE('',*,*,#21035,.F.);
#30347=ORIENTED_EDGE('',*,*,#21036,.T.);
#30348=ORIENTED_EDGE('',*,*,#21037,.T.);
#30349=ORIENTED_EDGE('',*,*,#21023,.F.);
#30350=ORIENTED_EDGE('',*,*,#21038,.T.);
#30351=ORIENTED_EDGE('',*,*,#21038,.F.);
#30352=ORIENTED_EDGE('',*,*,#21036,.F.);
#30353=ORIENTED_EDGE('',*,*,#21035,.T.);
#30354=ORIENTED_EDGE('',*,*,#21039,.T.);
#30355=ORIENTED_EDGE('',*,*,#21040,.F.);
#30356=ORIENTED_EDGE('',*,*,#21041,.T.);
#30357=ORIENTED_EDGE('',*,*,#21032,.T.);
#30358=ORIENTED_EDGE('',*,*,#20536,.F.);
#30359=ORIENTED_EDGE('',*,*,#20316,.T.);
#30360=ORIENTED_EDGE('',*,*,#21042,.F.);
#30361=ORIENTED_EDGE('',*,*,#21043,.F.);
#30362=ORIENTED_EDGE('',*,*,#21042,.T.);
#30363=ORIENTED_EDGE('',*,*,#21033,.T.);
#30364=ORIENTED_EDGE('',*,*,#21041,.F.);
#30365=ORIENTED_EDGE('',*,*,#21044,.F.);
#30366=ORIENTED_EDGE('',*,*,#21045,.T.);
#30367=ORIENTED_EDGE('',*,*,#20624,.T.);
#30368=ORIENTED_EDGE('',*,*,#20518,.F.);
#30369=ORIENTED_EDGE('',*,*,#21037,.F.);
#30370=ORIENTED_EDGE('',*,*,#21045,.F.);
#30371=ORIENTED_EDGE('',*,*,#21040,.T.);
#30372=ORIENTED_EDGE('',*,*,#21046,.T.);
#30373=ORIENTED_EDGE('',*,*,#20625,.T.);
#30374=ORIENTED_EDGE('',*,*,#20319,.T.);
#30375=ORIENTED_EDGE('',*,*,#21043,.T.);
#30376=ORIENTED_EDGE('',*,*,#21047,.F.);
#30377=ORIENTED_EDGE('',*,*,#20553,.F.);
#30378=ORIENTED_EDGE('',*,*,#21047,.T.);
#30379=ORIENTED_EDGE('',*,*,#21044,.T.);
#30380=ORIENTED_EDGE('',*,*,#20538,.F.);
#30381=ORIENTED_EDGE('',*,*,#20555,.F.);
#30382=ORIENTED_EDGE('',*,*,#20834,.T.);
#30383=ORIENTED_EDGE('',*,*,#21046,.F.);
#30384=ORIENTED_EDGE('',*,*,#21048,.F.);
#30385=ORIENTED_EDGE('',*,*,#21049,.T.);
#30386=ORIENTED_EDGE('',*,*,#21050,.T.);
#30387=ORIENTED_EDGE('',*,*,#21048,.T.);
#30388=ORIENTED_EDGE('',*,*,#21039,.F.);
#30389=ORIENTED_EDGE('',*,*,#21050,.F.);
#30390=ORIENTED_EDGE('',*,*,#21034,.F.);
#30391=ORIENTED_EDGE('',*,*,#21015,.F.);
#30392=ORIENTED_EDGE('',*,*,#21051,.T.);
#30393=ORIENTED_EDGE('',*,*,#21052,.T.);
#30394=ORIENTED_EDGE('',*,*,#21049,.F.);
#30395=ORIENTED_EDGE('',*,*,#21051,.F.);
#30396=ORIENTED_EDGE('',*,*,#21018,.F.);
#30397=ORIENTED_EDGE('',*,*,#20836,.T.);
#30398=ORIENTED_EDGE('',*,*,#21053,.T.);
#30399=ORIENTED_EDGE('',*,*,#20832,.F.);
#30400=ORIENTED_EDGE('',*,*,#21052,.F.);
#30401=ORIENTED_EDGE('',*,*,#21054,.T.);
#30402=ORIENTED_EDGE('',*,*,#20449,.F.);
#30403=ORIENTED_EDGE('',*,*,#21055,.F.);
#30404=ORIENTED_EDGE('',*,*,#21056,.T.);
#30405=ORIENTED_EDGE('',*,*,#21057,.F.);
#30406=ORIENTED_EDGE('',*,*,#20686,.F.);
#30407=ORIENTED_EDGE('',*,*,#21054,.F.);
#30408=ORIENTED_EDGE('',*,*,#21057,.T.);
#30409=ORIENTED_EDGE('',*,*,#21058,.T.);
#30410=ORIENTED_EDGE('',*,*,#21059,.F.);
#30411=ORIENTED_EDGE('',*,*,#20692,.F.);
#30412=ORIENTED_EDGE('',*,*,#21059,.T.);
#30413=ORIENTED_EDGE('',*,*,#21060,.T.);
#30414=ORIENTED_EDGE('',*,*,#21061,.F.);
#30415=ORIENTED_EDGE('',*,*,#20697,.F.);
#30416=ORIENTED_EDGE('',*,*,#21061,.T.);
#30417=ORIENTED_EDGE('',*,*,#21062,.T.);
#30418=ORIENTED_EDGE('',*,*,#21063,.F.);
#30419=ORIENTED_EDGE('',*,*,#20698,.F.);
#30420=ORIENTED_EDGE('',*,*,#21063,.T.);
#30421=ORIENTED_EDGE('',*,*,#21064,.T.);
#30422=ORIENTED_EDGE('',*,*,#21065,.F.);
#30423=ORIENTED_EDGE('',*,*,#20703,.F.);
#30424=ORIENTED_EDGE('',*,*,#20690,.F.);
#30425=ORIENTED_EDGE('',*,*,#20704,.F.);
#30426=ORIENTED_EDGE('',*,*,#21066,.T.);
#30427=ORIENTED_EDGE('',*,*,#21067,.T.);
#30428=ORIENTED_EDGE('',*,*,#21068,.T.);
#30429=ORIENTED_EDGE('',*,*,#21069,.T.);
#30430=ORIENTED_EDGE('',*,*,#21066,.F.);
#30431=ORIENTED_EDGE('',*,*,#21065,.T.);
#30432=ORIENTED_EDGE('',*,*,#21070,.T.);
#30433=ORIENTED_EDGE('',*,*,#21071,.F.);
#30434=ORIENTED_EDGE('',*,*,#20707,.F.);
#30435=ORIENTED_EDGE('',*,*,#21071,.T.);
#30436=ORIENTED_EDGE('',*,*,#21072,.T.);
#30437=ORIENTED_EDGE('',*,*,#21068,.F.);
#30438=ORIENTED_EDGE('',*,*,#20710,.F.);
#30439=ORIENTED_EDGE('',*,*,#21073,.T.);
#30440=ORIENTED_EDGE('',*,*,#21055,.T.);
#30441=ORIENTED_EDGE('',*,*,#20448,.F.);
#30442=ORIENTED_EDGE('',*,*,#21074,.F.);
#30443=ORIENTED_EDGE('',*,*,#21075,.T.);
#30444=ORIENTED_EDGE('',*,*,#21074,.T.);
#30445=ORIENTED_EDGE('',*,*,#20451,.F.);
#30446=ORIENTED_EDGE('',*,*,#21076,.F.);
#30447=ORIENTED_EDGE('',*,*,#21077,.T.);
#30448=ORIENTED_EDGE('',*,*,#20638,.T.);
#30449=ORIENTED_EDGE('',*,*,#21078,.F.);
#30450=ORIENTED_EDGE('',*,*,#21079,.F.);
#30451=ORIENTED_EDGE('',*,*,#20908,.T.);
#30452=ORIENTED_EDGE('',*,*,#20912,.T.);
#30453=ORIENTED_EDGE('',*,*,#21077,.F.);
#30454=ORIENTED_EDGE('',*,*,#21080,.F.);
#30455=ORIENTED_EDGE('',*,*,#21080,.T.);
#30456=ORIENTED_EDGE('',*,*,#21079,.T.);
#30457=ORIENTED_EDGE('',*,*,#21081,.F.);
#30458=ORIENTED_EDGE('',*,*,#21082,.F.);
#30459=ORIENTED_EDGE('',*,*,#20479,.T.);
#30460=ORIENTED_EDGE('',*,*,#21083,.T.);
#30461=ORIENTED_EDGE('',*,*,#20636,.T.);
#30462=ORIENTED_EDGE('',*,*,#20541,.T.);
#30463=ORIENTED_EDGE('',*,*,#21084,.F.);
#30464=ORIENTED_EDGE('',*,*,#21084,.T.);
#30465=ORIENTED_EDGE('',*,*,#20520,.F.);
#30466=ORIENTED_EDGE('',*,*,#20623,.F.);
#30467=ORIENTED_EDGE('',*,*,#21085,.T.);
#30468=ORIENTED_EDGE('',*,*,#21086,.T.);
#30469=ORIENTED_EDGE('',*,*,#20679,.T.);
#30470=ORIENTED_EDGE('',*,*,#20684,.F.);
#30471=ORIENTED_EDGE('',*,*,#21087,.F.);
#30472=ORIENTED_EDGE('',*,*,#21087,.T.);
#30473=ORIENTED_EDGE('',*,*,#20691,.F.);
#30474=ORIENTED_EDGE('',*,*,#21067,.F.);
#30475=ORIENTED_EDGE('',*,*,#21088,.T.);
#30476=ORIENTED_EDGE('',*,*,#21078,.T.);
#30477=ORIENTED_EDGE('',*,*,#20637,.T.);
#30478=ORIENTED_EDGE('',*,*,#21083,.F.);
#30479=ORIENTED_EDGE('',*,*,#21089,.F.);
#30480=ORIENTED_EDGE('',*,*,#20680,.F.);
#30481=ORIENTED_EDGE('',*,*,#21086,.F.);
#30482=ORIENTED_EDGE('',*,*,#21090,.T.);
#30483=ORIENTED_EDGE('',*,*,#20361,.T.);
#30484=ORIENTED_EDGE('',*,*,#21091,.T.);
#30485=ORIENTED_EDGE('',*,*,#21092,.T.);
#30486=ORIENTED_EDGE('',*,*,#21093,.F.);
#30487=ORIENTED_EDGE('',*,*,#19950,.F.);
#30488=ORIENTED_EDGE('',*,*,#20077,.T.);
#30489=ORIENTED_EDGE('',*,*,#21094,.T.);
#30490=ORIENTED_EDGE('',*,*,#21095,.F.);
#30491=ORIENTED_EDGE('',*,*,#19967,.F.);
#30492=ORIENTED_EDGE('',*,*,#20060,.T.);
#30493=ORIENTED_EDGE('',*,*,#21096,.T.);
#30494=ORIENTED_EDGE('',*,*,#20080,.F.);
#30495=ORIENTED_EDGE('',*,*,#19975,.F.);
#30496=ORIENTED_EDGE('',*,*,#21097,.T.);
#30497=ORIENTED_EDGE('',*,*,#21098,.T.);
#30498=ORIENTED_EDGE('',*,*,#20052,.F.);
#30499=ORIENTED_EDGE('',*,*,#19982,.F.);
#30500=ORIENTED_EDGE('',*,*,#21093,.T.);
#30501=ORIENTED_EDGE('',*,*,#21099,.T.);
#30502=ORIENTED_EDGE('',*,*,#21097,.F.);
#30503=ORIENTED_EDGE('',*,*,#19986,.F.);
#30504=ORIENTED_EDGE('',*,*,#21100,.T.);
#30505=ORIENTED_EDGE('',*,*,#21101,.T.);
#30506=ORIENTED_EDGE('',*,*,#21091,.F.);
#30507=ORIENTED_EDGE('',*,*,#20630,.F.);
#30508=ORIENTED_EDGE('',*,*,#21102,.T.);
#30509=ORIENTED_EDGE('',*,*,#21103,.T.);
#30510=ORIENTED_EDGE('',*,*,#21100,.F.);
#30511=ORIENTED_EDGE('',*,*,#20632,.F.);
#30512=ORIENTED_EDGE('',*,*,#21095,.T.);
#30513=ORIENTED_EDGE('',*,*,#21104,.T.);
#30514=ORIENTED_EDGE('',*,*,#21105,.F.);
#30515=ORIENTED_EDGE('',*,*,#20648,.F.);
#30516=ORIENTED_EDGE('',*,*,#21105,.T.);
#30517=ORIENTED_EDGE('',*,*,#21106,.T.);
#30518=ORIENTED_EDGE('',*,*,#20767,.F.);
#30519=ORIENTED_EDGE('',*,*,#20650,.F.);
#30520=ORIENTED_EDGE('',*,*,#20773,.T.);
#30521=ORIENTED_EDGE('',*,*,#21107,.T.);
#30522=ORIENTED_EDGE('',*,*,#20750,.F.);
#30523=ORIENTED_EDGE('',*,*,#20658,.F.);
#30524=ORIENTED_EDGE('',*,*,#20746,.T.);
#30525=ORIENTED_EDGE('',*,*,#21108,.T.);
#30526=ORIENTED_EDGE('',*,*,#21109,.F.);
#30527=ORIENTED_EDGE('',*,*,#20667,.F.);
#30528=ORIENTED_EDGE('',*,*,#21109,.T.);
#30529=ORIENTED_EDGE('',*,*,#21110,.T.);
#30530=ORIENTED_EDGE('',*,*,#21102,.F.);
#30531=ORIENTED_EDGE('',*,*,#20671,.F.);
#30532=ORIENTED_EDGE('',*,*,#21085,.F.);
#30533=ORIENTED_EDGE('',*,*,#20627,.F.);
#30534=ORIENTED_EDGE('',*,*,#20833,.F.);
#30535=ORIENTED_EDGE('',*,*,#21053,.F.);
#30536=ORIENTED_EDGE('',*,*,#20835,.F.);
#30537=ORIENTED_EDGE('',*,*,#20829,.F.);
#30538=ORIENTED_EDGE('',*,*,#20826,.F.);
#30539=ORIENTED_EDGE('',*,*,#20713,.F.);
#30540=ORIENTED_EDGE('',*,*,#20619,.T.);
#30541=ORIENTED_EDGE('',*,*,#19941,.F.);
#30542=ORIENTED_EDGE('',*,*,#20022,.T.);
#30543=ORIENTED_EDGE('',*,*,#20136,.T.);
#30544=ORIENTED_EDGE('',*,*,#20139,.T.);
#30545=ORIENTED_EDGE('',*,*,#20145,.T.);
#30546=ORIENTED_EDGE('',*,*,#20326,.T.);
#30547=ORIENTED_EDGE('',*,*,#20141,.T.);
#30548=ORIENTED_EDGE('',*,*,#19945,.T.);
#30549=ORIENTED_EDGE('',*,*,#20358,.T.);
#30550=ORIENTED_EDGE('',*,*,#20363,.F.);
#30551=ORIENTED_EDGE('',*,*,#20355,.F.);
#30552=ORIENTED_EDGE('',*,*,#20373,.T.);
#30553=ORIENTED_EDGE('',*,*,#20376,.T.);
#30554=ORIENTED_EDGE('',*,*,#20379,.T.);
#30555=ORIENTED_EDGE('',*,*,#20382,.T.);
#30556=ORIENTED_EDGE('',*,*,#20385,.T.);
#30557=ORIENTED_EDGE('',*,*,#20388,.T.);
#30558=ORIENTED_EDGE('',*,*,#20392,.T.);
#30559=ORIENTED_EDGE('',*,*,#20349,.T.);
#30560=ORIENTED_EDGE('',*,*,#20347,.T.);
#30561=ORIENTED_EDGE('',*,*,#20330,.T.);
#30562=ORIENTED_EDGE('',*,*,#20332,.T.);
#30563=ORIENTED_EDGE('',*,*,#20334,.T.);
#30564=ORIENTED_EDGE('',*,*,#20336,.T.);
#30565=ORIENTED_EDGE('',*,*,#20338,.T.);
#30566=ORIENTED_EDGE('',*,*,#20344,.T.);
#30567=ORIENTED_EDGE('',*,*,#20345,.T.);
#30568=ORIENTED_EDGE('',*,*,#20341,.T.);
#30569=ORIENTED_EDGE('',*,*,#20362,.T.);
#30570=ORIENTED_EDGE('',*,*,#21090,.F.);
#30571=ORIENTED_EDGE('',*,*,#21088,.F.);
#30572=ORIENTED_EDGE('',*,*,#21069,.F.);
#30573=ORIENTED_EDGE('',*,*,#21072,.F.);
#30574=ORIENTED_EDGE('',*,*,#21070,.F.);
#30575=ORIENTED_EDGE('',*,*,#21064,.F.);
#30576=ORIENTED_EDGE('',*,*,#21062,.F.);
#30577=ORIENTED_EDGE('',*,*,#21060,.F.);
#30578=ORIENTED_EDGE('',*,*,#21058,.F.);
#30579=ORIENTED_EDGE('',*,*,#21056,.F.);
#30580=ORIENTED_EDGE('',*,*,#21073,.F.);
#30581=ORIENTED_EDGE('',*,*,#21075,.F.);
#30582=ORIENTED_EDGE('',*,*,#21111,.F.);
#30583=ORIENTED_EDGE('',*,*,#21112,.F.);
#30584=ORIENTED_EDGE('',*,*,#21113,.F.);
#30585=ORIENTED_EDGE('',*,*,#21114,.F.);
#30586=ORIENTED_EDGE('',*,*,#21115,.F.);
#30587=ORIENTED_EDGE('',*,*,#21116,.F.);
#30588=ORIENTED_EDGE('',*,*,#21117,.F.);
#30589=ORIENTED_EDGE('',*,*,#21081,.T.);
#30590=ORIENTED_EDGE('',*,*,#21089,.T.);
#30591=ORIENTED_EDGE('',*,*,#20034,.F.);
#30592=ORIENTED_EDGE('',*,*,#20037,.F.);
#30593=ORIENTED_EDGE('',*,*,#20043,.F.);
#30594=ORIENTED_EDGE('',*,*,#20046,.F.);
#30595=ORIENTED_EDGE('',*,*,#20040,.F.);
#30596=ORIENTED_EDGE('',*,*,#20024,.F.);
#30597=ORIENTED_EDGE('',*,*,#20028,.F.);
#30598=ORIENTED_EDGE('',*,*,#20031,.F.);
#30599=ORIENTED_EDGE('',*,*,#20739,.T.);
#30600=ORIENTED_EDGE('',*,*,#20737,.T.);
#30601=ORIENTED_EDGE('',*,*,#20731,.T.);
#30602=ORIENTED_EDGE('',*,*,#20728,.T.);
#30603=ORIENTED_EDGE('',*,*,#20725,.T.);
#30604=ORIENTED_EDGE('',*,*,#20722,.T.);
#30605=ORIENTED_EDGE('',*,*,#20719,.T.);
#30606=ORIENTED_EDGE('',*,*,#20734,.T.);
#30607=ORIENTED_EDGE('',*,*,#20614,.F.);
#30608=ORIENTED_EDGE('',*,*,#20596,.F.);
#30609=ORIENTED_EDGE('',*,*,#20610,.F.);
#30610=ORIENTED_EDGE('',*,*,#20608,.F.);
#30611=ORIENTED_EDGE('',*,*,#20616,.F.);
#30612=ORIENTED_EDGE('',*,*,#20604,.F.);
#30613=ORIENTED_EDGE('',*,*,#20615,.F.);
#30614=ORIENTED_EDGE('',*,*,#20600,.F.);
#30615=ORIENTED_EDGE('',*,*,#21107,.F.);
#30616=ORIENTED_EDGE('',*,*,#20778,.T.);
#30617=ORIENTED_EDGE('',*,*,#20793,.T.);
#30618=ORIENTED_EDGE('',*,*,#20798,.T.);
#30619=ORIENTED_EDGE('',*,*,#20796,.T.);
#30620=ORIENTED_EDGE('',*,*,#20790,.T.);
#30621=ORIENTED_EDGE('',*,*,#20787,.T.);
#30622=ORIENTED_EDGE('',*,*,#20784,.T.);
#30623=ORIENTED_EDGE('',*,*,#20781,.T.);
#30624=ORIENTED_EDGE('',*,*,#20774,.T.);
#30625=ORIENTED_EDGE('',*,*,#21106,.F.);
#30626=ORIENTED_EDGE('',*,*,#21104,.F.);
#30627=ORIENTED_EDGE('',*,*,#21094,.F.);
#30628=ORIENTED_EDGE('',*,*,#20086,.F.);
#30629=ORIENTED_EDGE('',*,*,#20087,.F.);
#30630=ORIENTED_EDGE('',*,*,#20090,.F.);
#30631=ORIENTED_EDGE('',*,*,#20093,.F.);
#30632=ORIENTED_EDGE('',*,*,#20096,.F.);
#30633=ORIENTED_EDGE('',*,*,#20102,.F.);
#30634=ORIENTED_EDGE('',*,*,#20105,.F.);
#30635=ORIENTED_EDGE('',*,*,#20099,.F.);
#30636=ORIENTED_EDGE('',*,*,#20082,.F.);
#30637=ORIENTED_EDGE('',*,*,#21096,.F.);
#30638=ORIENTED_EDGE('',*,*,#20066,.T.);
#30639=ORIENTED_EDGE('',*,*,#20072,.T.);
#30640=ORIENTED_EDGE('',*,*,#20074,.T.);
#30641=ORIENTED_EDGE('',*,*,#20068,.T.);
#30642=ORIENTED_EDGE('',*,*,#20050,.T.);
#30643=ORIENTED_EDGE('',*,*,#20055,.T.);
#30644=ORIENTED_EDGE('',*,*,#21098,.F.);
#30645=ORIENTED_EDGE('',*,*,#21099,.F.);
#30646=ORIENTED_EDGE('',*,*,#21092,.F.);
#30647=ORIENTED_EDGE('',*,*,#21101,.F.);
#30648=ORIENTED_EDGE('',*,*,#21103,.F.);
#30649=ORIENTED_EDGE('',*,*,#21110,.F.);
#30650=ORIENTED_EDGE('',*,*,#21108,.F.);
#30651=ORIENTED_EDGE('',*,*,#20749,.F.);
#30652=ORIENTED_EDGE('',*,*,#20741,.F.);
#30653=ORIENTED_EDGE('',*,*,#20760,.F.);
#30654=ORIENTED_EDGE('',*,*,#20765,.F.);
#30655=ORIENTED_EDGE('',*,*,#20762,.F.);
#30656=ORIENTED_EDGE('',*,*,#20756,.F.);
#30657=ORIENTED_EDGE('',*,*,#19931,.T.);
#30658=ORIENTED_EDGE('',*,*,#19917,.T.);
#30659=ORIENTED_EDGE('',*,*,#19935,.T.);
#30660=ORIENTED_EDGE('',*,*,#19921,.T.);
#30661=ORIENTED_EDGE('',*,*,#19936,.T.);
#30662=ORIENTED_EDGE('',*,*,#19925,.T.);
#30663=ORIENTED_EDGE('',*,*,#19937,.T.);
#30664=ORIENTED_EDGE('',*,*,#19929,.T.);
#30665=ORIENTED_EDGE('',*,*,#21118,.F.);
#30666=ORIENTED_EDGE('',*,*,#21119,.T.);
#30667=ORIENTED_EDGE('',*,*,#20457,.T.);
#30668=ORIENTED_EDGE('',*,*,#21120,.F.);
#30669=ORIENTED_EDGE('',*,*,#20476,.T.);
#30670=ORIENTED_EDGE('',*,*,#21121,.T.);
#30671=ORIENTED_EDGE('',*,*,#21122,.F.);
#30672=ORIENTED_EDGE('',*,*,#21123,.F.);
#30673=ORIENTED_EDGE('',*,*,#20480,.T.);
#30674=ORIENTED_EDGE('',*,*,#21082,.T.);
#30675=ORIENTED_EDGE('',*,*,#21124,.F.);
#30676=ORIENTED_EDGE('',*,*,#21121,.F.);
#30677=ORIENTED_EDGE('',*,*,#21117,.T.);
#30678=ORIENTED_EDGE('',*,*,#21125,.F.);
#30679=ORIENTED_EDGE('',*,*,#21126,.F.);
#30680=ORIENTED_EDGE('',*,*,#21122,.T.);
#30681=ORIENTED_EDGE('',*,*,#21124,.T.);
#30682=ORIENTED_EDGE('',*,*,#21125,.T.);
#30683=ORIENTED_EDGE('',*,*,#21116,.T.);
#30684=ORIENTED_EDGE('',*,*,#21127,.F.);
#30685=ORIENTED_EDGE('',*,*,#21128,.F.);
#30686=ORIENTED_EDGE('',*,*,#21127,.T.);
#30687=ORIENTED_EDGE('',*,*,#21115,.T.);
#30688=ORIENTED_EDGE('',*,*,#21129,.F.);
#30689=ORIENTED_EDGE('',*,*,#21130,.F.);
#30690=ORIENTED_EDGE('',*,*,#21129,.T.);
#30691=ORIENTED_EDGE('',*,*,#21114,.T.);
#30692=ORIENTED_EDGE('',*,*,#21131,.F.);
#30693=ORIENTED_EDGE('',*,*,#21132,.F.);
#30694=ORIENTED_EDGE('',*,*,#21131,.T.);
#30695=ORIENTED_EDGE('',*,*,#21113,.T.);
#30696=ORIENTED_EDGE('',*,*,#21133,.F.);
#30697=ORIENTED_EDGE('',*,*,#21134,.F.);
#30698=ORIENTED_EDGE('',*,*,#21133,.T.);
#30699=ORIENTED_EDGE('',*,*,#21112,.T.);
#30700=ORIENTED_EDGE('',*,*,#21135,.F.);
#30701=ORIENTED_EDGE('',*,*,#21136,.F.);
#30702=ORIENTED_EDGE('',*,*,#21137,.T.);
#30703=ORIENTED_EDGE('',*,*,#21076,.T.);
#30704=ORIENTED_EDGE('',*,*,#20450,.F.);
#30705=ORIENTED_EDGE('',*,*,#21138,.F.);
#30706=ORIENTED_EDGE('',*,*,#21139,.T.);
#30707=ORIENTED_EDGE('',*,*,#21138,.T.);
#30708=ORIENTED_EDGE('',*,*,#20456,.F.);
#30709=ORIENTED_EDGE('',*,*,#21140,.F.);
#30710=ORIENTED_EDGE('',*,*,#21135,.T.);
#30711=ORIENTED_EDGE('',*,*,#21111,.T.);
#30712=ORIENTED_EDGE('',*,*,#21137,.F.);
#30713=ORIENTED_EDGE('',*,*,#21139,.F.);
#30714=ORIENTED_EDGE('',*,*,#21119,.F.);
#30715=ORIENTED_EDGE('',*,*,#21141,.F.);
#30716=ORIENTED_EDGE('',*,*,#21142,.F.);
#30717=ORIENTED_EDGE('',*,*,#21143,.F.);
#30718=ORIENTED_EDGE('',*,*,#20498,.F.);
#30719=ORIENTED_EDGE('',*,*,#20458,.T.);
#30720=ORIENTED_EDGE('',*,*,#21118,.T.);
#30721=ORIENTED_EDGE('',*,*,#21144,.F.);
#30722=ORIENTED_EDGE('',*,*,#21145,.F.);
#30723=ORIENTED_EDGE('',*,*,#21141,.T.);
#30724=ORIENTED_EDGE('',*,*,#21120,.T.);
#30725=ORIENTED_EDGE('',*,*,#20460,.F.);
#30726=ORIENTED_EDGE('',*,*,#20503,.F.);
#30727=ORIENTED_EDGE('',*,*,#20462,.T.);
#30728=ORIENTED_EDGE('',*,*,#21146,.F.);
#30729=ORIENTED_EDGE('',*,*,#21144,.T.);
#30730=ORIENTED_EDGE('',*,*,#20477,.T.);
#30731=ORIENTED_EDGE('',*,*,#21123,.T.);
#30732=ORIENTED_EDGE('',*,*,#21147,.F.);
#30733=ORIENTED_EDGE('',*,*,#21148,.F.);
#30734=ORIENTED_EDGE('',*,*,#21147,.T.);
#30735=ORIENTED_EDGE('',*,*,#21126,.T.);
#30736=ORIENTED_EDGE('',*,*,#21149,.T.);
#30737=ORIENTED_EDGE('',*,*,#21150,.F.);
#30738=ORIENTED_EDGE('',*,*,#21128,.T.);
#30739=ORIENTED_EDGE('',*,*,#21151,.T.);
#30740=ORIENTED_EDGE('',*,*,#21152,.T.);
#30741=ORIENTED_EDGE('',*,*,#21149,.F.);
#30742=ORIENTED_EDGE('',*,*,#21153,.T.);
#30743=ORIENTED_EDGE('',*,*,#21154,.F.);
#30744=ORIENTED_EDGE('',*,*,#21151,.F.);
#30745=ORIENTED_EDGE('',*,*,#21130,.T.);
#30746=ORIENTED_EDGE('',*,*,#21132,.T.);
#30747=ORIENTED_EDGE('',*,*,#21155,.T.);
#30748=ORIENTED_EDGE('',*,*,#21156,.T.);
#30749=ORIENTED_EDGE('',*,*,#21153,.F.);
#30750=ORIENTED_EDGE('',*,*,#21157,.T.);
#30751=ORIENTED_EDGE('',*,*,#21158,.F.);
#30752=ORIENTED_EDGE('',*,*,#21155,.F.);
#30753=ORIENTED_EDGE('',*,*,#21134,.T.);
#30754=ORIENTED_EDGE('',*,*,#21136,.T.);
#30755=ORIENTED_EDGE('',*,*,#21159,.T.);
#30756=ORIENTED_EDGE('',*,*,#21160,.T.);
#30757=ORIENTED_EDGE('',*,*,#21157,.F.);
#30758=ORIENTED_EDGE('',*,*,#21159,.F.);
#30759=ORIENTED_EDGE('',*,*,#21140,.T.);
#30760=ORIENTED_EDGE('',*,*,#20455,.T.);
#30761=ORIENTED_EDGE('',*,*,#20492,.F.);
#30762=ORIENTED_EDGE('',*,*,#21161,.T.);
#30763=ORIENTED_EDGE('',*,*,#21162,.F.);
#30764=ORIENTED_EDGE('',*,*,#21163,.F.);
#30765=ORIENTED_EDGE('',*,*,#21161,.F.);
#30766=ORIENTED_EDGE('',*,*,#20495,.F.);
#30767=ORIENTED_EDGE('',*,*,#21143,.T.);
#30768=ORIENTED_EDGE('',*,*,#21164,.T.);
#30769=ORIENTED_EDGE('',*,*,#21163,.T.);
#30770=ORIENTED_EDGE('',*,*,#21165,.F.);
#30771=ORIENTED_EDGE('',*,*,#21165,.T.);
#30772=ORIENTED_EDGE('',*,*,#21142,.T.);
#30773=ORIENTED_EDGE('',*,*,#21166,.T.);
#30774=ORIENTED_EDGE('',*,*,#21167,.F.);
#30775=ORIENTED_EDGE('',*,*,#21145,.T.);
#30776=ORIENTED_EDGE('',*,*,#21168,.T.);
#30777=ORIENTED_EDGE('',*,*,#21169,.F.);
#30778=ORIENTED_EDGE('',*,*,#21166,.F.);
#30779=ORIENTED_EDGE('',*,*,#20461,.T.);
#30780=ORIENTED_EDGE('',*,*,#21170,.T.);
#30781=ORIENTED_EDGE('',*,*,#21171,.F.);
#30782=ORIENTED_EDGE('',*,*,#21171,.T.);
#30783=ORIENTED_EDGE('',*,*,#21172,.F.);
#30784=ORIENTED_EDGE('',*,*,#21168,.F.);
#30785=ORIENTED_EDGE('',*,*,#21146,.T.);
#30786=ORIENTED_EDGE('',*,*,#21148,.T.);
#30787=ORIENTED_EDGE('',*,*,#21173,.F.);
#30788=ORIENTED_EDGE('',*,*,#21174,.F.);
#30789=ORIENTED_EDGE('',*,*,#21173,.T.);
#30790=ORIENTED_EDGE('',*,*,#21150,.T.);
#30791=ORIENTED_EDGE('',*,*,#21175,.T.);
#30792=ORIENTED_EDGE('',*,*,#21176,.F.);
#30793=ORIENTED_EDGE('',*,*,#21177,.T.);
#30794=ORIENTED_EDGE('',*,*,#21175,.F.);
#30795=ORIENTED_EDGE('',*,*,#21152,.F.);
#30796=ORIENTED_EDGE('',*,*,#21178,.T.);
#30797=ORIENTED_EDGE('',*,*,#21179,.F.);
#30798=ORIENTED_EDGE('',*,*,#21177,.F.);
#30799=ORIENTED_EDGE('',*,*,#21154,.T.);
#30800=ORIENTED_EDGE('',*,*,#21180,.T.);
#30801=ORIENTED_EDGE('',*,*,#21178,.F.);
#30802=ORIENTED_EDGE('',*,*,#21156,.F.);
#30803=ORIENTED_EDGE('',*,*,#21180,.F.);
#30804=ORIENTED_EDGE('',*,*,#21158,.T.);
#30805=ORIENTED_EDGE('',*,*,#21181,.T.);
#30806=ORIENTED_EDGE('',*,*,#21182,.F.);
#30807=ORIENTED_EDGE('',*,*,#21183,.T.);
#30808=ORIENTED_EDGE('',*,*,#21181,.F.);
#30809=ORIENTED_EDGE('',*,*,#21160,.F.);
#30810=ORIENTED_EDGE('',*,*,#21183,.F.);
#30811=ORIENTED_EDGE('',*,*,#21162,.T.);
#30812=ORIENTED_EDGE('',*,*,#21164,.F.);
#30813=ORIENTED_EDGE('',*,*,#21184,.F.);
#30814=ORIENTED_EDGE('',*,*,#20465,.T.);
#30815=ORIENTED_EDGE('',*,*,#21185,.T.);
#30816=ORIENTED_EDGE('',*,*,#21186,.F.);
#30817=ORIENTED_EDGE('',*,*,#21170,.F.);
#30818=ORIENTED_EDGE('',*,*,#20470,.T.);
#30819=ORIENTED_EDGE('',*,*,#21187,.T.);
#30820=ORIENTED_EDGE('',*,*,#21188,.F.);
#30821=ORIENTED_EDGE('',*,*,#21185,.F.);
#30822=ORIENTED_EDGE('',*,*,#20471,.T.);
#30823=ORIENTED_EDGE('',*,*,#21189,.T.);
#30824=ORIENTED_EDGE('',*,*,#21190,.F.);
#30825=ORIENTED_EDGE('',*,*,#21187,.F.);
#30826=ORIENTED_EDGE('',*,*,#20478,.T.);
#30827=ORIENTED_EDGE('',*,*,#21174,.T.);
#30828=ORIENTED_EDGE('',*,*,#21191,.F.);
#30829=ORIENTED_EDGE('',*,*,#21189,.F.);
#30830=ORIENTED_EDGE('',*,*,#21186,.T.);
#30831=ORIENTED_EDGE('',*,*,#21188,.T.);
#30832=ORIENTED_EDGE('',*,*,#21190,.T.);
#30833=ORIENTED_EDGE('',*,*,#21191,.T.);
#30834=ORIENTED_EDGE('',*,*,#21176,.T.);
#30835=ORIENTED_EDGE('',*,*,#21179,.T.);
#30836=ORIENTED_EDGE('',*,*,#21182,.T.);
#30837=ORIENTED_EDGE('',*,*,#21184,.T.);
#30838=ORIENTED_EDGE('',*,*,#21167,.T.);
#30839=ORIENTED_EDGE('',*,*,#21169,.T.);
#30840=ORIENTED_EDGE('',*,*,#21172,.T.);
#33285=ADVANCED_FACE('',(#4537),#2941,.T.);
#33286=ADVANCED_FACE('',(#4538),#2942,.F.);
#33287=ADVANCED_FACE('',(#4539),#2943,.T.);
#33288=ADVANCED_FACE('',(#4540),#2944,.F.);
#33289=ADVANCED_FACE('',(#4541),#2945,.F.);
#33290=ADVANCED_FACE('',(#4542),#2374,.T.);
#33291=ADVANCED_FACE('',(#4543),#2946,.T.);
#33292=ADVANCED_FACE('',(#4544),#2947,.F.);
#33293=ADVANCED_FACE('',(#4545),#2948,.T.);
#33294=ADVANCED_FACE('',(#4546),#2375,.F.);
#33295=ADVANCED_FACE('',(#4547),#2949,.T.);
#33296=ADVANCED_FACE('',(#4548),#759,.T.);
#33297=ADVANCED_FACE('',(#4549),#217,.T.);
#33298=ADVANCED_FACE('',(#4550),#760,.T.);
#33299=ADVANCED_FACE('',(#4551),#2950,.T.);
#33300=ADVANCED_FACE('',(#4552),#218,.T.);
#33301=ADVANCED_FACE('',(#4553),#219,.T.);
#33302=ADVANCED_FACE('',(#4554),#220,.T.);
#33303=ADVANCED_FACE('',(#4555),#221,.T.);
#33304=ADVANCED_FACE('',(#4556),#222,.T.);
#33305=ADVANCED_FACE('',(#4557),#2951,.T.);
#33306=ADVANCED_FACE('',(#4558),#761,.T.);
#33307=ADVANCED_FACE('',(#4559),#223,.T.);
#33308=ADVANCED_FACE('',(#4560),#762,.T.);
#33309=ADVANCED_FACE('',(#4561),#2952,.T.);
#33310=ADVANCED_FACE('',(#4562),#2376,.T.);
#33311=ADVANCED_FACE('',(#4563),#2377,.T.);
#33312=ADVANCED_FACE('',(#4564),#2953,.T.);
#33313=ADVANCED_FACE('',(#4565),#2954,.F.);
#33314=ADVANCED_FACE('',(#4566),#2955,.T.);
#33315=ADVANCED_FACE('',(#4567),#2378,.F.);
#33316=ADVANCED_FACE('',(#4568),#2956,.F.);
#33317=ADVANCED_FACE('',(#4569),#2957,.T.);
#33318=ADVANCED_FACE('',(#4570),#2958,.T.);
#33319=ADVANCED_FACE('',(#4571),#763,.T.);
#33320=ADVANCED_FACE('',(#4572),#224,.T.);
#33321=ADVANCED_FACE('',(#4573),#764,.T.);
#33322=ADVANCED_FACE('',(#4574),#2959,.T.);
#33323=ADVANCED_FACE('',(#4575),#225,.T.);
#33324=ADVANCED_FACE('',(#4576),#226,.T.);
#33325=ADVANCED_FACE('',(#4577),#765,.T.);
#33326=ADVANCED_FACE('',(#4578),#227,.T.);
#33327=ADVANCED_FACE('',(#4579),#2960,.F.);
#33328=ADVANCED_FACE('',(#4580),#228,.F.);
#33329=ADVANCED_FACE('',(#4581),#2961,.F.);
#33330=ADVANCED_FACE('',(#4582),#229,.F.);
#33331=ADVANCED_FACE('',(#4583),#766,.F.);
#33332=ADVANCED_FACE('',(#4584),#2379,.F.);
#33333=ADVANCED_FACE('',(#4585),#767,.F.);
#33334=ADVANCED_FACE('',(#4586),#2962,.T.);
#33335=ADVANCED_FACE('',(#4587),#768,.F.);
#33336=ADVANCED_FACE('',(#4588),#2380,.F.);
#33337=ADVANCED_FACE('',(#4589),#769,.F.);
#33338=ADVANCED_FACE('',(#4590),#2963,.F.);
#33339=ADVANCED_FACE('',(#4591),#2964,.F.);
#33340=ADVANCED_FACE('',(#4592),#2965,.T.);
#33341=ADVANCED_FACE('',(#4593),#2966,.F.);
#33342=ADVANCED_FACE('',(#4594),#230,.T.);
#33343=ADVANCED_FACE('',(#4595),#2967,.F.);
#33344=ADVANCED_FACE('',(#4596),#2968,.T.);
#33345=ADVANCED_FACE('',(#4597),#2969,.F.);
#33346=ADVANCED_FACE('',(#4598),#231,.T.);
#33347=ADVANCED_FACE('',(#4599),#232,.T.);
#33348=ADVANCED_FACE('',(#4600),#770,.F.);
#33349=ADVANCED_FACE('',(#4601),#233,.T.);
#33350=ADVANCED_FACE('',(#4602),#234,.T.);
#33351=ADVANCED_FACE('',(#4603),#235,.T.);
#33352=ADVANCED_FACE('',(#4604),#236,.T.);
#33353=ADVANCED_FACE('',(#4605),#2381,.F.);
#33354=ADVANCED_FACE('',(#4606),#1192,.T.);
#33355=ADVANCED_FACE('',(#4607),#237,.T.);
#33356=ADVANCED_FACE('',(#4608),#2382,.F.);
#33357=ADVANCED_FACE('',(#4609),#2970,.T.);
#33358=ADVANCED_FACE('',(#4610),#2383,.F.);
#33359=ADVANCED_FACE('',(#4611),#2971,.F.);
#33360=ADVANCED_FACE('',(#4612),#2384,.F.);
#33361=ADVANCED_FACE('',(#4613),#2972,.F.);
#33362=ADVANCED_FACE('',(#4614),#2385,.F.);
#33363=ADVANCED_FACE('',(#4615),#2973,.F.);
#33364=ADVANCED_FACE('',(#4616),#771,.T.);
#33365=ADVANCED_FACE('',(#4617),#238,.T.);
#33366=ADVANCED_FACE('',(#4618),#2974,.T.);
#33367=ADVANCED_FACE('',(#4619),#2386,.F.);
#33368=ADVANCED_FACE('',(#4620),#2975,.F.);
#33369=ADVANCED_FACE('',(#4621),#2976,.T.);
#33370=ADVANCED_FACE('',(#4622),#2977,.F.);
#33371=ADVANCED_FACE('',(#4623),#2387,.F.);
#33372=ADVANCED_FACE('',(#4624),#2978,.F.);
#33373=ADVANCED_FACE('',(#4625),#2979,.F.);
#33374=ADVANCED_FACE('',(#4626),#2980,.F.);
#33375=ADVANCED_FACE('',(#4627),#2981,.T.);
#33376=ADVANCED_FACE('',(#4628),#239,.T.);
#33377=ADVANCED_FACE('',(#4629),#240,.T.);
#33378=ADVANCED_FACE('',(#4630),#2982,.T.);
#33379=ADVANCED_FACE('',(#4631),#241,.T.);
#33380=ADVANCED_FACE('',(#4632),#242,.T.);
#33381=ADVANCED_FACE('',(#4633),#243,.T.);
#33382=ADVANCED_FACE('',(#4634),#244,.T.);
#33383=ADVANCED_FACE('',(#4635),#2983,.T.);
#33384=ADVANCED_FACE('',(#4636),#245,.T.);
#33385=ADVANCED_FACE('',(#4637),#1193,.F.);
#33386=ADVANCED_FACE('',(#4638),#246,.T.);
#33387=ADVANCED_FACE('',(#4639),#1194,.F.);
#33388=ADVANCED_FACE('',(#4640),#1195,.F.);
#33389=ADVANCED_FACE('',(#4641),#1196,.F.);
#33390=ADVANCED_FACE('',(#4642),#247,.T.);
#33391=ADVANCED_FACE('',(#4643),#248,.T.);
#33392=ADVANCED_FACE('',(#4644),#249,.T.);
#33393=ADVANCED_FACE('',(#4645),#2984,.T.);
#33394=ADVANCED_FACE('',(#4646),#1197,.F.);
#33395=ADVANCED_FACE('',(#4647),#1198,.F.);
#33396=ADVANCED_FACE('',(#4648),#1199,.F.);
#33397=ADVANCED_FACE('',(#4649),#250,.T.);
#33398=ADVANCED_FACE('',(#4650),#251,.T.);
#33399=ADVANCED_FACE('',(#4651),#2985,.T.);
#33400=ADVANCED_FACE('',(#4652),#252,.T.);
#33401=ADVANCED_FACE('',(#4653),#253,.T.);
#33402=ADVANCED_FACE('',(#4654),#254,.T.);
#33403=ADVANCED_FACE('',(#4655),#255,.T.);
#33404=ADVANCED_FACE('',(#4656),#2986,.T.);
#33405=ADVANCED_FACE('',(#4657),#2987,.F.);
#33406=ADVANCED_FACE('',(#4658),#2988,.F.);
#33407=ADVANCED_FACE('',(#4659),#256,.F.);
#33408=ADVANCED_FACE('',(#4660),#772,.F.);
#33409=ADVANCED_FACE('',(#4661),#257,.F.);
#33410=ADVANCED_FACE('',(#4662),#773,.F.);
#33411=ADVANCED_FACE('',(#4663),#774,.F.);
#33412=ADVANCED_FACE('',(#4664),#775,.F.);
#33413=ADVANCED_FACE('',(#4665),#2989,.F.);
#33414=ADVANCED_FACE('',(#4666),#258,.F.);
#33415=ADVANCED_FACE('',(#4667),#259,.T.);
#33416=ADVANCED_FACE('',(#4668),#260,.T.);
#33417=ADVANCED_FACE('',(#4669),#261,.T.);
#33418=ADVANCED_FACE('',(#4670),#262,.T.);
#33419=ADVANCED_FACE('',(#4671),#776,.F.);
#33420=ADVANCED_FACE('',(#4672),#2990,.T.);
#33421=ADVANCED_FACE('',(#4673),#777,.T.);
#33422=ADVANCED_FACE('',(#4674),#263,.F.);
#33423=ADVANCED_FACE('',(#4675),#2991,.F.);
#33424=ADVANCED_FACE('',(#4676),#264,.F.);
#33425=ADVANCED_FACE('',(#4677),#2388,.T.);
#33426=ADVANCED_FACE('',(#4678),#265,.T.);
#33427=ADVANCED_FACE('',(#4679),#266,.T.);
#33428=ADVANCED_FACE('',(#4680),#267,.T.);
#33429=ADVANCED_FACE('',(#4681),#268,.T.);
#33430=ADVANCED_FACE('',(#4682),#2992,.T.);
#33431=ADVANCED_FACE('',(#4683),#778,.T.);
#33432=ADVANCED_FACE('',(#4684),#269,.T.);
#33433=ADVANCED_FACE('',(#4685),#270,.T.);
#33434=ADVANCED_FACE('',(#4686),#2993,.T.);
#33435=ADVANCED_FACE('',(#4687),#1200,.F.);
#33436=ADVANCED_FACE('',(#4688),#271,.T.);
#33437=ADVANCED_FACE('',(#4689),#1201,.F.);
#33438=ADVANCED_FACE('',(#4690),#779,.T.);
#33439=ADVANCED_FACE('',(#4691),#2994,.T.);
#33440=ADVANCED_FACE('',(#4692),#2995,.T.);
#33441=ADVANCED_FACE('',(#4693),#780,.T.);
#33442=ADVANCED_FACE('',(#4694),#2996,.T.);
#33443=ADVANCED_FACE('',(#4695),#2997,.T.);
#33444=ADVANCED_FACE('',(#4696),#2389,.F.);
#33445=ADVANCED_FACE('',(#4697),#1202,.F.);
#33446=ADVANCED_FACE('',(#4698),#2998,.F.);
#33447=ADVANCED_FACE('',(#4699),#2999,.F.);
#33448=ADVANCED_FACE('',(#4700),#781,.F.);
#33449=ADVANCED_FACE('',(#4701),#272,.F.);
#33450=ADVANCED_FACE('',(#4702),#782,.F.);
#33451=ADVANCED_FACE('',(#4703),#3000,.F.);
#33452=ADVANCED_FACE('',(#4704),#783,.F.);
#33453=ADVANCED_FACE('',(#4705),#784,.F.);
#33454=ADVANCED_FACE('',(#4706),#273,.F.);
#33455=ADVANCED_FACE('',(#4707),#2390,.F.);
#33456=ADVANCED_FACE('',(#4708),#785,.F.);
#33457=ADVANCED_FACE('',(#4709),#2391,.F.);
#33458=ADVANCED_FACE('',(#4710),#3001,.T.);
#33459=ADVANCED_FACE('',(#4711),#3002,.F.);
#33460=ADVANCED_FACE('',(#4712),#2392,.F.);
#33461=ADVANCED_FACE('',(#4713),#3003,.F.);
#33462=ADVANCED_FACE('',(#4714),#3004,.F.);
#33463=ADVANCED_FACE('',(#4715),#3005,.F.);
#33464=ADVANCED_FACE('',(#4716),#3006,.F.);
#33465=ADVANCED_FACE('',(#4717),#2393,.F.);
#33466=ADVANCED_FACE('',(#4718),#3007,.F.);
#33467=ADVANCED_FACE('',(#4719),#3008,.F.);
#33468=ADVANCED_FACE('',(#4720),#3009,.T.);
#33469=ADVANCED_FACE('',(#4721),#3010,.F.);
#33470=ADVANCED_FACE('',(#4722),#3011,.F.);
#33471=ADVANCED_FACE('',(#4723),#2394,.F.);
#33472=ADVANCED_FACE('',(#4724),#3012,.T.);
#33473=ADVANCED_FACE('',(#4725),#3013,.F.);
#33474=ADVANCED_FACE('',(#4726),#2395,.T.);
#33475=ADVANCED_FACE('',(#4727),#3014,.F.);
#33476=ADVANCED_FACE('',(#4728),#3015,.F.);
#33477=ADVANCED_FACE('',(#4729),#3016,.F.);
#33478=ADVANCED_FACE('',(#4730),#3017,.F.);
#33479=ADVANCED_FACE('',(#4731),#2396,.T.);
#33480=ADVANCED_FACE('',(#4732),#786,.F.);
#33481=ADVANCED_FACE('',(#4733),#274,.F.);
#33482=ADVANCED_FACE('',(#4734),#787,.F.);
#33483=ADVANCED_FACE('',(#4735),#788,.F.);
#33484=ADVANCED_FACE('',(#4736),#3018,.F.);
#33485=ADVANCED_FACE('',(#4737),#2397,.F.);
#33486=ADVANCED_FACE('',(#4738),#789,.T.);
#33487=ADVANCED_FACE('',(#4739),#790,.F.);
#33488=ADVANCED_FACE('',(#4740),#2398,.F.);
#33489=ADVANCED_FACE('',(#4741),#2399,.F.);
#33490=ADVANCED_FACE('',(#4742),#3019,.F.);
#33491=ADVANCED_FACE('',(#4743),#3020,.F.);
#33492=ADVANCED_FACE('',(#4744),#791,.F.);
#33493=ADVANCED_FACE('',(#4745),#275,.F.);
#33494=ADVANCED_FACE('',(#4746),#3021,.T.);
#33495=ADVANCED_FACE('',(#4747),#1203,.T.);
#33496=ADVANCED_FACE('',(#4748),#3022,.F.);
#33497=ADVANCED_FACE('',(#4749),#3023,.F.);
#33498=ADVANCED_FACE('',(#4750),#792,.F.);
#33499=ADVANCED_FACE('',(#4751),#276,.F.);
#33500=ADVANCED_FACE('',(#4752),#277,.T.);
#33501=ADVANCED_FACE('',(#4753),#793,.F.);
#33502=ADVANCED_FACE('',(#4754),#3024,.F.);
#33503=ADVANCED_FACE('',(#4755),#3025,.T.);
#33504=ADVANCED_FACE('',(#4756),#278,.F.);
#33505=ADVANCED_FACE('',(#4757),#3026,.F.);
#33506=ADVANCED_FACE('',(#4758),#279,.F.);
#33507=ADVANCED_FACE('',(#4759),#280,.F.);
#33508=ADVANCED_FACE('',(#4760),#281,.F.);
#33509=ADVANCED_FACE('',(#4761),#3027,.F.);
#33510=ADVANCED_FACE('',(#4762),#794,.F.);
#33511=ADVANCED_FACE('',(#4763),#282,.F.);
#33512=ADVANCED_FACE('',(#4764),#795,.F.);
#33513=ADVANCED_FACE('',(#4765),#283,.F.);
#33514=ADVANCED_FACE('',(#4766),#3028,.F.);
#33515=ADVANCED_FACE('',(#4767),#3029,.F.);
#33516=ADVANCED_FACE('',(#4768),#3030,.F.);
#33517=ADVANCED_FACE('',(#4769),#3031,.F.);
#33518=ADVANCED_FACE('',(#4770),#796,.F.);
#33519=ADVANCED_FACE('',(#4771),#3032,.F.);
#33520=ADVANCED_FACE('',(#4772),#2400,.T.);
#33521=ADVANCED_FACE('',(#4773),#3033,.T.);
#33522=ADVANCED_FACE('',(#4774),#1204,.F.);
#33523=ADVANCED_FACE('',(#4775),#3034,.T.);
#33524=ADVANCED_FACE('',(#4776),#284,.T.);
#33525=ADVANCED_FACE('',(#4777),#285,.T.);
#33526=ADVANCED_FACE('',(#4778),#286,.T.);
#33527=ADVANCED_FACE('',(#4779),#3035,.T.);
#33528=ADVANCED_FACE('',(#4780),#1205,.F.);
#33529=ADVANCED_FACE('',(#4781),#287,.T.);
#33530=ADVANCED_FACE('',(#4782),#288,.T.);
#33531=ADVANCED_FACE('',(#4783),#289,.T.);
#33532=ADVANCED_FACE('',(#4784),#290,.F.);
#33533=ADVANCED_FACE('',(#4785),#291,.F.);
#33534=ADVANCED_FACE('',(#4786),#1206,.F.);
#33535=ADVANCED_FACE('',(#4787),#1207,.F.);
#33536=ADVANCED_FACE('',(#4788),#3036,.F.);
#33537=ADVANCED_FACE('',(#4789),#1208,.F.);
#33538=ADVANCED_FACE('',(#4790),#3037,.F.);
#33539=ADVANCED_FACE('',(#4791),#1209,.F.);
#33540=ADVANCED_FACE('',(#4792),#3038,.F.);
#33541=ADVANCED_FACE('',(#4793),#292,.T.);
#33542=ADVANCED_FACE('',(#4794),#293,.T.);
#33543=ADVANCED_FACE('',(#4795),#1210,.F.);
#33544=ADVANCED_FACE('',(#4796),#1211,.F.);
#33545=ADVANCED_FACE('',(#4797),#294,.T.);
#33546=ADVANCED_FACE('',(#4798),#295,.T.);
#33547=ADVANCED_FACE('',(#4799),#3039,.T.);
#33548=ADVANCED_FACE('',(#4800),#296,.T.);
#33549=ADVANCED_FACE('',(#4801),#297,.T.);
#33550=ADVANCED_FACE('',(#4802),#298,.T.);
#33551=ADVANCED_FACE('',(#4803),#1212,.T.);
#33552=ADVANCED_FACE('',(#4804),#1213,.F.);
#33553=ADVANCED_FACE('',(#4805),#3040,.T.);
#33554=ADVANCED_FACE('',(#4806),#3041,.F.);
#33555=ADVANCED_FACE('',(#4807),#3042,.F.);
#33556=ADVANCED_FACE('',(#4808),#3043,.F.);
#33557=ADVANCED_FACE('',(#4809),#3044,.F.);
#33558=ADVANCED_FACE('',(#4810),#3045,.F.);
#33559=ADVANCED_FACE('',(#4811),#3046,.F.);
#33560=ADVANCED_FACE('',(#4812),#2401,.T.);
#33561=ADVANCED_FACE('',(#4813),#3047,.F.);
#33562=ADVANCED_FACE('',(#4814),#3048,.T.);
#33563=ADVANCED_FACE('',(#4815),#3049,.F.);
#33564=ADVANCED_FACE('',(#4816),#2402,.T.);
#33565=ADVANCED_FACE('',(#4817),#3050,.F.);
#33566=ADVANCED_FACE('',(#4818),#797,.F.);
#33567=ADVANCED_FACE('',(#4819),#299,.F.);
#33568=ADVANCED_FACE('',(#4820),#300,.F.);
#33569=ADVANCED_FACE('',(#4821),#798,.F.);
#33570=ADVANCED_FACE('',(#4822),#301,.F.);
#33571=ADVANCED_FACE('',(#4823),#799,.F.);
#33572=ADVANCED_FACE('',(#4824),#302,.F.);
#33573=ADVANCED_FACE('',(#4825),#800,.F.);
#33574=ADVANCED_FACE('',(#4826),#3051,.F.);
#33575=ADVANCED_FACE('',(#4827),#801,.F.);
#33576=ADVANCED_FACE('',(#4828),#303,.F.);
#33577=ADVANCED_FACE('',(#4829),#802,.F.);
#33578=ADVANCED_FACE('',(#4830),#3052,.F.);
#33579=ADVANCED_FACE('',(#4831),#3053,.F.);
#33580=ADVANCED_FACE('',(#4832),#304,.F.);
#33581=ADVANCED_FACE('',(#4833),#305,.F.);
#33582=ADVANCED_FACE('',(#4834),#306,.F.);
#33583=ADVANCED_FACE('',(#4835),#2403,.F.);
#33584=ADVANCED_FACE('',(#4836),#3054,.T.);
#33585=ADVANCED_FACE('',(#4837),#3055,.F.);
#33586=ADVANCED_FACE('',(#4838),#3056,.T.);
#33587=ADVANCED_FACE('',(#4839),#3057,.F.);
#33588=ADVANCED_FACE('',(#4840),#3058,.F.);
#33589=ADVANCED_FACE('',(#4841),#2404,.F.);
#33590=ADVANCED_FACE('',(#4842),#3059,.T.);
#33591=ADVANCED_FACE('',(#4843),#3060,.F.);
#33592=ADVANCED_FACE('',(#4844),#3061,.T.);
#33593=ADVANCED_FACE('',(#4845),#2405,.T.);
#33594=ADVANCED_FACE('',(#4846),#3062,.T.);
#33595=ADVANCED_FACE('',(#4847),#803,.T.);
#33596=ADVANCED_FACE('',(#4848),#307,.T.);
#33597=ADVANCED_FACE('',(#4849),#804,.T.);
#33598=ADVANCED_FACE('',(#4850),#3063,.T.);
#33599=ADVANCED_FACE('',(#4851),#308,.T.);
#33600=ADVANCED_FACE('',(#4852),#309,.T.);
#33601=ADVANCED_FACE('',(#4853),#310,.T.);
#33602=ADVANCED_FACE('',(#4854),#311,.T.);
#33603=ADVANCED_FACE('',(#4855),#312,.T.);
#33604=ADVANCED_FACE('',(#4856),#3064,.T.);
#33605=ADVANCED_FACE('',(#4857),#805,.T.);
#33606=ADVANCED_FACE('',(#4858),#313,.T.);
#33607=ADVANCED_FACE('',(#4859),#806,.T.);
#33608=ADVANCED_FACE('',(#4860),#3065,.T.);
#33609=ADVANCED_FACE('',(#4861),#2406,.T.);
#33610=ADVANCED_FACE('',(#4862),#2407,.F.);
#33611=ADVANCED_FACE('',(#4863),#3066,.T.);
#33612=ADVANCED_FACE('',(#4864),#3067,.F.);
#33613=ADVANCED_FACE('',(#4865),#3068,.T.);
#33614=ADVANCED_FACE('',(#4866),#2408,.T.);
#33615=ADVANCED_FACE('',(#4867),#3069,.F.);
#33616=ADVANCED_FACE('',(#4868),#3070,.T.);
#33617=ADVANCED_FACE('',(#4869),#3071,.T.);
#33618=ADVANCED_FACE('',(#4870),#807,.T.);
#33619=ADVANCED_FACE('',(#4871),#314,.T.);
#33620=ADVANCED_FACE('',(#4872),#808,.T.);
#33621=ADVANCED_FACE('',(#4873),#3072,.T.);
#33622=ADVANCED_FACE('',(#4874),#315,.T.);
#33623=ADVANCED_FACE('',(#4875),#1214,.F.);
#33624=ADVANCED_FACE('',(#4876),#316,.T.);
#33625=ADVANCED_FACE('',(#4877),#809,.T.);
#33626=ADVANCED_FACE('',(#4878),#1215,.F.);
#33627=ADVANCED_FACE('',(#4879),#317,.T.);
#33628=ADVANCED_FACE('',(#4880),#2409,.T.);
#33629=ADVANCED_FACE('',(#4881),#3073,.F.);
#33630=ADVANCED_FACE('',(#4882),#318,.F.);
#33631=ADVANCED_FACE('',(#4883),#3074,.F.);
#33632=ADVANCED_FACE('',(#4884),#319,.F.);
#33633=ADVANCED_FACE('',(#4885),#810,.F.);
#33634=ADVANCED_FACE('',(#4886),#2410,.T.);
#33635=ADVANCED_FACE('',(#4887),#811,.F.);
#33636=ADVANCED_FACE('',(#4888),#3075,.T.);
#33637=ADVANCED_FACE('',(#4889),#812,.F.);
#33638=ADVANCED_FACE('',(#4890),#2411,.F.);
#33639=ADVANCED_FACE('',(#4891),#813,.F.);
#33640=ADVANCED_FACE('',(#4892),#3076,.F.);
#33641=ADVANCED_FACE('',(#4893),#3077,.F.);
#33642=ADVANCED_FACE('',(#4894),#3078,.T.);
#33643=ADVANCED_FACE('',(#4895),#3079,.F.);
#33644=ADVANCED_FACE('',(#4896),#320,.T.);
#33645=ADVANCED_FACE('',(#4897),#3080,.F.);
#33646=ADVANCED_FACE('',(#4898),#3081,.T.);
#33647=ADVANCED_FACE('',(#4899),#3082,.F.);
#33648=ADVANCED_FACE('',(#4900),#321,.T.);
#33649=ADVANCED_FACE('',(#4901),#322,.T.);
#33650=ADVANCED_FACE('',(#4902),#814,.F.);
#33651=ADVANCED_FACE('',(#4903),#323,.T.);
#33652=ADVANCED_FACE('',(#4904),#324,.T.);
#33653=ADVANCED_FACE('',(#4905),#325,.T.);
#33654=ADVANCED_FACE('',(#4906),#1216,.F.);
#33655=ADVANCED_FACE('',(#4907),#326,.T.);
#33656=ADVANCED_FACE('',(#4908),#2412,.F.);
#33657=ADVANCED_FACE('',(#4909),#1217,.F.);
#33658=ADVANCED_FACE('',(#4910),#327,.T.);
#33659=ADVANCED_FACE('',(#4911),#3083,.F.);
#33660=ADVANCED_FACE('',(#4912),#2413,.T.);
#33661=ADVANCED_FACE('',(#4913),#3084,.T.);
#33662=ADVANCED_FACE('',(#4914),#3085,.T.);
#33663=ADVANCED_FACE('',(#4915),#3086,.F.);
#33664=ADVANCED_FACE('',(#4916),#2414,.T.);
#33665=ADVANCED_FACE('',(#4917),#3087,.F.);
#33666=ADVANCED_FACE('',(#4918),#2415,.T.);
#33667=ADVANCED_FACE('',(#4919),#3088,.F.);
#33668=ADVANCED_FACE('',(#4920),#2416,.T.);
#33669=ADVANCED_FACE('',(#4921),#3089,.F.);
#33670=ADVANCED_FACE('',(#4922),#815,.T.);
#33671=ADVANCED_FACE('',(#4923),#328,.T.);
#33672=ADVANCED_FACE('',(#4924),#3090,.T.);
#33673=ADVANCED_FACE('',(#4925),#3091,.T.);
#33674=ADVANCED_FACE('',(#4926),#2417,.T.);
#33675=ADVANCED_FACE('',(#4927),#3092,.F.);
#33676=ADVANCED_FACE('',(#4928),#3093,.T.);
#33677=ADVANCED_FACE('',(#4929),#3094,.F.);
#33678=ADVANCED_FACE('',(#4930),#2418,.T.);
#33679=ADVANCED_FACE('',(#4931),#3095,.F.);
#33680=ADVANCED_FACE('',(#4932),#3096,.F.);
#33681=ADVANCED_FACE('',(#4933),#3097,.F.);
#33682=ADVANCED_FACE('',(#4934),#3098,.T.);
#33683=ADVANCED_FACE('',(#4935),#329,.T.);
#33684=ADVANCED_FACE('',(#4936),#330,.T.);
#33685=ADVANCED_FACE('',(#4937),#3099,.T.);
#33686=ADVANCED_FACE('',(#4938),#331,.T.);
#33687=ADVANCED_FACE('',(#4939),#332,.T.);
#33688=ADVANCED_FACE('',(#4940),#333,.T.);
#33689=ADVANCED_FACE('',(#4941),#334,.T.);
#33690=ADVANCED_FACE('',(#4942),#3100,.T.);
#33691=ADVANCED_FACE('',(#4943),#335,.T.);
#33692=ADVANCED_FACE('',(#4944),#1218,.F.);
#33693=ADVANCED_FACE('',(#4945),#336,.T.);
#33694=ADVANCED_FACE('',(#4946),#1219,.F.);
#33695=ADVANCED_FACE('',(#4947),#1220,.T.);
#33696=ADVANCED_FACE('',(#4948),#1221,.F.);
#33697=ADVANCED_FACE('',(#4949),#337,.T.);
#33698=ADVANCED_FACE('',(#4950),#338,.T.);
#33699=ADVANCED_FACE('',(#4951),#339,.T.);
#33700=ADVANCED_FACE('',(#4952),#3101,.T.);
#33701=ADVANCED_FACE('',(#4953),#1222,.F.);
#33702=ADVANCED_FACE('',(#4954),#1223,.T.);
#33703=ADVANCED_FACE('',(#4955),#1224,.F.);
#33704=ADVANCED_FACE('',(#4956),#340,.T.);
#33705=ADVANCED_FACE('',(#4957),#341,.T.);
#33706=ADVANCED_FACE('',(#4958),#3102,.T.);
#33707=ADVANCED_FACE('',(#4959),#342,.T.);
#33708=ADVANCED_FACE('',(#4960),#343,.T.);
#33709=ADVANCED_FACE('',(#4961),#344,.T.);
#33710=ADVANCED_FACE('',(#4962),#345,.T.);
#33711=ADVANCED_FACE('',(#4963),#3103,.T.);
#33712=ADVANCED_FACE('',(#4964),#3104,.F.);
#33713=ADVANCED_FACE('',(#4965),#3105,.F.);
#33714=ADVANCED_FACE('',(#4966),#346,.F.);
#33715=ADVANCED_FACE('',(#4967),#816,.F.);
#33716=ADVANCED_FACE('',(#4968),#347,.F.);
#33717=ADVANCED_FACE('',(#4969),#817,.F.);
#33718=ADVANCED_FACE('',(#4970),#818,.F.);
#33719=ADVANCED_FACE('',(#4971),#819,.F.);
#33720=ADVANCED_FACE('',(#4972),#3106,.F.);
#33721=ADVANCED_FACE('',(#4973),#348,.F.);
#33722=ADVANCED_FACE('',(#4974),#349,.T.);
#33723=ADVANCED_FACE('',(#4975),#350,.T.);
#33724=ADVANCED_FACE('',(#4976),#351,.T.);
#33725=ADVANCED_FACE('',(#4977),#352,.T.);
#33726=ADVANCED_FACE('',(#4978),#820,.F.);
#33727=ADVANCED_FACE('',(#4979),#3107,.T.);
#33728=ADVANCED_FACE('',(#4980),#3108,.T.);
#33729=ADVANCED_FACE('',(#4981),#821,.T.);
#33730=ADVANCED_FACE('',(#4982),#1225,.T.);
#33731=ADVANCED_FACE('',(#4983),#353,.F.);
#33732=ADVANCED_FACE('',(#4984),#3109,.F.);
#33733=ADVANCED_FACE('',(#4985),#354,.F.);
#33734=ADVANCED_FACE('',(#4986),#2419,.T.);
#33735=ADVANCED_FACE('',(#4987),#355,.T.);
#33736=ADVANCED_FACE('',(#4988),#356,.T.);
#33737=ADVANCED_FACE('',(#4989),#3110,.T.);
#33738=ADVANCED_FACE('',(#4990),#3111,.T.);
#33739=ADVANCED_FACE('',(#4991),#357,.T.);
#33740=ADVANCED_FACE('',(#4992),#3112,.T.);
#33741=ADVANCED_FACE('',(#4993),#358,.T.);
#33742=ADVANCED_FACE('',(#4994),#3113,.T.);
#33743=ADVANCED_FACE('',(#4995),#359,.T.);
#33744=ADVANCED_FACE('',(#4996),#360,.T.);
#33745=ADVANCED_FACE('',(#4997),#3114,.T.);
#33746=ADVANCED_FACE('',(#4998),#361,.T.);
#33747=ADVANCED_FACE('',(#4999),#3115,.T.);
#33748=ADVANCED_FACE('',(#5000),#362,.T.);
#33749=ADVANCED_FACE('',(#5001),#3116,.T.);
#33750=ADVANCED_FACE('',(#5002),#363,.T.);
#33751=ADVANCED_FACE('',(#5003),#3117,.T.);
#33752=ADVANCED_FACE('',(#5004),#364,.T.);
#33753=ADVANCED_FACE('',(#5005,#1309),#2420,.F.);
#33754=ADVANCED_FACE('',(#5006),#1226,.F.);
#33755=ADVANCED_FACE('',(#5007),#365,.T.);
#33756=ADVANCED_FACE('',(#5008),#366,.T.);
#33757=ADVANCED_FACE('',(#5009),#3118,.T.);
#33758=ADVANCED_FACE('',(#5010),#822,.T.);
#33759=ADVANCED_FACE('',(#5011),#367,.T.);
#33760=ADVANCED_FACE('',(#5012),#368,.T.);
#33761=ADVANCED_FACE('',(#5013),#3119,.T.);
#33762=ADVANCED_FACE('',(#5014),#1227,.T.);
#33763=ADVANCED_FACE('',(#5015),#369,.T.);
#33764=ADVANCED_FACE('',(#5016),#1228,.T.);
#33765=ADVANCED_FACE('',(#5017),#823,.T.);
#33766=ADVANCED_FACE('',(#5018),#3120,.T.);
#33767=ADVANCED_FACE('',(#5019),#3121,.T.);
#33768=ADVANCED_FACE('',(#5020),#3122,.T.);
#33769=ADVANCED_FACE('',(#5021),#2421,.F.);
#33770=ADVANCED_FACE('',(#5022),#3123,.F.);
#33771=ADVANCED_FACE('',(#5023),#370,.T.);
#33772=ADVANCED_FACE('',(#5024),#2422,.T.);
#33773=ADVANCED_FACE('',(#5025),#824,.T.);
#33774=ADVANCED_FACE('',(#5026),#3124,.T.);
#33775=ADVANCED_FACE('',(#5027),#3125,.T.);
#33776=ADVANCED_FACE('',(#5028),#2423,.T.);
#33777=ADVANCED_FACE('',(#5029),#1229,.T.);
#33778=ADVANCED_FACE('',(#5030),#3126,.F.);
#33779=ADVANCED_FACE('',(#5031),#3127,.F.);
#33780=ADVANCED_FACE('',(#5032),#825,.F.);
#33781=ADVANCED_FACE('',(#5033),#371,.F.);
#33782=ADVANCED_FACE('',(#5034),#826,.F.);
#33783=ADVANCED_FACE('',(#5035),#3128,.F.);
#33784=ADVANCED_FACE('',(#5036),#827,.F.);
#33785=ADVANCED_FACE('',(#5037),#828,.F.);
#33786=ADVANCED_FACE('',(#5038),#372,.F.);
#33787=ADVANCED_FACE('',(#5039),#2424,.F.);
#33788=ADVANCED_FACE('',(#5040),#829,.F.);
#33789=ADVANCED_FACE('',(#5041),#2425,.T.);
#33790=ADVANCED_FACE('',(#5042),#3129,.T.);
#33791=ADVANCED_FACE('',(#5043),#3130,.F.);
#33792=ADVANCED_FACE('',(#5044),#2426,.T.);
#33793=ADVANCED_FACE('',(#5045),#3131,.F.);
#33794=ADVANCED_FACE('',(#5046),#3132,.F.);
#33795=ADVANCED_FACE('',(#5047),#3133,.F.);
#33796=ADVANCED_FACE('',(#5048),#3134,.F.);
#33797=ADVANCED_FACE('',(#5049),#2427,.T.);
#33798=ADVANCED_FACE('',(#5050),#3135,.F.);
#33799=ADVANCED_FACE('',(#5051),#3136,.F.);
#33800=ADVANCED_FACE('',(#5052),#3137,.T.);
#33801=ADVANCED_FACE('',(#5053),#3138,.F.);
#33802=ADVANCED_FACE('',(#5054),#3139,.F.);
#33803=ADVANCED_FACE('',(#5055),#2428,.F.);
#33804=ADVANCED_FACE('',(#5056),#3140,.T.);
#33805=ADVANCED_FACE('',(#5057),#3141,.F.);
#33806=ADVANCED_FACE('',(#5058),#2429,.F.);
#33807=ADVANCED_FACE('',(#5059),#3142,.F.);
#33808=ADVANCED_FACE('',(#5060),#3143,.F.);
#33809=ADVANCED_FACE('',(#5061),#3144,.F.);
#33810=ADVANCED_FACE('',(#5062),#3145,.F.);
#33811=ADVANCED_FACE('',(#5063),#2430,.T.);
#33812=ADVANCED_FACE('',(#5064),#830,.F.);
#33813=ADVANCED_FACE('',(#5065),#373,.F.);
#33814=ADVANCED_FACE('',(#5066),#831,.F.);
#33815=ADVANCED_FACE('',(#5067),#832,.F.);
#33816=ADVANCED_FACE('',(#5068),#3146,.F.);
#33817=ADVANCED_FACE('',(#5069),#2431,.F.);
#33818=ADVANCED_FACE('',(#5070),#833,.T.);
#33819=ADVANCED_FACE('',(#5071),#834,.F.);
#33820=ADVANCED_FACE('',(#5072),#2432,.F.);
#33821=ADVANCED_FACE('',(#5073),#2433,.F.);
#33822=ADVANCED_FACE('',(#5074),#3147,.F.);
#33823=ADVANCED_FACE('',(#5075),#3148,.F.);
#33824=ADVANCED_FACE('',(#5076),#835,.F.);
#33825=ADVANCED_FACE('',(#5077),#374,.F.);
#33826=ADVANCED_FACE('',(#5078),#3149,.T.);
#33827=ADVANCED_FACE('',(#5079),#1230,.F.);
#33828=ADVANCED_FACE('',(#5080),#3150,.F.);
#33829=ADVANCED_FACE('',(#5081),#3151,.F.);
#33830=ADVANCED_FACE('',(#5082),#836,.F.);
#33831=ADVANCED_FACE('',(#5083),#375,.F.);
#33832=ADVANCED_FACE('',(#5084),#376,.T.);
#33833=ADVANCED_FACE('',(#5085),#837,.F.);
#33834=ADVANCED_FACE('',(#5086),#3152,.F.);
#33835=ADVANCED_FACE('',(#5087),#3153,.T.);
#33836=ADVANCED_FACE('',(#5088),#377,.F.);
#33837=ADVANCED_FACE('',(#5089),#3154,.F.);
#33838=ADVANCED_FACE('',(#5090),#378,.F.);
#33839=ADVANCED_FACE('',(#5091),#379,.F.);
#33840=ADVANCED_FACE('',(#5092),#380,.F.);
#33841=ADVANCED_FACE('',(#5093),#3155,.F.);
#33842=ADVANCED_FACE('',(#5094),#2434,.F.);
#33843=ADVANCED_FACE('',(#5095),#838,.F.);
#33844=ADVANCED_FACE('',(#5096),#381,.F.);
#33845=ADVANCED_FACE('',(#5097),#839,.F.);
#33846=ADVANCED_FACE('',(#5098),#1231,.T.);
#33847=ADVANCED_FACE('',(#5099),#382,.F.);
#33848=ADVANCED_FACE('',(#5100),#3156,.F.);
#33849=ADVANCED_FACE('',(#5101),#3157,.F.);
#33850=ADVANCED_FACE('',(#5102),#3158,.F.);
#33851=ADVANCED_FACE('',(#5103),#3159,.F.);
#33852=ADVANCED_FACE('',(#5104),#3160,.F.);
#33853=ADVANCED_FACE('',(#5105),#840,.F.);
#33854=ADVANCED_FACE('',(#5106),#3161,.F.);
#33855=ADVANCED_FACE('',(#5107),#2435,.F.);
#33856=ADVANCED_FACE('',(#5108),#3162,.T.);
#33857=ADVANCED_FACE('',(#5109),#1232,.T.);
#33858=ADVANCED_FACE('',(#5110),#3163,.T.);
#33859=ADVANCED_FACE('',(#5111),#383,.T.);
#33860=ADVANCED_FACE('',(#5112),#384,.T.);
#33861=ADVANCED_FACE('',(#5113),#385,.T.);
#33862=ADVANCED_FACE('',(#5114),#3164,.T.);
#33863=ADVANCED_FACE('',(#5115),#1233,.T.);
#33864=ADVANCED_FACE('',(#5116),#386,.T.);
#33865=ADVANCED_FACE('',(#5117),#387,.T.);
#33866=ADVANCED_FACE('',(#5118),#388,.T.);
#33867=ADVANCED_FACE('',(#5119),#389,.F.);
#33868=ADVANCED_FACE('',(#5120),#390,.F.);
#33869=ADVANCED_FACE('',(#5121),#1234,.T.);
#33870=ADVANCED_FACE('',(#5122),#1235,.T.);
#33871=ADVANCED_FACE('',(#5123),#3165,.F.);
#33872=ADVANCED_FACE('',(#5124),#1236,.T.);
#33873=ADVANCED_FACE('',(#5125),#3166,.F.);
#33874=ADVANCED_FACE('',(#5126),#1237,.T.);
#33875=ADVANCED_FACE('',(#5127),#3167,.F.);
#33876=ADVANCED_FACE('',(#5128),#391,.T.);
#33877=ADVANCED_FACE('',(#5129),#392,.T.);
#33878=ADVANCED_FACE('',(#5130),#3168,.T.);
#33879=ADVANCED_FACE('',(#5131),#3169,.T.);
#33880=ADVANCED_FACE('',(#5132),#3170,.T.);
#33881=ADVANCED_FACE('',(#5133),#3171,.T.);
#33882=ADVANCED_FACE('',(#5134),#393,.T.);
#33883=ADVANCED_FACE('',(#5135),#394,.T.);
#33884=ADVANCED_FACE('',(#5136),#3172,.T.);
#33885=ADVANCED_FACE('',(#5137),#395,.T.);
#33886=ADVANCED_FACE('',(#5138),#3173,.T.);
#33887=ADVANCED_FACE('',(#5139),#3174,.T.);
#33888=ADVANCED_FACE('',(#5140),#3175,.T.);
#33889=ADVANCED_FACE('',(#5141),#396,.T.);
#33890=ADVANCED_FACE('',(#5142,#1310,#1311,#1312,#1313,#1314),#2436,.T.);
#33891=ADVANCED_FACE('',(#5143),#397,.T.);
#33892=ADVANCED_FACE('',(#5144),#1238,.T.);
#33893=ADVANCED_FACE('',(#5145),#1239,.T.);
#33894=ADVANCED_FACE('',(#5146),#398,.T.);
#33895=ADVANCED_FACE('',(#5147),#399,.T.);
#33896=ADVANCED_FACE('',(#5148),#3176,.T.);
#33897=ADVANCED_FACE('',(#5149),#400,.T.);
#33898=ADVANCED_FACE('',(#5150),#401,.T.);
#33899=ADVANCED_FACE('',(#5151),#402,.T.);
#33900=ADVANCED_FACE('',(#5152),#1240,.F.);
#33901=ADVANCED_FACE('',(#5153),#1241,.T.);
#33902=ADVANCED_FACE('',(#5154),#3177,.T.);
#33903=ADVANCED_FACE('',(#5155),#3178,.F.);
#33904=ADVANCED_FACE('',(#5156),#3179,.F.);
#33905=ADVANCED_FACE('',(#5157),#3180,.F.);
#33906=ADVANCED_FACE('',(#5158),#3181,.F.);
#33907=ADVANCED_FACE('',(#5159),#3182,.F.);
#33908=ADVANCED_FACE('',(#5160),#3183,.F.);
#33909=ADVANCED_FACE('',(#5161),#2437,.T.);
#33910=ADVANCED_FACE('',(#5162),#3184,.F.);
#33911=ADVANCED_FACE('',(#5163),#3185,.T.);
#33912=ADVANCED_FACE('',(#5164),#3186,.F.);
#33913=ADVANCED_FACE('',(#5165),#2438,.F.);
#33914=ADVANCED_FACE('',(#5166),#3187,.F.);
#33915=ADVANCED_FACE('',(#5167),#841,.F.);
#33916=ADVANCED_FACE('',(#5168),#403,.F.);
#33917=ADVANCED_FACE('',(#5169),#404,.F.);
#33918=ADVANCED_FACE('',(#5170),#842,.F.);
#33919=ADVANCED_FACE('',(#5171),#405,.F.);
#33920=ADVANCED_FACE('',(#5172),#843,.F.);
#33921=ADVANCED_FACE('',(#5173),#406,.F.);
#33922=ADVANCED_FACE('',(#5174),#844,.F.);
#33923=ADVANCED_FACE('',(#5175),#3188,.F.);
#33924=ADVANCED_FACE('',(#5176),#845,.F.);
#33925=ADVANCED_FACE('',(#5177),#407,.F.);
#33926=ADVANCED_FACE('',(#5178),#846,.F.);
#33927=ADVANCED_FACE('',(#5179),#3189,.F.);
#33928=ADVANCED_FACE('',(#5180),#3190,.F.);
#33929=ADVANCED_FACE('',(#5181),#408,.F.);
#33930=ADVANCED_FACE('',(#5182),#409,.F.);
#33931=ADVANCED_FACE('',(#5183),#410,.F.);
#33932=ADVANCED_FACE('',(#5184),#2439,.F.);
#34176=CLOSED_SHELL('',(#33285,#33286,#33287,#33288,#33289,#33290,#33291,
#33292,#33293,#33294,#33295,#33296,#33297,#33298,#33299,#33300,#33301,#33302,
#33303,#33304,#33305,#33306,#33307,#33308,#33309,#33310,#33311,#33312,#33313,
#33314,#33315,#33316,#33317,#33318,#33319,#33320,#33321,#33322,#33323,#33324,
#33325,#33326,#33327,#33328,#33329,#33330,#33331,#33332,#33333,#33334,#33335,
#33336,#33337,#33338,#33339,#33340,#33341,#33342,#33343,#33344,#33345,#33346,
#33347,#33348,#33349,#33350,#33351,#33352,#33353,#33354,#33355,#33356,#33357,
#33358,#33359,#33360,#33361,#33362,#33363,#33364,#33365,#33366,#33367,#33368,
#33369,#33370,#33371,#33372,#33373,#33374,#33375,#33376,#33377,#33378,#33379,
#33380,#33381,#33382,#33383,#33384,#33385,#33386,#33387,#33388,#33389,#33390,
#33391,#33392,#33393,#33394,#33395,#33396,#33397,#33398,#33399,#33400,#33401,
#33402,#33403,#33404,#33405,#33406,#33407,#33408,#33409,#33410,#33411,#33412,
#33413,#33414,#33415,#33416,#33417,#33418,#33419,#33420,#33421,#33422,#33423,
#33424,#33425,#33426,#33427,#33428,#33429,#33430,#33431,#33432,#33433,#33434,
#33435,#33436,#33437,#33438,#33439,#33440,#33441,#33442,#33443,#33444,#33445,
#33446,#33447,#33448,#33449,#33450,#33451,#33452,#33453,#33454,#33455,#33456,
#33457,#33458,#33459,#33460,#33461,#33462,#33463,#33464,#33465,#33466,#33467,
#33468,#33469,#33470,#33471,#33472,#33473,#33474,#33475,#33476,#33477,#33478,
#33479,#33480,#33481,#33482,#33483,#33484,#33485,#33486,#33487,#33488,#33489,
#33490,#33491,#33492,#33493,#33494,#33495,#33496,#33497,#33498,#33499,#33500,
#33501,#33502,#33503,#33504,#33505,#33506,#33507,#33508,#33509,#33510,#33511,
#33512,#33513,#33514,#33515,#33516,#33517,#33518,#33519,#33520,#33521,#33522,
#33523,#33524,#33525,#33526,#33527,#33528,#33529,#33530,#33531,#33532,#33533,
#33534,#33535,#33536,#33537,#33538,#33539,#33540,#33541,#33542,#33543,#33544,
#33545,#33546,#33547,#33548,#33549,#33550,#33551,#33552,#33553,#33554,#33555,
#33556,#33557,#33558,#33559,#33560,#33561,#33562,#33563,#33564,#33565,#33566,
#33567,#33568,#33569,#33570,#33571,#33572,#33573,#33574,#33575,#33576,#33577,
#33578,#33579,#33580,#33581,#33582,#33583,#33584,#33585,#33586,#33587,#33588,
#33589,#33590,#33591,#33592,#33593,#33594,#33595,#33596,#33597,#33598,#33599,
#33600,#33601,#33602,#33603,#33604,#33605,#33606,#33607,#33608,#33609,#33610,
#33611,#33612,#33613,#33614,#33615,#33616,#33617,#33618,#33619,#33620,#33621,
#33622,#33623,#33624,#33625,#33626,#33627,#33628,#33629,#33630,#33631,#33632,
#33633,#33634,#33635,#33636,#33637,#33638,#33639,#33640,#33641,#33642,#33643,
#33644,#33645,#33646,#33647,#33648,#33649,#33650,#33651,#33652,#33653,#33654,
#33655,#33656,#33657,#33658,#33659,#33660,#33661,#33662,#33663,#33664,#33665,
#33666,#33667,#33668,#33669,#33670,#33671,#33672,#33673,#33674,#33675,#33676,
#33677,#33678,#33679,#33680,#33681,#33682,#33683,#33684,#33685,#33686,#33687,
#33688,#33689,#33690,#33691,#33692,#33693,#33694,#33695,#33696,#33697,#33698,
#33699,#33700,#33701,#33702,#33703,#33704,#33705,#33706,#33707,#33708,#33709,
#33710,#33711,#33712,#33713,#33714,#33715,#33716,#33717,#33718,#33719,#33720,
#33721,#33722,#33723,#33724,#33725,#33726,#33727,#33728,#33729,#33730,#33731,
#33732,#33733,#33734,#33735,#33736,#33737,#33738,#33739,#33740,#33741,#33742,
#33743,#33744,#33745,#33746,#33747,#33748,#33749,#33750,#33751,#33752,#33753,
#33754,#33755,#33756,#33757,#33758,#33759,#33760,#33761,#33762,#33763,#33764,
#33765,#33766,#33767,#33768,#33769,#33770,#33771,#33772,#33773,#33774,#33775,
#33776,#33777,#33778,#33779,#33780,#33781,#33782,#33783,#33784,#33785,#33786,
#33787,#33788,#33789,#33790,#33791,#33792,#33793,#33794,#33795,#33796,#33797,
#33798,#33799,#33800,#33801,#33802,#33803,#33804,#33805,#33806,#33807,#33808,
#33809,#33810,#33811,#33812,#33813,#33814,#33815,#33816,#33817,#33818,#33819,
#33820,#33821,#33822,#33823,#33824,#33825,#33826,#33827,#33828,#33829,#33830,
#33831,#33832,#33833,#33834,#33835,#33836,#33837,#33838,#33839,#33840,#33841,
#33842,#33843,#33844,#33845,#33846,#33847,#33848,#33849,#33850,#33851,#33852,
#33853,#33854,#33855,#33856,#33857,#33858,#33859,#33860,#33861,#33862,#33863,
#33864,#33865,#33866,#33867,#33868,#33869,#33870,#33871,#33872,#33873,#33874,
#33875,#33876,#33877,#33878,#33879,#33880,#33881,#33882,#33883,#33884,#33885,
#33886,#33887,#33888,#33889,#33890,#33891,#33892,#33893,#33894,#33895,#33896,
#33897,#33898,#33899,#33900,#33901,#33902,#33903,#33904,#33905,#33906,#33907,
#33908,#33909,#33910,#33911,#33912,#33913,#33914,#33915,#33916,#33917,#33918,
#33919,#33920,#33921,#33922,#33923,#33924,#33925,#33926,#33927,#33928,#33929,
#33930,#33931,#33932));
#36602=AXIS2_PLACEMENT_3D('',#85187,#44415,#44416);
#36603=AXIS2_PLACEMENT_3D('',#85188,#44417,#44418);
#36604=AXIS2_PLACEMENT_3D('',#85210,#44419,#44420);
#36605=AXIS2_PLACEMENT_3D('',#85214,#44422,#44423);
#36606=AXIS2_PLACEMENT_3D('',#85216,#44425,#44426);
#36607=AXIS2_PLACEMENT_3D('',#85220,#44428,#44429);
#36608=AXIS2_PLACEMENT_3D('',#85222,#44430,#44431);
#36609=AXIS2_PLACEMENT_3D('',#85223,#44432,#44433);
#36610=AXIS2_PLACEMENT_3D('',#85224,#44434,#44435);
#36611=AXIS2_PLACEMENT_3D('',#85277,#44437,#44438);
#36612=AXIS2_PLACEMENT_3D('',#85278,#44439,#44440);
#36613=AXIS2_PLACEMENT_3D('',#85283,#44442,#44443);
#36614=AXIS2_PLACEMENT_3D('',#85301,#44445,#44446);
#36615=AXIS2_PLACEMENT_3D('',#85306,#44448,#44449);
#36616=AXIS2_PLACEMENT_3D('',#85309,#44451,#44452);
#36617=AXIS2_PLACEMENT_3D('',#85310,#44453,#44454);
#36618=AXIS2_PLACEMENT_3D('',#85316,#44458,#44459);
#36619=AXIS2_PLACEMENT_3D('',#85318,#44460,#44461);
#36620=AXIS2_PLACEMENT_3D('',#85321,#44463,#44464);
#36621=AXIS2_PLACEMENT_3D('',#85322,#44465,#44466);
#36622=AXIS2_PLACEMENT_3D('',#85326,#44468,#44469);
#36623=AXIS2_PLACEMENT_3D('',#85327,#44470,#44471);
#36624=AXIS2_PLACEMENT_3D('',#85328,#44472,#44473);
#36625=AXIS2_PLACEMENT_3D('',#85330,#44474,#44475);
#36626=AXIS2_PLACEMENT_3D('',#85391,#44478,#44479);
#36627=AXIS2_PLACEMENT_3D('',#85392,#44480,#44481);
#36628=AXIS2_PLACEMENT_3D('',#85398,#44484,#44485);
#36629=AXIS2_PLACEMENT_3D('',#85400,#44487,#44488);
#36630=AXIS2_PLACEMENT_3D('',#85457,#44490,#44491);
#36631=AXIS2_PLACEMENT_3D('',#85459,#44493,#44494);
#36632=AXIS2_PLACEMENT_3D('',#85460,#44495,#44496);
#36633=AXIS2_PLACEMENT_3D('',#85461,#44497,#44498);
#36634=AXIS2_PLACEMENT_3D('',#85463,#44499,#44500);
#36635=AXIS2_PLACEMENT_3D('',#85464,#44501,#44502);
#36636=AXIS2_PLACEMENT_3D('',#85465,#44503,#44504);
#36637=AXIS2_PLACEMENT_3D('',#85466,#44505,#44506);
#36638=AXIS2_PLACEMENT_3D('',#85467,#44507,#44508);
#36639=AXIS2_PLACEMENT_3D('',#85472,#44511,#44512);
#36640=AXIS2_PLACEMENT_3D('',#85473,#44513,#44514);
#36641=AXIS2_PLACEMENT_3D('',#85475,#44515,#44516);
#36642=AXIS2_PLACEMENT_3D('',#85477,#44517,#44518);
#36643=AXIS2_PLACEMENT_3D('',#85478,#44519,#44520);
#36644=AXIS2_PLACEMENT_3D('',#85479,#44521,#44522);
#36645=AXIS2_PLACEMENT_3D('',#85481,#44523,#44524);
#36646=AXIS2_PLACEMENT_3D('',#85482,#44525,#44526);
#36647=AXIS2_PLACEMENT_3D('',#85483,#44527,#44528);
#36648=AXIS2_PLACEMENT_3D('',#85484,#44529,#44530);
#36649=AXIS2_PLACEMENT_3D('',#85486,#44531,#44532);
#36650=AXIS2_PLACEMENT_3D('',#85487,#44533,#44534);
#36651=AXIS2_PLACEMENT_3D('',#85488,#44535,#44536);
#36652=AXIS2_PLACEMENT_3D('',#85490,#44537,#44538);
#36653=AXIS2_PLACEMENT_3D('',#85491,#44539,#44540);
#36654=AXIS2_PLACEMENT_3D('',#85492,#44541,#44542);
#36655=AXIS2_PLACEMENT_3D('',#85493,#44543,#44544);
#36656=AXIS2_PLACEMENT_3D('',#85495,#44545,#44546);
#36657=AXIS2_PLACEMENT_3D('',#85496,#44547,#44548);
#36658=AXIS2_PLACEMENT_3D('',#85497,#44549,#44550);
#36659=AXIS2_PLACEMENT_3D('',#85500,#44552,#44553);
#36660=AXIS2_PLACEMENT_3D('',#85501,#44554,#44555);
#36661=AXIS2_PLACEMENT_3D('',#85502,#44556,#44557);
#36662=AXIS2_PLACEMENT_3D('',#85503,#44558,#44559);
#36663=AXIS2_PLACEMENT_3D('',#85505,#44560,#44561);
#36664=AXIS2_PLACEMENT_3D('',#85506,#44562,#44563);
#36665=AXIS2_PLACEMENT_3D('',#85507,#44564,#44565);
#36666=AXIS2_PLACEMENT_3D('',#85508,#44566,#44567);
#36667=AXIS2_PLACEMENT_3D('',#85509,#44568,#44569);
#36668=AXIS2_PLACEMENT_3D('',#85555,#44571,#44572);
#36669=AXIS2_PLACEMENT_3D('',#85557,#44573,#44574);
#36670=AXIS2_PLACEMENT_3D('',#85558,#44575,#44576);
#36671=AXIS2_PLACEMENT_3D('',#85559,#44577,#44578);
#36672=AXIS2_PLACEMENT_3D('',#85616,#44585,#44586);
#36673=AXIS2_PLACEMENT_3D('',#85618,#44587,#44588);
#36674=AXIS2_PLACEMENT_3D('',#85621,#44590,#44591);
#36675=AXIS2_PLACEMENT_3D('',#85622,#44592,#44593);
#36676=AXIS2_PLACEMENT_3D('',#85626,#44595,#44596);
#36677=AXIS2_PLACEMENT_3D('',#85627,#44597,#44598);
#36678=AXIS2_PLACEMENT_3D('',#85628,#44599,#44600);
#36679=AXIS2_PLACEMENT_3D('',#85630,#44601,#44602);
#36680=AXIS2_PLACEMENT_3D('',#85633,#44604,#44605);
#36681=AXIS2_PLACEMENT_3D('',#85634,#44606,#44607);
#36682=AXIS2_PLACEMENT_3D('',#85640,#44611,#44612);
#36683=AXIS2_PLACEMENT_3D('',#85644,#44614,#44615);
#36684=AXIS2_PLACEMENT_3D('',#85682,#44616,#44617);
#36685=AXIS2_PLACEMENT_3D('',#85684,#44618,#44619);
#36686=AXIS2_PLACEMENT_3D('',#85686,#44620,#44621);
#36687=AXIS2_PLACEMENT_3D('',#85688,#44623,#44624);
#36688=AXIS2_PLACEMENT_3D('',#85692,#44626,#44627);
#36689=AXIS2_PLACEMENT_3D('',#85693,#44628,#44629);
#36690=AXIS2_PLACEMENT_3D('',#85694,#44630,#44631);
#36691=AXIS2_PLACEMENT_3D('',#85695,#44632,#44633);
#36692=AXIS2_PLACEMENT_3D('',#85696,#44634,#44635);
#36693=AXIS2_PLACEMENT_3D('',#85698,#44636,#44637);
#36694=AXIS2_PLACEMENT_3D('',#85699,#44638,#44639);
#36695=AXIS2_PLACEMENT_3D('',#85700,#44640,#44641);
#36696=AXIS2_PLACEMENT_3D('',#85701,#44642,#44643);
#36697=AXIS2_PLACEMENT_3D('',#85702,#44644,#44645);
#36698=AXIS2_PLACEMENT_3D('',#85705,#44647,#44648);
#36699=AXIS2_PLACEMENT_3D('',#85706,#44649,#44650);
#36700=AXIS2_PLACEMENT_3D('',#85708,#44651,#44652);
#36701=AXIS2_PLACEMENT_3D('',#85709,#44653,#44654);
#36702=AXIS2_PLACEMENT_3D('',#85710,#44655,#44656);
#36703=AXIS2_PLACEMENT_3D('',#85719,#44657,#44658);
#36704=AXIS2_PLACEMENT_3D('',#85720,#44659,#44660);
#36705=AXIS2_PLACEMENT_3D('',#85721,#44661,#44662);
#36706=AXIS2_PLACEMENT_3D('',#85722,#44663,#44664);
#36707=AXIS2_PLACEMENT_3D('',#85723,#44665,#44666);
#36708=AXIS2_PLACEMENT_3D('',#85820,#44667,#44668);
#36709=AXIS2_PLACEMENT_3D('',#85821,#44669,#44670);
#36710=AXIS2_PLACEMENT_3D('',#85822,#44671,#44672);
#36711=AXIS2_PLACEMENT_3D('',#85960,#44675,#44676);
#36712=AXIS2_PLACEMENT_3D('',#85962,#44677,#44678);
#36713=AXIS2_PLACEMENT_3D('',#86023,#44679,#44680);
#36714=AXIS2_PLACEMENT_3D('',#86024,#44681,#44682);
#36715=AXIS2_PLACEMENT_3D('',#86025,#44683,#44684);
#36716=AXIS2_PLACEMENT_3D('',#86077,#44687,#44688);
#36717=AXIS2_PLACEMENT_3D('',#86078,#44689,#44690);
#36718=AXIS2_PLACEMENT_3D('',#86081,#44691,#44692);
#36719=AXIS2_PLACEMENT_3D('',#86191,#44693,#44694);
#36720=AXIS2_PLACEMENT_3D('',#86192,#44695,#44696);
#36721=AXIS2_PLACEMENT_3D('',#86193,#44697,#44698);
#36722=AXIS2_PLACEMENT_3D('',#86194,#44699,#44700);
#36723=AXIS2_PLACEMENT_3D('',#86195,#44701,#44702);
#36724=AXIS2_PLACEMENT_3D('',#86201,#44706,#44707);
#36725=AXIS2_PLACEMENT_3D('',#86202,#44708,#44709);
#36726=AXIS2_PLACEMENT_3D('',#86203,#44710,#44711);
#36727=AXIS2_PLACEMENT_3D('',#86206,#44712,#44713);
#36728=AXIS2_PLACEMENT_3D('',#86209,#44716,#44717);
#36729=AXIS2_PLACEMENT_3D('',#86210,#44718,#44719);
#36730=AXIS2_PLACEMENT_3D('',#86211,#44720,#44721);
#36731=AXIS2_PLACEMENT_3D('',#86217,#44725,#44726);
#36732=AXIS2_PLACEMENT_3D('',#86218,#44727,#44728);
#36733=AXIS2_PLACEMENT_3D('',#86219,#44729,#44730);
#36734=AXIS2_PLACEMENT_3D('',#86224,#44733,#44734);
#36735=AXIS2_PLACEMENT_3D('',#86225,#44735,#44736);
#36736=AXIS2_PLACEMENT_3D('',#86226,#44737,#44738);
#36737=AXIS2_PLACEMENT_3D('',#86227,#44739,#44740);
#36738=AXIS2_PLACEMENT_3D('',#86229,#44741,#44742);
#36739=AXIS2_PLACEMENT_3D('',#86232,#44744,#44745);
#36740=AXIS2_PLACEMENT_3D('',#86233,#44746,#44747);
#36741=AXIS2_PLACEMENT_3D('',#86234,#44748,#44749);
#36742=AXIS2_PLACEMENT_3D('',#86235,#44750,#44751);
#36743=AXIS2_PLACEMENT_3D('',#86237,#44752,#44753);
#36744=AXIS2_PLACEMENT_3D('',#86239,#44754,#44755);
#36745=AXIS2_PLACEMENT_3D('',#86240,#44756,#44757);
#36746=AXIS2_PLACEMENT_3D('',#86241,#44758,#44759);
#36747=AXIS2_PLACEMENT_3D('',#86242,#44760,#44761);
#36748=AXIS2_PLACEMENT_3D('',#86243,#44762,#44763);
#36749=AXIS2_PLACEMENT_3D('',#86245,#44764,#44765);
#36750=AXIS2_PLACEMENT_3D('',#86248,#44767,#44768);
#36751=AXIS2_PLACEMENT_3D('',#86249,#44769,#44770);
#36752=AXIS2_PLACEMENT_3D('',#86250,#44771,#44772);
#36753=AXIS2_PLACEMENT_3D('',#86251,#44773,#44774);
#36754=AXIS2_PLACEMENT_3D('',#86253,#44775,#44776);
#36755=AXIS2_PLACEMENT_3D('',#86255,#44777,#44778);
#36756=AXIS2_PLACEMENT_3D('',#86256,#44779,#44780);
#36757=AXIS2_PLACEMENT_3D('',#86257,#44781,#44782);
#36758=AXIS2_PLACEMENT_3D('',#86258,#44783,#44784);
#36759=AXIS2_PLACEMENT_3D('',#86259,#44785,#44786);
#36760=AXIS2_PLACEMENT_3D('',#86262,#44787,#44788);
#36761=AXIS2_PLACEMENT_3D('',#86264,#44789,#44790);
#36762=AXIS2_PLACEMENT_3D('',#86265,#44791,#44792);
#36763=AXIS2_PLACEMENT_3D('',#86266,#44793,#44794);
#36764=AXIS2_PLACEMENT_3D('',#86267,#44795,#44796);
#36765=AXIS2_PLACEMENT_3D('',#86268,#44797,#44798);
#36766=AXIS2_PLACEMENT_3D('',#86269,#44799,#44800);
#36767=AXIS2_PLACEMENT_3D('',#86270,#44801,#44802);
#36768=AXIS2_PLACEMENT_3D('',#86271,#44803,#44804);
#36769=AXIS2_PLACEMENT_3D('',#86272,#44805,#44806);
#36770=AXIS2_PLACEMENT_3D('',#86282,#44807,#44808);
#36771=AXIS2_PLACEMENT_3D('',#86284,#44809,#44810);
#36772=AXIS2_PLACEMENT_3D('',#86285,#44811,#44812);
#36773=AXIS2_PLACEMENT_3D('',#86286,#44813,#44814);
#36774=AXIS2_PLACEMENT_3D('',#86349,#44815,#44816);
#36775=AXIS2_PLACEMENT_3D('',#86426,#44817,#44818);
#36776=AXIS2_PLACEMENT_3D('',#86428,#44819,#44820);
#36777=AXIS2_PLACEMENT_3D('',#86430,#44821,#44822);
#36778=AXIS2_PLACEMENT_3D('',#86431,#44823,#44824);
#36779=AXIS2_PLACEMENT_3D('',#86432,#44825,#44826);
#36780=AXIS2_PLACEMENT_3D('',#86441,#44831,#44832);
#36781=AXIS2_PLACEMENT_3D('',#86444,#44833,#44834);
#36782=AXIS2_PLACEMENT_3D('',#86507,#44836,#44837);
#36783=AXIS2_PLACEMENT_3D('',#86570,#44839,#44840);
#36784=AXIS2_PLACEMENT_3D('',#86574,#44842,#44843);
#36785=AXIS2_PLACEMENT_3D('',#86576,#44844,#44845);
#36786=AXIS2_PLACEMENT_3D('',#86618,#44847,#44848);
#36787=AXIS2_PLACEMENT_3D('',#86625,#44851,#44852);
#36788=AXIS2_PLACEMENT_3D('',#86629,#44855,#44856);
#36789=AXIS2_PLACEMENT_3D('',#86631,#44857,#44858);
#36790=AXIS2_PLACEMENT_3D('',#86674,#44860,#44861);
#36791=AXIS2_PLACEMENT_3D('',#86680,#44864,#44865);
#36792=AXIS2_PLACEMENT_3D('',#86683,#44867,#44868);
#36793=AXIS2_PLACEMENT_3D('',#86684,#44869,#44870);
#36794=AXIS2_PLACEMENT_3D('',#86686,#44871,#44872);
#36795=AXIS2_PLACEMENT_3D('',#86729,#44874,#44875);
#36796=AXIS2_PLACEMENT_3D('',#86743,#44879,#44880);
#36797=AXIS2_PLACEMENT_3D('',#86744,#44881,#44882);
#36798=AXIS2_PLACEMENT_3D('',#86745,#44883,#44884);
#36799=AXIS2_PLACEMENT_3D('',#86746,#44885,#44886);
#36800=AXIS2_PLACEMENT_3D('',#86747,#44887,#44888);
#36801=AXIS2_PLACEMENT_3D('',#86749,#44889,#44890);
#36802=AXIS2_PLACEMENT_3D('',#86750,#44891,#44892);
#36803=AXIS2_PLACEMENT_3D('',#86751,#44893,#44894);
#36804=AXIS2_PLACEMENT_3D('',#86753,#44895,#44896);
#36805=AXIS2_PLACEMENT_3D('',#86754,#44897,#44898);
#36806=AXIS2_PLACEMENT_3D('',#86755,#44899,#44900);
#36807=AXIS2_PLACEMENT_3D('',#86760,#44903,#44904);
#36808=AXIS2_PLACEMENT_3D('',#86761,#44905,#44906);
#36809=AXIS2_PLACEMENT_3D('',#86765,#44908,#44909);
#36810=AXIS2_PLACEMENT_3D('',#86773,#44914,#44915);
#36811=AXIS2_PLACEMENT_3D('',#86775,#44916,#44917);
#36812=AXIS2_PLACEMENT_3D('',#86778,#44919,#44920);
#36813=AXIS2_PLACEMENT_3D('',#86779,#44921,#44922);
#36814=AXIS2_PLACEMENT_3D('',#86781,#44923,#44924);
#36815=AXIS2_PLACEMENT_3D('',#86783,#44925,#44926);
#36816=AXIS2_PLACEMENT_3D('',#86785,#44928,#44929);
#36817=AXIS2_PLACEMENT_3D('',#86787,#44930,#44931);
#36818=AXIS2_PLACEMENT_3D('',#86790,#44933,#44934);
#36819=AXIS2_PLACEMENT_3D('',#86791,#44935,#44936);
#36820=AXIS2_PLACEMENT_3D('',#86797,#44940,#44941);
#36821=AXIS2_PLACEMENT_3D('',#86801,#44943,#44944);
#36822=AXIS2_PLACEMENT_3D('',#86808,#44945,#44946);
#36823=AXIS2_PLACEMENT_3D('',#86810,#44947,#44948);
#36824=AXIS2_PLACEMENT_3D('',#86813,#44950,#44951);
#36825=AXIS2_PLACEMENT_3D('',#86814,#44952,#44953);
#36826=AXIS2_PLACEMENT_3D('',#86815,#44954,#44955);
#36827=AXIS2_PLACEMENT_3D('',#86816,#44956,#44957);
#36828=AXIS2_PLACEMENT_3D('',#86817,#44958,#44959);
#36829=AXIS2_PLACEMENT_3D('',#86822,#44961,#44962);
#36830=AXIS2_PLACEMENT_3D('',#86824,#44964,#44965);
#36831=AXIS2_PLACEMENT_3D('',#86825,#44966,#44967);
#36832=AXIS2_PLACEMENT_3D('',#86828,#44968,#44969);
#36833=AXIS2_PLACEMENT_3D('',#86830,#44970,#44971);
#36834=AXIS2_PLACEMENT_3D('',#86832,#44972,#44973);
#36835=AXIS2_PLACEMENT_3D('',#86833,#44974,#44975);
#36836=AXIS2_PLACEMENT_3D('',#86834,#44976,#44977);
#36837=AXIS2_PLACEMENT_3D('',#86836,#44978,#44979);
#36838=AXIS2_PLACEMENT_3D('',#86838,#44980,#44981);
#36839=AXIS2_PLACEMENT_3D('',#86839,#44982,#44983);
#36840=AXIS2_PLACEMENT_3D('',#86840,#44984,#44985);
#36841=AXIS2_PLACEMENT_3D('',#86845,#44988,#44989);
#36842=AXIS2_PLACEMENT_3D('',#86846,#44990,#44991);
#36843=AXIS2_PLACEMENT_3D('',#86848,#44992,#44993);
#36844=AXIS2_PLACEMENT_3D('',#86850,#44994,#44995);
#36845=AXIS2_PLACEMENT_3D('',#86851,#44996,#44997);
#36846=AXIS2_PLACEMENT_3D('',#86852,#44998,#44999);
#36847=AXIS2_PLACEMENT_3D('',#86854,#45000,#45001);
#36848=AXIS2_PLACEMENT_3D('',#86856,#45002,#45003);
#36849=AXIS2_PLACEMENT_3D('',#86857,#45004,#45005);
#36850=AXIS2_PLACEMENT_3D('',#86858,#45006,#45007);
#36851=AXIS2_PLACEMENT_3D('',#86860,#45008,#45009);
#36852=AXIS2_PLACEMENT_3D('',#86862,#45010,#45011);
#36853=AXIS2_PLACEMENT_3D('',#86863,#45012,#45013);
#36854=AXIS2_PLACEMENT_3D('',#86864,#45014,#45015);
#36855=AXIS2_PLACEMENT_3D('',#86866,#45016,#45017);
#36856=AXIS2_PLACEMENT_3D('',#86868,#45018,#45019);
#36857=AXIS2_PLACEMENT_3D('',#86869,#45020,#45021);
#36858=AXIS2_PLACEMENT_3D('',#86870,#45022,#45023);
#36859=AXIS2_PLACEMENT_3D('',#86873,#45026,#45027);
#36860=AXIS2_PLACEMENT_3D('',#86876,#45028,#45029);
#36861=AXIS2_PLACEMENT_3D('',#86878,#45030,#45031);
#36862=AXIS2_PLACEMENT_3D('',#86880,#45032,#45033);
#36863=AXIS2_PLACEMENT_3D('',#86881,#45034,#45035);
#36864=AXIS2_PLACEMENT_3D('',#86919,#45036,#45037);
#36865=AXIS2_PLACEMENT_3D('',#86925,#45038,#45039);
#36866=AXIS2_PLACEMENT_3D('',#86926,#45040,#45041);
#36867=AXIS2_PLACEMENT_3D('',#86927,#45042,#45043);
#36868=AXIS2_PLACEMENT_3D('',#86929,#45044,#45045);
#36869=AXIS2_PLACEMENT_3D('',#86930,#45046,#45047);
#36870=AXIS2_PLACEMENT_3D('',#86968,#45048,#45049);
#36871=AXIS2_PLACEMENT_3D('',#86970,#45050,#45051);
#36872=AXIS2_PLACEMENT_3D('',#86971,#45052,#45053);
#36873=AXIS2_PLACEMENT_3D('',#87009,#45054,#45055);
#36874=AXIS2_PLACEMENT_3D('',#87068,#45056,#45057);
#36875=AXIS2_PLACEMENT_3D('',#87069,#45058,#45059);
#36876=AXIS2_PLACEMENT_3D('',#87071,#45060,#45061);
#36877=AXIS2_PLACEMENT_3D('',#87073,#45062,#45063);
#36878=AXIS2_PLACEMENT_3D('',#87074,#45064,#45065);
#36879=AXIS2_PLACEMENT_3D('',#87075,#45066,#45067);
#36880=AXIS2_PLACEMENT_3D('',#87077,#45068,#45069);
#36881=AXIS2_PLACEMENT_3D('',#87079,#45070,#45071);
#36882=AXIS2_PLACEMENT_3D('',#87080,#45072,#45073);
#36883=AXIS2_PLACEMENT_3D('',#87081,#45074,#45075);
#36884=AXIS2_PLACEMENT_3D('',#87083,#45076,#45077);
#36885=AXIS2_PLACEMENT_3D('',#87085,#45078,#45079);
#36886=AXIS2_PLACEMENT_3D('',#87086,#45080,#45081);
#36887=AXIS2_PLACEMENT_3D('',#87087,#45082,#45083);
#36888=AXIS2_PLACEMENT_3D('',#87127,#45086,#45087);
#36889=AXIS2_PLACEMENT_3D('',#87129,#45088,#45089);
#36890=AXIS2_PLACEMENT_3D('',#87130,#45090,#45091);
#36891=AXIS2_PLACEMENT_3D('',#87168,#45092,#45093);
#36892=AXIS2_PLACEMENT_3D('',#87234,#45094,#45095);
#36893=AXIS2_PLACEMENT_3D('',#87235,#45096,#45097);
#36894=AXIS2_PLACEMENT_3D('',#87236,#45098,#45099);
#36895=AXIS2_PLACEMENT_3D('',#87238,#45100,#45101);
#36896=AXIS2_PLACEMENT_3D('',#87240,#45102,#45103);
#36897=AXIS2_PLACEMENT_3D('',#87242,#45104,#45105);
#36898=AXIS2_PLACEMENT_3D('',#87244,#45106,#45107);
#36899=AXIS2_PLACEMENT_3D('',#87245,#45108,#45109);
#36900=AXIS2_PLACEMENT_3D('',#87246,#45110,#45111);
#36901=AXIS2_PLACEMENT_3D('',#87248,#45112,#45113);
#36902=AXIS2_PLACEMENT_3D('',#87250,#45114,#45115);
#36903=AXIS2_PLACEMENT_3D('',#87251,#45116,#45117);
#36904=AXIS2_PLACEMENT_3D('',#87252,#45118,#45119);
#36905=AXIS2_PLACEMENT_3D('',#87257,#45122,#45123);
#36906=AXIS2_PLACEMENT_3D('',#87258,#45124,#45125);
#36907=AXIS2_PLACEMENT_3D('',#87260,#45126,#45127);
#36908=AXIS2_PLACEMENT_3D('',#87262,#45128,#45129);
#36909=AXIS2_PLACEMENT_3D('',#87263,#45130,#45131);
#36910=AXIS2_PLACEMENT_3D('',#87264,#45132,#45133);
#36911=AXIS2_PLACEMENT_3D('',#87266,#45134,#45135);
#36912=AXIS2_PLACEMENT_3D('',#87268,#45136,#45137);
#36913=AXIS2_PLACEMENT_3D('',#87269,#45138,#45139);
#36914=AXIS2_PLACEMENT_3D('',#87270,#45140,#45141);
#36915=AXIS2_PLACEMENT_3D('',#87272,#45142,#45143);
#36916=AXIS2_PLACEMENT_3D('',#87274,#45144,#45145);
#36917=AXIS2_PLACEMENT_3D('',#87275,#45146,#45147);
#36918=AXIS2_PLACEMENT_3D('',#87276,#45148,#45149);
#36919=AXIS2_PLACEMENT_3D('',#87278,#45150,#45151);
#36920=AXIS2_PLACEMENT_3D('',#87280,#45152,#45153);
#36921=AXIS2_PLACEMENT_3D('',#87281,#45154,#45155);
#36922=AXIS2_PLACEMENT_3D('',#87282,#45156,#45157);
#36923=AXIS2_PLACEMENT_3D('',#87285,#45160,#45161);
#36924=AXIS2_PLACEMENT_3D('',#87290,#45163,#45164);
#36925=AXIS2_PLACEMENT_3D('',#87372,#45166,#45167);
#36926=AXIS2_PLACEMENT_3D('',#87438,#45170,#45171);
#36927=AXIS2_PLACEMENT_3D('',#87441,#45172,#45173);
#36928=AXIS2_PLACEMENT_3D('',#87544,#45174,#45175);
#36929=AXIS2_PLACEMENT_3D('',#87545,#45176,#45177);
#36930=AXIS2_PLACEMENT_3D('',#87546,#45178,#45179);
#36931=AXIS2_PLACEMENT_3D('',#87548,#45180,#45181);
#36932=AXIS2_PLACEMENT_3D('',#87549,#45182,#45183);
#36933=AXIS2_PLACEMENT_3D('',#87550,#45184,#45185);
#36934=AXIS2_PLACEMENT_3D('',#87552,#45186,#45187);
#36935=AXIS2_PLACEMENT_3D('',#87554,#45188,#45189);
#36936=AXIS2_PLACEMENT_3D('',#87628,#45190,#45191);
#36937=AXIS2_PLACEMENT_3D('',#87630,#45192,#45193);
#36938=AXIS2_PLACEMENT_3D('',#87631,#45194,#45195);
#36939=AXIS2_PLACEMENT_3D('',#87632,#45196,#45197);
#36940=AXIS2_PLACEMENT_3D('',#87634,#45198,#45199);
#36941=AXIS2_PLACEMENT_3D('',#87635,#45200,#45201);
#36942=AXIS2_PLACEMENT_3D('',#87636,#45202,#45203);
#36943=AXIS2_PLACEMENT_3D('',#87638,#45204,#45205);
#36944=AXIS2_PLACEMENT_3D('',#87639,#45206,#45207);
#36945=AXIS2_PLACEMENT_3D('',#87640,#45208,#45209);
#36946=AXIS2_PLACEMENT_3D('',#87643,#45212,#45213);
#36947=AXIS2_PLACEMENT_3D('',#87645,#45214,#45215);
#36948=AXIS2_PLACEMENT_3D('',#87647,#45216,#45217);
#36949=AXIS2_PLACEMENT_3D('',#87648,#45218,#45219);
#36950=AXIS2_PLACEMENT_3D('',#87649,#45220,#45221);
#36951=AXIS2_PLACEMENT_3D('',#87651,#45222,#45223);
#36952=AXIS2_PLACEMENT_3D('',#87653,#45224,#45225);
#36953=AXIS2_PLACEMENT_3D('',#87654,#45226,#45227);
#36954=AXIS2_PLACEMENT_3D('',#87655,#45228,#45229);
#36955=AXIS2_PLACEMENT_3D('',#87657,#45230,#45231);
#36956=AXIS2_PLACEMENT_3D('',#87659,#45232,#45233);
#36957=AXIS2_PLACEMENT_3D('',#87660,#45234,#45235);
#36958=AXIS2_PLACEMENT_3D('',#87661,#45236,#45237);
#36959=AXIS2_PLACEMENT_3D('',#87663,#45238,#45239);
#36960=AXIS2_PLACEMENT_3D('',#87665,#45240,#45241);
#36961=AXIS2_PLACEMENT_3D('',#87666,#45242,#45243);
#36962=AXIS2_PLACEMENT_3D('',#87667,#45244,#45245);
#36963=AXIS2_PLACEMENT_3D('',#87669,#45246,#45247);
#36964=AXIS2_PLACEMENT_3D('',#87671,#45248,#45249);
#36965=AXIS2_PLACEMENT_3D('',#87672,#45250,#45251);
#36966=AXIS2_PLACEMENT_3D('',#87673,#45252,#45253);
#36967=AXIS2_PLACEMENT_3D('',#87675,#45254,#45255);
#36968=AXIS2_PLACEMENT_3D('',#87676,#45256,#45257);
#36969=AXIS2_PLACEMENT_3D('',#87677,#45258,#45259);
#36970=AXIS2_PLACEMENT_3D('',#87680,#45260,#45261);
#36971=AXIS2_PLACEMENT_3D('',#87683,#45264,#45265);
#36972=AXIS2_PLACEMENT_3D('',#87684,#45266,#45267);
#36973=AXIS2_PLACEMENT_3D('',#87685,#45268,#45269);
#36974=AXIS2_PLACEMENT_3D('',#87688,#45270,#45271);
#36975=AXIS2_PLACEMENT_3D('',#87725,#45272,#45273);
#36976=AXIS2_PLACEMENT_3D('',#87730,#45275,#45276);
#36977=AXIS2_PLACEMENT_3D('',#87733,#45278,#45279);
#36978=AXIS2_PLACEMENT_3D('',#87734,#45280,#45281);
#36979=AXIS2_PLACEMENT_3D('',#87736,#45282,#45283);
#36980=AXIS2_PLACEMENT_3D('',#87796,#45284,#45285);
#36981=AXIS2_PLACEMENT_3D('',#87797,#45286,#45287);
#36982=AXIS2_PLACEMENT_3D('',#87800,#45288,#45289);
#36983=AXIS2_PLACEMENT_3D('',#87801,#45290,#45291);
#36984=AXIS2_PLACEMENT_3D('',#87802,#45292,#45293);
#36985=AXIS2_PLACEMENT_3D('',#87805,#45294,#45295);
#36986=AXIS2_PLACEMENT_3D('',#87806,#45296,#45297);
#36987=AXIS2_PLACEMENT_3D('',#87807,#45298,#45299);
#36988=AXIS2_PLACEMENT_3D('',#87808,#45300,#45301);
#36989=AXIS2_PLACEMENT_3D('',#87811,#45302,#45303);
#36990=AXIS2_PLACEMENT_3D('',#87813,#45304,#45305);
#36991=AXIS2_PLACEMENT_3D('',#87815,#45306,#45307);
#36992=AXIS2_PLACEMENT_3D('',#87816,#45308,#45309);
#36993=AXIS2_PLACEMENT_3D('',#87817,#45310,#45311);
#36994=AXIS2_PLACEMENT_3D('',#87911,#45312,#45313);
#36995=AXIS2_PLACEMENT_3D('',#87912,#45314,#45315);
#36996=AXIS2_PLACEMENT_3D('',#87913,#45316,#45317);
#36997=AXIS2_PLACEMENT_3D('',#87974,#45318,#45319);
#36998=AXIS2_PLACEMENT_3D('',#87975,#45320,#45321);
#36999=AXIS2_PLACEMENT_3D('',#87976,#45322,#45323);
#37000=AXIS2_PLACEMENT_3D('',#87977,#45324,#45325);
#37001=AXIS2_PLACEMENT_3D('',#87979,#45326,#45327);
#37002=AXIS2_PLACEMENT_3D('',#87982,#45329,#45330);
#37003=AXIS2_PLACEMENT_3D('',#87983,#45331,#45332);
#37004=AXIS2_PLACEMENT_3D('',#87984,#45333,#45334);
#37005=AXIS2_PLACEMENT_3D('',#87985,#45335,#45336);
#37006=AXIS2_PLACEMENT_3D('',#87986,#45337,#45338);
#37007=AXIS2_PLACEMENT_3D('',#87987,#45339,#45340);
#37008=AXIS2_PLACEMENT_3D('',#87988,#45341,#45342);
#37009=AXIS2_PLACEMENT_3D('',#87989,#45343,#45344);
#37010=AXIS2_PLACEMENT_3D('',#87990,#45345,#45346);
#37011=AXIS2_PLACEMENT_3D('',#88124,#45348,#45349);
#37012=AXIS2_PLACEMENT_3D('',#88125,#45350,#45351);
#37013=AXIS2_PLACEMENT_3D('',#88126,#45352,#45353);
#37014=AXIS2_PLACEMENT_3D('',#88127,#45354,#45355);
#37015=AXIS2_PLACEMENT_3D('',#88223,#45356,#45357);
#37016=AXIS2_PLACEMENT_3D('',#88224,#45358,#45359);
#37017=AXIS2_PLACEMENT_3D('',#88225,#45360,#45361);
#37018=AXIS2_PLACEMENT_3D('',#88226,#45362,#45363);
#37019=AXIS2_PLACEMENT_3D('',#88228,#45365,#45366);
#37020=AXIS2_PLACEMENT_3D('',#88230,#45368,#45369);
#37021=AXIS2_PLACEMENT_3D('',#88231,#45370,#45371);
#37022=AXIS2_PLACEMENT_3D('',#88233,#45372,#45373);
#37023=AXIS2_PLACEMENT_3D('',#88234,#45374,#45375);
#37024=AXIS2_PLACEMENT_3D('',#88236,#45376,#45377);
#37025=AXIS2_PLACEMENT_3D('',#88237,#45378,#45379);
#37026=AXIS2_PLACEMENT_3D('',#88240,#45381,#45382);
#37027=AXIS2_PLACEMENT_3D('',#88242,#45384,#45385);
#37028=AXIS2_PLACEMENT_3D('',#88246,#45387,#45388);
#37029=AXIS2_PLACEMENT_3D('',#88248,#45390,#45391);
#37030=AXIS2_PLACEMENT_3D('',#88315,#45393,#45394);
#37031=AXIS2_PLACEMENT_3D('',#88356,#45395,#45396);
#37032=AXIS2_PLACEMENT_3D('',#88358,#45397,#45398);
#37033=AXIS2_PLACEMENT_3D('',#88360,#45399,#45400);
#37034=AXIS2_PLACEMENT_3D('',#88388,#45403,#45404);
#37035=AXIS2_PLACEMENT_3D('',#88390,#45405,#45406);
#37036=AXIS2_PLACEMENT_3D('',#88392,#45407,#45408);
#37037=AXIS2_PLACEMENT_3D('',#88394,#45410,#45411);
#37038=AXIS2_PLACEMENT_3D('',#88395,#45412,#45413);
#37039=AXIS2_PLACEMENT_3D('',#88396,#45414,#45415);
#37040=AXIS2_PLACEMENT_3D('',#88398,#45416,#45417);
#37041=AXIS2_PLACEMENT_3D('',#88399,#45418,#45419);
#37042=AXIS2_PLACEMENT_3D('',#88428,#45420,#45421);
#37043=AXIS2_PLACEMENT_3D('',#88429,#45422,#45423);
#37044=AXIS2_PLACEMENT_3D('',#88431,#45424,#45425);
#37045=AXIS2_PLACEMENT_3D('',#88432,#45426,#45427);
#37046=AXIS2_PLACEMENT_3D('',#88433,#45428,#45429);
#37047=AXIS2_PLACEMENT_3D('',#88436,#45431,#45432);
#37048=AXIS2_PLACEMENT_3D('',#88437,#45433,#45434);
#37049=AXIS2_PLACEMENT_3D('',#88438,#45435,#45436);
#37050=AXIS2_PLACEMENT_3D('',#88439,#45437,#45438);
#37051=AXIS2_PLACEMENT_3D('',#88441,#45439,#45440);
#37052=AXIS2_PLACEMENT_3D('',#88442,#45441,#45442);
#37053=AXIS2_PLACEMENT_3D('',#88443,#45443,#45444);
#37054=AXIS2_PLACEMENT_3D('',#88444,#45445,#45446);
#37055=AXIS2_PLACEMENT_3D('',#88445,#45447,#45448);
#37056=AXIS2_PLACEMENT_3D('',#88446,#45449,#45450);
#37057=AXIS2_PLACEMENT_3D('',#88447,#45451,#45452);
#37058=AXIS2_PLACEMENT_3D('',#88448,#45453,#45454);
#37059=AXIS2_PLACEMENT_3D('',#88449,#45455,#45456);
#37060=AXIS2_PLACEMENT_3D('',#88455,#45460,#45461);
#37061=AXIS2_PLACEMENT_3D('',#88458,#45464,#45465);
#37062=AXIS2_PLACEMENT_3D('',#88460,#45466,#45467);
#37063=AXIS2_PLACEMENT_3D('',#88462,#45469,#45470);
#37064=AXIS2_PLACEMENT_3D('',#88466,#45473,#45474);
#37065=AXIS2_PLACEMENT_3D('',#88468,#45475,#45476);
#37066=AXIS2_PLACEMENT_3D('',#88470,#45478,#45479);
#37067=AXIS2_PLACEMENT_3D('',#88471,#45480,#45481);
#37068=AXIS2_PLACEMENT_3D('',#88473,#45483,#45484);
#37069=AXIS2_PLACEMENT_3D('',#88475,#45486,#45487);
#37070=AXIS2_PLACEMENT_3D('',#88477,#45489,#45490);
#37071=AXIS2_PLACEMENT_3D('',#88478,#45491,#45492);
#37072=AXIS2_PLACEMENT_3D('',#88481,#45495,#45496);
#37073=AXIS2_PLACEMENT_3D('',#88483,#45498,#45499);
#37074=AXIS2_PLACEMENT_3D('',#88485,#45501,#45502);
#37075=AXIS2_PLACEMENT_3D('',#88487,#45504,#45505);
#37076=AXIS2_PLACEMENT_3D('',#88489,#45507,#45508);
#37077=AXIS2_PLACEMENT_3D('',#88490,#45509,#45510);
#37078=AXIS2_PLACEMENT_3D('',#88493,#45513,#45514);
#37079=AXIS2_PLACEMENT_3D('',#88495,#45516,#45517);
#37080=AXIS2_PLACEMENT_3D('',#88497,#45519,#45520);
#37081=AXIS2_PLACEMENT_3D('',#88499,#45521,#45522);
#37082=AXIS2_PLACEMENT_3D('',#88501,#45524,#45525);
#37083=AXIS2_PLACEMENT_3D('',#88503,#45526,#45527);
#37084=AXIS2_PLACEMENT_3D('',#88505,#45529,#45530);
#37085=AXIS2_PLACEMENT_3D('',#88508,#45532,#45533);
#37086=AXIS2_PLACEMENT_3D('',#88509,#45534,#45535);
#37087=AXIS2_PLACEMENT_3D('',#88511,#45536,#45537);
#37088=AXIS2_PLACEMENT_3D('',#88513,#45539,#45540);
#37089=AXIS2_PLACEMENT_3D('',#88515,#45542,#45543);
#37090=AXIS2_PLACEMENT_3D('',#88516,#45544,#45545);
#37091=AXIS2_PLACEMENT_3D('',#88517,#45546,#45547);
#37092=AXIS2_PLACEMENT_3D('',#88519,#45548,#45549);
#37093=AXIS2_PLACEMENT_3D('',#88578,#45550,#45551);
#37094=AXIS2_PLACEMENT_3D('',#88579,#45552,#45553);
#37095=AXIS2_PLACEMENT_3D('',#88580,#45554,#45555);
#37096=AXIS2_PLACEMENT_3D('',#88581,#45556,#45557);
#37097=AXIS2_PLACEMENT_3D('',#88582,#45558,#45559);
#37098=AXIS2_PLACEMENT_3D('',#88584,#45561,#45562);
#37099=AXIS2_PLACEMENT_3D('',#88587,#45564,#45565);
#37100=AXIS2_PLACEMENT_3D('',#88588,#45566,#45567);
#37101=AXIS2_PLACEMENT_3D('',#88589,#45568,#45569);
#37102=AXIS2_PLACEMENT_3D('',#88591,#45570,#45571);
#37103=AXIS2_PLACEMENT_3D('',#88593,#45572,#45573);
#37104=AXIS2_PLACEMENT_3D('',#88594,#45574,#45575);
#37105=AXIS2_PLACEMENT_3D('',#88595,#45576,#45577);
#37106=AXIS2_PLACEMENT_3D('',#88596,#45578,#45579);
#37107=AXIS2_PLACEMENT_3D('',#88597,#45580,#45581);
#37108=AXIS2_PLACEMENT_3D('',#88599,#45583,#45584);
#37109=AXIS2_PLACEMENT_3D('',#88600,#45585,#45586);
#37110=AXIS2_PLACEMENT_3D('',#88601,#45587,#45588);
#37111=AXIS2_PLACEMENT_3D('',#88602,#45589,#45590);
#37112=AXIS2_PLACEMENT_3D('',#88603,#45591,#45592);
#37113=AXIS2_PLACEMENT_3D('',#88683,#45593,#45594);
#37114=AXIS2_PLACEMENT_3D('',#88684,#45595,#45596);
#37115=AXIS2_PLACEMENT_3D('',#88770,#45597,#45598);
#37116=AXIS2_PLACEMENT_3D('',#88823,#45599,#45600);
#37117=AXIS2_PLACEMENT_3D('',#88825,#45602,#45603);
#37118=AXIS2_PLACEMENT_3D('',#88826,#45604,#45605);
#37119=AXIS2_PLACEMENT_3D('',#88827,#45606,#45607);
#37120=AXIS2_PLACEMENT_3D('',#88829,#45608,#45609);
#37121=AXIS2_PLACEMENT_3D('',#88830,#45610,#45611);
#37122=AXIS2_PLACEMENT_3D('',#88831,#45612,#45613);
#37123=AXIS2_PLACEMENT_3D('',#88834,#45614,#45615);
#37124=AXIS2_PLACEMENT_3D('',#88836,#45616,#45617);
#37125=AXIS2_PLACEMENT_3D('',#88837,#45618,#45619);
#37126=AXIS2_PLACEMENT_3D('',#88838,#45620,#45621);
#37127=AXIS2_PLACEMENT_3D('',#88841,#45624,#45625);
#37128=AXIS2_PLACEMENT_3D('',#88842,#45626,#45627);
#37129=AXIS2_PLACEMENT_3D('',#88843,#45628,#45629);
#37130=AXIS2_PLACEMENT_3D('',#88844,#45630,#45631);
#37131=AXIS2_PLACEMENT_3D('',#88845,#45632,#45633);
#37132=AXIS2_PLACEMENT_3D('',#88847,#45634,#45635);
#37133=AXIS2_PLACEMENT_3D('',#88849,#45636,#45637);
#37134=AXIS2_PLACEMENT_3D('',#88851,#45639,#45640);
#37135=AXIS2_PLACEMENT_3D('',#88853,#45641,#45642);
#37136=AXIS2_PLACEMENT_3D('',#88854,#45643,#45644);
#37137=AXIS2_PLACEMENT_3D('',#88855,#45645,#45646);
#37138=AXIS2_PLACEMENT_3D('',#88857,#45647,#45648);
#37139=AXIS2_PLACEMENT_3D('',#88858,#45649,#45650);
#37140=AXIS2_PLACEMENT_3D('',#88859,#45651,#45652);
#37141=AXIS2_PLACEMENT_3D('',#88861,#45653,#45654);
#37142=AXIS2_PLACEMENT_3D('',#88862,#45655,#45656);
#37143=AXIS2_PLACEMENT_3D('',#88863,#45657,#45658);
#37144=AXIS2_PLACEMENT_3D('',#88865,#45659,#45660);
#37145=AXIS2_PLACEMENT_3D('',#88867,#45662,#45663);
#37146=AXIS2_PLACEMENT_3D('',#88869,#45664,#45665);
#37147=AXIS2_PLACEMENT_3D('',#88870,#45666,#45667);
#37148=AXIS2_PLACEMENT_3D('',#88872,#45668,#45669);
#37149=AXIS2_PLACEMENT_3D('',#88873,#45670,#45671);
#37150=AXIS2_PLACEMENT_3D('',#88875,#45672,#45673);
#37151=AXIS2_PLACEMENT_3D('',#88953,#45674,#45675);
#37152=AXIS2_PLACEMENT_3D('',#88954,#45676,#45677);
#37153=AXIS2_PLACEMENT_3D('',#88955,#45678,#45679);
#37154=AXIS2_PLACEMENT_3D('',#88956,#45680,#45681);
#37155=AXIS2_PLACEMENT_3D('',#88958,#45682,#45683);
#37156=AXIS2_PLACEMENT_3D('',#88960,#45684,#45685);
#37157=AXIS2_PLACEMENT_3D('',#88966,#45686,#45687);
#37158=AXIS2_PLACEMENT_3D('',#88968,#45689,#45690);
#37159=AXIS2_PLACEMENT_3D('',#88970,#45692,#45693);
#37160=AXIS2_PLACEMENT_3D('',#88972,#45695,#45696);
#37161=AXIS2_PLACEMENT_3D('',#88975,#45698,#45699);
#37162=AXIS2_PLACEMENT_3D('',#88976,#45700,#45701);
#37163=AXIS2_PLACEMENT_3D('',#88977,#45702,#45703);
#37164=AXIS2_PLACEMENT_3D('',#88978,#45704,#45705);
#37165=AXIS2_PLACEMENT_3D('',#88981,#45708,#45709);
#37166=AXIS2_PLACEMENT_3D('',#88983,#45711,#45712);
#37167=AXIS2_PLACEMENT_3D('',#89094,#45714,#45715);
#37168=AXIS2_PLACEMENT_3D('',#89159,#45716,#45717);
#37169=AXIS2_PLACEMENT_3D('',#89161,#45718,#45719);
#37170=AXIS2_PLACEMENT_3D('',#89163,#45721,#45722);
#37171=AXIS2_PLACEMENT_3D('',#89165,#45723,#45724);
#37172=AXIS2_PLACEMENT_3D('',#89166,#45725,#45726);
#37173=AXIS2_PLACEMENT_3D('',#89167,#45727,#45728);
#37174=AXIS2_PLACEMENT_3D('',#89169,#45729,#45730);
#37175=AXIS2_PLACEMENT_3D('',#89170,#45731,#45732);
#37176=AXIS2_PLACEMENT_3D('',#89171,#45733,#45734);
#37177=AXIS2_PLACEMENT_3D('',#89173,#45735,#45736);
#37178=AXIS2_PLACEMENT_3D('',#89174,#45737,#45738);
#37179=AXIS2_PLACEMENT_3D('',#89175,#45739,#45740);
#37180=AXIS2_PLACEMENT_3D('',#89177,#45741,#45742);
#37181=AXIS2_PLACEMENT_3D('',#89234,#45744,#45745);
#37182=AXIS2_PLACEMENT_3D('',#89314,#45746,#45747);
#37183=AXIS2_PLACEMENT_3D('',#89316,#45748,#45749);
#37184=AXIS2_PLACEMENT_3D('',#89317,#45750,#45751);
#37185=AXIS2_PLACEMENT_3D('',#89318,#45752,#45753);
#37186=AXIS2_PLACEMENT_3D('',#89320,#45754,#45755);
#37187=AXIS2_PLACEMENT_3D('',#89321,#45756,#45757);
#37188=AXIS2_PLACEMENT_3D('',#89322,#45758,#45759);
#37189=AXIS2_PLACEMENT_3D('',#89323,#45760,#45761);
#37190=AXIS2_PLACEMENT_3D('',#89324,#45762,#45763);
#37191=AXIS2_PLACEMENT_3D('',#89326,#45764,#45765);
#37192=AXIS2_PLACEMENT_3D('',#89327,#45766,#45767);
#37193=AXIS2_PLACEMENT_3D('',#89328,#45768,#45769);
#37194=AXIS2_PLACEMENT_3D('',#89330,#45770,#45771);
#37195=AXIS2_PLACEMENT_3D('',#89331,#45772,#45773);
#37196=AXIS2_PLACEMENT_3D('',#89370,#45774,#45775);
#37197=AXIS2_PLACEMENT_3D('',#89371,#45776,#45777);
#37198=AXIS2_PLACEMENT_3D('',#89372,#45778,#45779);
#37199=AXIS2_PLACEMENT_3D('',#89436,#45780,#45781);
#37200=AXIS2_PLACEMENT_3D('',#89438,#45782,#45783);
#37201=AXIS2_PLACEMENT_3D('',#89504,#45785,#45786);
#37202=AXIS2_PLACEMENT_3D('',#89505,#45787,#45788);
#37203=AXIS2_PLACEMENT_3D('',#89622,#45790,#45791);
#37204=AXIS2_PLACEMENT_3D('',#89623,#45792,#45793);
#37205=AXIS2_PLACEMENT_3D('',#89625,#45795,#45796);
#37206=AXIS2_PLACEMENT_3D('',#89626,#45797,#45798);
#37207=AXIS2_PLACEMENT_3D('',#89627,#45799,#45800);
#37208=AXIS2_PLACEMENT_3D('',#89650,#45801,#45802);
#37209=AXIS2_PLACEMENT_3D('',#89706,#45803,#45804);
#37210=AXIS2_PLACEMENT_3D('',#89784,#45805,#45806);
#37211=AXIS2_PLACEMENT_3D('',#89785,#45807,#45808);
#37212=AXIS2_PLACEMENT_3D('',#89787,#45809,#45810);
#37213=AXIS2_PLACEMENT_3D('',#89789,#45811,#45812);
#37214=AXIS2_PLACEMENT_3D('',#89790,#45813,#45814);
#37215=AXIS2_PLACEMENT_3D('',#89791,#45815,#45816);
#37216=AXIS2_PLACEMENT_3D('',#89793,#45817,#45818);
#37217=AXIS2_PLACEMENT_3D('',#89795,#45819,#45820);
#37218=AXIS2_PLACEMENT_3D('',#89796,#45821,#45822);
#37219=AXIS2_PLACEMENT_3D('',#89797,#45823,#45824);
#37220=AXIS2_PLACEMENT_3D('',#89801,#45826,#45827);
#37221=AXIS2_PLACEMENT_3D('',#89803,#45829,#45830);
#37222=AXIS2_PLACEMENT_3D('',#89805,#45831,#45832);
#37223=AXIS2_PLACEMENT_3D('',#89807,#45833,#45834);
#37224=AXIS2_PLACEMENT_3D('',#89808,#45835,#45836);
#37225=AXIS2_PLACEMENT_3D('',#89809,#45837,#45838);
#37226=AXIS2_PLACEMENT_3D('',#89811,#45839,#45840);
#37227=AXIS2_PLACEMENT_3D('',#89813,#45841,#45842);
#37228=AXIS2_PLACEMENT_3D('',#89814,#45843,#45844);
#37229=AXIS2_PLACEMENT_3D('',#89815,#45845,#45846);
#37230=AXIS2_PLACEMENT_3D('',#89817,#45847,#45848);
#37231=AXIS2_PLACEMENT_3D('',#89819,#45849,#45850);
#37232=AXIS2_PLACEMENT_3D('',#89820,#45851,#45852);
#37233=AXIS2_PLACEMENT_3D('',#89858,#45853,#45854);
#37234=AXIS2_PLACEMENT_3D('',#89859,#45855,#45856);
#37235=AXIS2_PLACEMENT_3D('',#89960,#45857,#45858);
#37236=AXIS2_PLACEMENT_3D('',#89963,#45861,#45862);
#37237=AXIS2_PLACEMENT_3D('',#89967,#45864,#45865);
#37238=AXIS2_PLACEMENT_3D('',#89969,#45867,#45868);
#37239=AXIS2_PLACEMENT_3D('',#89971,#45869,#45870);
#37240=AXIS2_PLACEMENT_3D('',#89973,#45872,#45873);
#37241=AXIS2_PLACEMENT_3D('',#89974,#45874,#45875);
#37242=AXIS2_PLACEMENT_3D('',#89975,#45876,#45877);
#37243=AXIS2_PLACEMENT_3D('',#89977,#45878,#45879);
#37244=AXIS2_PLACEMENT_3D('',#89979,#45881,#45882);
#37245=AXIS2_PLACEMENT_3D('',#89981,#45883,#45884);
#37246=AXIS2_PLACEMENT_3D('',#89983,#45886,#45887);
#37247=AXIS2_PLACEMENT_3D('',#89985,#45888,#45889);
#37248=AXIS2_PLACEMENT_3D('',#89987,#45891,#45892);
#37249=AXIS2_PLACEMENT_3D('',#89991,#45895,#45896);
#37250=AXIS2_PLACEMENT_3D('',#89993,#45897,#45898);
#37251=AXIS2_PLACEMENT_3D('',#89995,#45900,#45901);
#37252=AXIS2_PLACEMENT_3D('',#89997,#45902,#45903);
#37253=AXIS2_PLACEMENT_3D('',#89999,#45905,#45906);
#37254=AXIS2_PLACEMENT_3D('',#90001,#45907,#45908);
#37255=AXIS2_PLACEMENT_3D('',#90003,#45910,#45911);
#37256=AXIS2_PLACEMENT_3D('',#90007,#45914,#45915);
#37257=AXIS2_PLACEMENT_3D('',#90008,#45916,#45917);
#37258=AXIS2_PLACEMENT_3D('',#90009,#45918,#45919);
#37259=AXIS2_PLACEMENT_3D('',#90011,#45920,#45921);
#37260=AXIS2_PLACEMENT_3D('',#90012,#45922,#45923);
#37261=AXIS2_PLACEMENT_3D('',#90013,#45924,#45925);
#37262=AXIS2_PLACEMENT_3D('',#90015,#45926,#45927);
#37263=AXIS2_PLACEMENT_3D('',#90016,#45928,#45929);
#37264=AXIS2_PLACEMENT_3D('',#90017,#45930,#45931);
#37265=AXIS2_PLACEMENT_3D('',#90019,#45932,#45933);
#37266=AXIS2_PLACEMENT_3D('',#90020,#45934,#45935);
#37267=AXIS2_PLACEMENT_3D('',#90021,#45936,#45937);
#37268=AXIS2_PLACEMENT_3D('',#90023,#45938,#45939);
#37269=AXIS2_PLACEMENT_3D('',#90024,#45940,#45941);
#37270=AXIS2_PLACEMENT_3D('',#90025,#45942,#45943);
#37271=AXIS2_PLACEMENT_3D('',#90026,#45944,#45945);
#37272=AXIS2_PLACEMENT_3D('',#90027,#45946,#45947);
#37273=AXIS2_PLACEMENT_3D('',#90029,#45948,#45949);
#37274=AXIS2_PLACEMENT_3D('',#90030,#45950,#45951);
#37275=AXIS2_PLACEMENT_3D('',#90031,#45952,#45953);
#37276=AXIS2_PLACEMENT_3D('',#90033,#45954,#45955);
#37277=AXIS2_PLACEMENT_3D('',#90089,#45956,#45957);
#37278=AXIS2_PLACEMENT_3D('',#90090,#45958,#45959);
#37279=AXIS2_PLACEMENT_3D('',#90091,#45960,#45961);
#37280=AXIS2_PLACEMENT_3D('',#90149,#45963,#45964);
#37281=AXIS2_PLACEMENT_3D('',#90150,#45965,#45966);
#37282=AXIS2_PLACEMENT_3D('',#90151,#45967,#45968);
#37283=AXIS2_PLACEMENT_3D('',#90153,#45969,#45970);
#37284=AXIS2_PLACEMENT_3D('',#90209,#45971,#45972);
#37285=AXIS2_PLACEMENT_3D('',#90210,#45973,#45974);
#37286=AXIS2_PLACEMENT_3D('',#90211,#45975,#45976);
#37287=AXIS2_PLACEMENT_3D('',#90213,#45978,#45979);
#37288=AXIS2_PLACEMENT_3D('',#90216,#45981,#45982);
#37289=AXIS2_PLACEMENT_3D('',#90217,#45983,#45984);
#37290=AXIS2_PLACEMENT_3D('',#90219,#45985,#45986);
#37291=AXIS2_PLACEMENT_3D('',#90220,#45987,#45988);
#37292=AXIS2_PLACEMENT_3D('',#90221,#45989,#45990);
#37293=AXIS2_PLACEMENT_3D('',#90223,#45991,#45992);
#37294=AXIS2_PLACEMENT_3D('',#90224,#45993,#45994);
#37295=AXIS2_PLACEMENT_3D('',#90225,#45995,#45996);
#37296=AXIS2_PLACEMENT_3D('',#90226,#45997,#45998);
#37297=AXIS2_PLACEMENT_3D('',#90227,#45999,#46000);
#37298=AXIS2_PLACEMENT_3D('',#90228,#46001,#46002);
#37299=AXIS2_PLACEMENT_3D('',#90233,#46004,#46005);
#37300=AXIS2_PLACEMENT_3D('',#90237,#46007,#46008);
#37301=AXIS2_PLACEMENT_3D('',#90302,#46009,#46010);
#37302=AXIS2_PLACEMENT_3D('',#90305,#46011,#46012);
#37303=AXIS2_PLACEMENT_3D('',#90306,#46013,#46014);
#37304=AXIS2_PLACEMENT_3D('',#90308,#46015,#46016);
#37305=AXIS2_PLACEMENT_3D('',#90310,#46018,#46019);
#37306=AXIS2_PLACEMENT_3D('',#90312,#46020,#46021);
#37307=AXIS2_PLACEMENT_3D('',#90388,#46023,#46024);
#37308=AXIS2_PLACEMENT_3D('',#90409,#46026,#46027);
#37309=AXIS2_PLACEMENT_3D('',#90411,#46029,#46030);
#37310=AXIS2_PLACEMENT_3D('',#90451,#46032,#46033);
#37311=AXIS2_PLACEMENT_3D('',#90453,#46035,#46036);
#37312=AXIS2_PLACEMENT_3D('',#90459,#46040,#46041);
#37313=AXIS2_PLACEMENT_3D('',#90461,#46042,#46043);
#37314=AXIS2_PLACEMENT_3D('',#90464,#46045,#46046);
#37315=AXIS2_PLACEMENT_3D('',#90465,#46047,#46048);
#37316=AXIS2_PLACEMENT_3D('',#90467,#46049,#46050);
#37317=AXIS2_PLACEMENT_3D('',#90469,#46051,#46052);
#37318=AXIS2_PLACEMENT_3D('',#90471,#46054,#46055);
#37319=AXIS2_PLACEMENT_3D('',#90473,#46056,#46057);
#37320=AXIS2_PLACEMENT_3D('',#90488,#46060,#46061);
#37321=AXIS2_PLACEMENT_3D('',#90489,#46062,#46063);
#37322=AXIS2_PLACEMENT_3D('',#90493,#46065,#46066);
#37323=AXIS2_PLACEMENT_3D('',#90497,#46069,#46070);
#37324=AXIS2_PLACEMENT_3D('',#90501,#46072,#46073);
#37325=AXIS2_PLACEMENT_3D('',#90504,#46075,#46076);
#37326=AXIS2_PLACEMENT_3D('',#90505,#46077,#46078);
#37327=AXIS2_PLACEMENT_3D('',#90506,#46079,#46080);
#37328=AXIS2_PLACEMENT_3D('',#90507,#46081,#46082);
#37329=AXIS2_PLACEMENT_3D('',#90509,#46083,#46084);
#37330=AXIS2_PLACEMENT_3D('',#90510,#46085,#46086);
#37331=AXIS2_PLACEMENT_3D('',#90511,#46087,#46088);
#37332=AXIS2_PLACEMENT_3D('',#90512,#46089,#46090);
#37333=AXIS2_PLACEMENT_3D('',#90513,#46091,#46092);
#37334=AXIS2_PLACEMENT_3D('',#90516,#46093,#46094);
#37335=AXIS2_PLACEMENT_3D('',#90519,#46097,#46098);
#37336=AXIS2_PLACEMENT_3D('',#90522,#46099,#46100);
#37337=AXIS2_PLACEMENT_3D('',#90523,#46101,#46102);
#37338=AXIS2_PLACEMENT_3D('',#90524,#46103,#46104);
#37339=AXIS2_PLACEMENT_3D('',#90525,#46105,#46106);
#37340=AXIS2_PLACEMENT_3D('',#90527,#46107,#46108);
#37341=AXIS2_PLACEMENT_3D('',#90528,#46109,#46110);
#37342=AXIS2_PLACEMENT_3D('',#90529,#46111,#46112);
#37343=AXIS2_PLACEMENT_3D('',#90530,#46113,#46114);
#37344=AXIS2_PLACEMENT_3D('',#90532,#46115,#46116);
#37345=AXIS2_PLACEMENT_3D('',#90533,#46117,#46118);
#37346=AXIS2_PLACEMENT_3D('',#90534,#46119,#46120);
#37347=AXIS2_PLACEMENT_3D('',#90536,#46121,#46122);
#37348=AXIS2_PLACEMENT_3D('',#90537,#46123,#46124);
#37349=AXIS2_PLACEMENT_3D('',#90538,#46125,#46126);
#37350=AXIS2_PLACEMENT_3D('',#90539,#46127,#46128);
#37351=AXIS2_PLACEMENT_3D('',#90541,#46129,#46130);
#37352=AXIS2_PLACEMENT_3D('',#90542,#46131,#46132);
#37353=AXIS2_PLACEMENT_3D('',#90543,#46133,#46134);
#37354=AXIS2_PLACEMENT_3D('',#90545,#46135,#46136);
#37355=AXIS2_PLACEMENT_3D('',#90547,#46138,#46139);
#37356=AXIS2_PLACEMENT_3D('',#90548,#46140,#46141);
#37357=AXIS2_PLACEMENT_3D('',#90549,#46142,#46143);
#37358=AXIS2_PLACEMENT_3D('',#90551,#46144,#46145);
#37359=AXIS2_PLACEMENT_3D('',#90552,#46146,#46147);
#37360=AXIS2_PLACEMENT_3D('',#90553,#46148,#46149);
#37361=AXIS2_PLACEMENT_3D('',#90554,#46150,#46151);
#37362=AXIS2_PLACEMENT_3D('',#90555,#46152,#46153);
#37363=AXIS2_PLACEMENT_3D('',#90558,#46155,#46156);
#37364=AXIS2_PLACEMENT_3D('',#90559,#46157,#46158);
#37365=AXIS2_PLACEMENT_3D('',#90561,#46159,#46160);
#37366=AXIS2_PLACEMENT_3D('',#90562,#46161,#46162);
#37367=AXIS2_PLACEMENT_3D('',#90563,#46163,#46164);
#37368=AXIS2_PLACEMENT_3D('',#90620,#46171,#46172);
#37369=AXIS2_PLACEMENT_3D('',#90622,#46173,#46174);
#37370=AXIS2_PLACEMENT_3D('',#90625,#46176,#46177);
#37371=AXIS2_PLACEMENT_3D('',#90626,#46178,#46179);
#37372=AXIS2_PLACEMENT_3D('',#90628,#46180,#46181);
#37373=AXIS2_PLACEMENT_3D('',#90630,#46182,#46183);
#37374=AXIS2_PLACEMENT_3D('',#90632,#46185,#46186);
#37375=AXIS2_PLACEMENT_3D('',#90634,#46187,#46188);
#37376=AXIS2_PLACEMENT_3D('',#90637,#46190,#46191);
#37377=AXIS2_PLACEMENT_3D('',#90638,#46192,#46193);
#37378=AXIS2_PLACEMENT_3D('',#90644,#46197,#46198);
#37379=AXIS2_PLACEMENT_3D('',#90646,#46199,#46200);
#37380=AXIS2_PLACEMENT_3D('',#90648,#46201,#46202);
#37381=AXIS2_PLACEMENT_3D('',#90650,#46204,#46205);
#37382=AXIS2_PLACEMENT_3D('',#90654,#46207,#46208);
#37383=AXIS2_PLACEMENT_3D('',#90655,#46209,#46210);
#37384=AXIS2_PLACEMENT_3D('',#90656,#46211,#46212);
#37385=AXIS2_PLACEMENT_3D('',#90658,#46213,#46214);
#37386=AXIS2_PLACEMENT_3D('',#90660,#46215,#46216);
#37387=AXIS2_PLACEMENT_3D('',#90662,#46218,#46219);
#37388=AXIS2_PLACEMENT_3D('',#90663,#46220,#46221);
#37389=AXIS2_PLACEMENT_3D('',#90664,#46222,#46223);
#37390=AXIS2_PLACEMENT_3D('',#90666,#46224,#46225);
#37391=AXIS2_PLACEMENT_3D('',#90667,#46226,#46227);
#37392=AXIS2_PLACEMENT_3D('',#90668,#46228,#46229);
#37393=AXIS2_PLACEMENT_3D('',#90669,#46230,#46231);
#37394=AXIS2_PLACEMENT_3D('',#90670,#46232,#46233);
#37395=AXIS2_PLACEMENT_3D('',#90672,#46234,#46235);
#37396=AXIS2_PLACEMENT_3D('',#90674,#46237,#46238);
#37397=AXIS2_PLACEMENT_3D('',#90676,#46239,#46240);
#37398=AXIS2_PLACEMENT_3D('',#90677,#46241,#46242);
#37399=AXIS2_PLACEMENT_3D('',#90715,#46243,#46244);
#37400=AXIS2_PLACEMENT_3D('',#90771,#46245,#46246);
#37401=AXIS2_PLACEMENT_3D('',#90772,#46247,#46248);
#37402=AXIS2_PLACEMENT_3D('',#90773,#46249,#46250);
#37403=AXIS2_PLACEMENT_3D('',#90774,#46251,#46252);
#37404=AXIS2_PLACEMENT_3D('',#90775,#46253,#46254);
#37405=AXIS2_PLACEMENT_3D('',#90907,#46255,#46256);
#37406=AXIS2_PLACEMENT_3D('',#90908,#46257,#46258);
#37407=AXIS2_PLACEMENT_3D('',#90909,#46259,#46260);
#37408=AXIS2_PLACEMENT_3D('',#90910,#46261,#46262);
#37409=AXIS2_PLACEMENT_3D('',#90911,#46263,#46264);
#37410=AXIS2_PLACEMENT_3D('',#90912,#46265,#46266);
#37411=AXIS2_PLACEMENT_3D('',#90915,#46267,#46268);
#37412=AXIS2_PLACEMENT_3D('',#91059,#46271,#46272);
#37413=AXIS2_PLACEMENT_3D('',#91117,#46273,#46274);
#37414=AXIS2_PLACEMENT_3D('',#91119,#46275,#46276);
#37415=AXIS2_PLACEMENT_3D('',#91120,#46277,#46278);
#37416=AXIS2_PLACEMENT_3D('',#91121,#46279,#46280);
#37417=AXIS2_PLACEMENT_3D('',#91252,#46283,#46284);
#37418=AXIS2_PLACEMENT_3D('',#91312,#46285,#46286);
#37419=AXIS2_PLACEMENT_3D('',#91314,#46287,#46288);
#37420=AXIS2_PLACEMENT_3D('',#91315,#46289,#46290);
#37421=AXIS2_PLACEMENT_3D('',#91316,#46291,#46292);
#37422=AXIS2_PLACEMENT_3D('',#91317,#46293,#46294);
#37423=AXIS2_PLACEMENT_3D('',#91318,#46295,#46296);
#37424=AXIS2_PLACEMENT_3D('',#91324,#46300,#46301);
#37425=AXIS2_PLACEMENT_3D('',#91325,#46302,#46303);
#37426=AXIS2_PLACEMENT_3D('',#91326,#46304,#46305);
#37427=AXIS2_PLACEMENT_3D('',#91331,#46308,#46309);
#37428=AXIS2_PLACEMENT_3D('',#91332,#46310,#46311);
#37429=AXIS2_PLACEMENT_3D('',#91333,#46312,#46313);
#37430=AXIS2_PLACEMENT_3D('',#91334,#46314,#46315);
#37431=AXIS2_PLACEMENT_3D('',#91340,#46319,#46320);
#37432=AXIS2_PLACEMENT_3D('',#91341,#46321,#46322);
#37433=AXIS2_PLACEMENT_3D('',#91342,#46323,#46324);
#37434=AXIS2_PLACEMENT_3D('',#91345,#46325,#46326);
#37435=AXIS2_PLACEMENT_3D('',#91348,#46329,#46330);
#37436=AXIS2_PLACEMENT_3D('',#91349,#46331,#46332);
#37437=AXIS2_PLACEMENT_3D('',#91350,#46333,#46334);
#37438=AXIS2_PLACEMENT_3D('',#91352,#46335,#46336);
#37439=AXIS2_PLACEMENT_3D('',#91355,#46338,#46339);
#37440=AXIS2_PLACEMENT_3D('',#91356,#46340,#46341);
#37441=AXIS2_PLACEMENT_3D('',#91357,#46342,#46343);
#37442=AXIS2_PLACEMENT_3D('',#91358,#46344,#46345);
#37443=AXIS2_PLACEMENT_3D('',#91360,#46346,#46347);
#37444=AXIS2_PLACEMENT_3D('',#91362,#46348,#46349);
#37445=AXIS2_PLACEMENT_3D('',#91363,#46350,#46351);
#37446=AXIS2_PLACEMENT_3D('',#91364,#46352,#46353);
#37447=AXIS2_PLACEMENT_3D('',#91365,#46354,#46355);
#37448=AXIS2_PLACEMENT_3D('',#91366,#46356,#46357);
#37449=AXIS2_PLACEMENT_3D('',#91368,#46358,#46359);
#37450=AXIS2_PLACEMENT_3D('',#91371,#46361,#46362);
#37451=AXIS2_PLACEMENT_3D('',#91372,#46363,#46364);
#37452=AXIS2_PLACEMENT_3D('',#91373,#46365,#46366);
#37453=AXIS2_PLACEMENT_3D('',#91374,#46367,#46368);
#37454=AXIS2_PLACEMENT_3D('',#91376,#46369,#46370);
#37455=AXIS2_PLACEMENT_3D('',#91378,#46371,#46372);
#37456=AXIS2_PLACEMENT_3D('',#91379,#46373,#46374);
#37457=AXIS2_PLACEMENT_3D('',#91380,#46375,#46376);
#37458=AXIS2_PLACEMENT_3D('',#91381,#46377,#46378);
#37459=AXIS2_PLACEMENT_3D('',#91382,#46379,#46380);
#37460=AXIS2_PLACEMENT_3D('',#91385,#46381,#46382);
#37461=AXIS2_PLACEMENT_3D('',#91387,#46383,#46384);
#37462=AXIS2_PLACEMENT_3D('',#91388,#46385,#46386);
#37463=AXIS2_PLACEMENT_3D('',#91389,#46387,#46388);
#37464=AXIS2_PLACEMENT_3D('',#91390,#46389,#46390);
#37465=AXIS2_PLACEMENT_3D('',#91391,#46391,#46392);
#37466=AXIS2_PLACEMENT_3D('',#91392,#46393,#46394);
#37467=AXIS2_PLACEMENT_3D('',#91393,#46395,#46396);
#37468=AXIS2_PLACEMENT_3D('',#91394,#46397,#46398);
#37469=AXIS2_PLACEMENT_3D('',#91432,#46399,#46400);
#37470=AXIS2_PLACEMENT_3D('',#91488,#46401,#46402);
#37471=AXIS2_PLACEMENT_3D('',#91490,#46403,#46404);
#37472=AXIS2_PLACEMENT_3D('',#91492,#46405,#46406);
#37473=AXIS2_PLACEMENT_3D('',#91493,#46407,#46408);
#37474=AXIS2_PLACEMENT_3D('',#91494,#46409,#46410);
#37475=AXIS2_PLACEMENT_3D('',#91560,#46411,#46412);
#37476=AXIS2_PLACEMENT_3D('',#91598,#46413,#46414);
#37477=AXIS2_PLACEMENT_3D('',#91600,#46415,#46416);
#37478=AXIS2_PLACEMENT_3D('',#91602,#46417,#46418);
#37479=AXIS2_PLACEMENT_3D('',#91603,#46419,#46420);
#37480=AXIS2_PLACEMENT_3D('',#91604,#46421,#46422);
#37481=AXIS2_PLACEMENT_3D('',#91606,#46423,#46424);
#37482=AXIS2_PLACEMENT_3D('',#91609,#46426,#46427);
#37483=AXIS2_PLACEMENT_3D('',#91610,#46428,#46429);
#37484=AXIS2_PLACEMENT_3D('',#91616,#46433,#46434);
#37485=AXIS2_PLACEMENT_3D('',#91619,#46436,#46437);
#37486=AXIS2_PLACEMENT_3D('',#91620,#46438,#46439);
#37487=AXIS2_PLACEMENT_3D('',#91663,#46440,#46441);
#37488=AXIS2_PLACEMENT_3D('',#91665,#46442,#46443);
#37489=AXIS2_PLACEMENT_3D('',#91669,#46445,#46446);
#37490=AXIS2_PLACEMENT_3D('',#91732,#46448,#46449);
#37491=AXIS2_PLACEMENT_3D('',#91794,#46451,#46452);
#37492=AXIS2_PLACEMENT_3D('',#91795,#46453,#46454);
#37493=AXIS2_PLACEMENT_3D('',#91797,#46455,#46456);
#37494=AXIS2_PLACEMENT_3D('',#91799,#46457,#46458);
#37495=AXIS2_PLACEMENT_3D('',#91801,#46460,#46461);
#37496=AXIS2_PLACEMENT_3D('',#91805,#46463,#46464);
#37497=AXIS2_PLACEMENT_3D('',#91809,#46467,#46468);
#37498=AXIS2_PLACEMENT_3D('',#91811,#46469,#46470);
#37499=AXIS2_PLACEMENT_3D('',#91851,#46472,#46473);
#37500=AXIS2_PLACEMENT_3D('',#91853,#46474,#46475);
#37501=AXIS2_PLACEMENT_3D('',#91857,#46477,#46478);
#37502=AXIS2_PLACEMENT_3D('',#91861,#46481,#46482);
#37503=AXIS2_PLACEMENT_3D('',#91863,#46483,#46484);
#37504=AXIS2_PLACEMENT_3D('',#91903,#46486,#46487);
#37505=AXIS2_PLACEMENT_3D('',#91919,#46491,#46492);
#37506=AXIS2_PLACEMENT_3D('',#91920,#46493,#46494);
#37507=AXIS2_PLACEMENT_3D('',#91921,#46495,#46496);
#37508=AXIS2_PLACEMENT_3D('',#91922,#46497,#46498);
#37509=AXIS2_PLACEMENT_3D('',#91924,#46499,#46500);
#37510=AXIS2_PLACEMENT_3D('',#91925,#46501,#46502);
#37511=AXIS2_PLACEMENT_3D('',#91926,#46503,#46504);
#37512=AXIS2_PLACEMENT_3D('',#91928,#46505,#46506);
#37513=AXIS2_PLACEMENT_3D('',#91929,#46507,#46508);
#37514=AXIS2_PLACEMENT_3D('',#91930,#46509,#46510);
#37515=AXIS2_PLACEMENT_3D('',#91933,#46511,#46512);
#37516=AXIS2_PLACEMENT_3D('',#91944,#46515,#46516);
#37517=AXIS2_PLACEMENT_3D('',#91946,#46517,#46518);
#37518=AXIS2_PLACEMENT_3D('',#91989,#46520,#46521);
#37519=AXIS2_PLACEMENT_3D('',#91991,#46522,#46523);
#37520=AXIS2_PLACEMENT_3D('',#91993,#46525,#46526);
#37521=AXIS2_PLACEMENT_3D('',#92003,#46531,#46532);
#37522=AXIS2_PLACEMENT_3D('',#92005,#46534,#46535);
#37523=AXIS2_PLACEMENT_3D('',#92007,#46536,#46537);
#37524=AXIS2_PLACEMENT_3D('',#92010,#46539,#46540);
#37525=AXIS2_PLACEMENT_3D('',#92011,#46541,#46542);
#37526=AXIS2_PLACEMENT_3D('',#92015,#46544,#46545);
#37527=AXIS2_PLACEMENT_3D('',#92016,#46546,#46547);
#37528=AXIS2_PLACEMENT_3D('',#92017,#46548,#46549);
#37529=AXIS2_PLACEMENT_3D('',#92019,#46550,#46551);
#37530=AXIS2_PLACEMENT_3D('',#92022,#46553,#46554);
#37531=AXIS2_PLACEMENT_3D('',#92023,#46555,#46556);
#37532=AXIS2_PLACEMENT_3D('',#92029,#46560,#46561);
#37533=AXIS2_PLACEMENT_3D('',#92063,#46562,#46563);
#37534=AXIS2_PLACEMENT_3D('',#92065,#46565,#46566);
#37535=AXIS2_PLACEMENT_3D('',#92067,#46567,#46568);
#37536=AXIS2_PLACEMENT_3D('',#92070,#46570,#46571);
#37537=AXIS2_PLACEMENT_3D('',#92071,#46572,#46573);
#37538=AXIS2_PLACEMENT_3D('',#92072,#46574,#46575);
#37539=AXIS2_PLACEMENT_3D('',#92073,#46576,#46577);
#37540=AXIS2_PLACEMENT_3D('',#92074,#46578,#46579);
#37541=AXIS2_PLACEMENT_3D('',#92076,#46580,#46581);
#37542=AXIS2_PLACEMENT_3D('',#92080,#46583,#46584);
#37543=AXIS2_PLACEMENT_3D('',#92082,#46586,#46587);
#37544=AXIS2_PLACEMENT_3D('',#92085,#46588,#46589);
#37545=AXIS2_PLACEMENT_3D('',#92087,#46590,#46591);
#37546=AXIS2_PLACEMENT_3D('',#92089,#46592,#46593);
#37547=AXIS2_PLACEMENT_3D('',#92090,#46594,#46595);
#37548=AXIS2_PLACEMENT_3D('',#92091,#46596,#46597);
#37549=AXIS2_PLACEMENT_3D('',#92094,#46598,#46599);
#37550=AXIS2_PLACEMENT_3D('',#92095,#46600,#46601);
#37551=AXIS2_PLACEMENT_3D('',#92096,#46602,#46603);
#37552=AXIS2_PLACEMENT_3D('',#92097,#46604,#46605);
#37553=AXIS2_PLACEMENT_3D('',#92100,#46606,#46607);
#37554=AXIS2_PLACEMENT_3D('',#92103,#46610,#46611);
#37555=AXIS2_PLACEMENT_3D('',#92106,#46612,#46613);
#37556=AXIS2_PLACEMENT_3D('',#92107,#46614,#46615);
#37557=AXIS2_PLACEMENT_3D('',#92108,#46616,#46617);
#37558=AXIS2_PLACEMENT_3D('',#92109,#46618,#46619);
#37559=AXIS2_PLACEMENT_3D('',#92112,#46620,#46621);
#37560=AXIS2_PLACEMENT_3D('',#92113,#46622,#46623);
#37561=AXIS2_PLACEMENT_3D('',#92114,#46624,#46625);
#37562=AXIS2_PLACEMENT_3D('',#92115,#46626,#46627);
#37563=AXIS2_PLACEMENT_3D('',#92117,#46628,#46629);
#37564=AXIS2_PLACEMENT_3D('',#92119,#46630,#46631);
#37565=AXIS2_PLACEMENT_3D('',#92120,#46632,#46633);
#37566=AXIS2_PLACEMENT_3D('',#92121,#46634,#46635);
#37567=AXIS2_PLACEMENT_3D('',#92124,#46636,#46637);
#37568=AXIS2_PLACEMENT_3D('',#92125,#46638,#46639);
#37569=AXIS2_PLACEMENT_3D('',#92126,#46640,#46641);
#37570=AXIS2_PLACEMENT_3D('',#92127,#46642,#46643);
#37571=AXIS2_PLACEMENT_3D('',#92130,#46646,#46647);
#37572=AXIS2_PLACEMENT_3D('',#92133,#46648,#46649);
#37573=AXIS2_PLACEMENT_3D('',#92135,#46650,#46651);
#37574=AXIS2_PLACEMENT_3D('',#92137,#46652,#46653);
#37575=AXIS2_PLACEMENT_3D('',#92138,#46654,#46655);
#37576=AXIS2_PLACEMENT_3D('',#92170,#46656,#46657);
#37577=AXIS2_PLACEMENT_3D('',#92176,#46658,#46659);
#37578=AXIS2_PLACEMENT_3D('',#92177,#46660,#46661);
#37579=AXIS2_PLACEMENT_3D('',#92179,#46662,#46663);
#37580=AXIS2_PLACEMENT_3D('',#92180,#46664,#46665);
#37581=AXIS2_PLACEMENT_3D('',#92181,#46666,#46667);
#37582=AXIS2_PLACEMENT_3D('',#92219,#46668,#46669);
#37583=AXIS2_PLACEMENT_3D('',#92221,#46670,#46671);
#37584=AXIS2_PLACEMENT_3D('',#92222,#46672,#46673);
#37585=AXIS2_PLACEMENT_3D('',#92288,#46674,#46675);
#37586=AXIS2_PLACEMENT_3D('',#92317,#46676,#46677);
#37587=AXIS2_PLACEMENT_3D('',#92319,#46678,#46679);
#37588=AXIS2_PLACEMENT_3D('',#92321,#46680,#46681);
#37589=AXIS2_PLACEMENT_3D('',#92322,#46682,#46683);
#37590=AXIS2_PLACEMENT_3D('',#92323,#46684,#46685);
#37591=AXIS2_PLACEMENT_3D('',#92326,#46686,#46687);
#37592=AXIS2_PLACEMENT_3D('',#92327,#46688,#46689);
#37593=AXIS2_PLACEMENT_3D('',#92328,#46690,#46691);
#37594=AXIS2_PLACEMENT_3D('',#92329,#46692,#46693);
#37595=AXIS2_PLACEMENT_3D('',#92331,#46694,#46695);
#37596=AXIS2_PLACEMENT_3D('',#92333,#46696,#46697);
#37597=AXIS2_PLACEMENT_3D('',#92334,#46698,#46699);
#37598=AXIS2_PLACEMENT_3D('',#92335,#46700,#46701);
#37599=AXIS2_PLACEMENT_3D('',#92375,#46704,#46705);
#37600=AXIS2_PLACEMENT_3D('',#92377,#46706,#46707);
#37601=AXIS2_PLACEMENT_3D('',#92378,#46708,#46709);
#37602=AXIS2_PLACEMENT_3D('',#92444,#46710,#46711);
#37603=AXIS2_PLACEMENT_3D('',#92482,#46712,#46713);
#37604=AXIS2_PLACEMENT_3D('',#92483,#46714,#46715);
#37605=AXIS2_PLACEMENT_3D('',#92484,#46716,#46717);
#37606=AXIS2_PLACEMENT_3D('',#92486,#46718,#46719);
#37607=AXIS2_PLACEMENT_3D('',#92488,#46720,#46721);
#37608=AXIS2_PLACEMENT_3D('',#92490,#46722,#46723);
#37609=AXIS2_PLACEMENT_3D('',#92492,#46724,#46725);
#37610=AXIS2_PLACEMENT_3D('',#92493,#46726,#46727);
#37611=AXIS2_PLACEMENT_3D('',#92494,#46728,#46729);
#37612=AXIS2_PLACEMENT_3D('',#92497,#46730,#46731);
#37613=AXIS2_PLACEMENT_3D('',#92498,#46732,#46733);
#37614=AXIS2_PLACEMENT_3D('',#92499,#46734,#46735);
#37615=AXIS2_PLACEMENT_3D('',#92500,#46736,#46737);
#37616=AXIS2_PLACEMENT_3D('',#92503,#46738,#46739);
#37617=AXIS2_PLACEMENT_3D('',#92506,#46742,#46743);
#37618=AXIS2_PLACEMENT_3D('',#92509,#46744,#46745);
#37619=AXIS2_PLACEMENT_3D('',#92510,#46746,#46747);
#37620=AXIS2_PLACEMENT_3D('',#92511,#46748,#46749);
#37621=AXIS2_PLACEMENT_3D('',#92512,#46750,#46751);
#37622=AXIS2_PLACEMENT_3D('',#92515,#46752,#46753);
#37623=AXIS2_PLACEMENT_3D('',#92516,#46754,#46755);
#37624=AXIS2_PLACEMENT_3D('',#92517,#46756,#46757);
#37625=AXIS2_PLACEMENT_3D('',#92518,#46758,#46759);
#37626=AXIS2_PLACEMENT_3D('',#92520,#46760,#46761);
#37627=AXIS2_PLACEMENT_3D('',#92522,#46762,#46763);
#37628=AXIS2_PLACEMENT_3D('',#92523,#46764,#46765);
#37629=AXIS2_PLACEMENT_3D('',#92524,#46766,#46767);
#37630=AXIS2_PLACEMENT_3D('',#92527,#46768,#46769);
#37631=AXIS2_PLACEMENT_3D('',#92528,#46770,#46771);
#37632=AXIS2_PLACEMENT_3D('',#92529,#46772,#46773);
#37633=AXIS2_PLACEMENT_3D('',#92530,#46774,#46775);
#37634=AXIS2_PLACEMENT_3D('',#92533,#46778,#46779);
#37635=AXIS2_PLACEMENT_3D('',#92674,#46782,#46783);
#37636=AXIS2_PLACEMENT_3D('',#92678,#46785,#46786);
#37637=AXIS2_PLACEMENT_3D('',#92680,#46788,#46789);
#37638=AXIS2_PLACEMENT_3D('',#92757,#46790,#46791);
#37639=AXIS2_PLACEMENT_3D('',#92826,#46792,#46793);
#37640=AXIS2_PLACEMENT_3D('',#92827,#46794,#46795);
#37641=AXIS2_PLACEMENT_3D('',#92829,#46796,#46797);
#37642=AXIS2_PLACEMENT_3D('',#92830,#46798,#46799);
#37643=AXIS2_PLACEMENT_3D('',#92831,#46800,#46801);
#37644=AXIS2_PLACEMENT_3D('',#92946,#46802,#46803);
#37645=AXIS2_PLACEMENT_3D('',#92947,#46804,#46805);
#37646=AXIS2_PLACEMENT_3D('',#92948,#46806,#46807);
#37647=AXIS2_PLACEMENT_3D('',#92950,#46808,#46809);
#37648=AXIS2_PLACEMENT_3D('',#92951,#46810,#46811);
#37649=AXIS2_PLACEMENT_3D('',#92952,#46812,#46813);
#37650=AXIS2_PLACEMENT_3D('',#92954,#46814,#46815);
#37651=AXIS2_PLACEMENT_3D('',#92955,#46816,#46817);
#37652=AXIS2_PLACEMENT_3D('',#92956,#46818,#46819);
#37653=AXIS2_PLACEMENT_3D('',#92958,#46820,#46821);
#37654=AXIS2_PLACEMENT_3D('',#92959,#46822,#46823);
#37655=AXIS2_PLACEMENT_3D('',#92960,#46824,#46825);
#37656=AXIS2_PLACEMENT_3D('',#92963,#46828,#46829);
#37657=AXIS2_PLACEMENT_3D('',#93024,#46830,#46831);
#37658=AXIS2_PLACEMENT_3D('',#93025,#46832,#46833);
#37659=AXIS2_PLACEMENT_3D('',#93026,#46834,#46835);
#37660=AXIS2_PLACEMENT_3D('',#93028,#46836,#46837);
#37661=AXIS2_PLACEMENT_3D('',#93030,#46838,#46839);
#37662=AXIS2_PLACEMENT_3D('',#93031,#46840,#46841);
#37663=AXIS2_PLACEMENT_3D('',#93032,#46842,#46843);
#37664=AXIS2_PLACEMENT_3D('',#93034,#46844,#46845);
#37665=AXIS2_PLACEMENT_3D('',#93036,#46846,#46847);
#37666=AXIS2_PLACEMENT_3D('',#93037,#46848,#46849);
#37667=AXIS2_PLACEMENT_3D('',#93038,#46850,#46851);
#37668=AXIS2_PLACEMENT_3D('',#93041,#46852,#46853);
#37669=AXIS2_PLACEMENT_3D('',#93042,#46854,#46855);
#37670=AXIS2_PLACEMENT_3D('',#93043,#46856,#46857);
#37671=AXIS2_PLACEMENT_3D('',#93044,#46858,#46859);
#37672=AXIS2_PLACEMENT_3D('',#93046,#46860,#46861);
#37673=AXIS2_PLACEMENT_3D('',#93048,#46862,#46863);
#37674=AXIS2_PLACEMENT_3D('',#93049,#46864,#46865);
#37675=AXIS2_PLACEMENT_3D('',#93050,#46866,#46867);
#37676=AXIS2_PLACEMENT_3D('',#93052,#46868,#46869);
#37677=AXIS2_PLACEMENT_3D('',#93053,#46870,#46871);
#37678=AXIS2_PLACEMENT_3D('',#93054,#46872,#46873);
#37679=AXIS2_PLACEMENT_3D('',#93056,#46874,#46875);
#37680=AXIS2_PLACEMENT_3D('',#93058,#46877,#46878);
#37681=AXIS2_PLACEMENT_3D('',#93061,#46880,#46881);
#37682=AXIS2_PLACEMENT_3D('',#93062,#46882,#46883);
#37683=AXIS2_PLACEMENT_3D('',#93063,#46884,#46885);
#37684=AXIS2_PLACEMENT_3D('',#93164,#46886,#46887);
#37685=AXIS2_PLACEMENT_3D('',#93215,#46888,#46889);
#37686=AXIS2_PLACEMENT_3D('',#93216,#46890,#46891);
#37687=AXIS2_PLACEMENT_3D('',#93219,#46892,#46893);
#37688=AXIS2_PLACEMENT_3D('',#93223,#46895,#46896);
#37689=AXIS2_PLACEMENT_3D('',#93225,#46898,#46899);
#37690=AXIS2_PLACEMENT_3D('',#93227,#46900,#46901);
#37691=AXIS2_PLACEMENT_3D('',#93229,#46902,#46903);
#37692=AXIS2_PLACEMENT_3D('',#93230,#46904,#46905);
#37693=AXIS2_PLACEMENT_3D('',#93231,#46906,#46907);
#37694=AXIS2_PLACEMENT_3D('',#93234,#46908,#46909);
#37695=AXIS2_PLACEMENT_3D('',#93235,#46910,#46911);
#37696=AXIS2_PLACEMENT_3D('',#93236,#46912,#46913);
#37697=AXIS2_PLACEMENT_3D('',#93238,#46914,#46915);
#37698=AXIS2_PLACEMENT_3D('',#93240,#46916,#46917);
#37699=AXIS2_PLACEMENT_3D('',#93241,#46918,#46919);
#37700=AXIS2_PLACEMENT_3D('',#93242,#46920,#46921);
#37701=AXIS2_PLACEMENT_3D('',#93244,#46922,#46923);
#37702=AXIS2_PLACEMENT_3D('',#93246,#46924,#46925);
#37703=AXIS2_PLACEMENT_3D('',#93247,#46926,#46927);
#37704=AXIS2_PLACEMENT_3D('',#93248,#46928,#46929);
#37705=AXIS2_PLACEMENT_3D('',#93250,#46930,#46931);
#37706=AXIS2_PLACEMENT_3D('',#93253,#46933,#46934);
#37707=AXIS2_PLACEMENT_3D('',#93254,#46935,#46936);
#37708=AXIS2_PLACEMENT_3D('',#93256,#46937,#46938);
#37709=AXIS2_PLACEMENT_3D('',#93259,#46940,#46941);
#37710=AXIS2_PLACEMENT_3D('',#93260,#46942,#46943);
#37711=AXIS2_PLACEMENT_3D('',#93262,#46944,#46945);
#37712=AXIS2_PLACEMENT_3D('',#93263,#46946,#46947);
#37713=AXIS2_PLACEMENT_3D('',#93264,#46948,#46949);
#37714=AXIS2_PLACEMENT_3D('',#93267,#46951,#46952);
#37715=AXIS2_PLACEMENT_3D('',#93268,#46953,#46954);
#37716=AXIS2_PLACEMENT_3D('',#93270,#46955,#46956);
#37717=AXIS2_PLACEMENT_3D('',#93271,#46957,#46958);
#37718=AXIS2_PLACEMENT_3D('',#93272,#46959,#46960);
#37719=AXIS2_PLACEMENT_3D('',#93275,#46962,#46963);
#37720=AXIS2_PLACEMENT_3D('',#93276,#46964,#46965);
#37721=AXIS2_PLACEMENT_3D('',#93277,#46966,#46967);
#37722=AXIS2_PLACEMENT_3D('',#93278,#46968,#46969);
#37723=AXIS2_PLACEMENT_3D('',#93280,#46970,#46971);
#37724=AXIS2_PLACEMENT_3D('',#93281,#46972,#46973);
#37725=AXIS2_PLACEMENT_3D('',#93282,#46974,#46975);
#37726=AXIS2_PLACEMENT_3D('',#93285,#46977,#46978);
#37727=AXIS2_PLACEMENT_3D('',#93286,#46979,#46980);
#37728=AXIS2_PLACEMENT_3D('',#93288,#46981,#46982);
#37729=AXIS2_PLACEMENT_3D('',#93289,#46983,#46984);
#37730=AXIS2_PLACEMENT_3D('',#93290,#46985,#46986);
#37731=AXIS2_PLACEMENT_3D('',#93292,#46987,#46988);
#37732=AXIS2_PLACEMENT_3D('',#93294,#46990,#46991);
#37733=AXIS2_PLACEMENT_3D('',#93296,#46992,#46993);
#37734=AXIS2_PLACEMENT_3D('',#93297,#46994,#46995);
#37735=AXIS2_PLACEMENT_3D('',#93298,#46996,#46997);
#37736=AXIS2_PLACEMENT_3D('',#93300,#46998,#46999);
#37737=AXIS2_PLACEMENT_3D('',#93302,#47001,#47002);
#37738=AXIS2_PLACEMENT_3D('',#93304,#47003,#47004);
#37739=AXIS2_PLACEMENT_3D('',#93305,#47005,#47006);
#37740=AXIS2_PLACEMENT_3D('',#93306,#47007,#47008);
#37741=AXIS2_PLACEMENT_3D('',#93308,#47009,#47010);
#37742=AXIS2_PLACEMENT_3D('',#93310,#47012,#47013);
#37743=AXIS2_PLACEMENT_3D('',#93311,#47014,#47015);
#37744=AXIS2_PLACEMENT_3D('',#93312,#47016,#47017);
#37745=AXIS2_PLACEMENT_3D('',#93313,#47018,#47019);
#37746=AXIS2_PLACEMENT_3D('',#93317,#47021,#47022);
#37747=AXIS2_PLACEMENT_3D('',#93320,#47024,#47025);
#37748=AXIS2_PLACEMENT_3D('',#93321,#47026,#47027);
#37749=AXIS2_PLACEMENT_3D('',#93476,#47028,#47029);
#37750=AXIS2_PLACEMENT_3D('',#93523,#47030,#47031);
#37751=AXIS2_PLACEMENT_3D('',#93525,#47032,#47033);
#37752=AXIS2_PLACEMENT_3D('',#93527,#47034,#47035);
#37753=AXIS2_PLACEMENT_3D('',#93528,#47036,#47037);
#37754=AXIS2_PLACEMENT_3D('',#93529,#47038,#47039);
#37755=AXIS2_PLACEMENT_3D('',#93531,#47040,#47041);
#37756=AXIS2_PLACEMENT_3D('',#93534,#47043,#47044);
#37757=AXIS2_PLACEMENT_3D('',#93535,#47045,#47046);
#37758=AXIS2_PLACEMENT_3D('',#93536,#47047,#47048);
#37759=AXIS2_PLACEMENT_3D('',#93537,#47049,#47050);
#37760=AXIS2_PLACEMENT_3D('',#93538,#47051,#47052);
#37761=AXIS2_PLACEMENT_3D('',#93539,#47053,#47054);
#37762=AXIS2_PLACEMENT_3D('',#93540,#47055,#47056);
#37763=AXIS2_PLACEMENT_3D('',#93541,#47057,#47058);
#37764=AXIS2_PLACEMENT_3D('',#93631,#47059,#47060);
#37765=AXIS2_PLACEMENT_3D('',#93632,#47061,#47062);
#37766=AXIS2_PLACEMENT_3D('',#93694,#47063,#47064);
#37767=AXIS2_PLACEMENT_3D('',#93695,#47065,#47066);
#37768=AXIS2_PLACEMENT_3D('',#93751,#47067,#47068);
#37769=AXIS2_PLACEMENT_3D('',#93810,#47069,#47070);
#37770=AXIS2_PLACEMENT_3D('',#93811,#47071,#47072);
#37771=AXIS2_PLACEMENT_3D('',#93812,#47073,#47074);
#37772=AXIS2_PLACEMENT_3D('',#93814,#47076,#47077);
#37773=AXIS2_PLACEMENT_3D('',#93815,#47078,#47079);
#37774=AXIS2_PLACEMENT_3D('',#93817,#47081,#47082);
#37775=AXIS2_PLACEMENT_3D('',#93818,#47083,#47084);
#37776=AXIS2_PLACEMENT_3D('',#93820,#47086,#47087);
#37777=AXIS2_PLACEMENT_3D('',#93822,#47089,#47090);
#37778=AXIS2_PLACEMENT_3D('',#93824,#47091,#47092);
#37779=AXIS2_PLACEMENT_3D('',#93839,#47094,#47095);
#37780=AXIS2_PLACEMENT_3D('',#93841,#47096,#47097);
#37781=AXIS2_PLACEMENT_3D('',#93842,#47098,#47099);
#37782=AXIS2_PLACEMENT_3D('',#93843,#47100,#47101);
#37783=AXIS2_PLACEMENT_3D('',#93845,#47102,#47103);
#37784=AXIS2_PLACEMENT_3D('',#93847,#47104,#47105);
#37785=AXIS2_PLACEMENT_3D('',#93851,#47107,#47108);
#37786=AXIS2_PLACEMENT_3D('',#93853,#47109,#47110);
#37787=AXIS2_PLACEMENT_3D('',#93855,#47112,#47113);
#37788=AXIS2_PLACEMENT_3D('',#93857,#47114,#47115);
#37789=AXIS2_PLACEMENT_3D('',#93858,#47116,#47117);
#37790=AXIS2_PLACEMENT_3D('',#93860,#47118,#47119);
#37791=AXIS2_PLACEMENT_3D('',#93861,#47120,#47121);
#37792=AXIS2_PLACEMENT_3D('',#93863,#47123,#47124);
#37793=AXIS2_PLACEMENT_3D('',#93864,#47125,#47126);
#37794=AXIS2_PLACEMENT_3D('',#93873,#47128,#47129);
#37795=AXIS2_PLACEMENT_3D('',#93993,#47131,#47132);
#37796=AXIS2_PLACEMENT_3D('',#94021,#47134,#47135);
#37797=AXIS2_PLACEMENT_3D('',#94022,#47136,#47137);
#37798=AXIS2_PLACEMENT_3D('',#94023,#47138,#47139);
#37799=AXIS2_PLACEMENT_3D('',#94027,#47141,#47142);
#37800=AXIS2_PLACEMENT_3D('',#94028,#47143,#47144);
#37801=AXIS2_PLACEMENT_3D('',#94029,#47145,#47146);
#37802=AXIS2_PLACEMENT_3D('',#94030,#47147,#47148);
#37803=AXIS2_PLACEMENT_3D('',#94031,#47149,#47150);
#37804=AXIS2_PLACEMENT_3D('',#94048,#47151,#47152);
#37805=AXIS2_PLACEMENT_3D('',#94049,#47153,#47154);
#37806=AXIS2_PLACEMENT_3D('',#94050,#47155,#47156);
#37807=AXIS2_PLACEMENT_3D('',#94051,#47157,#47158);
#37808=AXIS2_PLACEMENT_3D('',#94052,#47159,#47160);
#37809=AXIS2_PLACEMENT_3D('',#94053,#47161,#47162);
#37810=AXIS2_PLACEMENT_3D('',#94054,#47163,#47164);
#37811=AXIS2_PLACEMENT_3D('',#94055,#47165,#47166);
#37812=AXIS2_PLACEMENT_3D('',#94056,#47167,#47168);
#37813=AXIS2_PLACEMENT_3D('',#94057,#47169,#47170);
#37814=AXIS2_PLACEMENT_3D('',#94058,#47171,#47172);
#37815=AXIS2_PLACEMENT_3D('',#94059,#47173,#47174);
#37816=AXIS2_PLACEMENT_3D('',#94060,#47175,#47176);
#37817=AXIS2_PLACEMENT_3D('',#94061,#47177,#47178);
#37818=AXIS2_PLACEMENT_3D('',#94062,#47179,#47180);
#37819=AXIS2_PLACEMENT_3D('',#94068,#47184,#47185);
#37820=AXIS2_PLACEMENT_3D('',#94071,#47188,#47189);
#37821=AXIS2_PLACEMENT_3D('',#94074,#47191,#47192);
#37822=AXIS2_PLACEMENT_3D('',#94075,#47193,#47194);
#37823=AXIS2_PLACEMENT_3D('',#94079,#47197,#47198);
#37824=AXIS2_PLACEMENT_3D('',#94082,#47200,#47201);
#37825=AXIS2_PLACEMENT_3D('',#94083,#47202,#47203);
#37826=AXIS2_PLACEMENT_3D('',#94085,#47205,#47206);
#37827=AXIS2_PLACEMENT_3D('',#94086,#47207,#47208);
#37828=AXIS2_PLACEMENT_3D('',#94088,#47210,#47211);
#37829=AXIS2_PLACEMENT_3D('',#94090,#47213,#47214);
#37830=AXIS2_PLACEMENT_3D('',#94091,#47215,#47216);
#37831=AXIS2_PLACEMENT_3D('',#94094,#47219,#47220);
#37832=AXIS2_PLACEMENT_3D('',#94096,#47222,#47223);
#37833=AXIS2_PLACEMENT_3D('',#94098,#47225,#47226);
#37834=AXIS2_PLACEMENT_3D('',#94100,#47228,#47229);
#37835=AXIS2_PLACEMENT_3D('',#94102,#47231,#47232);
#37836=AXIS2_PLACEMENT_3D('',#94103,#47233,#47234);
#37837=AXIS2_PLACEMENT_3D('',#94106,#47237,#47238);
#37838=AXIS2_PLACEMENT_3D('',#94108,#47240,#47241);
#37839=AXIS2_PLACEMENT_3D('',#94110,#47243,#47244);
#37840=AXIS2_PLACEMENT_3D('',#94113,#47246,#47247);
#37841=AXIS2_PLACEMENT_3D('',#94114,#47248,#47249);
#37842=AXIS2_PLACEMENT_3D('',#94117,#47251,#47252);
#37843=AXIS2_PLACEMENT_3D('',#94118,#47253,#47254);
#37844=AXIS2_PLACEMENT_3D('',#94120,#47255,#47256);
#37845=AXIS2_PLACEMENT_3D('',#94122,#47258,#47259);
#37846=AXIS2_PLACEMENT_3D('',#94125,#47261,#47262);
#37847=AXIS2_PLACEMENT_3D('',#94126,#47263,#47264);
#37848=AXIS2_PLACEMENT_3D('',#94128,#47266,#47267);
#37849=AXIS2_PLACEMENT_3D('',#94129,#47268,#47269);
#37850=AXIS2_PLACEMENT_3D('',#94130,#47270,#47271);
#37851=AXIS2_PLACEMENT_3D('',#94205,#47272,#47273);
#37852=AXIS2_PLACEMENT_3D('',#94206,#47274,#47275);
#37853=AXIS2_PLACEMENT_3D('',#94207,#47276,#47277);
#37854=AXIS2_PLACEMENT_3D('',#94208,#47278,#47279);
#37855=AXIS2_PLACEMENT_3D('',#94209,#47280,#47281);
#37856=AXIS2_PLACEMENT_3D('',#94210,#47282,#47283);
#37857=AXIS2_PLACEMENT_3D('',#94212,#47285,#47286);
#37858=AXIS2_PLACEMENT_3D('',#94214,#47287,#47288);
#37859=AXIS2_PLACEMENT_3D('',#94216,#47290,#47291);
#37860=AXIS2_PLACEMENT_3D('',#94217,#47292,#47293);
#37861=AXIS2_PLACEMENT_3D('',#94220,#47294,#47295);
#37862=AXIS2_PLACEMENT_3D('',#94221,#47296,#47297);
#37863=AXIS2_PLACEMENT_3D('',#94222,#47298,#47299);
#37864=AXIS2_PLACEMENT_3D('',#94223,#47300,#47301);
#37865=AXIS2_PLACEMENT_3D('',#94224,#47302,#47303);
#37866=AXIS2_PLACEMENT_3D('',#94225,#47304,#47305);
#37867=AXIS2_PLACEMENT_3D('',#94227,#47307,#47308);
#37868=AXIS2_PLACEMENT_3D('',#94228,#47309,#47310);
#37869=AXIS2_PLACEMENT_3D('',#94229,#47311,#47312);
#37870=AXIS2_PLACEMENT_3D('',#94230,#47313,#47314);
#37871=AXIS2_PLACEMENT_3D('',#94231,#47315,#47316);
#37872=AXIS2_PLACEMENT_3D('',#94272,#47317,#47318);
#37873=AXIS2_PLACEMENT_3D('',#94273,#47319,#47320);
#37874=AXIS2_PLACEMENT_3D('',#94332,#47321,#47322);
#37875=AXIS2_PLACEMENT_3D('',#94403,#47323,#47324);
#37876=AXIS2_PLACEMENT_3D('',#94405,#47326,#47327);
#37877=AXIS2_PLACEMENT_3D('',#94406,#47328,#47329);
#37878=AXIS2_PLACEMENT_3D('',#94407,#47330,#47331);
#37879=AXIS2_PLACEMENT_3D('',#94408,#47332,#47333);
#37880=AXIS2_PLACEMENT_3D('',#94411,#47334,#47335);
#37881=AXIS2_PLACEMENT_3D('',#94413,#47336,#47337);
#37882=AXIS2_PLACEMENT_3D('',#94414,#47338,#47339);
#37883=AXIS2_PLACEMENT_3D('',#94415,#47340,#47341);
#37884=AXIS2_PLACEMENT_3D('',#94418,#47344,#47345);
#37885=AXIS2_PLACEMENT_3D('',#94419,#47346,#47347);
#37886=AXIS2_PLACEMENT_3D('',#94420,#47348,#47349);
#37887=AXIS2_PLACEMENT_3D('',#94421,#47350,#47351);
#37888=AXIS2_PLACEMENT_3D('',#94422,#47352,#47353);
#37889=AXIS2_PLACEMENT_3D('',#94426,#47355,#47356);
#37890=AXIS2_PLACEMENT_3D('',#94427,#47357,#47358);
#37891=AXIS2_PLACEMENT_3D('',#94428,#47359,#47360);
#37892=AXIS2_PLACEMENT_3D('',#94430,#47361,#47362);
#37893=AXIS2_PLACEMENT_3D('',#94431,#47363,#47364);
#37894=AXIS2_PLACEMENT_3D('',#94432,#47365,#47366);
#37895=AXIS2_PLACEMENT_3D('',#94434,#47367,#47368);
#37896=AXIS2_PLACEMENT_3D('',#94435,#47369,#47370);
#37897=AXIS2_PLACEMENT_3D('',#94436,#47371,#47372);
#37898=AXIS2_PLACEMENT_3D('',#94438,#47373,#47374);
#37899=AXIS2_PLACEMENT_3D('',#94439,#47375,#47376);
#37900=AXIS2_PLACEMENT_3D('',#94440,#47377,#47378);
#37901=AXIS2_PLACEMENT_3D('',#94443,#47380,#47381);
#37902=AXIS2_PLACEMENT_3D('',#94444,#47382,#47383);
#37903=AXIS2_PLACEMENT_3D('',#94445,#47384,#47385);
#37904=AXIS2_PLACEMENT_3D('',#94448,#47387,#47388);
#37905=AXIS2_PLACEMENT_3D('',#94449,#47389,#47390);
#37906=AXIS2_PLACEMENT_3D('',#94451,#47391,#47392);
#37907=AXIS2_PLACEMENT_3D('',#94452,#47393,#47394);
#37908=AXIS2_PLACEMENT_3D('',#94454,#47395,#47396);
#37909=AXIS2_PLACEMENT_3D('',#94455,#47397,#47398);
#37910=AXIS2_PLACEMENT_3D('',#94590,#47399,#47400);
#37911=AXIS2_PLACEMENT_3D('',#94591,#47401,#47402);
#37912=AXIS2_PLACEMENT_3D('',#94592,#47403,#47404);
#37913=AXIS2_PLACEMENT_3D('',#94679,#47405,#47406);
#37914=AXIS2_PLACEMENT_3D('',#94680,#47407,#47408);
#37915=AXIS2_PLACEMENT_3D('',#94681,#47409,#47410);
#37916=AXIS2_PLACEMENT_3D('',#94682,#47411,#47412);
#37917=AXIS2_PLACEMENT_3D('',#94684,#47414,#47415);
#37918=AXIS2_PLACEMENT_3D('',#94686,#47417,#47418);
#37919=AXIS2_PLACEMENT_3D('',#94688,#47420,#47421);
#37920=AXIS2_PLACEMENT_3D('',#94689,#47422,#47423);
#37921=AXIS2_PLACEMENT_3D('',#94691,#47424,#47425);
#37922=AXIS2_PLACEMENT_3D('',#94693,#47427,#47428);
#37923=AXIS2_PLACEMENT_3D('',#94694,#47429,#47430);
#37924=AXIS2_PLACEMENT_3D('',#94695,#47431,#47432);
#37925=AXIS2_PLACEMENT_3D('',#94697,#47434,#47435);
#37926=AXIS2_PLACEMENT_3D('',#94699,#47437,#47438);
#37927=AXIS2_PLACEMENT_3D('',#94828,#47440,#47441);
#37928=AXIS2_PLACEMENT_3D('',#94829,#47442,#47443);
#37929=AXIS2_PLACEMENT_3D('',#94832,#47445,#47446);
#37930=AXIS2_PLACEMENT_3D('',#94833,#47447,#47448);
#37931=AXIS2_PLACEMENT_3D('',#94835,#47449,#47450);
#37932=AXIS2_PLACEMENT_3D('',#94836,#47451,#47452);
#37933=AXIS2_PLACEMENT_3D('',#94837,#47453,#47454);
#37934=AXIS2_PLACEMENT_3D('',#94839,#47455,#47456);
#37935=AXIS2_PLACEMENT_3D('',#94840,#47457,#47458);
#37936=AXIS2_PLACEMENT_3D('',#94841,#47459,#47460);
#37937=AXIS2_PLACEMENT_3D('',#94843,#47461,#47462);
#37938=AXIS2_PLACEMENT_3D('',#94844,#47463,#47464);
#37939=AXIS2_PLACEMENT_3D('',#94845,#47465,#47466);
#37940=AXIS2_PLACEMENT_3D('',#94848,#47468,#47469);
#37941=AXIS2_PLACEMENT_3D('',#94913,#47470,#47471);
#37942=AXIS2_PLACEMENT_3D('',#94914,#47472,#47473);
#37943=AXIS2_PLACEMENT_3D('',#94916,#47474,#47475);
#37944=AXIS2_PLACEMENT_3D('',#94917,#47476,#47477);
#37945=AXIS2_PLACEMENT_3D('',#94918,#47478,#47479);
#37946=AXIS2_PLACEMENT_3D('',#94920,#47480,#47481);
#37947=AXIS2_PLACEMENT_3D('',#94921,#47482,#47483);
#37948=AXIS2_PLACEMENT_3D('',#94922,#47484,#47485);
#37949=AXIS2_PLACEMENT_3D('',#94923,#47486,#47487);
#37950=AXIS2_PLACEMENT_3D('',#94924,#47488,#47489);
#37951=AXIS2_PLACEMENT_3D('',#94926,#47490,#47491);
#37952=AXIS2_PLACEMENT_3D('',#94927,#47492,#47493);
#37953=AXIS2_PLACEMENT_3D('',#94928,#47494,#47495);
#37954=AXIS2_PLACEMENT_3D('',#94930,#47496,#47497);
#37955=AXIS2_PLACEMENT_3D('',#94931,#47498,#47499);
#37956=AXIS2_PLACEMENT_3D('',#94969,#47500,#47501);
#37957=AXIS2_PLACEMENT_3D('',#94971,#47502,#47503);
#37958=AXIS2_PLACEMENT_3D('',#94972,#47504,#47505);
#37959=AXIS2_PLACEMENT_3D('',#95055,#47506,#47507);
#37960=AXIS2_PLACEMENT_3D('',#95058,#47509,#47510);
#37961=AXIS2_PLACEMENT_3D('',#95114,#47511,#47512);
#37962=AXIS2_PLACEMENT_3D('',#95158,#47513,#47514);
#37963=AXIS2_PLACEMENT_3D('',#95197,#47516,#47517);
#37964=AXIS2_PLACEMENT_3D('',#95241,#47518,#47519);
#37965=AXIS2_PLACEMENT_3D('',#95243,#47521,#47522);
#37966=AXIS2_PLACEMENT_3D('',#95244,#47523,#47524);
#37967=AXIS2_PLACEMENT_3D('',#95245,#47525,#47526);
#37968=AXIS2_PLACEMENT_3D('',#95246,#47527,#47528);
#37969=AXIS2_PLACEMENT_3D('',#95247,#47529,#47530);
#37970=AXIS2_PLACEMENT_3D('',#95249,#47531,#47532);
#37971=AXIS2_PLACEMENT_3D('',#95252,#47534,#47535);
#37972=AXIS2_PLACEMENT_3D('',#95253,#47536,#47537);
#37973=AXIS2_PLACEMENT_3D('',#95256,#47539,#47540);
#37974=AXIS2_PLACEMENT_3D('',#95257,#47541,#47542);
#37975=AXIS2_PLACEMENT_3D('',#95259,#47544,#47545);
#37976=AXIS2_PLACEMENT_3D('',#95261,#47546,#47547);
#37977=AXIS2_PLACEMENT_3D('',#95263,#47549,#47550);
#37978=AXIS2_PLACEMENT_3D('',#95264,#47551,#47552);
#37979=AXIS2_PLACEMENT_3D('',#95265,#47553,#47554);
#37980=AXIS2_PLACEMENT_3D('',#95267,#47555,#47556);
#37981=AXIS2_PLACEMENT_3D('',#95268,#47557,#47558);
#37982=AXIS2_PLACEMENT_3D('',#95269,#47559,#47560);
#37983=AXIS2_PLACEMENT_3D('',#95271,#47561,#47562);
#37984=AXIS2_PLACEMENT_3D('',#95273,#47564,#47565);
#37985=AXIS2_PLACEMENT_3D('',#95275,#47566,#47567);
#37986=AXIS2_PLACEMENT_3D('',#95276,#47568,#47569);
#37987=AXIS2_PLACEMENT_3D('',#95277,#47570,#47571);
#37988=AXIS2_PLACEMENT_3D('',#95279,#47573,#47574);
#37989=AXIS2_PLACEMENT_3D('',#95281,#47576,#47577);
#37990=AXIS2_PLACEMENT_3D('',#95284,#47579,#47580);
#37991=AXIS2_PLACEMENT_3D('',#95285,#47581,#47582);
#37992=AXIS2_PLACEMENT_3D('',#95286,#47583,#47584);
#37993=AXIS2_PLACEMENT_3D('',#95287,#47585,#47586);
#37994=AXIS2_PLACEMENT_3D('',#95291,#47588,#47589);
#37995=AXIS2_PLACEMENT_3D('',#95293,#47590,#47591);
#37996=AXIS2_PLACEMENT_3D('',#95295,#47592,#47593);
#37997=AXIS2_PLACEMENT_3D('',#95299,#47595,#47596);
#37998=AXIS2_PLACEMENT_3D('',#95300,#47597,#47598);
#37999=AXIS2_PLACEMENT_3D('',#95301,#47599,#47600);
#38000=AXIS2_PLACEMENT_3D('',#95304,#47601,#47602);
#38001=AXIS2_PLACEMENT_3D('',#95503,#47603,#47604);
#38002=AXIS2_PLACEMENT_3D('',#95540,#47605,#47606);
#38003=AXIS2_PLACEMENT_3D('',#95541,#47607,#47608);
#38004=AXIS2_PLACEMENT_3D('',#95543,#47609,#47610);
#38005=AXIS2_PLACEMENT_3D('',#95544,#47611,#47612);
#38006=AXIS2_PLACEMENT_3D('',#95545,#47613,#47614);
#38007=AXIS2_PLACEMENT_3D('',#95547,#47615,#47616);
#38008=AXIS2_PLACEMENT_3D('',#95548,#47617,#47618);
#38009=AXIS2_PLACEMENT_3D('',#95549,#47619,#47620);
#38010=AXIS2_PLACEMENT_3D('',#95551,#47621,#47622);
#38011=AXIS2_PLACEMENT_3D('',#95553,#47624,#47625);
#38012=AXIS2_PLACEMENT_3D('',#95555,#47626,#47627);
#38013=AXIS2_PLACEMENT_3D('',#95556,#47628,#47629);
#38014=AXIS2_PLACEMENT_3D('',#95557,#47630,#47631);
#38015=AXIS2_PLACEMENT_3D('',#95559,#47632,#47633);
#38016=AXIS2_PLACEMENT_3D('',#95560,#47634,#47635);
#38017=AXIS2_PLACEMENT_3D('',#95561,#47636,#47637);
#38018=AXIS2_PLACEMENT_3D('',#95563,#47638,#47639);
#38019=AXIS2_PLACEMENT_3D('',#95564,#47640,#47641);
#38020=AXIS2_PLACEMENT_3D('',#95602,#47642,#47643);
#38021=AXIS2_PLACEMENT_3D('',#95603,#47644,#47645);
#38022=AXIS2_PLACEMENT_3D('',#95689,#47646,#47647);
#38023=AXIS2_PLACEMENT_3D('',#95691,#47649,#47650);
#38024=AXIS2_PLACEMENT_3D('',#95695,#47652,#47653);
#38025=AXIS2_PLACEMENT_3D('',#95697,#47655,#47656);
#38026=AXIS2_PLACEMENT_3D('',#95700,#47658,#47659);
#38027=AXIS2_PLACEMENT_3D('',#95701,#47660,#47661);
#38028=AXIS2_PLACEMENT_3D('',#95702,#47662,#47663);
#38029=AXIS2_PLACEMENT_3D('',#95703,#47664,#47665);
#38030=AXIS2_PLACEMENT_3D('',#95706,#47667,#47668);
#38031=AXIS2_PLACEMENT_3D('',#95707,#47669,#47670);
#38032=AXIS2_PLACEMENT_3D('',#95710,#47672,#47673);
#38033=AXIS2_PLACEMENT_3D('',#95711,#47674,#47675);
#38034=AXIS2_PLACEMENT_3D('',#95714,#47677,#47678);
#38035=AXIS2_PLACEMENT_3D('',#95715,#47679,#47680);
#38036=AXIS2_PLACEMENT_3D('',#95719,#47683,#47684);
#38037=AXIS2_PLACEMENT_3D('',#95722,#47686,#47687);
#38038=AXIS2_PLACEMENT_3D('',#95723,#47688,#47689);
#38039=AXIS2_PLACEMENT_3D('',#95726,#47691,#47692);
#38040=AXIS2_PLACEMENT_3D('',#95727,#47693,#47694);
#38041=AXIS2_PLACEMENT_3D('',#95730,#47696,#47697);
#38042=AXIS2_PLACEMENT_3D('',#95731,#47698,#47699);
#38043=AXIS2_PLACEMENT_3D('',#95735,#47702,#47703);
#38044=AXIS2_PLACEMENT_3D('',#95736,#47704,#47705);
#38045=AXIS2_PLACEMENT_3D('',#95737,#47706,#47707);
#38046=AXIS2_PLACEMENT_3D('',#95739,#47708,#47709);
#38047=AXIS2_PLACEMENT_3D('',#95740,#47710,#47711);
#38048=AXIS2_PLACEMENT_3D('',#95741,#47712,#47713);
#38049=AXIS2_PLACEMENT_3D('',#95743,#47714,#47715);
#38050=AXIS2_PLACEMENT_3D('',#95744,#47716,#47717);
#38051=AXIS2_PLACEMENT_3D('',#95745,#47718,#47719);
#38052=AXIS2_PLACEMENT_3D('',#95747,#47720,#47721);
#38053=AXIS2_PLACEMENT_3D('',#95748,#47722,#47723);
#38054=AXIS2_PLACEMENT_3D('',#95749,#47724,#47725);
#38055=AXIS2_PLACEMENT_3D('',#95751,#47726,#47727);
#38056=AXIS2_PLACEMENT_3D('',#95752,#47728,#47729);
#38057=AXIS2_PLACEMENT_3D('',#95753,#47730,#47731);
#38058=AXIS2_PLACEMENT_3D('',#95754,#47732,#47733);
#38059=AXIS2_PLACEMENT_3D('',#95755,#47734,#47735);
#38060=AXIS2_PLACEMENT_3D('',#95757,#47736,#47737);
#38061=AXIS2_PLACEMENT_3D('',#95758,#47738,#47739);
#38062=AXIS2_PLACEMENT_3D('',#95759,#47740,#47741);
#38063=AXIS2_PLACEMENT_3D('',#95761,#47742,#47743);
#38064=AXIS2_PLACEMENT_3D('',#95762,#47744,#47745);
#38065=AXIS2_PLACEMENT_3D('',#95763,#47746,#47747);
#38066=AXIS2_PLACEMENT_3D('',#95764,#47748,#47749);
#38067=AXIS2_PLACEMENT_3D('',#95765,#47750,#47751);
#38068=AXIS2_PLACEMENT_3D('',#95767,#47752,#47753);
#38069=AXIS2_PLACEMENT_3D('',#95769,#47755,#47756);
#38070=AXIS2_PLACEMENT_3D('',#95770,#47757,#47758);
#38071=AXIS2_PLACEMENT_3D('',#95771,#47759,#47760);
#38072=AXIS2_PLACEMENT_3D('',#95773,#47761,#47762);
#38073=AXIS2_PLACEMENT_3D('',#95774,#47763,#47764);
#38074=AXIS2_PLACEMENT_3D('',#95775,#47765,#47766);
#38075=AXIS2_PLACEMENT_3D('',#95776,#47767,#47768);
#38076=AXIS2_PLACEMENT_3D('',#95777,#47769,#47770);
#38077=AXIS2_PLACEMENT_3D('',#95779,#47772,#47773);
#38078=AXIS2_PLACEMENT_3D('',#95781,#47774,#47775);
#38079=AXIS2_PLACEMENT_3D('',#95783,#47777,#47778);
#38080=AXIS2_PLACEMENT_3D('',#95785,#47779,#47780);
#38081=AXIS2_PLACEMENT_3D('',#95786,#47781,#47782);
#38082=AXIS2_PLACEMENT_3D('',#95787,#47783,#47784);
#38083=AXIS2_PLACEMENT_3D('',#95789,#47785,#47786);
#38084=AXIS2_PLACEMENT_3D('',#95790,#47787,#47788);
#38085=AXIS2_PLACEMENT_3D('',#95791,#47789,#47790);
#38086=AXIS2_PLACEMENT_3D('',#95792,#47791,#47792);
#38087=AXIS2_PLACEMENT_3D('',#95793,#47793,#47794);
#44415=DIRECTION('axis',(0.,0.,1.));
#44416=DIRECTION('refdir',(1.,0.,0.));
#44417=DIRECTION('center_axis',(-1.224646799149E-16,-1.,-1.07595286226434E-28));
#44418=DIRECTION('ref_axis',(-0.67889125729581,8.31402005216767E-17,0.734238830876789));
#44419=DIRECTION('center_axis',(1.22464679915E-16,1.,1.23259516441E-32));
#44420=DIRECTION('ref_axis',(1.,-1.22464679915E-16,-1.50949372274247E-48));
#44421=DIRECTION('',(-2.85587916301E-16,-1.,0.));
#44422=DIRECTION('center_axis',(1.22464679915E-16,1.,0.));
#44423=DIRECTION('ref_axis',(1.,-1.22464679915E-16,0.));
#44424=DIRECTION('',(0.,-1.,0.));
#44425=DIRECTION('center_axis',(1.22464679914912E-16,1.,-1.26181562037188E-28));
#44426=DIRECTION('ref_axis',(0.572811155566786,-7.01491348180737E-17,0.819687367267694));
#44427=DIRECTION('',(0.,-1.,0.));
#44428=DIRECTION('center_axis',(-1.22464679915E-16,-1.,-1.23259516441E-32));
#44429=DIRECTION('ref_axis',(1.,-1.22464679915E-16,-1.50949372274247E-48));
#44430=DIRECTION('center_axis',(-1.22464679915E-16,-1.,-2.46519032882E-32));
#44431=DIRECTION('ref_axis',(1.,-1.22464679915E-16,-3.01898744548495E-48));
#44432=DIRECTION('center_axis',(-0.641370372756966,-0.046782002687993,-0.765803818986358));
#44433=DIRECTION('ref_axis',(0.766534261679224,-0.0816131667450425,-0.636996480905298));
#44434=DIRECTION('center_axis',(-1.22464679914824E-16,-1.,2.07760762711853E-28));
#44435=DIRECTION('ref_axis',(-0.646318112561793,7.91511407778746E-17,-0.763068081742751));
#44436=DIRECTION('',(0.,-1.,0.));
#44437=DIRECTION('center_axis',(1.22464679915E-16,1.,6.16297582204E-33));
#44438=DIRECTION('ref_axis',(1.,-1.22464679915E-16,-7.54746861370013E-49));
#44439=DIRECTION('center_axis',(1.22464679914844E-16,1.,-1.36792384183344E-28));
#44440=DIRECTION('ref_axis',(0.751089446707,-9.19819286783E-17,0.660200456713999));
#44441=DIRECTION('',(0.,1.,0.));
#44442=DIRECTION('center_axis',(-1.22464679915E-16,-1.,-1.23259516441E-32));
#44443=DIRECTION('ref_axis',(1.,-1.22464679915E-16,-1.50949372274247E-48));
#44444=DIRECTION('',(2.85587916301E-16,1.,0.));
#44445=DIRECTION('center_axis',(1.2246467991496E-16,1.,-1.2428667907779E-29));
#44446=DIRECTION('ref_axis',(0.953995514765253,-1.16830755356031E-16,0.299820876204076));
#44447=DIRECTION('',(0.,1.,0.));
#44448=DIRECTION('center_axis',(-1.22464679915E-16,-1.,0.));
#44449=DIRECTION('ref_axis',(1.,-1.22464679915E-16,0.));
#44450=DIRECTION('',(2.85587916301E-16,1.,0.));
#44451=DIRECTION('center_axis',(0.,1.,0.));
#44452=DIRECTION('ref_axis',(0.678891257321093,0.,-0.734238830853412));
#44453=DIRECTION('center_axis',(-0.678891257295808,8.31402005216763E-17,
0.734238830876792));
#44454=DIRECTION('ref_axis',(1.22464679914784E-16,1.,1.83887638005312E-34));
#44455=DIRECTION('',(0.,-1.,0.));
#44456=DIRECTION('',(0.734238830876791,0.,0.678891257295807));
#44457=DIRECTION('',(-0.734238830876791,0.,-0.678891257295807));
#44458=DIRECTION('center_axis',(-1.224646799149E-16,-1.,-1.07595286226434E-28));
#44459=DIRECTION('ref_axis',(-0.67889125729581,8.31402005216767E-17,0.734238830876789));
#44460=DIRECTION('center_axis',(-1.22464679915E-16,-1.,0.));
#44461=DIRECTION('ref_axis',(1.,-1.22464679915E-16,0.));
#44462=DIRECTION('',(0.,-1.,0.));
#44463=DIRECTION('center_axis',(1.22464679915E-16,1.,0.));
#44464=DIRECTION('ref_axis',(1.,-1.22464679915E-16,0.));
#44465=DIRECTION('center_axis',(1.22464679914912E-16,1.,-1.26181562037188E-28));
#44466=DIRECTION('ref_axis',(0.572811155566786,-7.01491348180737E-17,0.819687367267694));
#44467=DIRECTION('',(0.,-1.,0.));
#44468=DIRECTION('center_axis',(-1.22464679915E-16,-1.,-1.23259516441E-32));
#44469=DIRECTION('ref_axis',(1.,-1.22464679915E-16,-1.50949372274247E-48));
#44470=DIRECTION('center_axis',(1.22464679915E-16,1.,0.));
#44471=DIRECTION('ref_axis',(1.,-1.22464679915E-16,0.));
#44472=DIRECTION('center_axis',(1.224646799149E-16,1.,1.07586726537792E-28));
#44473=DIRECTION('ref_axis',(0.67889125729581,-8.31402005216767E-17,-0.734238830876789));
#44474=DIRECTION('center_axis',(-1.22464679915E-16,-1.,0.));
#44475=DIRECTION('ref_axis',(1.,-1.22464679915E-16,0.));
#44476=DIRECTION('',(0.,-1.,0.));
#44477=DIRECTION('',(0.,-1.,0.));
#44478=DIRECTION('center_axis',(1.22464679915E-16,1.,1.23259516441E-32));
#44479=DIRECTION('ref_axis',(1.,-1.22464679915E-16,-1.50949372274247E-48));
#44480=DIRECTION('center_axis',(-0.678891257295808,8.31402005216763E-17,
0.734238830876792));
#44481=DIRECTION('ref_axis',(1.22464679914784E-16,1.,1.83887638005312E-34));
#44482=DIRECTION('',(0.,1.,0.));
#44483=DIRECTION('',(-0.734238830876791,0.,-0.678891257295807));
#44484=DIRECTION('center_axis',(-0.678891258039564,-8.05580512386835E-9,
0.7342388301891));
#44485=DIRECTION('ref_axis',(1.90502136153082E-5,-0.999999999663608,1.76032200345041E-5));
#44486=DIRECTION('',(0.734238830876791,0.,0.678891257295807));
#44487=DIRECTION('center_axis',(0.734238830876792,-8.99183234042744E-17,
0.678891257295808));
#44488=DIRECTION('ref_axis',(-0.678891257295807,-3.46311205996404E-31,0.734238830876791));
#44489=DIRECTION('',(0.734238830876791,0.,0.678891257295807));
#44490=DIRECTION('center_axis',(-0.734238830876792,8.99183234042744E-17,
-0.678891257295808));
#44491=DIRECTION('ref_axis',(0.678891257295807,3.46311205996404E-31,-0.734238830876791));
#44492=DIRECTION('',(0.734238830876791,0.,0.678891257295807));
#44493=DIRECTION('center_axis',(0.,0.,1.));
#44494=DIRECTION('ref_axis',(1.,0.,0.));
#44495=DIRECTION('center_axis',(0.803996045360697,-9.84611183477626E-17,
-0.594634643326775));
#44496=DIRECTION('ref_axis',(0.594634643326775,4.97302608069436E-32,0.803996045360697));
#44497=DIRECTION('center_axis',(-7.91623497736024E-17,-1.,5.85483919904324E-17));
#44498=DIRECTION('ref_axis',(0.594634643326775,0.,0.803996045360696));
#44499=DIRECTION('center_axis',(-1.22464679915E-16,-1.,-5.47382212627E-48));
#44500=DIRECTION('ref_axis',(1.,-1.22464679915E-16,-6.703498746053E-64));
#44501=DIRECTION('center_axis',(0.763068081742753,-9.34488883837698E-17,
-0.646318112561791));
#44502=DIRECTION('ref_axis',(0.646318112561791,2.50438493602067E-31,0.763068081742753));
#44503=DIRECTION('center_axis',(1.,0.,0.));
#44504=DIRECTION('ref_axis',(0.,-1.,0.));
#44505=DIRECTION('center_axis',(0.734238830876792,-8.99183234042744E-17,
0.678891257295808));
#44506=DIRECTION('ref_axis',(0.678891257295807,3.46311205996404E-31,-0.734238830876791));
#44507=DIRECTION('center_axis',(-0.734238830876792,8.99183234042744E-17,
-0.678891257295808));
#44508=DIRECTION('ref_axis',(0.678891257295807,3.46311205996404E-31,-0.734238830876791));
#44509=DIRECTION('',(-0.734238830876791,0.,-0.678891257295807));
#44510=DIRECTION('',(-0.734238830876791,0.,-0.678891257295807));
#44511=DIRECTION('center_axis',(0.734238830876792,-8.99183234042744E-17,
0.678891257295808));
#44512=DIRECTION('ref_axis',(0.678891257295807,3.46311205996404E-31,-0.734238830876791));
#44513=DIRECTION('center_axis',(-6.60215246509141E-17,-1.,-6.10447636300053E-17));
#44514=DIRECTION('ref_axis',(-0.678891257295808,0.,0.734238830876791));
#44515=DIRECTION('center_axis',(-1.22464679915E-16,-1.,-5.47382212627E-48));
#44516=DIRECTION('ref_axis',(1.,-1.22464679915E-16,-6.703498746053E-64));
#44517=DIRECTION('center_axis',(-1.22464679915E-16,-1.,-1.23259516441E-32));
#44518=DIRECTION('ref_axis',(1.,-1.22464679915E-16,-1.50949372274247E-48));
#44519=DIRECTION('center_axis',(0.732027802944257,-8.96475505763315E-17,
-0.68127475787424));
#44520=DIRECTION('ref_axis',(0.68127475787424,-1.91888914560603E-31,0.732027802944257));
#44521=DIRECTION('center_axis',(-6.56244994878123E-17,-1.,6.10746133129891E-17));
#44522=DIRECTION('ref_axis',(0.681274757874239,0.,0.732027802944258));
#44523=DIRECTION('center_axis',(-1.22464679915E-16,-1.,-5.47382212627E-48));
#44524=DIRECTION('ref_axis',(1.,-1.22464679915E-16,5.9677926224237E-64));
#44525=DIRECTION('center_axis',(-1.22464679915E-16,-1.,-5.47382212627E-48));
#44526=DIRECTION('ref_axis',(1.,-1.22464679915E-16,6.22660996643423E-64));
#44527=DIRECTION('center_axis',(0.660200456714,-8.0851237611E-17,-0.751089446706999));
#44528=DIRECTION('ref_axis',(0.751089446706999,6.24086217807948E-32,0.660200456714));
#44529=DIRECTION('center_axis',(-5.33780239968174E-17,-1.,6.0726511322985E-17));
#44530=DIRECTION('ref_axis',(0.751089446706998,0.,0.660200456714001));
#44531=DIRECTION('center_axis',(-1.22464679915E-16,-1.,-5.47382212627E-48));
#44532=DIRECTION('ref_axis',(1.,-1.22464679915E-16,-6.703498746053E-64));
#44533=DIRECTION('center_axis',(0.315563048033822,-3.86453276703782E-17,
-0.948904612021463));
#44534=DIRECTION('ref_axis',(0.948904612021463,7.52823903108453E-32,0.315563048033822));
#44535=DIRECTION('center_axis',(-1.21950373919573E-17,-1.,3.66707296595837E-17));
#44536=DIRECTION('ref_axis',(0.948904612021463,0.,0.315563048033822));
#44537=DIRECTION('center_axis',(-1.22464679915E-16,-1.,-5.47382212627E-48));
#44538=DIRECTION('ref_axis',(1.,-1.22464679915E-16,5.9677926224237E-64));
#44539=DIRECTION('center_axis',(-1.22464679915E-16,-1.,-5.47382212627E-48));
#44540=DIRECTION('ref_axis',(1.,-1.22464679915E-16,6.22660996643423E-64));
#44541=DIRECTION('center_axis',(0.299820876204079,-3.67174676361097E-17,
-0.953995514765252));
#44542=DIRECTION('ref_axis',(0.953995514765252,-6.3869078326472E-32,0.299820876204079));
#44543=DIRECTION('center_axis',(-1.10086633186706E-17,-1.,3.5028299438442E-17));
#44544=DIRECTION('ref_axis',(0.953995514765252,0.,0.299820876204079));
#44545=DIRECTION('center_axis',(-1.22464679915E-16,-1.,-5.47382212627E-48));
#44546=DIRECTION('ref_axis',(1.,-1.22464679915E-16,-6.703498746053E-64));
#44547=DIRECTION('center_axis',(-0.734238830876792,8.99183234042744E-17,
-0.678891257295808));
#44548=DIRECTION('ref_axis',(0.678891257295807,3.46311205996404E-31,-0.734238830876791));
#44549=DIRECTION('center_axis',(0.734238830876792,-8.99183234042744E-17,
0.678891257295808));
#44550=DIRECTION('ref_axis',(-0.678891257295807,-3.46311205996404E-31,0.734238830876791));
#44551=DIRECTION('',(0.734238830876791,0.,0.678891257295807));
#44552=DIRECTION('center_axis',(-0.734238830876792,8.99183234042744E-17,
-0.678891257295808));
#44553=DIRECTION('ref_axis',(0.678891257295807,3.46311205996404E-31,-0.734238830876791));
#44554=DIRECTION('center_axis',(0.,0.,1.));
#44555=DIRECTION('ref_axis',(1.,0.,0.));
#44556=DIRECTION('center_axis',(0.613815420645987,-7.51707090161983E-17,
-0.789449573675983));
#44557=DIRECTION('ref_axis',(0.789449573675983,7.34020703099417E-32,0.613815420645987));
#44558=DIRECTION('center_axis',(-4.61409403750984E-17,-1.,5.93434841858408E-17));
#44559=DIRECTION('ref_axis',(0.789449573675983,0.,0.613815420645986));
#44560=DIRECTION('center_axis',(-1.22464679915E-16,-1.,-5.47382212627E-48));
#44561=DIRECTION('ref_axis',(1.,-1.22464679915E-16,-6.703498746053E-64));
#44562=DIRECTION('center_axis',(0.560738119471071,-6.86706143170087E-17,
-0.827993213361104));
#44563=DIRECTION('ref_axis',(0.827993213361104,-2.38131063616686E-32,0.560738119471071));
#44564=DIRECTION('center_axis',(1.,0.,0.));
#44565=DIRECTION('ref_axis',(0.,-1.,0.));
#44566=DIRECTION('center_axis',(0.734238830876792,-8.99183234042744E-17,
0.678891257295808));
#44567=DIRECTION('ref_axis',(0.678891257295807,3.46311205996404E-31,-0.734238830876791));
#44568=DIRECTION('center_axis',(0.734238830876792,-8.99183234044499E-17,
0.678891257295808));
#44569=DIRECTION('ref_axis',(-6.60215246508846E-17,-1.,-6.1044763629978E-17));
#44570=DIRECTION('',(-0.734238830876791,0.,-0.678891257295807));
#44571=DIRECTION('center_axis',(-1.22464679915E-16,-1.,-5.47382212627E-48));
#44572=DIRECTION('ref_axis',(-1.,1.22464679915E-16,0.));
#44573=DIRECTION('center_axis',(1.22464679915E-16,1.,1.23259516441E-32));
#44574=DIRECTION('ref_axis',(1.,-1.22464679915E-16,-1.50949372274247E-48));
#44575=DIRECTION('center_axis',(1.22464679915E-16,1.,0.));
#44576=DIRECTION('ref_axis',(1.,-1.22464679915E-16,0.));
#44577=DIRECTION('center_axis',(1.,-1.22464679915E-16,6.12323399574E-17));
#44578=DIRECTION('ref_axis',(-1.22464679915E-16,-1.,-6.67366607695787E-50));
#44579=DIRECTION('',(-1.26882631386E-16,-1.,0.));
#44580=DIRECTION('',(1.75377892382E-16,0.,-1.));
#44581=DIRECTION('',(-1.26882631386E-16,-1.,0.));
#44582=DIRECTION('',(2.21800239814E-16,0.,-1.));
#44583=DIRECTION('',(-1.34875042533E-16,-1.,0.));
#44584=DIRECTION('',(2.5585870064E-16,0.,-1.));
#44585=DIRECTION('center_axis',(-1.22464679915E-16,-1.,-7.60253073092891E-48));
#44586=DIRECTION('ref_axis',(1.,-1.22464679915E-16,-9.3104149250716E-64));
#44587=DIRECTION('center_axis',(1.22464679915E-16,1.,0.));
#44588=DIRECTION('ref_axis',(1.,-1.22464679915E-16,0.));
#44589=DIRECTION('',(-1.42793958151E-16,-1.,0.));
#44590=DIRECTION('center_axis',(1.22464679915E-16,1.,6.16297582204E-33));
#44591=DIRECTION('ref_axis',(1.,-1.22464679915E-16,-7.54746861370013E-49));
#44592=DIRECTION('center_axis',(1.22464679914955E-16,1.,8.72911003161552E-29));
#44593=DIRECTION('ref_axis',(0.457271150163836,-5.59995650390798E-17,-0.889327327381681));
#44594=DIRECTION('',(-1.26882631386E-16,-1.,0.));
#44595=DIRECTION('center_axis',(-1.22464679915E-16,-1.,0.));
#44596=DIRECTION('ref_axis',(1.,-1.22464679915E-16,0.));
#44597=DIRECTION('center_axis',(-1.22464679915E-16,-1.,6.16297582204E-33));
#44598=DIRECTION('ref_axis',(1.,-1.22464679915E-16,7.54746861370012E-49));
#44599=DIRECTION('center_axis',(1.22464679915E-16,1.,0.));
#44600=DIRECTION('ref_axis',(-1.,1.22464679915E-16,-2.89120579329468E-15));
#44601=DIRECTION('center_axis',(1.22464679915E-16,1.,0.));
#44602=DIRECTION('ref_axis',(1.,-1.22464679915E-16,0.));
#44603=DIRECTION('',(-2.0185873175E-16,-1.,0.));
#44604=DIRECTION('center_axis',(1.22464679915E-16,1.,6.16297582204E-33));
#44605=DIRECTION('ref_axis',(1.,-1.22464679915E-16,-7.54746861370013E-49));
#44606=DIRECTION('center_axis',(1.,-1.22464679915E-16,6.12323399574E-17));
#44607=DIRECTION('ref_axis',(-1.22464679915E-16,-1.,-6.67366607695787E-50));
#44608=DIRECTION('',(-2.58629566281E-16,0.,1.));
#44609=DIRECTION('',(1.26882631386E-16,1.,0.));
#44610=DIRECTION('',(-1.75377892382E-16,0.,1.));
#44611=DIRECTION('center_axis',(-1.22464679914969E-16,-1.,-8.28235472972929E-29));
#44612=DIRECTION('ref_axis',(0.345424032932988,-4.23022436279984E-17,-0.938446715307966));
#44613=DIRECTION('',(1.42793958151E-16,1.,0.));
#44614=DIRECTION('center_axis',(-1.22464679915E-16,-1.,0.));
#44615=DIRECTION('ref_axis',(1.,-1.22464679915E-16,0.));
#44616=DIRECTION('center_axis',(1.22464679915E-16,1.,6.16297582203999E-33));
#44617=DIRECTION('ref_axis',(1.,-1.22464679915E-16,-7.54746861370011E-49));
#44618=DIRECTION('center_axis',(0.,-1.,0.));
#44619=DIRECTION('ref_axis',(1.,0.,3.70074341541721E-15));
#44620=DIRECTION('center_axis',(1.22464679915E-16,1.,-6.16297582204E-33));
#44621=DIRECTION('ref_axis',(1.,-1.22464679915E-16,7.54746861370013E-49));
#44622=DIRECTION('',(0.,-1.,0.));
#44623=DIRECTION('center_axis',(2.17357452795E-16,-2.66186108837E-32,-1.));
#44624=DIRECTION('ref_axis',(1.,5.7857534586223E-48,2.17357452795E-16));
#44625=DIRECTION('',(2.0973706922E-16,0.,-1.));
#44626=DIRECTION('center_axis',(-4.62592926927E-17,5.6651294727E-33,1.));
#44627=DIRECTION('ref_axis',(1.,2.62064882419671E-49,4.62592926927E-17));
#44628=DIRECTION('center_axis',(-2.77555756156E-16,3.39907768362E-32,1.));
#44629=DIRECTION('ref_axis',(1.,9.43433576710134E-48,2.77555756156E-16));
#44630=DIRECTION('center_axis',(1.,0.,0.));
#44631=DIRECTION('ref_axis',(0.,-1.,0.));
#44632=DIRECTION('center_axis',(-0.904759192693671,1.1080104493296E-16,
-0.425923471102845));
#44633=DIRECTION('ref_axis',(0.425923471102845,3.65487816993661E-32,-0.904759192693671));
#44634=DIRECTION('center_axis',(-1.00248263963544E-16,-1.,-4.71927656598494E-17));
#44635=DIRECTION('ref_axis',(0.425923471102846,0.,-0.904759192693671));
#44636=DIRECTION('center_axis',(-1.22464679915E-16,-1.,-5.47382212627E-48));
#44637=DIRECTION('ref_axis',(1.,-1.22464679915E-16,-6.703498746053E-64));
#44638=DIRECTION('center_axis',(-0.916786704663777,1.12273990336973E-16,
-0.399377187820903));
#44639=DIRECTION('ref_axis',(0.399377187820903,3.93858763528754E-32,-0.916786704663777));
#44640=DIRECTION('center_axis',(0.,0.,1.));
#44641=DIRECTION('ref_axis',(1.,0.,0.));
#44642=DIRECTION('center_axis',(2.17357452795E-16,-2.66186108837E-32,-1.));
#44643=DIRECTION('ref_axis',(1.,5.7857534586223E-48,2.17357452795E-16));
#44644=DIRECTION('center_axis',(2.17357452795E-16,-2.66186108836821E-32,
-1.));
#44645=DIRECTION('ref_axis',(-5.78575345861839E-48,-1.,2.66186108836821E-32));
#44646=DIRECTION('',(0.,0.,1.));
#44647=DIRECTION('center_axis',(2.17357452795E-16,-2.66186108837E-32,-1.));
#44648=DIRECTION('ref_axis',(1.,5.7857534586223E-48,2.17357452795E-16));
#44649=DIRECTION('center_axis',(-1.07341775839004E-45,-1.,3.62568286252829E-31));
#44650=DIRECTION('ref_axis',(1.,0.,3.94745964311167E-15));
#44651=DIRECTION('center_axis',(-1.22464679915E-16,-1.,-5.47382212627E-48));
#44652=DIRECTION('ref_axis',(1.,-1.22464679915E-16,-6.703498746053E-64));
#44653=DIRECTION('center_axis',(-0.938446715307966,1.14926576606996E-16,
-0.345424032932987));
#44654=DIRECTION('ref_axis',(0.345424032932987,5.96953449650393E-32,-0.938446715307966));
#44655=DIRECTION('center_axis',(-1.07852468318872E-16,-1.,-3.96984015829353E-17));
#44656=DIRECTION('ref_axis',(0.345424032932988,0.,-0.938446715307966));
#44657=DIRECTION('center_axis',(-1.22464679915E-16,-1.,-5.47382212627E-48));
#44658=DIRECTION('ref_axis',(1.,-1.22464679915E-16,5.9677926224237E-64));
#44659=DIRECTION('center_axis',(-1.22464679915E-16,-1.,-5.47382212627E-48));
#44660=DIRECTION('ref_axis',(1.,-1.22464679915E-16,6.22660996643423E-64));
#44661=DIRECTION('center_axis',(0.,0.,1.));
#44662=DIRECTION('ref_axis',(1.,0.,0.));
#44663=DIRECTION('center_axis',(0.927477365469186,-1.13583218690023E-16,
0.373879307454075));
#44664=DIRECTION('ref_axis',(0.373879307454075,-5.54912062383212E-32,-0.927477365469186));
#44665=DIRECTION('center_axis',(-1.0534586443266E-16,-1.,-4.2466415142443E-17));
#44666=DIRECTION('ref_axis',(0.373879307454075,0.,-0.927477365469186));
#44667=DIRECTION('center_axis',(1.22464679915E-16,1.,5.47382212627E-48));
#44668=DIRECTION('ref_axis',(1.,-1.22464679915E-16,5.02845536814161E-64));
#44669=DIRECTION('center_axis',(1.22464679915E-16,1.,5.47382212627E-48));
#44670=DIRECTION('ref_axis',(1.,-1.22464679915E-16,5.24998673990483E-64));
#44671=DIRECTION('center_axis',(0.687199008140201,-8.41576065696246E-17,
-0.726469216974212));
#44672=DIRECTION('ref_axis',(-0.726469216974212,-1.50838013754883E-32,-0.687199008140201));
#44673=DIRECTION('',(-0.687199008140201,0.,0.726469216974212));
#44674=DIRECTION('',(-0.687199008140201,0.,0.726469216974212));
#44675=DIRECTION('center_axis',(1.68490994230906E-17,1.,-4.21844451941189E-17));
#44676=DIRECTION('ref_axis',(-0.928663912412966,0.,-0.370922279974987));
#44677=DIRECTION('center_axis',(-1.22464679915E-16,-1.,-5.47382212627E-48));
#44678=DIRECTION('ref_axis',(1.,-1.22464679915E-16,-6.703498746053E-64));
#44679=DIRECTION('center_axis',(-1.22464679915E-16,-1.,-5.47382212627E-48));
#44680=DIRECTION('ref_axis',(1.,-1.22464679915E-16,-6.703498746053E-64));
#44681=DIRECTION('center_axis',(-0.656401557315033,6.93091019571431E-12,
-0.754411688373397));
#44682=DIRECTION('ref_axis',(-9.95129904405703E-12,1.,1.78468351208498E-11));
#44683=DIRECTION('center_axis',(1.,-1.22464679915E-16,6.12323399574E-17));
#44684=DIRECTION('ref_axis',(1.22464679915E-16,1.,7.49879891332945E-33));
#44685=DIRECTION('',(1.,0.,2.21592204945E-16));
#44686=DIRECTION('',(1.,0.,1.4772813663E-16));
#44687=DIRECTION('center_axis',(-1.,0.,0.));
#44688=DIRECTION('ref_axis',(0.,1.,-3.70074341541716E-15));
#44689=DIRECTION('center_axis',(2.41898181523141E-16,1.,1.1741867647411E-17));
#44690=DIRECTION('ref_axis',(-0.99520202856178,2.41886400693281E-16,-0.0978413120645785));
#44691=DIRECTION('center_axis',(1.22464679915E-16,1.,5.47382212627E-48));
#44692=DIRECTION('ref_axis',(1.,-1.22464679915E-16,6.22660996643423E-64));
#44693=DIRECTION('center_axis',(1.22464679915E-16,1.,5.47382212627E-48));
#44694=DIRECTION('ref_axis',(1.,-1.22464679915E-16,6.49622071350503E-64));
#44695=DIRECTION('center_axis',(-0.668126653627122,3.01884491205213E-12,
-0.744047562130959));
#44696=DIRECTION('ref_axis',(0.744047562130959,1.48029736616688E-14,-0.668126653627122));
#44697=DIRECTION('center_axis',(0.,1.,0.));
#44698=DIRECTION('ref_axis',(0.0129687405446048,0.,-0.999915902348136));
#44699=DIRECTION('center_axis',(1.22464679915E-16,1.,0.));
#44700=DIRECTION('ref_axis',(1.,-1.22464679915E-16,0.));
#44701=DIRECTION('center_axis',(-0.726469216974212,8.89668201247259E-17,
-0.687199008140201));
#44702=DIRECTION('ref_axis',(-0.687199008140201,2.45619021304035E-33,0.726469216974212));
#44703=DIRECTION('',(-0.687199008140201,0.,0.726469216974212));
#44704=DIRECTION('',(0.,-1.,0.));
#44705=DIRECTION('',(0.,1.,0.));
#44706=DIRECTION('center_axis',(0.,0.,1.));
#44707=DIRECTION('ref_axis',(1.,0.,0.));
#44708=DIRECTION('center_axis',(-1.22464679915E-16,-1.,0.));
#44709=DIRECTION('ref_axis',(1.,-1.22464679915E-16,0.));
#44710=DIRECTION('center_axis',(1.22464679914998E-16,1.,-1.73663083545565E-29));
#44711=DIRECTION('ref_axis',(0.095298509688002,-1.16707014853003E-17,0.99544874004202));
#44712=DIRECTION('center_axis',(-1.22464679915E-16,-1.,0.));
#44713=DIRECTION('ref_axis',(1.,-1.22464679915E-16,0.));
#44714=DIRECTION('',(0.,1.,0.));
#44715=DIRECTION('',(0.,1.,0.));
#44716=DIRECTION('center_axis',(0.,0.,1.));
#44717=DIRECTION('ref_axis',(1.,0.,0.));
#44718=DIRECTION('center_axis',(-1.22464679915E-16,-1.,3.08148791102E-33));
#44719=DIRECTION('ref_axis',(1.,-1.22464679915E-16,3.77373430685006E-49));
#44720=DIRECTION('center_axis',(-2.17357452795E-16,2.66186108837E-32,1.));
#44721=DIRECTION('ref_axis',(1.,2.56447231488414E-65,2.17357452795E-16));
#44722=DIRECTION('',(0.,1.,0.));
#44723=DIRECTION('',(0.,-1.,0.));
#44724=DIRECTION('',(1.,0.,4.75520106567E-17));
#44725=DIRECTION('center_axis',(0.,1.,0.));
#44726=DIRECTION('ref_axis',(0.79266275948672,0.,0.609660356036784));
#44727=DIRECTION('center_axis',(1.22464679915E-16,1.,0.));
#44728=DIRECTION('ref_axis',(1.,-1.22464679915E-16,0.));
#44729=DIRECTION('center_axis',(1.22464679914586E-16,1.,-1.3947821589454E-28));
#44730=DIRECTION('ref_axis',(0.947590338356885,-1.16046347476986E-16,0.319487950715961));
#44731=DIRECTION('',(0.,-1.,0.));
#44732=DIRECTION('',(0.,-1.,0.));
#44733=DIRECTION('center_axis',(1.22464679915E-16,1.,0.));
#44734=DIRECTION('ref_axis',(1.,-1.22464679915E-16,0.));
#44735=DIRECTION('center_axis',(1.22464679914811E-16,1.,1.69670148256195E-28));
#44736=DIRECTION('ref_axis',(0.744047562132924,-9.11195465378906E-17,-0.668126653624934));
#44737=DIRECTION('center_axis',(1.22464679915E-16,1.,0.));
#44738=DIRECTION('ref_axis',(1.,-1.22464679915E-16,0.));
#44739=DIRECTION('center_axis',(0.687199008140201,-8.41576065696246E-17,
-0.726469216974212));
#44740=DIRECTION('ref_axis',(0.726469216974212,1.50838013754883E-32,0.687199008140201));
#44741=DIRECTION('center_axis',(0.687199008140201,-8.41576065696246E-17,
-0.726469216974212));
#44742=DIRECTION('ref_axis',(0.726469216974212,1.50838013754883E-32,0.687199008140201));
#44743=DIRECTION('',(-0.687199008140201,0.,0.726469216974212));
#44744=DIRECTION('center_axis',(0.687199008140201,-8.41576065696246E-17,
-0.726469216974212));
#44745=DIRECTION('ref_axis',(0.726469216974212,1.50838013754883E-32,0.687199008140201));
#44746=DIRECTION('center_axis',(1.22464679914912E-16,1.,-8.35682402091226E-29));
#44747=DIRECTION('ref_axis',(-0.726469216974212,8.89668201247259E-17,-0.687199008140201));
#44748=DIRECTION('center_axis',(1.22464679915E-16,1.,1.23259516441E-32));
#44749=DIRECTION('ref_axis',(1.,-1.22464679915E-16,-1.50949372274247E-48));
#44750=DIRECTION('center_axis',(-2.81810938552877E-18,-1.,-1.83623833789471E-17));
#44751=DIRECTION('ref_axis',(0.988427230781696,0.,-0.151695779272953));
#44752=DIRECTION('center_axis',(-0.151695779272953,1.85773750529943E-17,
-0.988427230781696));
#44753=DIRECTION('ref_axis',(0.988427230781695,3.4608594993322E-33,-0.151695779272953));
#44754=DIRECTION('center_axis',(-1.22464679915E-16,-1.,-5.47382212627E-48));
#44755=DIRECTION('ref_axis',(1.,-1.22464679915E-16,-6.703498746053E-64));
#44756=DIRECTION('center_axis',(-0.656401557320037,8.03860066128046E-17,
-0.754411688369043));
#44757=DIRECTION('ref_axis',(0.754411688369043,3.51059188021851E-32,-0.656401557320037));
#44758=DIRECTION('center_axis',(-1.22464679915E-16,-1.,3.04712758348345E-33));
#44759=DIRECTION('ref_axis',(3.73165504171468E-49,3.04712758348345E-33,
1.));
#44760=DIRECTION('center_axis',(1.22464679915E-16,1.,0.));
#44761=DIRECTION('ref_axis',(1.,-1.22464679915E-16,0.));
#44762=DIRECTION('center_axis',(1.,-1.22464679915E-16,6.12323399574E-17));
#44763=DIRECTION('ref_axis',(-1.22464679915E-16,-1.,-7.49879891332945E-33));
#44764=DIRECTION('center_axis',(-1.,1.22464679915E-16,5.91506623067E-14));
#44765=DIRECTION('ref_axis',(1.22464679915E-16,1.,-7.24386692615027E-30));
#44766=DIRECTION('',(1.,0.,1.4772813663E-16));
#44767=DIRECTION('center_axis',(-1.,1.22464679915E-16,6.05071548421E-15));
#44768=DIRECTION('ref_axis',(1.22464679915E-16,1.,-7.40998935030512E-31));
#44769=DIRECTION('center_axis',(-1.22464679914936E-16,-1.,-1.70680191515918E-29));
#44770=DIRECTION('ref_axis',(0.966510120331627,-1.18363352520954E-16,-0.2566285005539));
#44771=DIRECTION('center_axis',(1.22464679915E-16,1.,0.));
#44772=DIRECTION('ref_axis',(1.,-1.22464679915E-16,0.));
#44773=DIRECTION('center_axis',(-8.06530182705333E-18,-1.,-3.03754096780024E-17));
#44774=DIRECTION('ref_axis',(0.966510120331627,0.,-0.256628500553901));
#44775=DIRECTION('center_axis',(0.668126653624933,-8.18219167786918E-17,
0.744047562132925));
#44776=DIRECTION('ref_axis',(0.744047562132925,-1.50412683502806E-31,-0.668126653624933));
#44777=DIRECTION('center_axis',(1.22464679915E-16,1.,5.47382212627E-48));
#44778=DIRECTION('ref_axis',(1.,-1.22464679915E-16,5.9677926224237E-64));
#44779=DIRECTION('center_axis',(0.256628500553901,-3.14279271772879E-17,
0.966510120331627));
#44780=DIRECTION('ref_axis',(0.966510120331627,1.90417037848503E-32,-0.256628500553901));
#44781=DIRECTION('center_axis',(-5.46674034506358E-17,-1.,-6.0879397708352E-17));
#44782=DIRECTION('ref_axis',(0.744047562132925,0.,-0.668126653624934));
#44783=DIRECTION('center_axis',(1.22464679915E-16,1.,5.47382212627E-48));
#44784=DIRECTION('ref_axis',(1.,-1.22464679915E-16,-6.703498746053E-64));
#44785=DIRECTION('center_axis',(0.,1.,0.));
#44786=DIRECTION('ref_axis',(0.997344825668515,0.,0.0728237510173635));
#44787=DIRECTION('center_axis',(-1.22464679915E-16,-1.,0.));
#44788=DIRECTION('ref_axis',(1.,-1.22464679915E-16,0.));
#44789=DIRECTION('center_axis',(-0.825067330468845,1.01041606533981E-16,
0.565034423900893));
#44790=DIRECTION('ref_axis',(0.565034423900893,7.24547600115018E-32,0.825067330468845));
#44791=DIRECTION('center_axis',(0.734238830876792,-8.99183234042744E-17,
0.678891257295808));
#44792=DIRECTION('ref_axis',(0.678891257295808,1.51038693775819E-31,-0.734238830876792));
#44793=DIRECTION('center_axis',(-5.78330237622164E-17,-1.,6.11379105471829E-17));
#44794=DIRECTION('ref_axis',(-0.726469216974212,0.,-0.687199008140201));
#44795=DIRECTION('center_axis',(1.22464679915E-16,1.,5.47382212627E-48));
#44796=DIRECTION('ref_axis',(1.,-1.22464679915E-16,-6.703498746053E-64));
#44797=DIRECTION('center_axis',(-2.81810938552877E-18,-1.,-1.83623833789471E-17));
#44798=DIRECTION('ref_axis',(-0.988427230781696,0.,0.151695779272954));
#44799=DIRECTION('center_axis',(1.22464679915E-16,1.,5.47382212627E-48));
#44800=DIRECTION('ref_axis',(1.,-1.22464679915E-16,-6.703498746053E-64));
#44801=DIRECTION('center_axis',(-1.22464679915E-16,-1.,6.16366086630911E-30));
#44802=DIRECTION('ref_axis',(4.93432455388959E-14,0.,1.));
#44803=DIRECTION('center_axis',(1.22464679915E-16,1.,5.47382212627E-48));
#44804=DIRECTION('ref_axis',(1.,-1.22464679915E-16,-6.703498746053E-64));
#44805=DIRECTION('center_axis',(-1.13563209349214E-16,-1.,-3.17943322838876E-17));
#44806=DIRECTION('ref_axis',(0.269603455472075,0.,-0.962971430935268));
#44807=DIRECTION('center_axis',(1.22464679915E-16,1.,5.47382212627E-48));
#44808=DIRECTION('ref_axis',(1.,-1.22464679915E-16,-6.703498746053E-64));
#44809=DIRECTION('center_axis',(-0.962971430935267,1.17929988057033E-16,
-0.269603455472075));
#44810=DIRECTION('ref_axis',(0.269603455472075,3.05583905676118E-32,-0.962971430935268));
#44811=DIRECTION('center_axis',(1.22464679915E-16,1.,5.47382212627E-48));
#44812=DIRECTION('ref_axis',(1.,-1.22464679915E-16,-6.703498746053E-64));
#44813=DIRECTION('center_axis',(1.22464679915E-16,1.,5.47382212627E-48));
#44814=DIRECTION('ref_axis',(1.,-1.22464679915E-16,0.));
#44815=DIRECTION('center_axis',(0.,0.,1.));
#44816=DIRECTION('ref_axis',(-0.70710677910001,-0.707106783273086,0.));
#44817=DIRECTION('center_axis',(-7.24819500366175E-17,-1.,-6.01900799944532E-17));
#44818=DIRECTION('ref_axis',(0.638858327474962,0.,-0.769324403236954));
#44819=DIRECTION('center_axis',(1.22464679915E-16,1.,5.47382212627E-48));
#44820=DIRECTION('ref_axis',(1.,-1.22464679915E-16,5.9677926224237E-64));
#44821=DIRECTION('center_axis',(0.769324403236954,-9.42150667929943E-17,
0.638858327474961));
#44822=DIRECTION('ref_axis',(0.638858327474961,7.17307849792281E-32,-0.769324403236954));
#44823=DIRECTION('center_axis',(1.22464679915E-16,1.,5.47382212627E-48));
#44824=DIRECTION('ref_axis',(1.,-1.22464679915E-16,6.22660996643423E-64));
#44825=DIRECTION('center_axis',(0.382683432365114,-4.68652040533141E-17,
-0.923879532511277));
#44826=DIRECTION('ref_axis',(2.5429740769239E-34,-1.,5.07265313324192E-17));
#44827=DIRECTION('',(-0.923879532511277,1.79771717893054E-16,-0.382683432365114));
#44828=DIRECTION('',(-1.22604516347E-16,-1.,0.));
#44829=DIRECTION('',(0.923879532511277,-1.79771717893054E-16,0.382683432365114));
#44830=DIRECTION('',(-1.66950830771E-16,-1.,0.));
#44831=DIRECTION('center_axis',(-1.22464679914995E-16,-1.,-2.84643200354157E-29));
#44832=DIRECTION('ref_axis',(0.175818770215043,-2.15315894174053E-17,-0.984422551570244));
#44833=DIRECTION('center_axis',(-1.22464679915E-16,-1.,1.23259516441E-32));
#44834=DIRECTION('ref_axis',(1.,-1.22464679915E-16,-1.13230748611233E-48));
#44835=DIRECTION('',(0.,-1.,0.));
#44836=DIRECTION('center_axis',(-1.22464679915E-16,-1.,1.23259516441E-32));
#44837=DIRECTION('ref_axis',(1.,-1.22464679915E-16,-1.13230748611233E-48));
#44838=DIRECTION('',(0.,1.,0.));
#44839=DIRECTION('center_axis',(-1.22464679915E-16,-1.,3.08148791102E-33));
#44840=DIRECTION('ref_axis',(1.,-1.22464679915E-16,-2.83076871527624E-49));
#44841=DIRECTION('',(0.,-1.,0.));
#44842=DIRECTION('center_axis',(-0.978784588777817,0.0498161334628422,-0.198743758689054));
#44843=DIRECTION('ref_axis',(0.194346018843094,-0.0814603510708595,-0.9775448000799));
#44844=DIRECTION('center_axis',(1.22464679915E-16,1.,0.));
#44845=DIRECTION('ref_axis',(1.,-1.22464679915E-16,0.));
#44846=DIRECTION('',(1.23054276128E-16,1.,0.));
#44847=DIRECTION('center_axis',(0.382683432365114,-4.6865204053314E-17,
0.923879532511277));
#44848=DIRECTION('ref_axis',(-1.22464679914861E-16,-1.,3.33030126354153E-33));
#44849=DIRECTION('',(0.923879532511277,-1.79771717893054E-16,-0.382683432365114));
#44850=DIRECTION('',(-1.66950830771E-16,-1.,0.));
#44851=DIRECTION('center_axis',(-0.382683432285969,-1.4148764236578E-8,
-0.92387953254406));
#44852=DIRECTION('ref_axis',(0.907892103408984,-0.185229284331876,-0.376061219475649));
#44853=DIRECTION('',(-0.923879532511277,1.79771717893054E-16,0.382683432365114));
#44854=DIRECTION('',(-1.22604516347E-16,-1.,0.));
#44855=DIRECTION('center_axis',(-1.22464679915019E-16,-1.,-7.85779417309992E-30));
#44856=DIRECTION('ref_axis',(0.923879532511277,-1.13142611229034E-16,0.382683432365114));
#44857=DIRECTION('center_axis',(1.22464679915E-16,1.,0.));
#44858=DIRECTION('ref_axis',(1.,-1.22464679915E-16,0.));
#44859=DIRECTION('',(-1.16865581539E-16,-1.,0.));
#44860=DIRECTION('center_axis',(0.923879532511277,-1.13142611229034E-16,
0.382683432365114));
#44861=DIRECTION('ref_axis',(-1.31021084567677E-32,-1.,-2.95655891162504E-16));
#44862=DIRECTION('',(0.382683432365114,0.,-0.923879532511277));
#44863=DIRECTION('',(0.,-1.,0.));
#44864=DIRECTION('center_axis',(-0.923879532551608,-4.64401307323437E-9,
-0.382683432267745));
#44865=DIRECTION('ref_axis',(0.376061194482232,-0.185229675161476,-0.907892034023964));
#44866=DIRECTION('',(-0.382683432365114,0.,0.923879532511277));
#44867=DIRECTION('center_axis',(-0.923879532525146,-3.85070599698536E-9,
-0.382683432331632));
#44868=DIRECTION('ref_axis',(0.375653592878795,0.190793753652541,-0.906908000694903));
#44869=DIRECTION('center_axis',(-1.22464679915019E-16,-1.,7.85779417309992E-30));
#44870=DIRECTION('ref_axis',(0.923879532511276,-1.13142611229034E-16,-0.382683432365115));
#44871=DIRECTION('center_axis',(1.22464679915E-16,1.,6.16297582204E-33));
#44872=DIRECTION('ref_axis',(1.,-1.22464679915E-16,-7.54746861370013E-49));
#44873=DIRECTION('',(-2.33731163079E-16,-1.,0.));
#44874=DIRECTION('center_axis',(0.923879532511277,-1.13142611229034E-16,
-0.382683432365114));
#44875=DIRECTION('ref_axis',(-1.31021084567677E-32,-1.,2.95655891162504E-16));
#44876=DIRECTION('',(-0.382683432365114,0.,-0.923879532511277));
#44877=DIRECTION('',(-1.66950830771E-16,-1.,0.));
#44878=DIRECTION('',(0.382683432365114,0.,0.923879532511277));
#44879=DIRECTION('center_axis',(-0.923879531876915,-6.81101431042489E-8,
0.382683433896593));
#44880=DIRECTION('ref_axis',(0.372466611695662,-0.229527742255026,0.899213900419285));
#44881=DIRECTION('center_axis',(-1.2246467991498E-16,-1.,-4.9218209689896E-29));
#44882=DIRECTION('ref_axis',(0.382683432365114,-4.6865204053314E-17,-0.923879532511277));
#44883=DIRECTION('center_axis',(1.22464679915E-16,1.,0.));
#44884=DIRECTION('ref_axis',(1.,-1.22464679915E-16,0.));
#44885=DIRECTION('center_axis',(-1.22464679915E-16,-1.,0.));
#44886=DIRECTION('ref_axis',(1.,-1.22464679915E-16,0.));
#44887=DIRECTION('center_axis',(-0.766057840542209,-0.255399249832434,0.589853039433415));
#44888=DIRECTION('ref_axis',(0.202361789893946,-0.966835675378721,-0.155815540963958));
#44889=DIRECTION('center_axis',(-0.792335098973394,9.70330642810483E-17,
0.610086134029304));
#44890=DIRECTION('ref_axis',(0.610086134029304,5.05601228850744E-32,0.792335098973394));
#44891=DIRECTION('center_axis',(1.22464679915E-16,1.,0.));
#44892=DIRECTION('ref_axis',(1.,-1.22464679915E-16,0.));
#44893=DIRECTION('center_axis',(-7.68827025909336E-17,-1.,5.91985270603321E-17));
#44894=DIRECTION('ref_axis',(0.610086134029304,0.,0.792335098973394));
#44895=DIRECTION('center_axis',(-0.611236674075818,7.48549036428777E-17,
0.791447868317764));
#44896=DIRECTION('ref_axis',(0.791447868317764,-7.00049973634741E-32,0.611236674075818));
#44897=DIRECTION('center_axis',(1.22464679915E-16,1.,5.47382212627E-48));
#44898=DIRECTION('ref_axis',(1.,-1.22464679915E-16,5.40238148608971E-64));
#44899=DIRECTION('center_axis',(-1.22464679914914E-16,-1.,1.11943608056428E-28));
#44900=DIRECTION('ref_axis',(0.610086134029304,-7.47140031243373E-17,0.792335098973394));
#44901=DIRECTION('',(0.,-1.,0.));
#44902=DIRECTION('',(0.,-1.,0.));
#44903=DIRECTION('center_axis',(0.,1.,0.));
#44904=DIRECTION('ref_axis',(0.998985821715464,0.,0.0450258593641339));
#44905=DIRECTION('center_axis',(0.678891257295808,-8.31402005216764E-17,
-0.734238830876792));
#44906=DIRECTION('ref_axis',(4.92781901212525E-33,-1.,1.13233183843457E-16));
#44907=DIRECTION('',(0.734238830876792,0.,0.678891257295808));
#44908=DIRECTION('center_axis',(-0.678891257318237,-7.43492351073594E-12,
0.734238830856053));
#44909=DIRECTION('ref_axis',(1.46208970879984E-10,-1.,1.25062923000865E-10));
#44910=DIRECTION('',(0.,-1.,0.));
#44911=DIRECTION('',(0.734238830876792,0.,0.678891257295808));
#44912=DIRECTION('',(0.,-1.,0.));
#44913=DIRECTION('',(-0.734238830876791,0.,-0.678891257295807));
#44914=DIRECTION('center_axis',(-1.22464679914942E-16,-1.,7.54279763108459E-29));
#44915=DIRECTION('ref_axis',(-0.612227349738988,7.49762264208985E-17,-0.790681776842982));
#44916=DIRECTION('center_axis',(-1.22464679915E-16,-1.,-6.16297582204E-33));
#44917=DIRECTION('ref_axis',(1.,-1.22464679915E-16,-7.54746861370013E-49));
#44918=DIRECTION('',(0.,-1.,0.));
#44919=DIRECTION('center_axis',(1.22464679915E-16,1.,1.23259516441E-32));
#44920=DIRECTION('ref_axis',(1.,-1.22464679915E-16,-1.50949372274247E-48));
#44921=DIRECTION('center_axis',(1.22464679914998E-16,1.,-1.73663083545565E-29));
#44922=DIRECTION('ref_axis',(0.095298509688002,-1.16707014853003E-17,0.99544874004202));
#44923=DIRECTION('center_axis',(-1.22464679915E-16,-1.,0.));
#44924=DIRECTION('ref_axis',(1.,-1.22464679915E-16,0.));
#44925=DIRECTION('center_axis',(1.22464679915E-16,1.,0.));
#44926=DIRECTION('ref_axis',(1.,-1.22464679915E-16,0.));
#44927=DIRECTION('',(-1.32169407693E-16,-1.,0.));
#44928=DIRECTION('center_axis',(-1.22464679915E-16,-1.,-7.60253073092891E-48));
#44929=DIRECTION('ref_axis',(-1.,1.22464679915E-16,9.3104149250716E-64));
#44930=DIRECTION('center_axis',(-1.22464679915E-16,-1.,6.16297582204E-33));
#44931=DIRECTION('ref_axis',(1.,-1.22464679915E-16,7.54746861370013E-49));
#44932=DIRECTION('',(-1.23358113847E-16,-1.,0.));
#44933=DIRECTION('center_axis',(1.22464679915E-16,1.,3.08148791102E-33));
#44934=DIRECTION('ref_axis',(1.,-1.22464679915E-16,-3.77373430685006E-49));
#44935=DIRECTION('center_axis',(-1.,1.22464679915E-16,-6.12323399574E-17));
#44936=DIRECTION('ref_axis',(-6.12323399574E-17,0.,1.));
#44937=DIRECTION('',(-2.17106560191E-16,0.,1.));
#44938=DIRECTION('',(2.19188076492E-16,0.,-1.));
#44939=DIRECTION('',(-1.32169407693E-16,-1.,0.));
#44940=DIRECTION('center_axis',(1.22464679914917E-16,1.,-1.21085355525786E-28));
#44941=DIRECTION('ref_axis',(0.566106835688783,-6.93280924301735E-17,0.824331881335687));
#44942=DIRECTION('',(0.,-1.,0.));
#44943=DIRECTION('center_axis',(-1.22464679915E-16,-1.,-1.23259516441E-32));
#44944=DIRECTION('ref_axis',(1.,-1.22464679915E-16,-1.50949372274247E-48));
#44945=DIRECTION('center_axis',(1.22464679915E-16,1.,-1.21640491694863E-46));
#44946=DIRECTION('ref_axis',(-1.,1.22464679915E-16,-5.78241158658936E-15));
#44947=DIRECTION('center_axis',(-1.22464679915E-16,-1.,-6.16297582204E-33));
#44948=DIRECTION('ref_axis',(1.,-1.22464679915E-16,-7.54746861370013E-49));
#44949=DIRECTION('',(-1.04083408559E-16,-1.,0.));
#44950=DIRECTION('center_axis',(1.22464679915E-16,1.,7.00649232162E-46));
#44951=DIRECTION('ref_axis',(1.,-1.22464679915E-16,-8.58047839494098E-62));
#44952=DIRECTION('center_axis',(1.22464679914999E-16,1.,-1.9442368107527E-29));
#44953=DIRECTION('ref_axis',(0.0510637267514752,-6.25350295186696E-18,0.998695396910515));
#44954=DIRECTION('center_axis',(-1.22464679915E-16,-1.,1.23259516441E-32));
#44955=DIRECTION('ref_axis',(1.,-1.22464679915E-16,-1.40210791623289E-48));
#44956=DIRECTION('center_axis',(1.22464679915E-16,1.,-1.54074395551E-33));
#44957=DIRECTION('ref_axis',(1.,-1.22464679915E-16,-1.75263489528827E-49));
#44958=DIRECTION('center_axis',(2.17357452795E-16,-2.66186108837E-32,-1.));
#44959=DIRECTION('ref_axis',(1.,5.7857534586223E-48,2.17357452795E-16));
#44960=DIRECTION('',(-8.96394535471E-17,0.,1.));
#44961=DIRECTION('center_axis',(1.65006284806E-14,-2.02074418527E-30,-1.));
#44962=DIRECTION('ref_axis',(1.,-1.71077471584193E-45,1.65006284806E-14));
#44963=DIRECTION('',(-8.96394535471E-17,0.,1.));
#44964=DIRECTION('center_axis',(-1.74860126378E-14,2.14141894068E-30,-1.));
#44965=DIRECTION('ref_axis',(1.,2.97181576564967E-46,-1.74860126378E-14));
#44966=DIRECTION('center_axis',(-1.17989839311979E-16,-1.,2.29779399358865E-17));
#44967=DIRECTION('ref_axis',(0.191153986297934,0.,0.981560061087659));
#44968=DIRECTION('center_axis',(1.22464679915E-16,1.,5.47382212627E-48));
#44969=DIRECTION('ref_axis',(1.,-1.22464679915E-16,-6.703498746053E-64));
#44970=DIRECTION('center_axis',(-0.973274002238674,1.1919168915396E-16,
0.229646938943923));
#44971=DIRECTION('ref_axis',(0.229646938943923,-2.91124363913666E-32,0.973274002238674));
#44972=DIRECTION('center_axis',(1.22464679915E-16,1.,5.47382212627E-48));
#44973=DIRECTION('ref_axis',(1.,-1.22464679915E-16,-6.703498746053E-64));
#44974=DIRECTION('center_axis',(-0.981560061087659,1.20206438697958E-16,
0.191153986297933));
#44975=DIRECTION('ref_axis',(0.191153986297933,-8.55574366268044E-33,0.981560061087659));
#44976=DIRECTION('center_axis',(-1.17989839311979E-16,-1.,2.29779399358865E-17));
#44977=DIRECTION('ref_axis',(-0.191153986297933,0.,-0.981560061087659));
#44978=DIRECTION('center_axis',(-1.22464679915E-16,-1.,-5.47382212627E-48));
#44979=DIRECTION('ref_axis',(1.,-1.22464679915E-16,-6.703498746053E-64));
#44980=DIRECTION('center_axis',(-1.22464679915E-16,-1.,0.));
#44981=DIRECTION('ref_axis',(1.,-1.22464679915E-16,0.));
#44982=DIRECTION('center_axis',(-2.17357452795E-16,2.66186108837E-32,1.));
#44983=DIRECTION('ref_axis',(1.,5.7857534586223E-48,2.17357452795E-16));
#44984=DIRECTION('center_axis',(-2.17357452795E-16,2.66186108835898E-32,
1.));
#44985=DIRECTION('ref_axis',(-3.61400724161833E-16,-1.,-5.19345299584946E-32));
#44986=DIRECTION('',(5.71347413162E-17,0.,-1.));
#44987=DIRECTION('',(7.61796550883E-17,0.,-1.));
#44988=DIRECTION('center_axis',(-6.13854691746E-15,7.51755183389E-31,1.));
#44989=DIRECTION('ref_axis',(1.,2.67726580969963E-46,6.13854691746E-15));
#44990=DIRECTION('center_axis',(-4.29367103357466E-45,-1.,7.25136572506882E-31));
#44991=DIRECTION('ref_axis',(-1.,0.,-5.9211894646675E-15));
#44992=DIRECTION('center_axis',(-1.22464679915E-16,-1.,-5.47382212627E-48));
#44993=DIRECTION('ref_axis',(1.,-1.22464679915E-16,-6.703498746053E-64));
#44994=DIRECTION('center_axis',(-1.22464679915E-16,-1.,-3.08148791102E-33));
#44995=DIRECTION('ref_axis',(1.,-1.22464679915E-16,-3.77373430685006E-49));
#44996=DIRECTION('center_axis',(0.984869499718035,-1.20611728041004E-16,
-0.173297629889006));
#44997=DIRECTION('ref_axis',(0.173297629889006,5.41148511020646E-32,0.984869499718035));
#44998=DIRECTION('center_axis',(-1.18786812255882E-16,-1.,2.09017266063253E-17));
#44999=DIRECTION('ref_axis',(0.173297629889006,0.,0.984869499718035));
#45000=DIRECTION('center_axis',(-1.22464679915E-16,-1.,-5.47382212627E-48));
#45001=DIRECTION('ref_axis',(1.,-1.22464679915E-16,-6.703498746053E-64));
#45002=DIRECTION('center_axis',(-1.22464679915E-16,-1.,-5.47382212627E-48));
#45003=DIRECTION('ref_axis',(1.,-1.22464679915E-16,-6.703498746053E-64));
#45004=DIRECTION('center_axis',(0.825067330468845,-1.01041606533981E-16,
-0.565034423900893));
#45005=DIRECTION('ref_axis',(0.565034423900893,7.24547600115018E-32,0.825067330468845));
#45006=DIRECTION('center_axis',(-6.60215246509141E-17,-1.,-6.10447636300053E-17));
#45007=DIRECTION('ref_axis',(0.678891257295808,0.,-0.734238830876792));
#45008=DIRECTION('center_axis',(-1.22464679915E-16,-1.,-5.47382212627E-48));
#45009=DIRECTION('ref_axis',(1.,-1.22464679915E-16,-6.703498746053E-64));
#45010=DIRECTION('center_axis',(-0.734238830876792,8.99183234042744E-17,
-0.678891257295808));
#45011=DIRECTION('ref_axis',(0.678891257295808,-2.24691316591619E-32,-0.734238830876792));
#45012=DIRECTION('center_axis',(-1.22464679915E-16,-1.,0.));
#45013=DIRECTION('ref_axis',(1.,-1.22464679915E-16,0.));
#45014=DIRECTION('center_axis',(-8.3366128569448E-17,-1.,5.70919859380671E-17));
#45015=DIRECTION('ref_axis',(0.565034423900894,0.,0.825067330468845));
#45016=DIRECTION('center_axis',(-1.22464679915E-16,-1.,-5.47382212627E-48));
#45017=DIRECTION('ref_axis',(1.,-1.22464679915E-16,-6.703498746053E-64));
#45018=DIRECTION('center_axis',(-1.22464679915E-16,-1.,0.));
#45019=DIRECTION('ref_axis',(1.,-1.22464679915E-16,0.));
#45020=DIRECTION('center_axis',(-0.734238830876792,8.99183234042744E-17,
-0.678891257295808));
#45021=DIRECTION('ref_axis',(0.678891257295808,-2.24691316591619E-32,-0.734238830876792));
#45022=DIRECTION('center_axis',(-0.734238830876792,8.99183234039869E-17,
-0.678891257295808));
#45023=DIRECTION('ref_axis',(-6.60215246505446E-17,-1.,-6.10447636296637E-17));
#45024=DIRECTION('',(0.734238830876791,0.,0.678891257295807));
#45025=DIRECTION('',(0.734238830876791,0.,0.678891257295807));
#45026=DIRECTION('center_axis',(-5.11601622893148E-18,-1.,-2.45021972047681E-17));
#45027=DIRECTION('ref_axis',(0.978889450967439,0.,-0.204390417546091));
#45028=DIRECTION('center_axis',(1.22464679915E-16,1.,5.47382212627E-48));
#45029=DIRECTION('ref_axis',(1.,-1.22464679915E-16,-6.703498746053E-64));
#45030=DIRECTION('center_axis',(0.419584599500152,-5.13842936749187E-17,
0.90771623531933));
#45031=DIRECTION('ref_axis',(0.90771623531933,-2.72267697829008E-32,-0.419584599500152));
#45032=DIRECTION('center_axis',(1.22464679915E-16,1.,5.47382212627E-48));
#45033=DIRECTION('ref_axis',(1.,-1.22464679915E-16,-6.703498746053E-64));
#45034=DIRECTION('center_axis',(0.204390417546092,-2.50306070625112E-17,
0.978889450967439));
#45035=DIRECTION('ref_axis',(0.978889450967439,-1.05289930055147E-32,-0.204390417546092));
#45036=DIRECTION('center_axis',(0.382683432358122,-7.15701713406616E-12,
0.923879532514173));
#45037=DIRECTION('ref_axis',(0.653281512864065,-0.707106748253927,-0.270598062675614));
#45038=DIRECTION('center_axis',(0.38263696551694,0.0155798009318935,0.923767407101436));
#45039=DIRECTION('ref_axis',(0.670813976387107,-0.692209320629282,-0.266185772568081));
#45040=DIRECTION('center_axis',(-2.15600582822439E-17,-1.,-4.66423576092589E-17));
#45041=DIRECTION('ref_axis',(0.90771623531933,0.,-0.419584599500153));
#45042=DIRECTION('center_axis',(1.22464679915E-16,1.,5.47382212627E-48));
#45043=DIRECTION('ref_axis',(1.,-1.22464679915E-16,-6.703498746053E-64));
#45044=DIRECTION('center_axis',(1.22464679915E-16,1.,-6.16297582204E-33));
#45045=DIRECTION('ref_axis',(1.,-1.22464679915E-16,7.54746861370013E-49));
#45046=DIRECTION('center_axis',(-0.0335155327516907,4.10446899060886E-18,
-0.999438196720723));
#45047=DIRECTION('ref_axis',(0.999438196720723,5.21239906410075E-34,-0.0335155327516907));
#45048=DIRECTION('center_axis',(-0.382579809484663,-0.023273941363381,0.923629261678133));
#45049=DIRECTION('ref_axis',(0.67915166414103,-0.684855543423067,0.264056626005038));
#45050=DIRECTION('center_axis',(-0.854119175465141,0.0486728274083025,-0.517794737299279));
#45051=DIRECTION('ref_axis',(0.493271987057746,-0.239694157277359,-0.836199412670925));
#45052=DIRECTION('center_axis',(-0.382683355639379,3.37879318962009E-8,
0.923879564292112));
#45053=DIRECTION('ref_axis',(0.653293929364642,-0.70709332290268,0.270603168055648));
#45054=DIRECTION('center_axis',(0.382579803835696,0.0232740021763249,0.923629262485624));
#45055=DIRECTION('ref_axis',(0.679151158571202,-0.684856150498969,-0.264056351817426));
#45056=DIRECTION('center_axis',(-0.854168457972516,0.0469001823254461,0.517877030097584));
#45057=DIRECTION('ref_axis',(0.479715571846213,-0.313264897733587,0.819596287190362));
#45058=DIRECTION('center_axis',(-5.06268119967007E-18,-1.,2.43796819441885E-17));
#45059=DIRECTION('ref_axis',(0.979111878581668,0.,0.203322230019931));
#45060=DIRECTION('center_axis',(-1.22464679915E-16,-1.,-5.47382212627E-48));
#45061=DIRECTION('ref_axis',(1.,-1.22464679915E-16,-6.703498746053E-64));
#45062=DIRECTION('center_axis',(0.203322230019931,-2.48997918188915E-17,
-0.979111878581668));
#45063=DIRECTION('ref_axis',(0.979111878581668,-1.33094098597294E-33,0.203322230019931));
#45064=DIRECTION('center_axis',(-1.22464679915E-16,-1.,-5.47382212627E-48));
#45065=DIRECTION('ref_axis',(1.,-1.22464679915E-16,-6.703498746053E-64));
#45066=DIRECTION('center_axis',(-1.22464679915E-16,-1.,0.));
#45067=DIRECTION('ref_axis',(0.,0.,1.));
#45068=DIRECTION('center_axis',(1.22464679915E-16,1.,5.47382212627E-48));
#45069=DIRECTION('ref_axis',(1.,-1.22464679915E-16,-6.703498746053E-64));
#45070=DIRECTION('center_axis',(1.22464679915E-16,1.,5.47382212627E-48));
#45071=DIRECTION('ref_axis',(1.,-1.22464679915E-16,-6.703498746053E-64));
#45072=DIRECTION('center_axis',(-1.,1.22464679915E-16,-6.12323399574E-17));
#45073=DIRECTION('ref_axis',(-1.22464679915E-16,-1.,-7.49879891332945E-33));
#45074=DIRECTION('center_axis',(-5.06268119967007E-18,-1.,2.43796819441885E-17));
#45075=DIRECTION('ref_axis',(-0.979111878581668,0.,-0.203322230019931));
#45076=DIRECTION('center_axis',(1.22464679915E-16,1.,-3.08148791102E-33));
#45077=DIRECTION('ref_axis',(1.,-1.22464679915E-16,3.77373430685006E-49));
#45078=DIRECTION('center_axis',(-1.,1.22464679915E-16,-6.12323399574E-17));
#45079=DIRECTION('ref_axis',(-1.22464679915E-16,-1.,-7.49879891332945E-33));
#45080=DIRECTION('center_axis',(1.22464679915E-16,1.,5.47382212627E-48));
#45081=DIRECTION('ref_axis',(1.,-1.22464679915E-16,-6.703498746053E-64));
#45082=DIRECTION('center_axis',(-1.,1.22464679915E-16,-6.12323399574E-17));
#45083=DIRECTION('ref_axis',(6.12323399574E-17,-7.49879891332945E-33,-1.));
#45084=DIRECTION('',(1.,0.,0.));
#45085=DIRECTION('',(1.,0.,0.));
#45086=DIRECTION('center_axis',(-0.923629285580912,-0.0232739550451307,
0.382579750945933));
#45087=DIRECTION('ref_axis',(0.293516536156795,-0.684855540988734,0.666948971795853));
#45088=DIRECTION('center_axis',(-0.237817287821767,0.0486733035113049,-0.970089607788062));
#45089=DIRECTION('ref_axis',(0.940079656645484,-0.239688427719097,-0.242486487827378));
#45090=DIRECTION('center_axis',(-0.923879500687952,3.38250871562384E-8,
0.382683509193406));
#45091=DIRECTION('ref_axis',(0.27060322877475,-0.707093332552184,0.653293893769816));
#45092=DIRECTION('center_axis',(-0.382579702456672,0.0232740169688495,0.923629304105439));
#45093=DIRECTION('ref_axis',(0.666946643181329,-0.68485819132246,0.293515643412214));
#45094=DIRECTION('center_axis',(-0.382683432278913,-8.22329173318955E-13,
0.923879532546982));
#45095=DIRECTION('ref_axis',(0.653281507495611,-0.707106754092149,0.270598060380203));
#45096=DIRECTION('center_axis',(-0.970090315877611,0.0486596525433631,-0.237817192933641));
#45097=DIRECTION('ref_axis',(0.242427238271629,0.244261263603387,-0.938917179120112));
#45098=DIRECTION('center_axis',(-7.79403475186991E-17,-1.,5.89087594505755E-17));
#45099=DIRECTION('ref_axis',(0.602966636474875,0.,0.797766403966835));
#45100=DIRECTION('center_axis',(1.22464679915E-16,1.,5.47382212627E-48));
#45101=DIRECTION('ref_axis',(1.,-1.22464679915E-16,-6.703498746053E-64));
#45102=DIRECTION('center_axis',(-0.585630202615096,7.17190153117117E-17,
0.810578352650132));
#45103=DIRECTION('ref_axis',(0.810578352650132,6.4321265031143E-32,0.585630202615096));
#45104=DIRECTION('center_axis',(1.22464679915E-16,1.,5.47382212627E-48));
#45105=DIRECTION('ref_axis',(1.,-1.22464679915E-16,-6.703498746053E-64));
#45106=DIRECTION('center_axis',(-0.797766403966835,9.76982073084798E-17,
0.602966636474875));
#45107=DIRECTION('ref_axis',(0.602966636474875,6.43171104150991E-32,0.797766403966835));
#45108=DIRECTION('center_axis',(1.22464679915E-16,1.,5.47382212627E-48));
#45109=DIRECTION('ref_axis',(1.,-1.22464679915E-16,-6.703498746053E-64));
#45110=DIRECTION('center_axis',(-7.79403475186991E-17,-1.,5.89087594505755E-17));
#45111=DIRECTION('ref_axis',(-0.602966636474876,0.,-0.797766403966835));
#45112=DIRECTION('center_axis',(-1.22464679915E-16,-1.,-5.47382212627E-48));
#45113=DIRECTION('ref_axis',(1.,-1.22464679915E-16,-6.703498746053E-64));
#45114=DIRECTION('center_axis',(-1.22464679915E-16,-1.,0.));
#45115=DIRECTION('ref_axis',(1.,-1.22464679915E-16,0.));
#45116=DIRECTION('center_axis',(0.734238830876792,-8.99183234042744E-17,
0.678891257295808));
#45117=DIRECTION('ref_axis',(0.678891257295808,-2.24691316591619E-32,-0.734238830876792));
#45118=DIRECTION('center_axis',(-0.734238830876792,8.99183234042744E-17,
-0.678891257295808));
#45119=DIRECTION('ref_axis',(0.678891257295808,1.51038693775819E-31,-0.734238830876792));
#45120=DIRECTION('',(-0.734238830876791,0.,-0.678891257295807));
#45121=DIRECTION('',(-0.734238830876791,0.,-0.678891257295807));
#45122=DIRECTION('center_axis',(0.73423883087825,-8.99183234044306E-17,
0.678891257294231));
#45123=DIRECTION('ref_axis',(0.678891257294231,1.10716302178481E-31,-0.73423883087825));
#45124=DIRECTION('center_axis',(-6.60215246511763E-17,-1.,-6.10447636299848E-17));
#45125=DIRECTION('ref_axis',(-0.678891257294231,0.,0.73423883087825));
#45126=DIRECTION('center_axis',(-1.22464679915E-16,-1.,-5.47382212627E-48));
#45127=DIRECTION('ref_axis',(1.,-1.22464679915E-16,-6.703498746053E-64));
#45128=DIRECTION('center_axis',(-1.22464679915E-16,-1.,0.));
#45129=DIRECTION('ref_axis',(1.,-1.22464679915E-16,0.));
#45130=DIRECTION('center_axis',(0.581646529321033,-7.12311560368041E-17,
-0.813441648140047));
#45131=DIRECTION('ref_axis',(0.813441648140047,-2.80119922649672E-32,0.581646529321033));
#45132=DIRECTION('center_axis',(-4.14313546884292E-17,-1.,5.79423889656346E-17));
#45133=DIRECTION('ref_axis',(0.813441648140047,0.,0.581646529321034));
#45134=DIRECTION('center_axis',(-1.22464679915E-16,-1.,-5.47382212627E-48));
#45135=DIRECTION('ref_axis',(1.,-1.22464679915E-16,-6.703498746053E-64));
#45136=DIRECTION('center_axis',(-1.22464679915E-16,-1.,-5.47382212627E-48));
#45137=DIRECTION('ref_axis',(1.,-1.22464679915E-16,-6.703498746053E-64));
#45138=DIRECTION('center_axis',(0.142980079684983,-1.75100096927979E-17,
-0.98972556641388));
#45139=DIRECTION('ref_axis',(0.98972556641388,3.23015489124122E-33,0.142980079684983));
#45140=DIRECTION('center_axis',(-1.22464679915E-16,-1.,0.));
#45141=DIRECTION('ref_axis',(0.,0.,-1.));
#45142=DIRECTION('center_axis',(-1.22464679915E-16,-1.,-5.47382212627E-48));
#45143=DIRECTION('ref_axis',(1.,-1.22464679915E-16,-6.703498746053E-64));
#45144=DIRECTION('center_axis',(-1.,1.22464679915E-16,-6.12323399574E-17));
#45145=DIRECTION('ref_axis',(-1.22464679915E-16,-1.,-7.49879891332945E-33));
#45146=DIRECTION('center_axis',(-1.22464679915E-16,-1.,-5.47382212627E-48));
#45147=DIRECTION('ref_axis',(1.,-1.22464679915E-16,-6.703498746053E-64));
#45148=DIRECTION('center_axis',(-2.50358258116745E-18,-1.,1.73301042611612E-17));
#45149=DIRECTION('ref_axis',(0.98972556641388,0.,0.142980079684983));
#45150=DIRECTION('center_axis',(-1.22464679915E-16,-1.,-5.47382212627E-48));
#45151=DIRECTION('ref_axis',(1.,-1.22464679915E-16,-6.703498746053E-64));
#45152=DIRECTION('center_axis',(-1.22464679915E-16,-1.,-5.47382212627E-48));
#45153=DIRECTION('ref_axis',(1.,-1.22464679915E-16,-6.703498746053E-64));
#45154=DIRECTION('center_axis',(-1.,1.22464679915E-16,-6.12323399574E-17));
#45155=DIRECTION('ref_axis',(-1.22464679915E-16,-1.,-7.49879891332945E-33));
#45156=DIRECTION('center_axis',(-1.,1.22464679915E-16,-6.12323399574E-17));
#45157=DIRECTION('ref_axis',(-1.22464679915E-16,-1.,-7.49879891332945E-33));
#45158=DIRECTION('',(1.,0.,2.89652532403E-16));
#45159=DIRECTION('',(1.,0.,2.89652532403E-16));
#45160=DIRECTION('center_axis',(-0.734238830876792,8.99183234042744E-17,
-0.678891257295808));
#45161=DIRECTION('ref_axis',(-0.678891257295808,2.24691316591619E-32,0.734238830876792));
#45162=DIRECTION('',(0.734238830876791,0.,0.678891257295807));
#45163=DIRECTION('center_axis',(0.734238830881723,7.25497069118018E-12,
0.678891257290474));
#45164=DIRECTION('ref_axis',(-0.678891257290474,0.,0.734238830881723));
#45165=DIRECTION('',(0.734238830876791,0.,0.678891257295807));
#45166=DIRECTION('center_axis',(-0.734238830876792,8.991832340449E-17,-0.678891257295808));
#45167=DIRECTION('ref_axis',(6.6021524650914E-17,1.,6.10447636300053E-17));
#45168=DIRECTION('',(-0.734238830876791,0.,-0.678891257295807));
#45169=DIRECTION('',(-0.734238830876791,0.,-0.678891257295807));
#45170=DIRECTION('center_axis',(1.69872863391202E-17,1.,-4.23293596334453E-17));
#45171=DIRECTION('ref_axis',(-0.928056183869048,0.,-0.37244022283102));
#45172=DIRECTION('center_axis',(-1.22464679915E-16,-1.,-5.47382212627E-48));
#45173=DIRECTION('ref_axis',(1.,-1.22464679915E-16,-6.703498746053E-64));
#45174=DIRECTION('center_axis',(-1.22464679915E-16,-1.,-5.47382212627E-48));
#45175=DIRECTION('ref_axis',(1.,-1.22464679915E-16,-6.703498746053E-64));
#45176=DIRECTION('center_axis',(0.204390417555875,-1.0300808526955E-11,
0.978889450965396));
#45177=DIRECTION('ref_axis',(-1.00253139123651E-11,1.,1.26158343031571E-11));
#45178=DIRECTION('center_axis',(0.,1.,0.));
#45179=DIRECTION('ref_axis',(-0.231145326606897,0.,-0.972919235079557));
#45180=DIRECTION('center_axis',(-1.22464679915E-16,-1.,6.16297582204E-33));
#45181=DIRECTION('ref_axis',(1.,-1.22464679915E-16,7.54746861370013E-49));
#45182=DIRECTION('center_axis',(-0.0335155327516907,4.10446899060886E-18,
-0.999438196720723));
#45183=DIRECTION('ref_axis',(0.999438196720723,5.21239906410075E-34,-0.0335155327516907));
#45184=DIRECTION('center_axis',(5.9296278727138E-17,1.,-6.12017248415691E-17));
#45185=DIRECTION('ref_axis',(-0.718198537785833,0.,-0.695838242928838));
#45186=DIRECTION('center_axis',(1.22464679915E-16,1.,5.47382212627E-48));
#45187=DIRECTION('ref_axis',(1.,-1.22464679915E-16,-6.703498746053E-64));
#45188=DIRECTION('center_axis',(1.22464679915E-16,1.,5.47382212627E-48));
#45189=DIRECTION('ref_axis',(1.,-1.22464679915E-16,-6.703498746053E-64));
#45190=DIRECTION('center_axis',(0.,1.,0.));
#45191=DIRECTION('ref_axis',(0.776012376688289,0.,0.630717679494236));
#45192=DIRECTION('center_axis',(-1.22464679915E-16,-1.,-5.47382212627E-48));
#45193=DIRECTION('ref_axis',(1.,-1.22464679915E-16,-6.703498746053E-64));
#45194=DIRECTION('center_axis',(-1.,1.22464679915E-16,-6.12323399574E-17));
#45195=DIRECTION('ref_axis',(-1.22464679915E-16,-1.,-7.49879891332945E-33));
#45196=DIRECTION('center_axis',(0.,0.,1.));
#45197=DIRECTION('ref_axis',(1.,0.,0.));
#45198=DIRECTION('center_axis',(-1.22464679915E-16,-1.,3.08148791102E-33));
#45199=DIRECTION('ref_axis',(1.,-1.22464679915E-16,3.77373430685006E-49));
#45200=DIRECTION('center_axis',(-1.,1.22464679915E-16,-6.12323399574E-17));
#45201=DIRECTION('ref_axis',(-1.22464679915E-16,-1.,-7.49879891332945E-33));
#45202=DIRECTION('center_axis',(0.,1.,0.));
#45203=DIRECTION('ref_axis',(-0.998774211147154,0.,-0.0494982337804088));
#45204=DIRECTION('center_axis',(1.22464679915E-16,1.,0.));
#45205=DIRECTION('ref_axis',(1.,-1.22464679915E-16,0.));
#45206=DIRECTION('center_axis',(-0.797766403966835,9.76982073084798E-17,
0.602966636474875));
#45207=DIRECTION('ref_axis',(0.602966636474875,6.43171104150991E-32,0.797766403966835));
#45208=DIRECTION('center_axis',(-1.,1.22464679915E-16,-6.12323399574E-17));
#45209=DIRECTION('ref_axis',(-6.12323399574E-17,7.49879891332945E-33,1.));
#45210=DIRECTION('',(-1.,0.,0.));
#45211=DIRECTION('',(-1.,0.,-4.09734305096E-16));
#45212=DIRECTION('center_axis',(5.9296278727138E-17,1.,-6.12017248415691E-17));
#45213=DIRECTION('ref_axis',(0.714687205042172,0.,0.699444207173816));
#45214=DIRECTION('center_axis',(-1.22464679915E-16,-1.,-5.47382212627E-48));
#45215=DIRECTION('ref_axis',(1.,-1.22464679915E-16,-6.703498746053E-64));
#45216=DIRECTION('center_axis',(-1.22464679915E-16,-1.,-5.47382212627E-48));
#45217=DIRECTION('ref_axis',(1.,-1.22464679915E-16,-6.703498746053E-64));
#45218=DIRECTION('center_axis',(0.585630202617415,2.24275747059828E-12,
-0.810578352648456));
#45219=DIRECTION('ref_axis',(1.0249208888998E-11,1.,1.01714932772742E-11));
#45220=DIRECTION('center_axis',(-2.68354439599323E-46,-1.,-1.81284143127026E-31));
#45221=DIRECTION('ref_axis',(-1.,0.,1.97372982155583E-15));
#45222=DIRECTION('center_axis',(1.22464679915E-16,1.,5.47382212627E-48));
#45223=DIRECTION('ref_axis',(1.,-1.22464679915E-16,-6.703498746053E-64));
#45224=DIRECTION('center_axis',(-0.991694064582439,1.21447496192053E-16,
-0.128619136492057));
#45225=DIRECTION('ref_axis',(0.128619136492057,-7.10548517584315E-33,-0.991694064582438));
#45226=DIRECTION('center_axis',(1.22464679915E-16,1.,5.47382212627E-48));
#45227=DIRECTION('ref_axis',(1.,-1.22464679915E-16,-6.703498746053E-64));
#45228=DIRECTION('center_axis',(-8.38660245249135E-17,-1.,-5.68956569482564E-17));
#45229=DIRECTION('ref_axis',(0.561410669601872,0.,-0.827537346623811));
#45230=DIRECTION('center_axis',(-1.22464679915E-16,-1.,-5.47382212627E-48));
#45231=DIRECTION('ref_axis',(1.,-1.22464679915E-16,-6.703498746053E-64));
#45232=DIRECTION('center_axis',(-0.827537346623811,1.01344096271977E-16,
-0.561410669601872));
#45233=DIRECTION('ref_axis',(0.561410669601872,-5.47362952277333E-32,-0.827537346623811));
#45234=DIRECTION('center_axis',(-1.22464679915E-16,-1.,-5.47382212627E-48));
#45235=DIRECTION('ref_axis',(1.,-1.22464679915E-16,-6.703498746053E-64));
#45236=DIRECTION('center_axis',(-5.78330237622164E-17,-1.,6.11379105471829E-17));
#45237=DIRECTION('ref_axis',(0.726469216974212,0.,0.687199008140201));
#45238=DIRECTION('center_axis',(1.22464679915E-16,1.,-1.23259516441E-32));
#45239=DIRECTION('ref_axis',(1.,-1.22464679915E-16,1.50949372274247E-48));
#45240=DIRECTION('center_axis',(1.22464679915E-16,1.,5.47382212627E-48));
#45241=DIRECTION('ref_axis',(1.,-1.22464679915E-16,-6.703498746053E-64));
#45242=DIRECTION('center_axis',(-0.687199008140201,8.41576065696246E-17,
0.726469216974212));
#45243=DIRECTION('ref_axis',(0.726469216974212,1.50838013754883E-32,0.687199008140201));
#45244=DIRECTION('center_axis',(-8.38660245249135E-17,-1.,-5.68956569482564E-17));
#45245=DIRECTION('ref_axis',(-0.561410669601872,0.,0.827537346623811));
#45246=DIRECTION('center_axis',(1.22464679915E-16,1.,0.));
#45247=DIRECTION('ref_axis',(1.,-1.22464679915E-16,0.));
#45248=DIRECTION('center_axis',(-0.687199008140201,8.41576065696246E-17,
0.726469216974212));
#45249=DIRECTION('ref_axis',(0.726469216974212,1.50838013754883E-32,0.687199008140201));
#45250=DIRECTION('center_axis',(1.22464679915E-16,1.,5.47382212627E-48));
#45251=DIRECTION('ref_axis',(1.,-1.22464679915E-16,-6.703498746053E-64));
#45252=DIRECTION('center_axis',(1.,0.,0.));
#45253=DIRECTION('ref_axis',(0.,-1.,0.));
#45254=DIRECTION('center_axis',(-1.22464679915E-16,-1.,0.));
#45255=DIRECTION('ref_axis',(1.,-1.22464679915E-16,0.));
#45256=DIRECTION('center_axis',(0.973274002238674,-1.1919168915396E-16,
-0.229646938943923));
#45257=DIRECTION('ref_axis',(0.229646938943923,-2.91124363913666E-32,0.973274002238674));
#45258=DIRECTION('center_axis',(1.22464679914958E-16,1.,1.38940690218481E-28));
#45259=DIRECTION('ref_axis',(0.287097106361984,-3.51592552349981E-17,-0.957901483200948));
#45260=DIRECTION('center_axis',(-1.22464679915E-16,-1.,0.));
#45261=DIRECTION('ref_axis',(1.,-1.22464679915E-16,0.));
#45262=DIRECTION('',(-1.13288063737E-16,-1.,0.));
#45263=DIRECTION('',(-1.21155290386E-16,-1.,0.));
#45264=DIRECTION('center_axis',(0.,0.,1.));
#45265=DIRECTION('ref_axis',(1.,0.,0.));
#45266=DIRECTION('center_axis',(-1.22464679915E-16,-1.,0.));
#45267=DIRECTION('ref_axis',(1.,-1.22464679915E-16,0.));
#45268=DIRECTION('center_axis',(1.16436507708486E-16,1.,2.6493382562289E-17));
#45269=DIRECTION('ref_axis',(0.221864286407976,0.,-0.975077555077892));
#45270=DIRECTION('center_axis',(-1.22464679915E-16,-1.,-5.47382212627E-48));
#45271=DIRECTION('ref_axis',(1.,-1.22464679915E-16,-6.703498746053E-64));
#45272=DIRECTION('center_axis',(1.22464679915E-16,1.,7.60253073092891E-48));
#45273=DIRECTION('ref_axis',(1.,-1.22464679915E-16,-9.3104149250716E-64));
#45274=DIRECTION('',(0.,1.,0.));
#45275=DIRECTION('center_axis',(1.22464679915E-16,1.,0.));
#45276=DIRECTION('ref_axis',(1.,-1.22464679915E-16,0.));
#45277=DIRECTION('',(0.,1.,0.));
#45278=DIRECTION('center_axis',(-1.22464679915E-16,-1.,-8.75811540203E-47));
#45279=DIRECTION('ref_axis',(1.,-1.22464679915E-16,-1.07255979936824E-62));
#45280=DIRECTION('center_axis',(5.9296278727138E-17,1.,-6.12017248415691E-17));
#45281=DIRECTION('ref_axis',(-0.718198537785833,0.,-0.695838242928838));
#45282=DIRECTION('center_axis',(-1.22464679915E-16,-1.,-5.47382212627E-48));
#45283=DIRECTION('ref_axis',(1.,-1.22464679915E-16,-6.703498746053E-64));
#45284=DIRECTION('center_axis',(-1.22464679915E-16,-1.,-5.47382212627E-48));
#45285=DIRECTION('ref_axis',(1.,-1.22464679915E-16,-6.703498746053E-64));
#45286=DIRECTION('center_axis',(1.22464679915E-16,1.,5.47382212627E-48));
#45287=DIRECTION('ref_axis',(1.,-1.22464679915E-16,0.));
#45288=DIRECTION('center_axis',(-1.22464679915E-16,-1.,1.23259516441E-32));
#45289=DIRECTION('ref_axis',(1.,-1.22464679915E-16,-1.1821919162786E-48));
#45290=DIRECTION('center_axis',(1.22464679915E-16,1.,-1.23259516441E-32));
#45291=DIRECTION('ref_axis',(1.,-1.22464679915E-16,1.50949372274247E-48));
#45292=DIRECTION('center_axis',(-2.24037888703029E-16,-1.,-2.20413632410453E-17));
#45293=DIRECTION('ref_axis',(0.977255721664238,-2.19472257881379E-16,0.212064269679052));
#45294=DIRECTION('center_axis',(-1.22464679915E-16,-1.,-5.47382212627E-48));
#45295=DIRECTION('ref_axis',(1.,-1.22464679915E-16,5.24998673990483E-64));
#45296=DIRECTION('center_axis',(0.212064269679051,-2.59703829076063E-17,
-0.977255721664238));
#45297=DIRECTION('ref_axis',(0.977255721664238,-7.13089940857179E-32,0.212064269679051));
#45298=DIRECTION('center_axis',(-0.458332816460024,-1.74027459110009E-14,
-0.888780641866047));
#45299=DIRECTION('ref_axis',(0.888780641866047,-1.15648231731787E-14,-0.458332816460024));
#45300=DIRECTION('center_axis',(-1.17653265936146E-16,-1.,2.37924056871716E-17));
#45301=DIRECTION('ref_axis',(0.198212453337067,0.,0.980159080630334));
#45302=DIRECTION('center_axis',(-1.22464679915E-16,-1.,-5.47382212627E-48));
#45303=DIRECTION('ref_axis',(1.,-1.22464679915E-16,5.63840144221543E-64));
#45304=DIRECTION('center_axis',(0.980159080630334,-5.75630344056195E-15,
-0.198212453337067));
#45305=DIRECTION('ref_axis',(0.198212453337067,2.31296463463575E-14,0.980159080630334));
#45306=DIRECTION('center_axis',(-1.22464679915E-16,-1.,-5.47382212627E-48));
#45307=DIRECTION('ref_axis',(1.,-1.22464679915E-16,5.40238148608971E-64));
#45308=DIRECTION('center_axis',(0.611236780892201,-7.48549167240244E-17,
-0.791447785823259));
#45309=DIRECTION('ref_axis',(0.79144778582326,2.17825094235712E-31,0.611236780892201));
#45310=DIRECTION('center_axis',(-2.77602545911041E-17,-1.,-5.12739598421612E-17));
#45311=DIRECTION('ref_axis',(0.879386330848967,0.,-0.476108896278982));
#45312=DIRECTION('center_axis',(-1.22464679915E-16,-1.,-5.47382212627E-48));
#45313=DIRECTION('ref_axis',(1.,-1.22464679915E-16,5.24998673990483E-64));
#45314=DIRECTION('center_axis',(-0.559052990415089,-2.56753050562791E-11,
-0.829131927927001));
#45315=DIRECTION('ref_axis',(0.829131927927002,1.48029736616685E-14,-0.559052990415088));
#45316=DIRECTION('center_axis',(-5.0552016865731E-17,-1.,6.02936991345387E-17));
#45317=DIRECTION('ref_axis',(-0.766297237624136,0.,-0.642486220560113));
#45318=DIRECTION('center_axis',(-1.22464679915E-16,-1.,-5.47382212627E-48));
#45319=DIRECTION('ref_axis',(1.,-1.22464679915E-16,-6.703498746053E-64));
#45320=DIRECTION('center_axis',(-0.642486220560114,6.96862835096123E-15,
0.766297237624136));
#45321=DIRECTION('ref_axis',(0.766297237624136,1.15648231731787E-14,0.642486220560114));
#45322=DIRECTION('center_axis',(-1.22464679915E-16,-1.,-5.47382212627E-48));
#45323=DIRECTION('ref_axis',(1.,-1.22464679915E-16,-6.703498746053E-64));
#45324=DIRECTION('center_axis',(1.2246467991484E-16,1.,-6.47882833291866E-29));
#45325=DIRECTION('ref_axis',(0.926909189979645,-1.13513637260957E-16,0.375285695878857));
#45326=DIRECTION('center_axis',(-4.11884479880182E-8,-0.99999999999998,
-1.97187671260168E-7));
#45327=DIRECTION('ref_axis',(0.926909250500652,-1.12179643352301E-7,0.375285546399414));
#45328=DIRECTION('',(0.,1.,0.));
#45329=DIRECTION('center_axis',(-5.3135481018E-17,-1.,-1.71234534908E-16));
#45330=DIRECTION('ref_axis',(1.,-5.3135481018E-17,-9.09862937923009E-33));
#45331=DIRECTION('center_axis',(0.103350672077944,-0.961332021496742,-0.255263360132284));
#45332=DIRECTION('ref_axis',(0.843470154480493,-0.0513051793170642,0.534720372789271));
#45333=DIRECTION('center_axis',(-0.375285695878857,4.59592426223824E-17,
0.926909189979645));
#45334=DIRECTION('ref_axis',(0.926909189979645,-3.61589631838611E-32,0.375285695878857));
#45335=DIRECTION('center_axis',(-4.57540623410157E-17,-1.,5.92437539213873E-17));
#45336=DIRECTION('ref_axis',(0.791447868317764,0.,0.611236674075818));
#45337=DIRECTION('center_axis',(1.22464679915E-16,1.,0.));
#45338=DIRECTION('ref_axis',(1.,-1.22464679915E-16,0.));
#45339=DIRECTION('center_axis',(-4.57540783324772E-17,-1.,5.92437580993829E-17));
#45340=DIRECTION('ref_axis',(0.791447785823259,0.,0.611236780892201));
#45341=DIRECTION('center_axis',(-1.22464679915E-16,-1.,-5.47382212627E-48));
#45342=DIRECTION('ref_axis',(1.,-1.22464679915E-16,-6.703498746053E-64));
#45343=DIRECTION('center_axis',(-1.22464679915E-16,-1.,0.));
#45344=DIRECTION('ref_axis',(1.,-1.22464679915E-16,0.));
#45345=DIRECTION('center_axis',(-1.22464679914331E-16,-1.,1.45068233549706E-28));
#45346=DIRECTION('ref_axis',(0.977255721664238,-1.19679309148029E-16,0.212064269679051));
#45347=DIRECTION('',(0.,-1.,0.));
#45348=DIRECTION('center_axis',(-0.522520932310171,-1.21282901894159E-7,
-0.852626457071146));
#45349=DIRECTION('ref_axis',(0.602898361866691,-0.707106350234053,-0.369478246608833));
#45350=DIRECTION('center_axis',(7.05590196885209E-7,0.999999999999712,2.79920545343458E-7));
#45351=DIRECTION('ref_axis',(-0.0522188519509896,-2.42693529929814E-7,0.998635665045497));
#45352=DIRECTION('center_axis',(3.34362886570006E-17,1.,5.45598660992754E-17));
#45353=DIRECTION('ref_axis',(0.852626520482788,0.,-0.52252082883787));
#45354=DIRECTION('center_axis',(-0.496495508439081,-1.68003954310796E-11,
-0.868039290642894));
#45355=DIRECTION('ref_axis',(0.868039290642894,-1.4802973661669E-14,-0.49649550843908));
#45356=DIRECTION('center_axis',(-4.27856758992442E-7,-0.999999999999565,
-8.29299662254113E-7));
#45357=DIRECTION('ref_axis',(0.900769689431461,-7.45562834001725E-7,0.434297094856728));
#45358=DIRECTION('center_axis',(0.707141467397435,0.692946912637,-0.140625464812931));
#45359=DIRECTION('ref_axis',(-0.32401455277391,0.140799773673971,-0.935515896884752));
#45360=DIRECTION('center_axis',(-1.22464679915E-16,-1.,1.23259516441E-32));
#45361=DIRECTION('ref_axis',(1.,-1.22464679915E-16,1.50949372274247E-48));
#45362=DIRECTION('center_axis',(-1.22464679914984E-16,-1.,7.84281471797691E-29));
#45363=DIRECTION('ref_axis',(-0.195045334687923,2.38861644813906E-17,-0.980794227866618));
#45364=DIRECTION('',(0.,1.,0.));
#45365=DIRECTION('center_axis',(1.22464679914868E-16,1.,-1.10437102855485E-28));
#45366=DIRECTION('ref_axis',(0.766297237624135,-9.38443459252164E-17,0.642486220560115));
#45367=DIRECTION('',(0.,-1.,0.));
#45368=DIRECTION('center_axis',(4.21917049212E-17,1.,9.57420673393E-17));
#45369=DIRECTION('ref_axis',(1.,-4.21917049212E-17,-4.03952105372541E-33));
#45370=DIRECTION('center_axis',(-0.258465262671631,0.964605492283562,0.0522680805891321));
#45371=DIRECTION('ref_axis',(-0.945466832487627,-0.263697258719896,0.191196821127928));
#45372=DIRECTION('center_axis',(-2.17357452795E-16,2.66186108837E-32,1.));
#45373=DIRECTION('ref_axis',(1.,5.7857534586223E-48,2.17357452795E-16));
#45374=DIRECTION('center_axis',(1.22464679915E-16,1.,0.));
#45375=DIRECTION('ref_axis',(1.,-1.22464679915E-16,0.));
#45376=DIRECTION('center_axis',(-0.198212453337055,3.33211467677212E-15,
-0.980159080630336));
#45377=DIRECTION('ref_axis',(0.945466832487629,0.263697258719893,-0.191196821127922));
#45378=DIRECTION('center_axis',(2.17357452795E-16,-2.66186108837E-32,-1.));
#45379=DIRECTION('ref_axis',(-1.,-5.7857534586223E-48,-2.17357452795E-16));
#45380=DIRECTION('',(-9.00454292637E-17,0.,1.));
#45381=DIRECTION('center_axis',(2.17357452795E-16,-2.66186108837E-32,-1.));
#45382=DIRECTION('ref_axis',(1.,5.7857534586223E-48,2.17357452795E-16));
#45383=DIRECTION('',(-9.00454292637E-17,0.,1.));
#45384=DIRECTION('center_axis',(-1.22464679914984E-16,-1.,8.09446956404351E-29));
#45385=DIRECTION('ref_axis',(0.198212453337068,-2.42740246530083E-17,0.980159080630333));
#45386=DIRECTION('',(0.,-1.,0.));
#45387=DIRECTION('center_axis',(-1.86287635502571E-7,0.999999999999971,
-1.51799658010565E-7));
#45388=DIRECTION('ref_axis',(0.198212596438356,1.85712364005507E-7,0.980159051691679));
#45389=DIRECTION('',(-1.16865581539E-16,-1.,0.));
#45390=DIRECTION('center_axis',(1.,-1.22464679915E-16,6.12323399574E-17));
#45391=DIRECTION('ref_axis',(-1.22464679915E-16,-1.,-6.67366607695787E-50));
#45392=DIRECTION('',(2.17371312249E-16,0.,-1.));
#45393=DIRECTION('center_axis',(0.987243152768062,-3.98507192708808E-11,
-0.159219839569627));
#45394=DIRECTION('ref_axis',(-0.112585427377888,0.707106786546493,-0.6980863227152));
#45395=DIRECTION('center_axis',(2.17357452795E-16,-2.66186108837E-32,-1.));
#45396=DIRECTION('ref_axis',(1.,5.7857534586223E-48,2.17357452795E-16));
#45397=DIRECTION('center_axis',(-1.38777878078E-16,1.69953884181E-32,1.));
#45398=DIRECTION('ref_axis',(1.,2.35858394177534E-48,1.38777878078E-16));
#45399=DIRECTION('center_axis',(-0.941574524866389,0.336804706456248,-6.18995477252445E-5));
#45400=DIRECTION('ref_axis',(0.257425228288326,0.719541944518793,-0.644974140503957));
#45401=DIRECTION('',(1.29439338185998E-7,0.,0.999999999999992));
#45402=DIRECTION('',(0.,0.,1.));
#45403=DIRECTION('center_axis',(0.734238830876792,-8.99183234042744E-17,
0.678891257295808));
#45404=DIRECTION('ref_axis',(0.678891257295808,1.51038693775819E-31,-0.734238830876792));
#45405=DIRECTION('center_axis',(-0.734238830876792,8.99183234042744E-17,
-0.678891257295808));
#45406=DIRECTION('ref_axis',(0.678891257295808,1.51038693775819E-31,-0.734238830876792));
#45407=DIRECTION('center_axis',(-0.734238830876792,8.99183234042744E-17,
-0.678891257295808));
#45408=DIRECTION('ref_axis',(0.678891257295807,3.46311205996404E-31,-0.734238830876791));
#45409=DIRECTION('',(0.734238830876791,0.,0.678891257295807));
#45410=DIRECTION('center_axis',(1.,0.,0.));
#45411=DIRECTION('ref_axis',(0.,-1.,0.));
#45412=DIRECTION('center_axis',(-0.790681776842983,9.68305907154979E-17,
0.612227349738987));
#45413=DIRECTION('ref_axis',(0.612227349738987,1.22226555802243E-31,0.790681776842983));
#45414=DIRECTION('center_axis',(7.65621835198448E-17,1.,-5.92823359275332E-17));
#45415=DIRECTION('ref_axis',(0.612227349738987,0.,0.790681776842983));
#45416=DIRECTION('center_axis',(-0.991694064582439,1.21447496192053E-16,
0.128619136492057));
#45417=DIRECTION('ref_axis',(0.128619136492057,-4.98879909760123E-32,0.991694064582438));
#45418=DIRECTION('center_axis',(1.22464679915E-16,1.,5.47382212627E-48));
#45419=DIRECTION('ref_axis',(1.,-1.22464679915E-16,-6.703498746053E-64));
#45420=DIRECTION('center_axis',(-1.22464679915E-16,-1.,-5.47382212627E-48));
#45421=DIRECTION('ref_axis',(1.,-1.22464679915E-16,-6.703498746053E-64));
#45422=DIRECTION('center_axis',(0.,0.,1.));
#45423=DIRECTION('ref_axis',(1.,0.,0.));
#45424=DIRECTION('center_axis',(1.22464679915E-16,1.,5.47382212627E-48));
#45425=DIRECTION('ref_axis',(1.,-1.22464679915E-16,-6.703498746053E-64));
#45426=DIRECTION('center_axis',(-2.17357452795E-16,2.66186108837E-32,1.));
#45427=DIRECTION('ref_axis',(1.,5.7857534586223E-48,2.17357452795E-16));
#45428=DIRECTION('center_axis',(2.17357452795E-16,-2.66186108837E-32,-1.));
#45429=DIRECTION('ref_axis',(-1.,-5.7857534586223E-48,-2.17357452795E-16));
#45430=DIRECTION('',(-5.32230154418998E-8,0.,0.999999999999999));
#45431=DIRECTION('center_axis',(-1.20274161001E-14,1.4729336629E-30,1.));
#45432=DIRECTION('ref_axis',(1.,6.81368694281801E-46,1.20274161001E-14));
#45433=DIRECTION('center_axis',(0.,0.,1.));
#45434=DIRECTION('ref_axis',(1.,0.,0.));
#45435=DIRECTION('center_axis',(0.824331881335686,-1.00951539990962E-16,
-0.566106835688784));
#45436=DIRECTION('ref_axis',(0.566106835688784,-1.17683260639136E-31,0.824331881335686));
#45437=DIRECTION('center_axis',(1.,0.,0.));
#45438=DIRECTION('ref_axis',(0.,-1.,0.));
#45439=DIRECTION('center_axis',(1.22464679915E-16,1.,5.47382212627E-48));
#45440=DIRECTION('ref_axis',(1.,-1.22464679915E-16,-6.703498746053E-64));
#45441=DIRECTION('center_axis',(0.99733341416283,-1.22138117333977E-16,
-0.0729798670477863));
#45442=DIRECTION('ref_axis',(0.0729798670477863,2.52018738244318E-32,0.99733341416283));
#45443=DIRECTION('center_axis',(8.32175728849317E-17,1.,-5.71493568625004E-17));
#45444=DIRECTION('ref_axis',(0.566106835688784,0.,0.824331881335686));
#45445=DIRECTION('center_axis',(-1.22464679915E-16,-1.,-5.47382212627E-48));
#45446=DIRECTION('ref_axis',(1.,-1.22464679915E-16,6.49622071350503E-64));
#45447=DIRECTION('center_axis',(1.22464679915E-16,1.,5.47382212627E-48));
#45448=DIRECTION('ref_axis',(1.,-1.22464679915E-16,6.2417319857974E-64));
#45449=DIRECTION('center_axis',(1.22464679915E-16,1.,5.47382212627E-48));
#45450=DIRECTION('ref_axis',(1.,-1.22464679915E-16,0.));
#45451=DIRECTION('center_axis',(0.,0.,1.));
#45452=DIRECTION('ref_axis',(1.,0.,0.));
#45453=DIRECTION('center_axis',(-1.,1.22464679915E-16,-6.12323399574E-17));
#45454=DIRECTION('ref_axis',(1.22464679915E-16,1.,7.49879891332945E-33));
#45455=DIRECTION('center_axis',(-1.,1.22464679915E-16,-6.12323399574E-17));
#45456=DIRECTION('ref_axis',(-6.12323399574E-17,0.,1.));
#45457=DIRECTION('',(-7.55253758248E-17,-1.,0.));
#45458=DIRECTION('',(-2.28870415168E-16,0.,1.));
#45459=DIRECTION('',(1.5105075165E-16,1.,0.));
#45460=DIRECTION('center_axis',(1.22464679914868E-16,1.,-1.27704300324719E-28));
#45461=DIRECTION('ref_axis',(-0.718198537785833,8.79539540451795E-17,-0.695838242928838));
#45462=DIRECTION('',(1.5105075165E-16,1.,0.));
#45463=DIRECTION('',(1.5105075165E-16,1.,0.));
#45464=DIRECTION('center_axis',(1.22464679914988E-16,1.,-5.97423468748921E-29));
#45465=DIRECTION('ref_axis',(-0.191153986297933,2.34096117463918E-17,-0.981560061087659));
#45466=DIRECTION('center_axis',(-1.69719902425E-16,-1.,-3.8940254264E-17));
#45467=DIRECTION('ref_axis',(1.,-1.69719902425E-16,-6.60893615409077E-33));
#45468=DIRECTION('',(1.23358113847E-16,1.,0.));
#45469=DIRECTION('center_axis',(-1.,1.22464679915E-16,-6.12323399574E-17));
#45470=DIRECTION('ref_axis',(-6.12323399574E-17,0.,1.));
#45471=DIRECTION('',(-1.74378361673E-16,0.,1.));
#45472=DIRECTION('',(-1.5105075165E-16,-1.,0.));
#45473=DIRECTION('center_axis',(1.22464679915E-16,1.,3.08148791102006E-33));
#45474=DIRECTION('ref_axis',(-1.,1.22464679915E-16,-5.78241158658936E-15));
#45475=DIRECTION('center_axis',(8.30969430144E-17,1.,4.68996881439E-17));
#45476=DIRECTION('ref_axis',(1.,-8.30969430144E-17,-3.89722071308679E-33));
#45477=DIRECTION('',(-1.75298372309E-16,-1.,0.));
#45478=DIRECTION('center_axis',(1.22464679915001E-16,1.,1.11184889946404E-29));
#45479=DIRECTION('ref_axis',(0.11782622263506,-1.44295506406073E-17,0.993034229651503));
#45480=DIRECTION('center_axis',(1.22464679915E-16,1.,0.));
#45481=DIRECTION('ref_axis',(1.,-1.22464679915E-16,0.));
#45482=DIRECTION('',(0.,1.,0.));
#45483=DIRECTION('center_axis',(1.224646799149E-16,1.,1.07595286226434E-28));
#45484=DIRECTION('ref_axis',(0.678891257295807,-8.31402005216763E-17,-0.734238830876792));
#45485=DIRECTION('',(1.23358113847E-16,1.,0.));
#45486=DIRECTION('center_axis',(-1.224646799149E-16,-1.,-1.07595286226434E-28));
#45487=DIRECTION('ref_axis',(0.678891257295809,-8.31402005216765E-17,-0.73423883087679));
#45488=DIRECTION('',(2.46716227694E-16,1.,0.));
#45489=DIRECTION('center_axis',(0.678891257295808,-8.31402005216764E-17,
-0.734238830876792));
#45490=DIRECTION('ref_axis',(4.92781901212525E-33,-1.,1.13233183843457E-16));
#45491=DIRECTION('center_axis',(1.22464679915001E-16,1.,1.11184889946404E-29));
#45492=DIRECTION('ref_axis',(0.11782622263506,-1.44295506406073E-17,0.993034229651503));
#45493=DIRECTION('',(0.,1.,0.));
#45494=DIRECTION('',(0.,1.,0.));
#45495=DIRECTION('center_axis',(-1.22464679914738E-16,-1.,-8.77635576046461E-30));
#45496=DIRECTION('ref_axis',(-0.999438196720723,1.22395878855966E-16,0.0335155327516906));
#45497=DIRECTION('',(0.,1.,0.));
#45498=DIRECTION('center_axis',(1.22464679914868E-16,1.,-1.27704300324719E-28));
#45499=DIRECTION('ref_axis',(-0.718198537785833,8.79539540451795E-17,-0.695838242928838));
#45500=DIRECTION('',(0.,1.,0.));
#45501=DIRECTION('center_axis',(1.22464679915E-16,1.,1.94567767731298E-44));
#45502=DIRECTION('ref_axis',(-2.38276793969895E-60,-1.94567767731298E-44,
1.));
#45503=DIRECTION('',(0.,1.,0.));
#45504=DIRECTION('center_axis',(-1.22464679915E-16,-1.,5.12446785619646E-33));
#45505=DIRECTION('ref_axis',(-2.89120579329468E-15,3.59195059900423E-31,
1.));
#45506=DIRECTION('',(0.,1.,0.));
#45507=DIRECTION('center_axis',(-2.17357452795E-16,2.66186108837E-32,1.));
#45508=DIRECTION('ref_axis',(1.,2.56447231488414E-65,2.17357452795E-16));
#45509=DIRECTION('center_axis',(1.22464679914868E-16,1.,-1.27704300324719E-28));
#45510=DIRECTION('ref_axis',(0.714687205042302,-8.75239398046679E-17,0.699444207173684));
#45511=DIRECTION('',(0.,1.,0.));
#45512=DIRECTION('',(0.,-1.,0.));
#45513=DIRECTION('center_axis',(1.22464679914919E-16,1.,-1.07732241244701E-28));
#45514=DIRECTION('ref_axis',(-0.602966636474876,7.38421161351848E-17,-0.797766403966835));
#45515=DIRECTION('',(-2.46716227694E-16,-1.,0.));
#45516=DIRECTION('center_axis',(0.678891257295808,-8.31402005216764E-17,
-0.734238830876792));
#45517=DIRECTION('ref_axis',(4.92781901212525E-33,-1.,1.13233183843457E-16));
#45518=DIRECTION('',(0.,-1.,0.));
#45519=DIRECTION('center_axis',(-1.22464679914841E-16,-1.,1.13510031077863E-28));
#45520=DIRECTION('ref_axis',(0.813441648140047,-9.96178710688057E-17,0.581646529321034));
#45521=DIRECTION('center_axis',(1.28693262473E-16,1.,6.09147290561E-17));
#45522=DIRECTION('ref_axis',(1.,-1.28693262473E-16,-7.83931521488836E-33));
#45523=DIRECTION('',(0.,-1.,0.));
#45524=DIRECTION('center_axis',(1.22464679915001E-16,1.,1.11184889946404E-29));
#45525=DIRECTION('ref_axis',(0.11782622263506,-1.44295506406073E-17,0.993034229651503));
#45526=DIRECTION('center_axis',(1.22464679915E-16,1.,0.));
#45527=DIRECTION('ref_axis',(1.,-1.22464679915E-16,0.));
#45528=DIRECTION('',(0.,-1.,0.));
#45529=DIRECTION('center_axis',(1.22464679915E-16,1.,1.94567767731298E-44));
#45530=DIRECTION('ref_axis',(2.38276793969895E-60,1.94567767731298E-44,
-1.));
#45531=DIRECTION('',(0.,1.,0.));
#45532=DIRECTION('center_axis',(-1.50336151828E-16,-1.,-5.4521376634E-17));
#45533=DIRECTION('ref_axis',(1.,-1.50336151828E-16,-8.19653395552059E-33));
#45534=DIRECTION('center_axis',(1.22464679914423E-16,1.,-8.33007499390688E-29));
#45535=DIRECTION('ref_axis',(0.98972556641388,-1.21206424693985E-16,0.142980079684982));
#45536=DIRECTION('center_axis',(-1.64046831707E-17,1.,1.20249303974E-16));
#45537=DIRECTION('ref_axis',(1.,1.64046831707E-17,1.97265173319067E-33));
#45538=DIRECTION('',(0.,-1.,0.));
#45539=DIRECTION('center_axis',(-2.17357452795E-16,2.66186108837E-32,1.));
#45540=DIRECTION('ref_axis',(1.,2.56447231488414E-65,2.17357452795E-16));
#45541=DIRECTION('',(-1.,0.,0.));
#45542=DIRECTION('center_axis',(0.,1.,0.));
#45543=DIRECTION('ref_axis',(0.10172047258397,0.,0.994813020349701));
#45544=DIRECTION('center_axis',(0.581646529321033,-7.12311560368041E-17,
-0.813441648140047));
#45545=DIRECTION('ref_axis',(0.813441648140047,-2.80119922649672E-32,0.581646529321033));
#45546=DIRECTION('center_axis',(1.69872863391202E-17,1.,-4.23293596334453E-17));
#45547=DIRECTION('ref_axis',(0.927897590989264,0.,0.372835165503899));
#45548=DIRECTION('center_axis',(1.22464679915E-16,1.,5.47382212627E-48));
#45549=DIRECTION('ref_axis',(1.,-1.22464679915E-16,-6.703498746053E-64));
#45550=DIRECTION('center_axis',(0.,0.,1.));
#45551=DIRECTION('ref_axis',(1.,0.,0.));
#45552=DIRECTION('center_axis',(1.,-1.22464679915E-16,6.12323399574E-17));
#45553=DIRECTION('ref_axis',(-1.22464679915E-16,-1.,-7.49879891332945E-33));
#45554=DIRECTION('center_axis',(0.,0.,1.));
#45555=DIRECTION('ref_axis',(1.,0.,0.));
#45556=DIRECTION('center_axis',(-1.,1.22464679915E-16,-6.12323399574E-17));
#45557=DIRECTION('ref_axis',(-1.22464679915E-16,-1.,-7.49879891332945E-33));
#45558=DIRECTION('center_axis',(-1.,1.22464679915E-16,-6.12323399574E-17));
#45559=DIRECTION('ref_axis',(1.22464679915E-16,1.,7.49879891332945E-33));
#45560=DIRECTION('',(-1.,0.,-2.89652532403E-16));
#45561=DIRECTION('center_axis',(1.22464679915E-16,1.,5.47382212627E-48));
#45562=DIRECTION('ref_axis',(1.,-1.22464679915E-16,0.));
#45563=DIRECTION('',(-1.74378361673E-16,0.,1.));
#45564=DIRECTION('center_axis',(1.22464679915E-16,1.,0.));
#45565=DIRECTION('ref_axis',(1.,-1.22464679915E-16,0.));
#45566=DIRECTION('center_axis',(0.62218556523187,0.249390626342792,-0.742084522079155));
#45567=DIRECTION('ref_axis',(-0.160230040961959,0.968402971645766,0.191107348055953));
#45568=DIRECTION('center_axis',(0.,1.,0.));
#45569=DIRECTION('ref_axis',(-0.751205410155072,0.,0.660068505349066));
#45570=DIRECTION('center_axis',(-1.22464679915E-16,-1.,-5.47382212627E-48));
#45571=DIRECTION('ref_axis',(1.,-1.22464679915E-16,-6.703498746053E-64));
#45572=DIRECTION('center_axis',(2.17357452795E-16,-2.66186108837E-32,-1.));
#45573=DIRECTION('ref_axis',(1.,5.7857534586223E-48,2.17357452795E-16));
#45574=DIRECTION('center_axis',(-0.991694064582439,1.21447496192053E-16,
-0.128619136492057));
#45575=DIRECTION('ref_axis',(0.128619136492057,-4.98879909760123E-32,-0.991694064582438));
#45576=DIRECTION('center_axis',(1.22464679915E-16,1.,5.47382212627E-48));
#45577=DIRECTION('ref_axis',(1.,-1.22464679915E-16,0.));
#45578=DIRECTION('center_axis',(1.22464679915E-16,1.,5.47382212627E-48));
#45579=DIRECTION('ref_axis',(1.,-1.22464679915E-16,0.));
#45580=DIRECTION('center_axis',(1.22464679915E-16,1.,7.60253073092891E-48));
#45581=DIRECTION('ref_axis',(-1.,1.22464679915E-16,9.3104149250716E-64));
#45582=DIRECTION('',(1.75298372309E-16,1.,0.));
#45583=DIRECTION('center_axis',(-1.22464679915E-16,-1.,-1.94578320706031E-44));
#45584=DIRECTION('ref_axis',(-2.38289717636624E-60,-1.94578320706031E-44,
1.));
#45585=DIRECTION('center_axis',(1.22464679915E-16,1.,-1.23259516441E-32));
#45586=DIRECTION('ref_axis',(1.,-1.22464679915E-16,1.50949372274247E-48));
#45587=DIRECTION('center_axis',(0.,0.,1.));
#45588=DIRECTION('ref_axis',(1.,0.,0.));
#45589=DIRECTION('center_axis',(2.17357452795E-16,-2.66186108837E-32,-1.));
#45590=DIRECTION('ref_axis',(1.,5.7857534586223E-48,2.17357452795E-16));
#45591=DIRECTION('center_axis',(1.69872863391202E-17,1.,-4.23293596334453E-17));
#45592=DIRECTION('ref_axis',(-0.928056183869048,0.,-0.37244022283102));
#45593=DIRECTION('center_axis',(-1.22464679914985E-16,-1.,-5.43497430306078E-29));
#45594=DIRECTION('ref_axis',(0.269603455472075,-3.30169008783092E-17,-0.962971430935268));
#45595=DIRECTION('center_axis',(-4.73893099620284E-8,0.999999999999998,
3.5943940930386E-8));
#45596=DIRECTION('ref_axis',(0.604316184158962,-1.36908907673765E-14,0.796744594938398));
#45597=DIRECTION('center_axis',(-2.17357452795E-16,2.66186108836794E-32,
1.));
#45598=DIRECTION('ref_axis',(5.78575345861782E-48,1.,-2.66186108836794E-32));
#45599=DIRECTION('center_axis',(2.17357452795E-16,-2.66186108837E-32,-1.));
#45600=DIRECTION('ref_axis',(-1.,-5.7857534586223E-48,-2.17357452795E-16));
#45601=DIRECTION('',(0.,0.,1.));
#45602=DIRECTION('center_axis',(0.,1.,0.));
#45603=DIRECTION('ref_axis',(-0.642923934113106,0.,0.765930032669124));
#45604=DIRECTION('center_axis',(9.19369336238712E-17,1.,-5.29776121060009E-17));
#45605=DIRECTION('ref_axis',(0.499277443708891,0.,0.86644217014381));
#45606=DIRECTION('center_axis',(0.,-1.,5.47382212627E-48));
#45607=DIRECTION('ref_axis',(1.,0.,0.));
#45608=DIRECTION('center_axis',(-1.22464679915E-16,-1.,-5.47382212627E-48));
#45609=DIRECTION('ref_axis',(1.,-1.22464679915E-16,-6.703498746053E-64));
#45610=DIRECTION('center_axis',(-1.,1.22464679915E-16,-6.12323399574E-17));
#45611=DIRECTION('ref_axis',(1.22464679915E-16,1.,7.49879891332945E-33));
#45612=DIRECTION('center_axis',(1.,0.,0.));
#45613=DIRECTION('ref_axis',(0.,-1.,0.));
#45614=DIRECTION('center_axis',(-1.22464679915E-16,-1.,0.));
#45615=DIRECTION('ref_axis',(1.,-1.22464679915E-16,0.));
#45616=DIRECTION('center_axis',(-0.827537346623811,1.01344096271977E-16,
-0.561410669601872));
#45617=DIRECTION('ref_axis',(0.561410669601872,-1.40589310424814E-31,-0.827537346623811));
#45618=DIRECTION('center_axis',(-0.687199008140201,8.41576065696246E-17,
0.726469216974212));
#45619=DIRECTION('ref_axis',(0.726469216974212,1.50838013754883E-32,0.687199008140201));
#45620=DIRECTION('center_axis',(-1.22464679914912E-16,-1.,8.35682402091226E-29));
#45621=DIRECTION('ref_axis',(0.726469216974212,-8.89668201247259E-17,0.687199008140201));
#45622=DIRECTION('',(0.,1.,0.));
#45623=DIRECTION('',(0.,1.,0.));
#45624=DIRECTION('center_axis',(1.22464679914998E-16,1.,-1.73663083545565E-29));
#45625=DIRECTION('ref_axis',(0.095298509688002,-1.16707014853003E-17,0.99544874004202));
#45626=DIRECTION('center_axis',(-1.22464679915E-16,-1.,0.));
#45627=DIRECTION('ref_axis',(1.,-1.22464679915E-16,0.));
#45628=DIRECTION('center_axis',(1.68490994230906E-17,1.,-4.21844451941189E-17));
#45629=DIRECTION('ref_axis',(-0.928663912412966,0.,-0.370922279974987));
#45630=DIRECTION('center_axis',(-1.22464679915E-16,-1.,-5.47382212627E-48));
#45631=DIRECTION('ref_axis',(1.,-1.22464679915E-16,-6.703498746053E-64));
#45632=DIRECTION('center_axis',(2.17357452795E-16,-2.66186108837E-32,-1.));
#45633=DIRECTION('ref_axis',(-1.,-5.7857534586223E-48,-2.17357452795E-16));
#45634=DIRECTION('center_axis',(2.74323727954E-15,-3.35949675369E-31,1.));
#45635=DIRECTION('ref_axis',(1.,-4.97099741607164E-47,-2.74323727954E-15));
#45636=DIRECTION('center_axis',(-2.17357452795E-16,5.59737441582E-15,1.));
#45637=DIRECTION('ref_axis',(1.,1.21663104536254E-30,2.17357452795E-16));
#45638=DIRECTION('',(0.,0.,-1.));
#45639=DIRECTION('center_axis',(2.68354439599323E-46,1.,-1.81284143127026E-31));
#45640=DIRECTION('ref_axis',(1.,0.,1.97372982155583E-15));
#45641=DIRECTION('center_axis',(-0.904759192693671,1.1080104493296E-16,
-0.425923471102845));
#45642=DIRECTION('ref_axis',(0.425923471102845,3.65487816993661E-32,-0.904759192693671));
#45643=DIRECTION('center_axis',(1.22464679915E-16,1.,5.47382212627E-48));
#45644=DIRECTION('ref_axis',(1.,-1.22464679915E-16,-6.703498746053E-64));
#45645=DIRECTION('center_axis',(1.0293130162049E-16,1.,4.48396705262131E-17));
#45646=DIRECTION('ref_axis',(0.399377187820903,0.,-0.916786704663777));
#45647=DIRECTION('center_axis',(-0.916786704663777,1.12273990336973E-16,
-0.399377187820903));
#45648=DIRECTION('ref_axis',(0.399377187820903,3.93858763528754E-32,-0.916786704663777));
#45649=DIRECTION('center_axis',(-1.22464679915E-16,-1.,-5.47382212627E-48));
#45650=DIRECTION('ref_axis',(1.,-1.22464679915E-16,-6.703498746053E-64));
#45651=DIRECTION('center_axis',(1.0293130162049E-16,1.,4.48396705262131E-17));
#45652=DIRECTION('ref_axis',(-0.399377187820903,0.,0.916786704663777));
#45653=DIRECTION('center_axis',(2.17357452795E-16,-2.66186108837E-32,-1.));
#45654=DIRECTION('ref_axis',(1.,5.7857534586223E-48,2.17357452795E-16));
#45655=DIRECTION('center_axis',(1.22464679915E-16,1.,5.47382212627E-48));
#45656=DIRECTION('ref_axis',(1.,-1.22464679915E-16,-6.703498746053E-64));
#45657=DIRECTION('center_axis',(2.17357452795E-16,-2.66186108836821E-32,
-1.));
#45658=DIRECTION('ref_axis',(5.78575345861839E-48,1.,-2.66186108836821E-32));
#45659=DIRECTION('center_axis',(8.746404436E-17,5.79129605623E-15,-1.));
#45660=DIRECTION('ref_axis',(1.,-5.06530175163994E-31,8.746404436E-17));
#45661=DIRECTION('',(0.,0.,1.));
#45662=DIRECTION('center_axis',(0.,0.957608642877659,-0.288072364321897));
#45663=DIRECTION('ref_axis',(0.,-0.288072364321899,-0.957608642877659));
#45664=DIRECTION('center_axis',(1.22464679915E-16,1.,5.47382212627E-48));
#45665=DIRECTION('ref_axis',(1.,-1.22464679915E-16,-6.703498746053E-64));
#45666=DIRECTION('center_axis',(-0.890715300400791,1.09081164158974E-16,
-0.454561605980893));
#45667=DIRECTION('ref_axis',(0.454561605980893,-9.65132779741589E-32,-0.890715300400791));
#45668=DIRECTION('center_axis',(-1.,1.2919345348203E-16,-3.88645861503935E-17));
#45669=DIRECTION('ref_axis',(0.,0.288072364321903,0.957608642877657));
#45670=DIRECTION('center_axis',(1.178693242477E-16,1.,2.32734068666895E-17));
#45671=DIRECTION('ref_axis',(0.193710935823942,0.,-0.981058649287703));
#45672=DIRECTION('center_axis',(-1.22464679915E-16,-1.,-5.47382212627E-48));
#45673=DIRECTION('ref_axis',(1.,-1.22464679915E-16,6.22660996643423E-64));
#45674=DIRECTION('center_axis',(-1.22464679915E-16,-1.,-5.47382212627E-48));
#45675=DIRECTION('ref_axis',(1.,-1.22464679915E-16,6.49622071350503E-64));
#45676=DIRECTION('center_axis',(0.684308456885095,0.684308456885093,0.25188066950658));
#45677=DIRECTION('ref_axis',(0.178106529457909,0.178106529457906,-0.967758300573505));
#45678=DIRECTION('center_axis',(0.938446715307966,-1.14926576606996E-16,
0.345424032932987));
#45679=DIRECTION('ref_axis',(0.345424032932987,5.96953449650393E-32,-0.938446715307966));
#45680=DIRECTION('center_axis',(1.178693242477E-16,1.,2.32734068666895E-17));
#45681=DIRECTION('ref_axis',(0.193710935823942,0.,-0.981058649287703));
#45682=DIRECTION('center_axis',(-1.22464679915E-16,-1.,-5.47382212627E-48));
#45683=DIRECTION('ref_axis',(1.,-1.22464679915E-16,6.22660996643423E-64));
#45684=DIRECTION('center_axis',(-1.22464679915E-16,-1.,-5.47382212627E-48));
#45685=DIRECTION('ref_axis',(1.,-1.22464679915E-16,6.49622071350503E-64));
#45686=DIRECTION('center_axis',(-1.22464679915E-16,-1.,-7.60253073092891E-48));
#45687=DIRECTION('ref_axis',(-1.,1.22464679915E-16,9.3104149250716E-64));
#45688=DIRECTION('',(-1.38777878078E-16,-1.,0.));
#45689=DIRECTION('center_axis',(1.22464679914586E-16,1.,-1.3947821589454E-28));
#45690=DIRECTION('ref_axis',(0.947590338356885,-1.16046347476986E-16,0.319487950715961));
#45691=DIRECTION('',(0.,-1.,0.));
#45692=DIRECTION('center_axis',(1.22464679914586E-16,1.,-1.3947821589454E-28));
#45693=DIRECTION('ref_axis',(0.947590338356885,-1.16046347476986E-16,0.319487950715961));
#45694=DIRECTION('',(1.21655932081E-16,1.,0.));
#45695=DIRECTION('center_axis',(-1.22464679914899E-16,-1.,-1.21650294976139E-28));
#45696=DIRECTION('ref_axis',(0.638858327474962,-7.82375805850953E-17,-0.769324403236954));
#45697=DIRECTION('',(0.,-1.,0.));
#45698=DIRECTION('center_axis',(1.83586547022E-16,1.,-3.67652253532E-18));
#45699=DIRECTION('ref_axis',(1.,-1.83586547022E-16,6.74960077307968E-34));
#45700=DIRECTION('center_axis',(0.,1.,0.));
#45701=DIRECTION('ref_axis',(0.998195841446114,0.,-0.0600421695118078));
#45702=DIRECTION('center_axis',(0.687199008140201,-8.41576065696246E-17,
-0.726469216974212));
#45703=DIRECTION('ref_axis',(0.726469216974212,1.50838013754883E-32,0.687199008140201));
#45704=DIRECTION('center_axis',(0.687199008140201,-8.41576065697951E-17,
-0.726469216974212));
#45705=DIRECTION('ref_axis',(5.78330237622164E-17,1.,-6.11379105471828E-17));
#45706=DIRECTION('',(0.687199008140201,0.,-0.726469216974212));
#45707=DIRECTION('',(0.687199008140201,0.,-0.726469216974212));
#45708=DIRECTION('center_axis',(-0.726469216974212,8.89668201247259E-17,
-0.687199008140201));
#45709=DIRECTION('ref_axis',(-0.687199008140201,2.45619021304035E-33,0.726469216974212));
#45710=DIRECTION('',(0.687199008140201,0.,-0.726469216974212));
#45711=DIRECTION('center_axis',(0.687199008140201,-8.41576065697951E-17,
-0.726469216974212));
#45712=DIRECTION('ref_axis',(-5.78330237622164E-17,-1.,6.11379105471828E-17));
#45713=DIRECTION('',(0.687199008140201,0.,-0.726469216974212));
#45714=DIRECTION('center_axis',(0.678891827805225,7.76974089072413E-7,-0.734238303372057));
#45715=DIRECTION('ref_axis',(0.519185258240454,-0.707106778553177,0.480048613527778));
#45716=DIRECTION('center_axis',(0.734238830876792,-8.99183234042744E-17,
0.678891257295808));
#45717=DIRECTION('ref_axis',(-0.678891257295808,-1.51038693775819E-31,0.734238830876792));
#45718=DIRECTION('center_axis',(0.734238830876792,-8.99183234042744E-17,
0.678891257295808));
#45719=DIRECTION('ref_axis',(0.678891257295808,1.51038693775819E-31,-0.734238830876792));
#45720=DIRECTION('',(-0.734238830876791,0.,-0.678891257295807));
#45721=DIRECTION('center_axis',(-6.60215246509141E-17,-1.,-6.10447636300053E-17));
#45722=DIRECTION('ref_axis',(0.678891257295808,0.,-0.734238830876791));
#45723=DIRECTION('center_axis',(0.790681776842983,-9.68305907154979E-17,
-0.612227349738987));
#45724=DIRECTION('ref_axis',(0.612227349738987,1.22226555802243E-31,0.790681776842983));
#45725=DIRECTION('center_axis',(1.22464679915E-16,1.,5.47382212627E-48));
#45726=DIRECTION('ref_axis',(1.,-1.22464679915E-16,-6.703498746053E-64));
#45727=DIRECTION('center_axis',(-1.20438761132693E-16,-1.,1.56204720894266E-17));
#45728=DIRECTION('ref_axis',(0.128619136492057,0.,0.991694064582438));
#45729=DIRECTION('center_axis',(0.991694064582439,-1.21447496192053E-16,
-0.128619136492057));
#45730=DIRECTION('ref_axis',(0.128619136492057,-7.10548517584315E-33,0.991694064582438));
#45731=DIRECTION('center_axis',(-1.22464679915E-16,-1.,-5.47382212627E-48));
#45732=DIRECTION('ref_axis',(1.,-1.22464679915E-16,-6.703498746053E-64));
#45733=DIRECTION('center_axis',(-1.20438761132693E-16,-1.,1.56204720894266E-17));
#45734=DIRECTION('ref_axis',(-0.128619136492057,0.,-0.991694064582438));
#45735=DIRECTION('center_axis',(2.17357452795E-16,-2.66186108837E-32,-1.));
#45736=DIRECTION('ref_axis',(1.,5.7857534586223E-48,2.17357452795E-16));
#45737=DIRECTION('center_axis',(1.22464679915E-16,1.,5.47382212627E-48));
#45738=DIRECTION('ref_axis',(1.,-1.22464679915E-16,-6.703498746053E-64));
#45739=DIRECTION('center_axis',(2.17357452795E-16,-2.66186108837E-32,-1.));
#45740=DIRECTION('ref_axis',(1.,5.7857534586223E-48,2.17357452795E-16));
#45741=DIRECTION('center_axis',(6.13854691746E-15,-7.51755183389E-31,-1.));
#45742=DIRECTION('ref_axis',(1.,2.67726580969963E-46,6.13854691746E-15));
#45743=DIRECTION('',(-5.89048887673E-17,0.,1.));
#45744=DIRECTION('center_axis',(-0.734238830876792,8.99183234042744E-17,
-0.678891257295808));
#45745=DIRECTION('ref_axis',(0.678891257295807,3.46311205996404E-31,-0.734238830876791));
#45746=DIRECTION('center_axis',(-8.32175728849317E-17,-1.,5.71493568625004E-17));
#45747=DIRECTION('ref_axis',(0.566106835688784,0.,0.824331881335687));
#45748=DIRECTION('center_axis',(1.22464679915E-16,1.,5.47382212627E-48));
#45749=DIRECTION('ref_axis',(1.,-1.22464679915E-16,-6.703498746053E-64));
#45750=DIRECTION('center_axis',(-0.824331881335686,1.00951539990962E-16,
0.566106835688784));
#45751=DIRECTION('ref_axis',(0.566106835688784,-1.17683260639136E-31,0.824331881335686));
#45752=DIRECTION('center_axis',(-1.07341775839004E-43,-1.,-3.62568286252829E-30));
#45753=DIRECTION('ref_axis',(-1.,0.,2.96059473233375E-14));
#45754=DIRECTION('center_axis',(-0.99733341416283,1.22138117333977E-16,
0.0729798670477863));
#45755=DIRECTION('ref_axis',(0.0729798670477863,-2.55070953490458E-32,0.99733341416283));
#45756=DIRECTION('center_axis',(1.22464679915E-16,1.,5.47382212627E-48));
#45757=DIRECTION('ref_axis',(1.,-1.22464679915E-16,-6.703498746053E-64));
#45758=DIRECTION('center_axis',(-1.21812425560124E-16,-1.,8.91362356450131E-18));
#45759=DIRECTION('ref_axis',(0.0729798670477876,0.,0.99733341416283));
#45760=DIRECTION('center_axis',(1.22464679915E-16,1.,5.47382212627E-48));
#45761=DIRECTION('ref_axis',(1.,-1.22464679915E-16,5.9677926224237E-64));
#45762=DIRECTION('center_axis',(-7.91623497736024E-17,-1.,5.85483919904324E-17));
#45763=DIRECTION('ref_axis',(-0.594634643326775,0.,-0.803996045360696));
#45764=DIRECTION('center_axis',(0.803996045360697,-9.84611183477626E-17,
-0.594634643326775));
#45765=DIRECTION('ref_axis',(0.594634643326775,4.97302608069436E-32,0.803996045360697));
#45766=DIRECTION('center_axis',(1.22464679915E-16,1.,5.47382212627E-48));
#45767=DIRECTION('ref_axis',(1.,-1.22464679915E-16,-6.703498746053E-64));
#45768=DIRECTION('center_axis',(-7.91623497736024E-17,-1.,5.85483919904324E-17));
#45769=DIRECTION('ref_axis',(0.594634643326775,0.,0.803996045360696));
#45770=DIRECTION('center_axis',(0.766648875028861,7.59597220210557E-12,
-0.642066587214272));
#45771=DIRECTION('ref_axis',(0.642066587214271,0.,0.766648875028862));
#45772=DIRECTION('center_axis',(-1.22464679915E-16,-1.,-5.47382212627E-48));
#45773=DIRECTION('ref_axis',(1.,-1.22464679915E-16,-6.703498746053E-64));
#45774=DIRECTION('center_axis',(-0.988161317760145,0.0726194459501342,0.135142984103609));
#45775=DIRECTION('ref_axis',(0.140217557783907,0.0700183990770855,0.987641868431973));
#45776=DIRECTION('center_axis',(-0.198845167758325,-4.16446674120852E-11,
0.980030917501669));
#45777=DIRECTION('ref_axis',(0.692986511637353,0.707106776997594,0.1406047673899));
#45778=DIRECTION('center_axis',(-0.204326613183897,-0.267662308375891,0.941598387753339));
#45779=DIRECTION('ref_axis',(-0.591797156233802,-0.732434393923313,-0.336624396726937));
#45780=DIRECTION('center_axis',(0.734238830876792,-8.991832340449E-17,0.678891257295808));
#45781=DIRECTION('ref_axis',(6.6021524650914E-17,1.,6.10447636300053E-17));
#45782=DIRECTION('center_axis',(-0.734238830865093,1.72051620514813E-11,
-0.67889125730846));
#45783=DIRECTION('ref_axis',(-5.25579579857545E-11,1.,8.21898105129997E-11));
#45784=DIRECTION('',(0.734238830876791,0.,0.678891257295807));
#45785=DIRECTION('center_axis',(0.911344477115603,-2.366403068759E-7,0.411644560307595));
#45786=DIRECTION('ref_axis',(0.291076810513629,0.707106786078308,-0.644417786426801));
#45787=DIRECTION('center_axis',(2.17357452795E-16,-2.66186108837E-32,-1.));
#45788=DIRECTION('ref_axis',(-1.,-5.7857534586223E-48,-2.17357452795E-16));
#45789=DIRECTION('',(0.,0.,-1.));
#45790=DIRECTION('center_axis',(-0.815922385281966,-1.22989217005322E-6,
0.578161449073072));
#45791=DIRECTION('ref_axis',(-0.408798373511725,-0.707146211104366,-0.576912580842979));
#45792=DIRECTION('center_axis',(0.734238830876792,-8.99183234042744E-17,
0.678891257295808));
#45793=DIRECTION('ref_axis',(0.678891257295808,1.51038693775819E-31,-0.734238830876792));
#45794=DIRECTION('',(0.734238830876791,0.,0.678891257295807));
#45795=DIRECTION('center_axis',(-2.19931778314037E-16,-1.,-1.97757654230408E-17));
#45796=DIRECTION('ref_axis',(0.980030917502135,-2.19472257881379E-16,0.198845167756028));
#45797=DIRECTION('center_axis',(1.22464679915E-16,1.,5.47382212627E-48));
#45798=DIRECTION('ref_axis',(1.,-1.22464679915E-16,5.24998673990483E-64));
#45799=DIRECTION('center_axis',(-5.46401789901627E-17,-1.,6.08764557973899E-17));
#45800=DIRECTION('ref_axis',(0.744196935834912,0.,0.667960268798922));
#45801=DIRECTION('center_axis',(1.22464679915E-16,1.,-6.16297582204E-33));
#45802=DIRECTION('ref_axis',(1.,-1.22464679915E-16,7.54746861370013E-49));
#45803=DIRECTION('center_axis',(-1.24015983872461E-7,0.999999999999986,
1.11611400503811E-7));
#45804=DIRECTION('ref_axis',(0.721583920149089,1.6675952356328E-7,-0.692326979239033));
#45805=DIRECTION('center_axis',(-0.884316205578325,0.0178356349302338,0.466547681033985));
#45806=DIRECTION('ref_axis',(-0.0157873708942533,-0.999840932052135,0.00829876577361474));
#45807=DIRECTION('center_axis',(-1.14444500362894E-17,-1.,3.5644992269101E-17));
#45808=DIRECTION('ref_axis',(0.952128653909774,0.,0.305697606146927));
#45809=DIRECTION('center_axis',(1.22464679915E-16,1.,5.47382212627E-48));
#45810=DIRECTION('ref_axis',(1.,-1.22464679915E-16,6.22660996643423E-64));
#45811=DIRECTION('center_axis',(0.110668766458005,-1.35530150608006E-17,
0.993857345966041));
#45812=DIRECTION('ref_axis',(0.993857345966041,-5.87811925404552E-33,-0.110668766458005));
#45813=DIRECTION('center_axis',(1.22464679915E-16,1.,5.47382212627E-48));
#45814=DIRECTION('ref_axis',(1.,-1.22464679915E-16,5.9677926224237E-64));
#45815=DIRECTION('center_axis',(-1.49989545857296E-18,-1.,-1.34697635782315E-17));
#45816=DIRECTION('ref_axis',(0.993857345966041,0.,-0.110668766458005));
#45817=DIRECTION('center_axis',(1.22464679915E-16,1.,1.54074395551E-33));
#45818=DIRECTION('ref_axis',(1.,-1.22464679915E-16,-1.88686715342503E-49));
#45819=DIRECTION('center_axis',(1.,-1.22464679915E-16,6.12323399574E-17));
#45820=DIRECTION('ref_axis',(1.22464679915E-16,1.,7.49879891332945E-33));
#45821=DIRECTION('center_axis',(1.22464679915E-16,1.,5.47382212627E-48));
#45822=DIRECTION('ref_axis',(1.,-1.22464679915E-16,-6.703498746053E-64));
#45823=DIRECTION('center_axis',(1.,-1.22464679915E-16,6.12323399574E-17));
#45824=DIRECTION('ref_axis',(-6.12323399574E-17,7.49879891332945E-33,1.));
#45825=DIRECTION('',(-1.,0.,-1.32512071049E-16));
#45826=DIRECTION('center_axis',(1.,-1.22464679915E-16,6.12323399574E-17));
#45827=DIRECTION('ref_axis',(-1.22464679915E-16,-1.,-7.49879891332945E-33));
#45828=DIRECTION('',(-1.,0.,-1.32512071049E-16));
#45829=DIRECTION('center_axis',(-1.22464679915E-16,-1.,1.81284143127026E-30));
#45830=DIRECTION('ref_axis',(-1.57898385724467E-14,0.,-1.));
#45831=DIRECTION('center_axis',(1.22464679915E-16,1.,5.47382212627E-48));
#45832=DIRECTION('ref_axis',(1.,-1.22464679915E-16,-6.703498746053E-64));
#45833=DIRECTION('center_axis',(0.106117864373042,-1.29956902936052E-17,
-0.994353558278395));
#45834=DIRECTION('ref_axis',(0.994353558278395,1.45479619498441E-32,0.106117864373042));
#45835=DIRECTION('center_axis',(1.22464679915E-16,1.,5.47382212627E-48));
#45836=DIRECTION('ref_axis',(1.,-1.22464679915E-16,-6.703498746053E-64));
#45837=DIRECTION('center_axis',(-4.52327322274045E-17,-1.,5.91050929206098E-17));
#45838=DIRECTION('ref_axis',(0.794132678900969,0.,0.607744426795977));
#45839=DIRECTION('center_axis',(-1.22464679915E-16,-1.,-5.47382212627E-48));
#45840=DIRECTION('ref_axis',(1.,-1.22464679915E-16,-6.703498746053E-64));
#45841=DIRECTION('center_axis',(0.607744426795977,-7.44272266974971E-17,
-0.794132678900969));
#45842=DIRECTION('ref_axis',(0.794132678900969,-2.10244190700647E-31,0.607744426795977));
#45843=DIRECTION('center_axis',(-1.22464679915E-16,-1.,-5.47382212627E-48));
#45844=DIRECTION('ref_axis',(1.,-1.22464679915E-16,-6.703498746053E-64));
#45845=DIRECTION('center_axis',(-4.52327322274045E-17,-1.,5.91050929206098E-17));
#45846=DIRECTION('ref_axis',(-0.794132678900969,0.,-0.607744426795977));
#45847=DIRECTION('center_axis',(1.22464679915E-16,1.,1.23259516441E-32));
#45848=DIRECTION('ref_axis',(1.,-1.22464679915E-16,-1.50949372274247E-48));
#45849=DIRECTION('center_axis',(-0.734238830876792,8.99183234042744E-17,
-0.678891257295808));
#45850=DIRECTION('ref_axis',(0.678891257295808,1.51038693775819E-31,-0.734238830876792));
#45851=DIRECTION('center_axis',(1.22464679915E-16,1.,5.47382212627E-48));
#45852=DIRECTION('ref_axis',(1.,-1.22464679915E-16,-6.703498746053E-64));
#45853=DIRECTION('center_axis',(0.757497881302333,0.120607621490521,-0.641600156998793));
#45854=DIRECTION('ref_axis',(0.519185231994408,-0.707106824013922,0.480048574950346));
#45855=DIRECTION('center_axis',(-0.540714503083014,-0.0890998529400356,
-0.836474173158833));
#45856=DIRECTION('ref_axis',(0.803860483463198,-0.347724019666725,-0.482593337369186));
#45857=DIRECTION('center_axis',(0.734238830876792,-8.991832340449E-17,0.678891257295808));
#45858=DIRECTION('ref_axis',(-6.6021524650914E-17,-1.,-6.10447636300053E-17));
#45859=DIRECTION('',(0.734238830876791,0.,0.678891257295807));
#45860=DIRECTION('',(0.734238830876791,0.,0.678891257295807));
#45861=DIRECTION('center_axis',(1.2246467991486E-16,1.,-1.56475089353662E-28));
#45862=DIRECTION('ref_axis',(0.667272304480808,-8.17172891841765E-17,0.744813850349785));
#45863=DIRECTION('',(0.,1.,0.));
#45864=DIRECTION('center_axis',(1.22464679915E-16,1.,6.16297582204E-33));
#45865=DIRECTION('ref_axis',(1.,-1.22464679915E-16,7.0105395811531E-49));
#45866=DIRECTION('',(0.,-1.,0.));
#45867=DIRECTION('center_axis',(-1.22464679915011E-16,-1.,-3.67313358993533E-30));
#45868=DIRECTION('ref_axis',(0.952128653909774,-1.16602130838972E-16,0.305697606146927));
#45869=DIRECTION('center_axis',(1.22464679915E-16,1.,-6.16297582204E-33));
#45870=DIRECTION('ref_axis',(1.,-1.22464679915E-16,7.54746861370013E-49));
#45871=DIRECTION('',(0.,-1.,0.));
#45872=DIRECTION('center_axis',(1.22464679914586E-16,1.,-1.3947821589454E-28));
#45873=DIRECTION('ref_axis',(0.947590338356885,-1.16046347476986E-16,0.319487950715961));
#45874=DIRECTION('center_axis',(1.22464679915E-16,1.,0.));
#45875=DIRECTION('ref_axis',(1.,-1.22464679915E-16,0.));
#45876=DIRECTION('center_axis',(1.22464679914997E-16,1.,-3.04211334326766E-29));
#45877=DIRECTION('ref_axis',(0.111333411199055,-1.36344105663067E-17,0.993783110920478));
#45878=DIRECTION('center_axis',(-1.75622944019E-17,1.,1.50524498801E-15));
#45879=DIRECTION('ref_axis',(1.,1.75622944019E-17,2.64355556264161E-32));
#45880=DIRECTION('',(-2.77555756156E-16,-1.,0.));
#45881=DIRECTION('center_axis',(1.22464679914586E-16,1.,-1.3947821589454E-28));
#45882=DIRECTION('ref_axis',(0.947590338356885,-1.16046347476986E-16,0.319487950715961));
#45883=DIRECTION('center_axis',(1.22464679915E-16,1.,0.));
#45884=DIRECTION('ref_axis',(1.,-1.22464679915E-16,0.));
#45885=DIRECTION('',(0.,1.,0.));
#45886=DIRECTION('center_axis',(-1.22464679915E-16,-1.,-1.69953884181051E-33));
#45887=DIRECTION('ref_axis',(2.08133480265435E-49,1.69953884181051E-33,
-1.));
#45888=DIRECTION('center_axis',(-2.44959827562E-16,-1.,1.36892417294E-16));
#45889=DIRECTION('ref_axis',(1.,-2.44959827562E-16,3.35331429348836E-32));
#45890=DIRECTION('',(0.,1.,0.));
#45891=DIRECTION('center_axis',(-2.17357452795E-16,2.66186108837E-32,1.));
#45892=DIRECTION('ref_axis',(1.,2.56447231488414E-65,2.17357452795E-16));
#45893=DIRECTION('',(-1.,0.,-1.09790153833E-16));
#45894=DIRECTION('',(0.,1.,0.));
#45895=DIRECTION('center_axis',(1.22464679915E-16,1.,1.94567767731298E-44));
#45896=DIRECTION('ref_axis',(2.38276793969895E-60,1.94567767731298E-44,
-1.));
#45897=DIRECTION('center_axis',(3.43485006637E-19,-1.,1.36611674972E-16));
#45898=DIRECTION('ref_axis',(1.,3.43485006637E-19,-4.69240620844491E-35));
#45899=DIRECTION('',(0.,1.,0.));
#45900=DIRECTION('center_axis',(1.22464679914998E-16,1.,-1.73663083545565E-29));
#45901=DIRECTION('ref_axis',(0.095298509688002,-1.16707014853003E-17,0.99544874004202));
#45902=DIRECTION('center_axis',(-1.22464679915E-16,-1.,0.));
#45903=DIRECTION('ref_axis',(1.,-1.22464679915E-16,0.));
#45904=DIRECTION('',(0.,1.,0.));
#45905=DIRECTION('center_axis',(-1.224646799149E-16,-1.,-1.07603845915075E-28));
#45906=DIRECTION('ref_axis',(-0.678891257295809,8.31402005216765E-17,0.73423883087679));
#45907=DIRECTION('center_axis',(-1.83472486973E-16,-1.,5.23898221099E-18));
#45908=DIRECTION('ref_axis',(1.,-1.83472486973E-16,9.61209095457641E-34));
#45909=DIRECTION('',(0.,1.,0.));
#45910=DIRECTION('center_axis',(0.678891257295808,-8.31402005216764E-17,
-0.734238830876792));
#45911=DIRECTION('ref_axis',(4.92781901212525E-33,-1.,1.13233183843457E-16));
#45912=DIRECTION('',(0.734238830876791,0.,0.678891257295807));
#45913=DIRECTION('',(0.,1.,0.));
#45914=DIRECTION('center_axis',(1.224646799149E-16,1.,1.07603845915075E-28));
#45915=DIRECTION('ref_axis',(-0.67889125729581,8.31402005216767E-17,0.734238830876789));
#45916=DIRECTION('center_axis',(1.22564216467E-16,1.,6.12322590562E-17));
#45917=DIRECTION('ref_axis',(1.,-1.22564216467E-16,-7.50488385372752E-33));
#45918=DIRECTION('center_axis',(0.,1.,0.));
#45919=DIRECTION('ref_axis',(0.00162555525320111,0.,0.999998678784187));
#45920=DIRECTION('center_axis',(0.732027802944257,-8.96475505763315E-17,
-0.68127475787424));
#45921=DIRECTION('ref_axis',(0.68127475787424,-1.91888914560603E-31,0.732027802944257));
#45922=DIRECTION('center_axis',(0.734238830876792,-8.99183234042744E-17,
0.678891257295808));
#45923=DIRECTION('ref_axis',(0.678891257295807,3.46311205996404E-31,-0.734238830876791));
#45924=DIRECTION('center_axis',(5.46401789901627E-17,1.,-6.08764557973899E-17));
#45925=DIRECTION('ref_axis',(0.744196935834912,0.,0.667960268798922));
#45926=DIRECTION('center_axis',(1.22464679915E-16,1.,5.47382212627E-48));
#45927=DIRECTION('ref_axis',(1.,-1.22464679915E-16,6.49622071350503E-64));
#45928=DIRECTION('center_axis',(-0.667960268798921,8.18015405141904E-17,
0.744196935834913));
#45929=DIRECTION('ref_axis',(0.744196935834913,-3.15837441223295E-32,0.667960268798921));
#45930=DIRECTION('center_axis',(1.14444500362894E-17,1.,-3.5644992269101E-17));
#45931=DIRECTION('ref_axis',(0.952128653909774,0.,0.305697606146927));
#45932=DIRECTION('center_axis',(1.22464679915E-16,1.,5.47382212627E-48));
#45933=DIRECTION('ref_axis',(1.,-1.22464679915E-16,-6.703498746053E-64));
#45934=DIRECTION('center_axis',(-0.305697606146928,3.74371594874912E-17,
0.952128653909774));
#45935=DIRECTION('ref_axis',(0.952128653909774,-6.76944606262743E-33,0.305697606146928));
#45936=DIRECTION('center_axis',(0.222411493783323,0.670605060062733,-0.707687770737441));
#45937=DIRECTION('ref_axis',(0.848579081651793,0.224251763465943,0.479191703564883));
#45938=DIRECTION('center_axis',(-0.299820876204079,3.67174676361097E-17,
0.953995514765252));
#45939=DIRECTION('ref_axis',(0.953995514765252,-6.3869078326472E-32,0.299820876204079));
#45940=DIRECTION('center_axis',(0.734238830876792,-8.99183234042744E-17,
0.678891257295808));
#45941=DIRECTION('ref_axis',(0.678891257295807,3.46311205996404E-31,-0.734238830876791));
#45942=DIRECTION('center_axis',(2.41898181523141E-16,1.,1.1741867647411E-17));
#45943=DIRECTION('ref_axis',(-0.99520202856178,2.41886400693281E-16,-0.0978413120645785));
#45944=DIRECTION('center_axis',(1.22464679915E-16,1.,5.47382212627E-48));
#45945=DIRECTION('ref_axis',(1.,-1.22464679915E-16,6.49622071350503E-64));
#45946=DIRECTION('center_axis',(0.962126872935794,0.250387400346799,-0.107786966384449));
#45947=DIRECTION('ref_axis',(-0.248830769651925,0.968145727536702,0.0278764834019926));
#45948=DIRECTION('center_axis',(-0.993783110920478,1.2170333058406E-16,
0.111333411199054));
#45949=DIRECTION('ref_axis',(0.111333411199054,1.57725565511394E-32,0.993783110920478));
#45950=DIRECTION('center_axis',(0.152411459643054,-1.86650206205066E-17,
-0.988317128744349));
#45951=DIRECTION('ref_axis',(0.988317128744349,-1.89428554374595E-32,0.152411459643054));
#45952=DIRECTION('center_axis',(2.41898181523141E-16,1.,1.1741867647411E-17));
#45953=DIRECTION('ref_axis',(0.99977954662694,-2.41886400693281E-16,0.0209966222623895));
#45954=DIRECTION('center_axis',(1.22464679915E-16,1.,5.47382212627E-48));
#45955=DIRECTION('ref_axis',(1.,-1.22464679915E-16,6.49622071350503E-64));
#45956=DIRECTION('center_axis',(0.,0.,1.));
#45957=DIRECTION('ref_axis',(1.,0.,0.));
#45958=DIRECTION('center_axis',(1.,-1.22464679915E-16,6.12323399574E-17));
#45959=DIRECTION('ref_axis',(1.22464679915E-16,1.,7.49879891332945E-33));
#45960=DIRECTION('center_axis',(1.,-1.22464679915E-16,6.12323399574E-17));
#45961=DIRECTION('ref_axis',(6.12323399574E-17,-7.49879891332945E-33,-1.));
#45962=DIRECTION('',(-1.,0.,-2.65024142098E-16));
#45963=DIRECTION('center_axis',(1.,0.,0.));
#45964=DIRECTION('ref_axis',(0.,-1.,0.));
#45965=DIRECTION('center_axis',(0.106117864373042,-1.29956902936052E-17,
-0.994353558278395));
#45966=DIRECTION('ref_axis',(0.994353558278395,-3.91187297993902E-33,0.106117864373042));
#45967=DIRECTION('center_axis',(1.68490994230906E-17,1.,-4.21844451941189E-17));
#45968=DIRECTION('ref_axis',(0.928711112494875,0.,0.37080408510227));
#45969=DIRECTION('center_axis',(-1.22464679915E-16,-1.,-5.47382212627E-48));
#45970=DIRECTION('ref_axis',(1.,-1.22464679915E-16,-6.703498746053E-64));
#45971=DIRECTION('center_axis',(0.,0.,1.));
#45972=DIRECTION('ref_axis',(1.,0.,0.));
#45973=DIRECTION('center_axis',(-0.734238830876792,8.99183234042744E-17,
-0.678891257295808));
#45974=DIRECTION('ref_axis',(0.678891257295808,-2.24691316591619E-32,-0.734238830876792));
#45975=DIRECTION('center_axis',(0.734238830876792,-8.991832340449E-17,0.678891257295808));
#45976=DIRECTION('ref_axis',(6.6021524650914E-17,1.,6.10447636300053E-17));
#45977=DIRECTION('',(0.734238830876791,0.,0.678891257295807));
#45978=DIRECTION('center_axis',(0.734238830876792,-8.99183234042744E-17,
0.678891257295808));
#45979=DIRECTION('ref_axis',(0.678891257295807,3.46311205996404E-31,-0.734238830876791));
#45980=DIRECTION('',(-0.734238830876791,0.,-0.678891257295807));
#45981=DIRECTION('center_axis',(0.734238830876792,-8.99183234042744E-17,
0.678891257295808));
#45982=DIRECTION('ref_axis',(0.678891257295807,3.46311205996404E-31,-0.734238830876791));
#45983=DIRECTION('center_axis',(6.60215246509141E-17,1.,6.10447636300053E-17));
#45984=DIRECTION('ref_axis',(-0.678891257295808,0.,0.734238830876791));
#45985=DIRECTION('center_axis',(-1.22464679915E-16,-1.,-5.47382212627E-48));
#45986=DIRECTION('ref_axis',(1.,-1.22464679915E-16,-6.703498746053E-64));
#45987=DIRECTION('center_axis',(-0.613815420645987,7.51707090161983E-17,
0.789449573675983));
#45988=DIRECTION('ref_axis',(0.789449573675983,7.34020703099417E-32,0.613815420645987));
#45989=DIRECTION('center_axis',(3.85062311351295E-17,1.,-5.68588026119494E-17));
#45990=DIRECTION('ref_axis',(0.827993213361104,0.,0.560738119471071));
#45991=DIRECTION('center_axis',(1.22464679915E-16,1.,5.47382212627E-48));
#45992=DIRECTION('ref_axis',(1.,-1.22464679915E-16,-6.703498746053E-64));
#45993=DIRECTION('center_axis',(-0.560738119471071,6.86706143170087E-17,
0.827993213361104));
#45994=DIRECTION('ref_axis',(0.827993213361104,-2.38131063616686E-32,0.560738119471071));
#45995=DIRECTION('center_axis',(3.85062311351295E-17,1.,-5.68588026119494E-17));
#45996=DIRECTION('ref_axis',(-0.827993213361104,0.,-0.560738119471072));
#45997=DIRECTION('center_axis',(-1.22464679915E-16,-1.,-5.47382212627E-48));
#45998=DIRECTION('ref_axis',(1.,-1.22464679915E-16,-6.703498746053E-64));
#45999=DIRECTION('center_axis',(1.22464679915E-16,1.,5.47382212627E-48));
#46000=DIRECTION('ref_axis',(1.,-1.22464679915E-16,0.));
#46001=DIRECTION('center_axis',(1.224646799149E-16,1.,-1.07595286226434E-28));
#46002=DIRECTION('ref_axis',(0.67889125729581,-8.31402005216767E-17,0.734238830876789));
#46003=DIRECTION('',(0.,-1.,0.));
#46004=DIRECTION('center_axis',(-1.22464679915E-16,-1.,-6.16297582204E-33));
#46005=DIRECTION('ref_axis',(1.,-1.22464679915E-16,-7.54746861370013E-49));
#46006=DIRECTION('',(-2.85587916301E-16,-1.,0.));
#46007=DIRECTION('center_axis',(-1.22464679915E-16,-1.,-1.23259516441E-32));
#46008=DIRECTION('ref_axis',(1.,-1.22464679915E-16,-1.50949372274247E-48));
#46009=DIRECTION('center_axis',(-1.22464679914912E-16,-1.,-1.26181562037188E-28));
#46010=DIRECTION('ref_axis',(-0.572811155566786,7.01491348180737E-17,0.819687367267694));
#46011=DIRECTION('center_axis',(-0.641370372756966,0.046782002687993,0.765803818986358));
#46012=DIRECTION('ref_axis',(0.766534261679224,0.0816131667450425,0.636996480905298));
#46013=DIRECTION('center_axis',(1.22464679915E-16,1.,0.));
#46014=DIRECTION('ref_axis',(1.,-1.22464679915E-16,0.));
#46015=DIRECTION('center_axis',(1.22464679915E-16,1.,-1.23259516441E-32));
#46016=DIRECTION('ref_axis',(1.,-1.22464679915E-16,1.50949372274247E-48));
#46017=DIRECTION('',(0.,-1.,0.));
#46018=DIRECTION('center_axis',(1.22464679914824E-16,1.,2.07777882089137E-28));
#46019=DIRECTION('ref_axis',(0.646318112561793,-7.91511407778746E-17,-0.763068081742751));
#46020=DIRECTION('center_axis',(-1.22464679915E-16,-1.,6.16297582204E-33));
#46021=DIRECTION('ref_axis',(1.,-1.22464679915E-16,7.54746861370013E-49));
#46022=DIRECTION('',(0.,-1.,0.));
#46023=DIRECTION('center_axis',(-1.22464679914844E-16,-1.,-1.36783824494702E-28));
#46024=DIRECTION('ref_axis',(-0.751089446707,9.19819286783E-17,0.660200456713999));
#46025=DIRECTION('',(2.85587916301E-16,1.,0.));
#46026=DIRECTION('center_axis',(1.22464679915E-16,1.,0.));
#46027=DIRECTION('ref_axis',(1.,-1.22464679915E-16,0.));
#46028=DIRECTION('',(2.85587916301E-16,1.,0.));
#46029=DIRECTION('center_axis',(-1.2246467991496E-16,-1.,-1.24243880634581E-29));
#46030=DIRECTION('ref_axis',(-0.953995514765253,1.16830755356031E-16,0.299820876204076));
#46031=DIRECTION('',(0.,1.,0.));
#46032=DIRECTION('center_axis',(1.22464679915E-16,1.,0.));
#46033=DIRECTION('ref_axis',(1.,-1.22464679915E-16,0.));
#46034=DIRECTION('',(0.,1.,0.));
#46035=DIRECTION('center_axis',(-0.678891257295808,8.31402005216763E-17,
-0.734238830876792));
#46036=DIRECTION('ref_axis',(-0.734238830876792,-5.02124004685594E-34,0.678891257295808));
#46037=DIRECTION('',(0.734238830876791,0.,-0.678891257295807));
#46038=DIRECTION('',(-0.734238830876791,0.,0.678891257295807));
#46039=DIRECTION('',(0.,-1.,0.));
#46040=DIRECTION('center_axis',(1.224646799149E-16,1.,-1.07595286226434E-28));
#46041=DIRECTION('ref_axis',(0.67889125729581,-8.31402005216767E-17,0.734238830876789));
#46042=DIRECTION('center_axis',(-1.22464679915E-16,-1.,0.));
#46043=DIRECTION('ref_axis',(1.,-1.22464679915E-16,0.));
#46044=DIRECTION('',(0.,-1.,0.));
#46045=DIRECTION('center_axis',(1.22464679915E-16,1.,-1.23259516441E-32));
#46046=DIRECTION('ref_axis',(1.,-1.22464679915E-16,1.50949372274247E-48));
#46047=DIRECTION('center_axis',(-1.22464679914912E-16,-1.,-1.26181562037188E-28));
#46048=DIRECTION('ref_axis',(-0.572811155566786,7.01491348180737E-17,0.819687367267694));
#46049=DIRECTION('center_axis',(-1.22464679915E-16,-1.,0.));
#46050=DIRECTION('ref_axis',(1.,-1.22464679915E-16,0.));
#46051=DIRECTION('center_axis',(1.22464679915E-16,1.,-1.23259516441E-32));
#46052=DIRECTION('ref_axis',(1.,-1.22464679915E-16,1.50949372274247E-48));
#46053=DIRECTION('',(0.,-1.,0.));
#46054=DIRECTION('center_axis',(-1.224646799149E-16,-1.,1.07603845915075E-28));
#46055=DIRECTION('ref_axis',(-0.67889125729581,8.31402005216767E-17,-0.734238830876789));
#46056=DIRECTION('center_axis',(-1.22464679915E-16,-1.,0.));
#46057=DIRECTION('ref_axis',(1.,-1.22464679915E-16,0.));
#46058=DIRECTION('',(0.,-1.,0.));
#46059=DIRECTION('',(0.,-1.,0.));
#46060=DIRECTION('center_axis',(1.22464679915E-16,1.,-2.46519032882E-32));
#46061=DIRECTION('ref_axis',(1.,-1.22464679915E-16,3.01898744548495E-48));
#46062=DIRECTION('center_axis',(-0.678891257295808,8.31402005216763E-17,
-0.734238830876792));
#46063=DIRECTION('ref_axis',(-0.734238830876792,-5.02124004685594E-34,0.678891257295808));
#46064=DIRECTION('',(-0.734238830876791,0.,0.678891257295807));
#46065=DIRECTION('center_axis',(-0.678891258039564,8.05580512386835E-9,
-0.7342388301891));
#46066=DIRECTION('ref_axis',(-1.90502136153082E-5,-0.999999999663608,1.76032200345041E-5));
#46067=DIRECTION('',(0.734238830876791,0.,-0.678891257295807));
#46068=DIRECTION('',(0.,1.,0.));
#46069=DIRECTION('center_axis',(0.734238830876792,-8.99183234042744E-17,
-0.678891257295808));
#46070=DIRECTION('ref_axis',(0.678891257295807,3.46311205996404E-31,0.734238830876791));
#46071=DIRECTION('',(-0.734238830876791,0.,0.678891257295807));
#46072=DIRECTION('center_axis',(-0.734238830876792,8.99183234042744E-17,
0.678891257295808));
#46073=DIRECTION('ref_axis',(0.678891257295807,3.46311205996404E-31,0.734238830876791));
#46074=DIRECTION('',(-0.734238830876791,0.,0.678891257295807));
#46075=DIRECTION('center_axis',(0.734238830904136,4.02815121124967E-11,
-0.678891257266234));
#46076=DIRECTION('ref_axis',(-4.69698354284746E-11,-1.,-1.10134124042815E-10));
#46077=DIRECTION('center_axis',(0.,0.,1.));
#46078=DIRECTION('ref_axis',(1.,0.,0.));
#46079=DIRECTION('center_axis',(0.803996045360697,-9.84611183477626E-17,
0.594634643326775));
#46080=DIRECTION('ref_axis',(0.594634643326775,4.97302608069436E-32,-0.803996045360697));
#46081=DIRECTION('center_axis',(-7.91623497736024E-17,-1.,-5.85483919904324E-17));
#46082=DIRECTION('ref_axis',(-0.594634643326775,0.,0.803996045360696));
#46083=DIRECTION('center_axis',(0.763068081742753,-9.34488883837698E-17,
0.646318112561791));
#46084=DIRECTION('ref_axis',(0.646318112561791,2.50438493602067E-31,-0.763068081742753));
#46085=DIRECTION('center_axis',(1.22464679915E-16,1.,5.47382212627E-48));
#46086=DIRECTION('ref_axis',(1.,-1.22464679915E-16,-6.703498746053E-64));
#46087=DIRECTION('center_axis',(1.,0.,0.));
#46088=DIRECTION('ref_axis',(0.,-1.,0.));
#46089=DIRECTION('center_axis',(0.734238830876792,-8.99183234042744E-17,
-0.678891257295808));
#46090=DIRECTION('ref_axis',(0.678891257295807,3.46311205996404E-31,0.734238830876791));
#46091=DIRECTION('center_axis',(-0.734238830876792,8.99183234042744E-17,
0.678891257295808));
#46092=DIRECTION('ref_axis',(-0.678891257295807,-3.46311205996404E-31,-0.734238830876791));
#46093=DIRECTION('center_axis',(0.734238830876792,-8.99183234042744E-17,
-0.678891257295808));
#46094=DIRECTION('ref_axis',(0.678891257295807,3.46311205996404E-31,0.734238830876791));
#46095=DIRECTION('',(0.734238830876791,0.,-0.678891257295807));
#46096=DIRECTION('',(0.734238830876791,0.,-0.678891257295807));
#46097=DIRECTION('center_axis',(-6.60215246509141E-17,-1.,6.10447636300053E-17));
#46098=DIRECTION('ref_axis',(0.678891257295808,0.,0.734238830876791));
#46099=DIRECTION('center_axis',(0.732027802944257,-8.96475505763315E-17,
0.68127475787424));
#46100=DIRECTION('ref_axis',(0.68127475787424,-1.91888914560603E-31,-0.732027802944257));
#46101=DIRECTION('center_axis',(1.22464679915E-16,1.,-1.23259516441E-32));
#46102=DIRECTION('ref_axis',(1.,-1.22464679915E-16,1.50949372274247E-48));
#46103=DIRECTION('center_axis',(1.22464679915E-16,1.,5.47382212627E-48));
#46104=DIRECTION('ref_axis',(1.,-1.22464679915E-16,-6.703498746053E-64));
#46105=DIRECTION('center_axis',(-6.56244994878123E-17,-1.,-6.10746133129891E-17));
#46106=DIRECTION('ref_axis',(-0.681274757874239,0.,0.732027802944258));
#46107=DIRECTION('center_axis',(0.660200456714,-8.0851237611E-17,0.751089446706999));
#46108=DIRECTION('ref_axis',(0.751089446706999,6.24086217807948E-32,-0.660200456714));
#46109=DIRECTION('center_axis',(1.22464679915E-16,1.,5.47382212627E-48));
#46110=DIRECTION('ref_axis',(1.,-1.22464679915E-16,6.22660996643423E-64));
#46111=DIRECTION('center_axis',(1.22464679915E-16,1.,5.47382212627E-48));
#46112=DIRECTION('ref_axis',(1.,-1.22464679915E-16,5.9677926224237E-64));
#46113=DIRECTION('center_axis',(-5.33780239968174E-17,-1.,-6.0726511322985E-17));
#46114=DIRECTION('ref_axis',(-0.751089446706998,0.,0.660200456714001));
#46115=DIRECTION('center_axis',(0.315563048033822,-3.86453276703782E-17,
0.948904612021463));
#46116=DIRECTION('ref_axis',(0.948904612021463,7.52823903108453E-32,-0.315563048033822));
#46117=DIRECTION('center_axis',(1.22464679915E-16,1.,5.47382212627E-48));
#46118=DIRECTION('ref_axis',(1.,-1.22464679915E-16,-6.703498746053E-64));
#46119=DIRECTION('center_axis',(-1.21950373919573E-17,-1.,-3.66707296595837E-17));
#46120=DIRECTION('ref_axis',(-0.948904612021463,0.,0.315563048033822));
#46121=DIRECTION('center_axis',(0.299820876204079,-3.67174676361097E-17,
0.953995514765252));
#46122=DIRECTION('ref_axis',(0.953995514765252,-6.3869078326472E-32,-0.299820876204079));
#46123=DIRECTION('center_axis',(1.22464679915E-16,1.,5.47382212627E-48));
#46124=DIRECTION('ref_axis',(1.,-1.22464679915E-16,6.22660996643423E-64));
#46125=DIRECTION('center_axis',(1.22464679915E-16,1.,5.47382212627E-48));
#46126=DIRECTION('ref_axis',(1.,-1.22464679915E-16,5.9677926224237E-64));
#46127=DIRECTION('center_axis',(-1.10086633186706E-17,-1.,-3.5028299438442E-17));
#46128=DIRECTION('ref_axis',(-0.953995514765252,0.,0.299820876204079));
#46129=DIRECTION('center_axis',(-0.734238830876792,8.99183234042744E-17,
0.678891257295808));
#46130=DIRECTION('ref_axis',(0.678891257295807,3.46311205996404E-31,0.734238830876791));
#46131=DIRECTION('center_axis',(1.22464679915E-16,1.,5.47382212627E-48));
#46132=DIRECTION('ref_axis',(1.,-1.22464679915E-16,-6.703498746053E-64));
#46133=DIRECTION('center_axis',(0.734238830876792,-8.99183234042744E-17,
-0.678891257295808));
#46134=DIRECTION('ref_axis',(0.678891257295807,3.46311205996404E-31,0.734238830876791));
#46135=DIRECTION('center_axis',(-0.734238830876792,8.99183234042744E-17,
0.678891257295808));
#46136=DIRECTION('ref_axis',(0.678891257295807,3.46311205996404E-31,0.734238830876791));
#46137=DIRECTION('',(-0.734238830876791,0.,0.678891257295807));
#46138=DIRECTION('center_axis',(0.,0.,1.));
#46139=DIRECTION('ref_axis',(1.,0.,0.));
#46140=DIRECTION('center_axis',(0.613815420645987,-7.51707090161983E-17,
0.789449573675983));
#46141=DIRECTION('ref_axis',(0.789449573675983,7.34020703099417E-32,-0.613815420645987));
#46142=DIRECTION('center_axis',(-4.61409403750984E-17,-1.,-5.93434841858408E-17));
#46143=DIRECTION('ref_axis',(-0.789449573675983,0.,0.613815420645986));
#46144=DIRECTION('center_axis',(0.560738119471071,-6.86706143170087E-17,
0.827993213361104));
#46145=DIRECTION('ref_axis',(0.827993213361104,-2.38131063616686E-32,-0.560738119471071));
#46146=DIRECTION('center_axis',(1.22464679915E-16,1.,5.47382212627E-48));
#46147=DIRECTION('ref_axis',(1.,-1.22464679915E-16,-6.703498746053E-64));
#46148=DIRECTION('center_axis',(1.,0.,0.));
#46149=DIRECTION('ref_axis',(0.,-1.,0.));
#46150=DIRECTION('center_axis',(0.734238830876792,-8.99183234042744E-17,
-0.678891257295808));
#46151=DIRECTION('ref_axis',(0.678891257295807,3.46311205996404E-31,0.734238830876791));
#46152=DIRECTION('center_axis',(0.734238830876792,-8.99183234039869E-17,
-0.678891257295808));
#46153=DIRECTION('ref_axis',(-6.60215246505446E-17,-1.,6.10447636296637E-17));
#46154=DIRECTION('',(0.734238830876791,0.,-0.678891257295807));
#46155=DIRECTION('center_axis',(0.734238830865106,1.72097426658295E-11,
-0.678891257308446));
#46156=DIRECTION('ref_axis',(-0.678891257308445,-1.48029736616684E-14,-0.734238830865107));
#46157=DIRECTION('center_axis',(-1.22464679915E-16,-1.,-5.47382212627E-48));
#46158=DIRECTION('ref_axis',(-1.,1.22464679915E-16,0.));
#46159=DIRECTION('center_axis',(-1.22464679915E-16,-1.,0.));
#46160=DIRECTION('ref_axis',(1.,-1.22464679915E-16,0.));
#46161=DIRECTION('center_axis',(-1.22464679915E-16,-1.,1.23259516441E-32));
#46162=DIRECTION('ref_axis',(1.,-1.22464679915E-16,1.50949372274247E-48));
#46163=DIRECTION('center_axis',(1.,-1.22464679915E-16,6.12323399574E-17));
#46164=DIRECTION('ref_axis',(-1.22464679915E-16,-1.,-6.67366607695787E-50));
#46165=DIRECTION('',(2.5585870064E-16,0.,-1.));
#46166=DIRECTION('',(-1.34875042533E-16,-1.,0.));
#46167=DIRECTION('',(2.21800239814E-16,0.,-1.));
#46168=DIRECTION('',(-1.26882631386E-16,-1.,0.));
#46169=DIRECTION('',(1.75377892382E-16,0.,-1.));
#46170=DIRECTION('',(-1.26882631386E-16,-1.,0.));
#46171=DIRECTION('center_axis',(1.22464679915E-16,1.,7.60253073092891E-48));
#46172=DIRECTION('ref_axis',(-1.,1.22464679915E-16,9.3104149250716E-64));
#46173=DIRECTION('center_axis',(-1.22464679915E-16,-1.,0.));
#46174=DIRECTION('ref_axis',(1.,-1.22464679915E-16,0.));
#46175=DIRECTION('',(-1.42793958151E-16,-1.,0.));
#46176=DIRECTION('center_axis',(-1.22464679915E-16,-1.,0.));
#46177=DIRECTION('ref_axis',(1.,-1.22464679915E-16,0.));
#46178=DIRECTION('center_axis',(-1.22464679914955E-16,-1.,8.72911003161552E-29));
#46179=DIRECTION('ref_axis',(-0.457271150163836,5.59995650390798E-17,-0.889327327381681));
#46180=DIRECTION('center_axis',(1.22464679915E-16,1.,6.16297582204E-33));
#46181=DIRECTION('ref_axis',(1.,-1.22464679915E-16,-7.54746861370012E-49));
#46182=DIRECTION('center_axis',(1.22464679915E-16,1.,0.));
#46183=DIRECTION('ref_axis',(1.,-1.22464679915E-16,0.));
#46184=DIRECTION('',(-1.26882631386E-16,-1.,0.));
#46185=DIRECTION('center_axis',(-1.22464679915E-16,-1.,-6.16297582204006E-33));
#46186=DIRECTION('ref_axis',(1.,-1.22464679915E-16,-2.89120579329468E-15));
#46187=DIRECTION('center_axis',(-1.22464679915E-16,-1.,0.));
#46188=DIRECTION('ref_axis',(1.,-1.22464679915E-16,0.));
#46189=DIRECTION('',(-2.0185873175E-16,-1.,0.));
#46190=DIRECTION('center_axis',(-1.22464679915E-16,-1.,-1.23259516441E-32));
#46191=DIRECTION('ref_axis',(1.,-1.22464679915E-16,-1.50949372274247E-48));
#46192=DIRECTION('center_axis',(1.,-1.22464679915E-16,6.12323399574E-17));
#46193=DIRECTION('ref_axis',(-1.22464679915E-16,-1.,-6.67366607695787E-50));
#46194=DIRECTION('',(-1.75377892382E-16,0.,1.));
#46195=DIRECTION('',(1.26882631386E-16,1.,0.));
#46196=DIRECTION('',(-2.58629566281E-16,0.,1.));
#46197=DIRECTION('center_axis',(1.22464679914969E-16,1.,-8.28235472972929E-29));
#46198=DIRECTION('ref_axis',(-0.345424032932988,4.23022436279984E-17,-0.938446715307966));
#46199=DIRECTION('center_axis',(0.,1.,0.));
#46200=DIRECTION('ref_axis',(-1.,0.,-3.70074341541717E-15));
#46201=DIRECTION('center_axis',(1.22464679915E-16,1.,4.37905770102E-47));
#46202=DIRECTION('ref_axis',(1.,-1.22464679915E-16,-5.3627989968473E-63));
#46203=DIRECTION('',(1.42793958151E-16,1.,0.));
#46204=DIRECTION('center_axis',(-1.22464679915E-16,-1.,0.));
#46205=DIRECTION('ref_axis',(-1.,1.22464679915E-16,0.));
#46206=DIRECTION('',(0.,-1.,0.));
#46207=DIRECTION('center_axis',(-1.22464679915E-16,-1.,-6.16297582204E-33));
#46208=DIRECTION('ref_axis',(1.,-1.22464679915E-16,-7.54746861370013E-49));
#46209=DIRECTION('center_axis',(-1.53814670812197E-6,0.999999999998278,
-1.03837087347816E-6));
#46210=DIRECTION('ref_axis',(-0.999999999998817,-1.53814670630209E-6,1.76525460915653E-12));
#46211=DIRECTION('center_axis',(-2.17357452795E-16,2.66186108837E-32,1.));
#46212=DIRECTION('ref_axis',(-1.,-5.7857534586223E-48,-2.17357452795E-16));
#46213=DIRECTION('center_axis',(2.31296463464E-16,-2.83256473635E-32,-1.));
#46214=DIRECTION('ref_axis',(1.,6.55162206050593E-48,2.31296463464E-16));
#46215=DIRECTION('center_axis',(4.16333634234E-16,-5.09861652543E-32,-1.));
#46216=DIRECTION('ref_axis',(1.,2.1227255475978E-47,4.16333634234E-16));
#46217=DIRECTION('',(2.0973706922E-16,0.,-1.));
#46218=DIRECTION('center_axis',(1.,0.,0.));
#46219=DIRECTION('ref_axis',(0.,-1.,0.));
#46220=DIRECTION('center_axis',(-0.904759192693671,1.1080104493296E-16,
0.425923471102845));
#46221=DIRECTION('ref_axis',(0.425923471102845,3.65487816993661E-32,0.904759192693671));
#46222=DIRECTION('center_axis',(-1.00248263963544E-16,-1.,4.71927656598494E-17));
#46223=DIRECTION('ref_axis',(-0.425923471102846,0.,-0.904759192693671));
#46224=DIRECTION('center_axis',(-0.916786704663777,1.12273990336973E-16,
0.399377187820903));
#46225=DIRECTION('ref_axis',(0.399377187820903,3.93858763528754E-32,0.916786704663777));
#46226=DIRECTION('center_axis',(1.22464679915E-16,1.,5.47382212627E-48));
#46227=DIRECTION('ref_axis',(1.,-1.22464679915E-16,-6.703498746053E-64));
#46228=DIRECTION('center_axis',(0.,0.,1.));
#46229=DIRECTION('ref_axis',(1.,0.,0.));
#46230=DIRECTION('center_axis',(-2.17357452795E-16,2.66186108837E-32,1.));
#46231=DIRECTION('ref_axis',(1.,5.7857534586223E-48,2.17357452795E-16));
#46232=DIRECTION('center_axis',(-2.17357452795E-16,2.66186108835898E-32,
1.));
#46233=DIRECTION('ref_axis',(-5.78575345859834E-48,-1.,2.66186108835898E-32));
#46234=DIRECTION('center_axis',(-2.17357452795E-16,2.66186108837E-32,1.));
#46235=DIRECTION('ref_axis',(1.,5.7857534586223E-48,2.17357452795E-16));
#46236=DIRECTION('',(0.,0.,1.));
#46237=DIRECTION('center_axis',(-1.07341775839004E-45,-1.,-3.62568286252829E-31));
#46238=DIRECTION('ref_axis',(-1.,0.,3.94745964311167E-15));
#46239=DIRECTION('center_axis',(-0.938446715307966,1.14926576606996E-16,
0.345424032932987));
#46240=DIRECTION('ref_axis',(0.345424032932987,5.96953449650393E-32,0.938446715307966));
#46241=DIRECTION('center_axis',(1.22464679915E-16,1.,5.47382212627E-48));
#46242=DIRECTION('ref_axis',(1.,-1.22464679915E-16,-6.703498746053E-64));
#46243=DIRECTION('center_axis',(1.22464679915E-16,1.,3.08148791102E-33));
#46244=DIRECTION('ref_axis',(1.,-1.22464679915E-16,-3.77373430685006E-49));
#46245=DIRECTION('center_axis',(-1.07852468318872E-16,-1.,3.96984015829353E-17));
#46246=DIRECTION('ref_axis',(-0.345424032932988,0.,-0.938446715307966));
#46247=DIRECTION('center_axis',(1.22464679915E-16,1.,5.47382212627E-48));
#46248=DIRECTION('ref_axis',(1.,-1.22464679915E-16,6.22660996643423E-64));
#46249=DIRECTION('center_axis',(1.22464679915E-16,1.,5.47382212627E-48));
#46250=DIRECTION('ref_axis',(1.,-1.22464679915E-16,5.9677926224237E-64));
#46251=DIRECTION('center_axis',(0.,0.,1.));
#46252=DIRECTION('ref_axis',(1.,0.,0.));
#46253=DIRECTION('center_axis',(0.927477365469186,-1.13583218690023E-16,
-0.373879307454075));
#46254=DIRECTION('ref_axis',(0.373879307454075,-5.54912062383212E-32,0.927477365469186));
#46255=DIRECTION('center_axis',(1.22464679915E-16,1.,3.08148791102E-33));
#46256=DIRECTION('ref_axis',(1.,-1.22464679915E-16,-3.77373430685006E-49));
#46257=DIRECTION('center_axis',(-1.0534586443266E-16,-1.,4.2466415142443E-17));
#46258=DIRECTION('ref_axis',(-0.373879307454075,0.,-0.927477365469186));
#46259=DIRECTION('center_axis',(-1.22464679915E-16,-1.,-5.47382212627E-48));
#46260=DIRECTION('ref_axis',(1.,-1.22464679915E-16,5.24998673990483E-64));
#46261=DIRECTION('center_axis',(-1.22464679915E-16,-1.,-5.47382212627E-48));
#46262=DIRECTION('ref_axis',(1.,-1.22464679915E-16,5.02845536814161E-64));
#46263=DIRECTION('center_axis',(-1.22464679915E-16,-1.,-5.47382212627E-48));
#46264=DIRECTION('ref_axis',(-1.,1.22464679915E-16,0.));
#46265=DIRECTION('center_axis',(0.687199008140201,-8.41576065696246E-17,
0.726469216974212));
#46266=DIRECTION('ref_axis',(0.726469216974212,1.50838013754883E-32,-0.687199008140201));
#46267=DIRECTION('center_axis',(0.687199008140272,-9.99737898630458E-14,
0.726469216974145));
#46268=DIRECTION('ref_axis',(-4.37797946043856E-12,1.,4.27898457407615E-12));
#46269=DIRECTION('',(0.687199008140201,0.,0.726469216974212));
#46270=DIRECTION('',(0.687199008140201,0.,0.726469216974212));
#46271=DIRECTION('center_axis',(1.68490994230906E-17,1.,4.21844451941189E-17));
#46272=DIRECTION('ref_axis',(0.928663912412966,0.,-0.370922279974987));
#46273=DIRECTION('center_axis',(1.22464679915E-16,1.,5.47382212627E-48));
#46274=DIRECTION('ref_axis',(1.,-1.22464679915E-16,-6.703498746053E-64));
#46275=DIRECTION('center_axis',(-0.151695779270758,-1.70262634961358E-12,
0.988427230782033));
#46276=DIRECTION('ref_axis',(5.62512999143433E-12,1.,2.58589446152285E-12));
#46277=DIRECTION('center_axis',(1.22464679915E-16,1.,5.47382212627E-48));
#46278=DIRECTION('ref_axis',(1.,-1.22464679915E-16,-6.703498746053E-64));
#46279=DIRECTION('center_axis',(1.,-1.22464679915E-16,6.12323399574E-17));
#46280=DIRECTION('ref_axis',(1.22464679915E-16,1.,7.49879891332945E-33));
#46281=DIRECTION('',(-1.,0.,-2.9545627326E-16));
#46282=DIRECTION('',(-1.,0.,-2.21592204945E-16));
#46283=DIRECTION('center_axis',(2.41898181523141E-16,1.,-1.1741867647411E-17));
#46284=DIRECTION('ref_axis',(0.99520202856178,-2.41886400693281E-16,-0.0978413120645785));
#46285=DIRECTION('center_axis',(-1.22464679915E-16,-1.,-5.47382212627E-48));
#46286=DIRECTION('ref_axis',(1.,-1.22464679915E-16,6.49622071350503E-64));
#46287=DIRECTION('center_axis',(-0.256628500559793,-5.7981162678719E-12,
0.966510120330063));
#46288=DIRECTION('ref_axis',(-0.966510120330063,0.,-0.256628500559793));
#46289=DIRECTION('center_axis',(-1.22464679915E-16,-1.,-5.47382212627E-48));
#46290=DIRECTION('ref_axis',(1.,-1.22464679915E-16,6.22660996643423E-64));
#46291=DIRECTION('center_axis',(0.,1.,0.));
#46292=DIRECTION('ref_axis',(-0.0129687405446048,0.,-0.999915902348136));
#46293=DIRECTION('center_axis',(-1.22464679915E-16,-1.,1.23259516441E-32));
#46294=DIRECTION('ref_axis',(1.,-1.22464679915E-16,1.50949372274247E-48));
#46295=DIRECTION('center_axis',(-0.726469216974212,8.89668201247259E-17,
0.687199008140201));
#46296=DIRECTION('ref_axis',(1.22464679914833E-16,1.,-2.7960247294612E-34));
#46297=DIRECTION('',(0.,1.,0.));
#46298=DIRECTION('',(0.,-1.,0.));
#46299=DIRECTION('',(0.687199008140201,0.,0.726469216974212));
#46300=DIRECTION('center_axis',(0.,0.,1.));
#46301=DIRECTION('ref_axis',(1.,0.,0.));
#46302=DIRECTION('center_axis',(1.22464679915E-16,1.,-1.23259516441E-32));
#46303=DIRECTION('ref_axis',(1.,-1.22464679915E-16,1.50949372274247E-48));
#46304=DIRECTION('center_axis',(-1.22464679914998E-16,-1.,-1.73663083545565E-29));
#46305=DIRECTION('ref_axis',(-0.095298509688002,1.16707014853003E-17,0.99544874004202));
#46306=DIRECTION('',(0.,1.,0.));
#46307=DIRECTION('',(0.,1.,0.));
#46308=DIRECTION('center_axis',(1.22464679915E-16,1.,-6.16297582204E-33));
#46309=DIRECTION('ref_axis',(1.,-1.22464679915E-16,7.54746861370013E-49));
#46310=DIRECTION('center_axis',(0.,0.,1.));
#46311=DIRECTION('ref_axis',(1.,0.,0.));
#46312=DIRECTION('center_axis',(1.22464679915E-16,1.,3.08148791102E-33));
#46313=DIRECTION('ref_axis',(1.,-1.22464679915E-16,-3.77373430685006E-49));
#46314=DIRECTION('center_axis',(-2.17357452795E-16,2.66186108837E-32,1.));
#46315=DIRECTION('ref_axis',(1.,2.56447231488414E-65,2.17357452795E-16));
#46316=DIRECTION('',(-1.,0.,-4.75520106567E-17));
#46317=DIRECTION('',(0.,-1.,0.));
#46318=DIRECTION('',(0.,1.,0.));
#46319=DIRECTION('center_axis',(0.,1.,0.));
#46320=DIRECTION('ref_axis',(-0.79266275948672,0.,0.609660356036784));
#46321=DIRECTION('center_axis',(-1.22464679915E-16,-1.,0.));
#46322=DIRECTION('ref_axis',(1.,-1.22464679915E-16,0.));
#46323=DIRECTION('center_axis',(-1.22464679914586E-16,-1.,-1.3947821589454E-28));
#46324=DIRECTION('ref_axis',(-0.947590338356885,1.16046347476986E-16,0.319487950715961));
#46325=DIRECTION('center_axis',(-1.22464679915E-16,-1.,0.));
#46326=DIRECTION('ref_axis',(1.,-1.22464679915E-16,0.));
#46327=DIRECTION('',(0.,-1.,0.));
#46328=DIRECTION('',(0.,-1.,0.));
#46329=DIRECTION('center_axis',(-1.22464679914811E-16,-1.,1.69678707944837E-28));
#46330=DIRECTION('ref_axis',(-0.744047562132924,9.11195465378906E-17,-0.668126653624934));
#46331=DIRECTION('center_axis',(-1.22464679915E-16,-1.,0.));
#46332=DIRECTION('ref_axis',(1.,-1.22464679915E-16,0.));
#46333=DIRECTION('center_axis',(0.687199008140201,-8.41576065696246E-17,
0.726469216974212));
#46334=DIRECTION('ref_axis',(-0.726469216974212,-1.50838013754883E-32,0.687199008140201));
#46335=DIRECTION('center_axis',(0.687199008140201,-8.41576065696246E-17,
0.726469216974212));
#46336=DIRECTION('ref_axis',(0.726469216974212,1.50838013754883E-32,-0.687199008140201));
#46337=DIRECTION('',(0.687199008140201,0.,0.726469216974212));
#46338=DIRECTION('center_axis',(0.687199008140201,-8.41576065696246E-17,
0.726469216974212));
#46339=DIRECTION('ref_axis',(0.726469216974212,1.50838013754883E-32,-0.687199008140201));
#46340=DIRECTION('center_axis',(-1.22464679914912E-16,-1.,-8.35596805204809E-29));
#46341=DIRECTION('ref_axis',(0.726469216974212,-8.89668201247259E-17,-0.687199008140201));
#46342=DIRECTION('center_axis',(-1.22464679915E-16,-1.,0.));
#46343=DIRECTION('ref_axis',(1.,-1.22464679915E-16,0.));
#46344=DIRECTION('center_axis',(-2.81810938552877E-18,-1.,1.83623833789471E-17));
#46345=DIRECTION('ref_axis',(-0.988427230781696,0.,-0.151695779272953));
#46346=DIRECTION('center_axis',(-0.656401557320037,8.03860066128046E-17,
0.754411688369043));
#46347=DIRECTION('ref_axis',(0.754411688369043,7.40115717670054E-32,0.656401557320037));
#46348=DIRECTION('center_axis',(1.22464679915E-16,1.,5.47382212627E-48));
#46349=DIRECTION('ref_axis',(1.,-1.22464679915E-16,-6.703498746053E-64));
#46350=DIRECTION('center_axis',(-0.151695779272953,1.85773750529943E-17,
0.988427230781696));
#46351=DIRECTION('ref_axis',(0.988427230781695,3.4608594993322E-33,0.151695779272953));
#46352=DIRECTION('center_axis',(1.22464679915E-16,1.,4.31748667364107E-33));
#46353=DIRECTION('ref_axis',(-5.28739623524732E-49,-4.31748667364107E-33,
1.));
#46354=DIRECTION('center_axis',(-1.22464679915E-16,-1.,-3.08148791102E-33));
#46355=DIRECTION('ref_axis',(1.,-1.22464679915E-16,-3.77373430685006E-49));
#46356=DIRECTION('center_axis',(1.,-1.22464679915E-16,6.12323399574E-17));
#46357=DIRECTION('ref_axis',(-1.22464679915E-16,-1.,-7.49879891332945E-33));
#46358=DIRECTION('center_axis',(-1.,1.22464679915E-16,-6.16173778667E-15));
#46359=DIRECTION('ref_axis',(1.22464679915E-16,1.,7.54595245764702E-31));
#46360=DIRECTION('',(-1.,0.,-1.4772813663E-16));
#46361=DIRECTION('center_axis',(-1.,1.22464679915E-16,-5.92731269866E-14));
#46362=DIRECTION('ref_axis',(1.22464679915E-16,1.,7.25886452397512E-30));
#46363=DIRECTION('center_axis',(1.22464679914936E-16,1.,-1.70680191515918E-29));
#46364=DIRECTION('ref_axis',(-0.966510120331627,1.18363352520954E-16,-0.2566285005539));
#46365=DIRECTION('center_axis',(-1.22464679915E-16,-1.,7.00649232162E-46));
#46366=DIRECTION('ref_axis',(1.,-1.22464679915E-16,8.58047839494098E-62));
#46367=DIRECTION('center_axis',(-8.06530182705333E-18,-1.,3.03754096780024E-17));
#46368=DIRECTION('ref_axis',(-0.966510120331627,0.,-0.256628500553901));
#46369=DIRECTION('center_axis',(0.256628500553901,-3.14279271772879E-17,
-0.966510120331627));
#46370=DIRECTION('ref_axis',(0.966510120331627,1.90417037848503E-32,0.256628500553901));
#46371=DIRECTION('center_axis',(-1.22464679915E-16,-1.,-5.47382212627E-48));
#46372=DIRECTION('ref_axis',(1.,-1.22464679915E-16,5.9677926224237E-64));
#46373=DIRECTION('center_axis',(0.668126653624933,-8.18219167786918E-17,
-0.744047562132925));
#46374=DIRECTION('ref_axis',(0.744047562132925,-1.50412683502806E-31,0.668126653624933));
#46375=DIRECTION('center_axis',(-5.46674034506358E-17,-1.,6.0879397708352E-17));
#46376=DIRECTION('ref_axis',(-0.744047562132925,0.,-0.668126653624934));
#46377=DIRECTION('center_axis',(-1.22464679915E-16,-1.,-5.47382212627E-48));
#46378=DIRECTION('ref_axis',(1.,-1.22464679915E-16,-6.703498746053E-64));
#46379=DIRECTION('center_axis',(0.,1.,0.));
#46380=DIRECTION('ref_axis',(-0.997344825668515,0.,0.0728237510173635));
#46381=DIRECTION('center_axis',(0.734238830876792,-8.99183234042744E-17,
-0.678891257295808));
#46382=DIRECTION('ref_axis',(0.678891257295808,1.51038693775819E-31,0.734238830876792));
#46383=DIRECTION('center_axis',(-0.825067330468845,1.01041606533981E-16,
-0.565034423900893));
#46384=DIRECTION('ref_axis',(0.565034423900893,7.24547600115018E-32,-0.825067330468845));
#46385=DIRECTION('center_axis',(1.22464679915E-16,1.,-1.23259516441E-32));
#46386=DIRECTION('ref_axis',(1.,-1.22464679915E-16,1.50949372274247E-48));
#46387=DIRECTION('center_axis',(-5.78330237622164E-17,-1.,-6.11379105471829E-17));
#46388=DIRECTION('ref_axis',(0.726469216974212,0.,-0.687199008140201));
#46389=DIRECTION('center_axis',(-1.22464679915E-16,-1.,-5.47382212627E-48));
#46390=DIRECTION('ref_axis',(1.,-1.22464679915E-16,-6.703498746053E-64));
#46391=DIRECTION('center_axis',(-2.81810938552877E-18,-1.,1.83623833789471E-17));
#46392=DIRECTION('ref_axis',(0.988427230781696,0.,0.151695779272954));
#46393=DIRECTION('center_axis',(-1.22464679915E-16,-1.,-5.47382212627E-48));
#46394=DIRECTION('ref_axis',(1.,-1.22464679915E-16,-6.703498746053E-64));
#46395=DIRECTION('center_axis',(-1.22464679915E-16,-1.,-6.16366086630911E-30));
#46396=DIRECTION('ref_axis',(-4.93432455388959E-14,0.,1.));
#46397=DIRECTION('center_axis',(-1.22464679915E-16,-1.,-5.47382212627E-48));
#46398=DIRECTION('ref_axis',(1.,-1.22464679915E-16,-6.703498746053E-64));
#46399=DIRECTION('center_axis',(-1.22464679915E-16,-1.,0.));
#46400=DIRECTION('ref_axis',(1.,-1.22464679915E-16,0.));
#46401=DIRECTION('center_axis',(-1.13563209349214E-16,-1.,3.17943322838876E-17));
#46402=DIRECTION('ref_axis',(-0.269603455472075,0.,-0.962971430935268));
#46403=DIRECTION('center_axis',(-1.22464679915E-16,-1.,-5.47382212627E-48));
#46404=DIRECTION('ref_axis',(1.,-1.22464679915E-16,-6.703498746053E-64));
#46405=DIRECTION('center_axis',(-0.962971430935267,1.17929988057033E-16,
0.269603455472075));
#46406=DIRECTION('ref_axis',(0.269603455472075,3.05583905676118E-32,0.962971430935268));
#46407=DIRECTION('center_axis',(-1.22464679915E-16,-1.,-5.47382212627E-48));
#46408=DIRECTION('ref_axis',(1.,-1.22464679915E-16,-6.703498746053E-64));
#46409=DIRECTION('center_axis',(1.22464679915E-16,1.,5.47382212627E-48));
#46410=DIRECTION('ref_axis',(1.,-1.22464679915E-16,0.));
#46411=DIRECTION('center_axis',(0.,0.,-1.));
#46412=DIRECTION('ref_axis',(-0.707106778693304,0.707106783679791,0.));
#46413=DIRECTION('center_axis',(-7.24819500366175E-17,-1.,6.01900799944532E-17));
#46414=DIRECTION('ref_axis',(-0.638858327474962,0.,-0.769324403236954));
#46415=DIRECTION('center_axis',(-1.22464679915E-16,-1.,-5.47382212627E-48));
#46416=DIRECTION('ref_axis',(1.,-1.22464679915E-16,6.22660996643423E-64));
#46417=DIRECTION('center_axis',(0.769324403236954,-9.42150667929943E-17,
-0.638858327474961));
#46418=DIRECTION('ref_axis',(0.638858327474961,7.17307849792281E-32,0.769324403236954));
#46419=DIRECTION('center_axis',(-1.22464679915E-16,-1.,-5.47382212627E-48));
#46420=DIRECTION('ref_axis',(1.,-1.22464679915E-16,5.9677926224237E-64));
#46421=DIRECTION('center_axis',(1.2246467991498E-16,1.,4.9218209689896E-29));
#46422=DIRECTION('ref_axis',(0.382683432365114,-4.6865204053314E-17,-0.923879532511277));
#46423=DIRECTION('center_axis',(1.22464679915E-16,1.,6.16297582204E-33));
#46424=DIRECTION('ref_axis',(1.,-1.22464679915E-16,-7.54746861370013E-49));
#46425=DIRECTION('',(-1.24169680386E-16,-1.,0.));
#46426=DIRECTION('center_axis',(-1.22464679915E-16,-1.,0.));
#46427=DIRECTION('ref_axis',(1.,-1.22464679915E-16,0.));
#46428=DIRECTION('center_axis',(0.382683432365114,-4.6865204053314E-17,
0.923879532511277));
#46429=DIRECTION('ref_axis',(-1.22464679914861E-16,-1.,3.33030126354153E-33));
#46430=DIRECTION('',(-1.66950830771E-16,-1.,0.));
#46431=DIRECTION('',(0.923879532511277,-1.79771717893054E-16,-0.382683432365114));
#46432=DIRECTION('',(-0.923879532511277,1.79771717893054E-16,0.382683432365114));
#46433=DIRECTION('center_axis',(-1.22464679914969E-16,-1.,1.40937670198757E-28));
#46434=DIRECTION('ref_axis',(-0.215815367394074,2.64297598885091E-17,-0.976434189895336));
#46435=DIRECTION('',(0.,1.,0.));
#46436=DIRECTION('center_axis',(0.,1.,5.04725420579478E-11));
#46437=DIRECTION('ref_axis',(-0.215814054939841,4.92832405001852E-11,-0.976434479978264));
#46438=DIRECTION('center_axis',(1.22464679914995E-16,1.,-2.84643200354157E-29));
#46439=DIRECTION('ref_axis',(-0.175818770215043,2.15315894174053E-17,-0.984422551570244));
#46440=DIRECTION('center_axis',(-1.22464679915E-16,-1.,-3.08148791102E-33));
#46441=DIRECTION('ref_axis',(1.,-1.22464679915E-16,2.83076871527624E-49));
#46442=DIRECTION('center_axis',(-0.978784588777817,-0.0498161334628422,
0.198743758689054));
#46443=DIRECTION('ref_axis',(0.194346018843094,0.0814603510708595,0.9775448000799));
#46444=DIRECTION('',(0.,-1.,0.));
#46445=DIRECTION('center_axis',(1.22464679915E-16,1.,3.08148791102E-33));
#46446=DIRECTION('ref_axis',(1.,-1.22464679915E-16,2.83076871527624E-49));
#46447=DIRECTION('',(0.,1.,0.));
#46448=DIRECTION('center_axis',(1.22464679915E-16,1.,-1.23259516441E-32));
#46449=DIRECTION('ref_axis',(1.,-1.22464679915E-16,-1.13230748611233E-48));
#46450=DIRECTION('',(0.,-1.,0.));
#46451=DIRECTION('center_axis',(1.22464679915E-16,1.,-6.16297582204E-33));
#46452=DIRECTION('ref_axis',(1.,-1.22464679915E-16,-5.66153743055249E-49));
#46453=DIRECTION('center_axis',(1.2246467991498E-16,1.,4.9218209689896E-29));
#46454=DIRECTION('ref_axis',(-0.382683432365115,4.68652040533141E-17,0.923879532511276));
#46455=DIRECTION('center_axis',(1.22464679915E-16,1.,-6.16297582204E-33));
#46456=DIRECTION('ref_axis',(1.,-1.22464679915E-16,7.54746861370013E-49));
#46457=DIRECTION('center_axis',(-1.22464679915E-16,-1.,-6.16297582204E-33));
#46458=DIRECTION('ref_axis',(1.,-1.22464679915E-16,-7.54746861370013E-49));
#46459=DIRECTION('',(-1.24169680386E-16,-1.,0.));
#46460=DIRECTION('center_axis',(0.382683432365114,-4.68652040533141E-17,
-0.923879532511277));
#46461=DIRECTION('ref_axis',(2.5429740769239E-34,-1.,5.07265313324192E-17));
#46462=DIRECTION('',(-0.923879532511277,1.79771717893054E-16,-0.382683432365114));
#46463=DIRECTION('center_axis',(0.382683432331542,-3.85987976375918E-9,
-0.923879532525183));
#46464=DIRECTION('ref_axis',(0.906907964349175,0.19079395606161,0.375653577821903));
#46465=DIRECTION('',(-1.66950830771E-16,-1.,0.));
#46466=DIRECTION('',(0.923879532511277,-1.79771717893054E-16,0.382683432365114));
#46467=DIRECTION('center_axis',(1.22464679915019E-16,1.,-7.85779417309992E-30));
#46468=DIRECTION('ref_axis',(-0.923879532511277,1.13142611229034E-16,0.382683432365114));
#46469=DIRECTION('center_axis',(1.22464679915E-16,1.,-6.16297582204E-33));
#46470=DIRECTION('ref_axis',(1.,-1.22464679915E-16,7.54746861370013E-49));
#46471=DIRECTION('',(-1.16865581539E-16,-1.,0.));
#46472=DIRECTION('center_axis',(0.923879532511277,-1.13142611229034E-16,
-0.382683432365114));
#46473=DIRECTION('ref_axis',(-1.31021084567677E-32,-1.,2.95655891162504E-16));
#46474=DIRECTION('center_axis',(0.923879532544053,-1.41481107281946E-8,
-0.382683432285984));
#46475=DIRECTION('ref_axis',(0.376061245770244,-0.185228919800991,0.907892166889378));
#46476=DIRECTION('',(-0.382683432365114,0.,-0.923879532511277));
#46477=DIRECTION('center_axis',(0.923879532507688,-2.76759523330007E-9,
-0.382683432373779));
#46478=DIRECTION('ref_axis',(0.375653574352959,0.190794018963353,0.906907952552881));
#46479=DIRECTION('',(0.,-1.,0.));
#46480=DIRECTION('',(0.382683432365114,0.,0.923879532511277));
#46481=DIRECTION('center_axis',(1.22464679915019E-16,1.,7.86635386174164E-30));
#46482=DIRECTION('ref_axis',(-0.923879532511276,1.13142611229034E-16,-0.382683432365115));
#46483=DIRECTION('center_axis',(1.22464679915E-16,1.,6.16297582204E-33));
#46484=DIRECTION('ref_axis',(1.,-1.22464679915E-16,-7.54746861370013E-49));
#46485=DIRECTION('',(-2.33731163079E-16,-1.,0.));
#46486=DIRECTION('center_axis',(0.923879532511277,-1.13142611229034E-16,
0.382683432365114));
#46487=DIRECTION('ref_axis',(-1.31021084567677E-32,-1.,-2.95655891162504E-16));
#46488=DIRECTION('',(0.382683432365114,0.,-0.923879532511277));
#46489=DIRECTION('',(-1.66950830771E-16,-1.,0.));
#46490=DIRECTION('',(-0.382683432365114,0.,0.923879532511277));
#46491=DIRECTION('center_axis',(1.2246467991498E-16,1.,-4.9218209689896E-29));
#46492=DIRECTION('ref_axis',(-0.382683432365114,4.6865204053314E-17,-0.923879532511277));
#46493=DIRECTION('center_axis',(1.22464679915E-16,1.,6.16297582204E-33));
#46494=DIRECTION('ref_axis',(1.,-1.22464679915E-16,-7.54746861370013E-49));
#46495=DIRECTION('center_axis',(-1.22464679915E-16,-1.,0.));
#46496=DIRECTION('ref_axis',(1.,-1.22464679915E-16,0.));
#46497=DIRECTION('center_axis',(0.766057840542209,-0.255399249832434,0.589853039433415));
#46498=DIRECTION('ref_axis',(-0.202361789893946,-0.966835675378721,-0.155815540963958));
#46499=DIRECTION('center_axis',(-1.22464679915E-16,-1.,0.));
#46500=DIRECTION('ref_axis',(1.,-1.22464679915E-16,0.));
#46501=DIRECTION('center_axis',(-0.792335098973394,9.70330642810483E-17,
-0.610086134029304));
#46502=DIRECTION('ref_axis',(0.610086134029304,5.05601228850744E-32,-0.792335098973394));
#46503=DIRECTION('center_axis',(-7.68827025909336E-17,-1.,-5.91985270603321E-17));
#46504=DIRECTION('ref_axis',(-0.610086134029304,0.,0.792335098973394));
#46505=DIRECTION('center_axis',(-1.22464679915E-16,-1.,-5.47382212627E-48));
#46506=DIRECTION('ref_axis',(1.,-1.22464679915E-16,5.40238148608971E-64));
#46507=DIRECTION('center_axis',(-0.611236674075818,7.48549036428777E-17,
-0.791447868317764));
#46508=DIRECTION('ref_axis',(0.791447868317764,-7.00049973634741E-32,-0.611236674075818));
#46509=DIRECTION('center_axis',(-1.22464679914949E-16,-1.,-1.08530702891677E-28));
#46510=DIRECTION('ref_axis',(2.12313165367255E-16,-1.08554598373815E-28,
1.));
#46511=DIRECTION('center_axis',(1.22464679915E-16,1.,0.));
#46512=DIRECTION('ref_axis',(1.,-1.22464679915E-16,0.));
#46513=DIRECTION('',(0.,-1.,0.));
#46514=DIRECTION('',(0.,-1.,0.));
#46515=DIRECTION('center_axis',(1.22464679915E-16,1.,1.54074395551E-33));
#46516=DIRECTION('ref_axis',(1.,-1.22464679915E-16,1.52063520297906E-49));
#46517=DIRECTION('center_axis',(-1.22464679915E-16,-1.,0.));
#46518=DIRECTION('ref_axis',(1.,-1.22464679915E-16,0.));
#46519=DIRECTION('',(-1.03939138974E-16,-1.,0.));
#46520=DIRECTION('center_axis',(1.22464679914914E-16,1.,1.11943608056428E-28));
#46521=DIRECTION('ref_axis',(-0.610086134029304,7.47140031243373E-17,0.792335098973394));
#46522=DIRECTION('center_axis',(0.,-1.,0.));
#46523=DIRECTION('ref_axis',(-0.610086133998045,0.,0.792335098997463));
#46524=DIRECTION('',(0.,-1.,0.));
#46525=DIRECTION('center_axis',(0.678891257295808,-8.31402005216763E-17,
0.734238830876792));
#46526=DIRECTION('ref_axis',(-1.22464679914784E-16,-1.,1.83887638005312E-34));
#46527=DIRECTION('',(0.734238830876791,0.,-0.678891257295807));
#46528=DIRECTION('',(0.,-1.,0.));
#46529=DIRECTION('',(-0.734238830876792,0.,0.678891257295808));
#46530=DIRECTION('',(0.,-1.,0.));
#46531=DIRECTION('center_axis',(-0.678891257318237,7.43492351073594E-12,
-0.734238830856053));
#46532=DIRECTION('ref_axis',(-1.46208970879984E-10,-1.,1.25062923000865E-10));
#46533=DIRECTION('',(-0.734238830876792,0.,0.678891257295808));
#46534=DIRECTION('center_axis',(1.22464679914942E-16,1.,7.54279763108459E-29));
#46535=DIRECTION('ref_axis',(0.612227349738988,-7.49762264208985E-17,-0.790681776842982));
#46536=DIRECTION('center_axis',(-1.22464679915E-16,-1.,0.));
#46537=DIRECTION('ref_axis',(1.,-1.22464679915E-16,0.));
#46538=DIRECTION('',(0.,-1.,0.));
#46539=DIRECTION('center_axis',(1.22464679915E-16,1.,-6.16297582204E-33));
#46540=DIRECTION('ref_axis',(1.,-1.22464679915E-16,7.54746861370013E-49));
#46541=DIRECTION('center_axis',(-1.22464679914998E-16,-1.,-1.73663083545565E-29));
#46542=DIRECTION('ref_axis',(-0.095298509688002,1.16707014853003E-17,0.99544874004202));
#46543=DIRECTION('',(-1.32169407693E-16,-1.,0.));
#46544=DIRECTION('center_axis',(-1.22464679915E-16,-1.,6.16297582204E-33));
#46545=DIRECTION('ref_axis',(1.,-1.22464679915E-16,7.54746861370013E-49));
#46546=DIRECTION('center_axis',(1.22464679915E-16,1.,0.));
#46547=DIRECTION('ref_axis',(1.,-1.22464679915E-16,0.));
#46548=DIRECTION('center_axis',(1.22464679915E-16,1.,7.60253073092891E-48));
#46549=DIRECTION('ref_axis',(1.,-1.22464679915E-16,-9.3104149250716E-64));
#46550=DIRECTION('center_axis',(-1.22464679915E-16,-1.,3.08148791102E-33));
#46551=DIRECTION('ref_axis',(1.,-1.22464679915E-16,3.77373430685006E-49));
#46552=DIRECTION('',(-1.23358113847E-16,-1.,0.));
#46553=DIRECTION('center_axis',(1.22464679915E-16,1.,0.));
#46554=DIRECTION('ref_axis',(1.,-1.22464679915E-16,0.));
#46555=DIRECTION('center_axis',(-1.,1.22464679915E-16,-6.12323399574E-17));
#46556=DIRECTION('ref_axis',(-6.12323399574E-17,0.,1.));
#46557=DIRECTION('',(-1.32169407693E-16,-1.,0.));
#46558=DIRECTION('',(2.19188076492E-16,0.,-1.));
#46559=DIRECTION('',(-2.17106560191E-16,0.,1.));
#46560=DIRECTION('center_axis',(-1.22464679914917E-16,-1.,-1.21085355525786E-28));
#46561=DIRECTION('ref_axis',(-0.566106835688783,6.93280924301735E-17,0.824331881335687));
#46562=DIRECTION('center_axis',(1.22464679915E-16,1.,0.));
#46563=DIRECTION('ref_axis',(1.,-1.22464679915E-16,0.));
#46564=DIRECTION('',(0.,-1.,0.));
#46565=DIRECTION('center_axis',(-1.22464679915E-16,-1.,1.54074395550985E-33));
#46566=DIRECTION('ref_axis',(1.,-1.22464679915E-16,-5.78241158658936E-15));
#46567=DIRECTION('center_axis',(-1.22464679915E-16,-1.,0.));
#46568=DIRECTION('ref_axis',(1.,-1.22464679915E-16,0.));
#46569=DIRECTION('',(-1.04083408559E-16,-1.,0.));
#46570=DIRECTION('center_axis',(1.22464679915E-16,1.,0.));
#46571=DIRECTION('ref_axis',(1.,-1.22464679915E-16,0.));
#46572=DIRECTION('center_axis',(-1.22464679914999E-16,-1.,-1.9442368107527E-29));
#46573=DIRECTION('ref_axis',(-0.0510637267514752,6.25350295186696E-18,0.998695396910515));
#46574=DIRECTION('center_axis',(-1.22464679915E-16,-1.,1.54074395551E-33));
#46575=DIRECTION('ref_axis',(1.,-1.22464679915E-16,-1.75263489528827E-49));
#46576=DIRECTION('center_axis',(1.22464679915E-16,1.,-1.23259516441E-32));
#46577=DIRECTION('ref_axis',(1.,-1.22464679915E-16,-1.40210791623289E-48));
#46578=DIRECTION('center_axis',(-2.17357452795E-16,2.66186108837E-32,1.));
#46579=DIRECTION('ref_axis',(-1.,-5.7857534586223E-48,-2.17357452795E-16));
#46580=DIRECTION('center_axis',(-1.78560869794E-14,2.18673997646E-30,1.));
#46581=DIRECTION('ref_axis',(1.,1.11272749077955E-45,1.78560869794E-14));
#46582=DIRECTION('',(-8.96394535471E-17,0.,1.));
#46583=DIRECTION('center_axis',(1.6065913575E-14,-1.96750696351E-30,1.));
#46584=DIRECTION('ref_axis',(1.,-2.52100835352406E-45,-1.6065913575E-14));
#46585=DIRECTION('',(-8.96394535471E-17,0.,1.));
#46586=DIRECTION('center_axis',(-1.17989839311979E-16,-1.,-2.29779399358865E-17));
#46587=DIRECTION('ref_axis',(-0.191153986297934,0.,0.981560061087659));
#46588=DIRECTION('center_axis',(-0.981560061087659,1.20206438697958E-16,
-0.191153986297933));
#46589=DIRECTION('ref_axis',(0.191153986297933,-8.55574366268044E-33,-0.981560061087659));
#46590=DIRECTION('center_axis',(-1.22464679915E-16,-1.,-5.47382212627E-48));
#46591=DIRECTION('ref_axis',(1.,-1.22464679915E-16,-6.703498746053E-64));
#46592=DIRECTION('center_axis',(-0.973274002238674,1.1919168915396E-16,
-0.229646938943923));
#46593=DIRECTION('ref_axis',(0.229646938943923,-2.91124363913666E-32,-0.973274002238674));
#46594=DIRECTION('center_axis',(-1.22464679915E-16,-1.,-5.47382212627E-48));
#46595=DIRECTION('ref_axis',(1.,-1.22464679915E-16,-6.703498746053E-64));
#46596=DIRECTION('center_axis',(-1.17989839311979E-16,-1.,-2.29779399358865E-17));
#46597=DIRECTION('ref_axis',(0.191153986297933,0.,-0.981560061087659));
#46598=DIRECTION('center_axis',(2.17357452795E-16,-2.66186108837E-32,-1.));
#46599=DIRECTION('ref_axis',(1.,5.7857534586223E-48,2.17357452795E-16));
#46600=DIRECTION('center_axis',(1.22464679915E-16,1.,3.08148791102E-33));
#46601=DIRECTION('ref_axis',(1.,-1.22464679915E-16,-3.77373430685006E-49));
#46602=DIRECTION('center_axis',(1.22464679915E-16,1.,5.47382212627E-48));
#46603=DIRECTION('ref_axis',(1.,-1.22464679915E-16,-6.703498746053E-64));
#46604=DIRECTION('center_axis',(2.17357452795E-16,-2.66186108836821E-32,
-1.));
#46605=DIRECTION('ref_axis',(-5.78575345861839E-48,-1.,2.66186108836821E-32));
#46606=DIRECTION('center_axis',(-5.70383201187E-15,6.98517961621E-31,-1.));
#46607=DIRECTION('ref_axis',(1.,-5.48892443580096E-47,-5.70383201187E-15));
#46608=DIRECTION('',(7.61796550883E-17,0.,-1.));
#46609=DIRECTION('',(5.71347413162E-17,0.,-1.));
#46610=DIRECTION('center_axis',(-4.29367103357466E-45,-1.,-7.25136572506882E-31));
#46611=DIRECTION('ref_axis',(1.,0.,-5.9211894646675E-15));
#46612=DIRECTION('center_axis',(0.984869499718035,-1.20611728041004E-16,
0.173297629889006));
#46613=DIRECTION('ref_axis',(0.173297629889006,5.41148511020646E-32,-0.984869499718035));
#46614=DIRECTION('center_axis',(1.22464679915E-16,1.,-3.08148791102E-33));
#46615=DIRECTION('ref_axis',(1.,-1.22464679915E-16,3.77373430685006E-49));
#46616=DIRECTION('center_axis',(1.22464679915E-16,1.,5.47382212627E-48));
#46617=DIRECTION('ref_axis',(1.,-1.22464679915E-16,-6.703498746053E-64));
#46618=DIRECTION('center_axis',(-1.18786812255882E-16,-1.,-2.09017266063253E-17));
#46619=DIRECTION('ref_axis',(-0.173297629889006,0.,0.984869499718035));
#46620=DIRECTION('center_axis',(0.825067330468845,-1.01041606533981E-16,
0.565034423900893));
#46621=DIRECTION('ref_axis',(0.565034423900893,7.24547600115018E-32,-0.825067330468845));
#46622=DIRECTION('center_axis',(1.22464679915E-16,1.,5.47382212627E-48));
#46623=DIRECTION('ref_axis',(1.,-1.22464679915E-16,-6.703498746053E-64));
#46624=DIRECTION('center_axis',(1.22464679915E-16,1.,5.47382212627E-48));
#46625=DIRECTION('ref_axis',(1.,-1.22464679915E-16,-6.703498746053E-64));
#46626=DIRECTION('center_axis',(-6.60215246509141E-17,-1.,6.10447636300053E-17));
#46627=DIRECTION('ref_axis',(-0.678891257295808,0.,-0.734238830876792));
#46628=DIRECTION('center_axis',(1.22464679915E-16,1.,-1.23259516441E-32));
#46629=DIRECTION('ref_axis',(1.,-1.22464679915E-16,1.50949372274247E-48));
#46630=DIRECTION('center_axis',(-0.734238830876792,8.99183234042744E-17,
0.678891257295808));
#46631=DIRECTION('ref_axis',(0.678891257295808,-2.24691316591619E-32,0.734238830876792));
#46632=DIRECTION('center_axis',(1.22464679915E-16,1.,5.47382212627E-48));
#46633=DIRECTION('ref_axis',(1.,-1.22464679915E-16,-6.703498746053E-64));
#46634=DIRECTION('center_axis',(-8.3366128569448E-17,-1.,-5.70919859380671E-17));
#46635=DIRECTION('ref_axis',(-0.565034423900894,0.,0.825067330468845));
#46636=DIRECTION('center_axis',(-0.734238830876792,8.99183234042744E-17,
0.678891257295808));
#46637=DIRECTION('ref_axis',(0.678891257295808,-2.24691316591619E-32,0.734238830876792));
#46638=DIRECTION('center_axis',(1.22464679915E-16,1.,-1.23259516441E-32));
#46639=DIRECTION('ref_axis',(1.,-1.22464679915E-16,1.50949372274247E-48));
#46640=DIRECTION('center_axis',(1.22464679915E-16,1.,5.47382212627E-48));
#46641=DIRECTION('ref_axis',(1.,-1.22464679915E-16,-6.703498746053E-64));
#46642=DIRECTION('center_axis',(-0.734238830876792,8.99183234044499E-17,
0.678891257295808));
#46643=DIRECTION('ref_axis',(-6.60215246508846E-17,-1.,6.1044763629978E-17));
#46644=DIRECTION('',(-0.734238830876791,0.,0.678891257295807));
#46645=DIRECTION('',(-0.734238830876791,0.,0.678891257295807));
#46646=DIRECTION('center_axis',(-5.11601622893148E-18,-1.,2.45021972047681E-17));
#46647=DIRECTION('ref_axis',(-0.978889450967439,0.,-0.204390417546091));
#46648=DIRECTION('center_axis',(0.204390417546092,-2.50306070625112E-17,
-0.978889450967439));
#46649=DIRECTION('ref_axis',(0.978889450967439,-1.05289930055147E-32,0.204390417546092));
#46650=DIRECTION('center_axis',(-1.22464679915E-16,-1.,-5.47382212627E-48));
#46651=DIRECTION('ref_axis',(1.,-1.22464679915E-16,-6.703498746053E-64));
#46652=DIRECTION('center_axis',(0.419584599500152,-5.13842936749187E-17,
-0.90771623531933));
#46653=DIRECTION('ref_axis',(0.90771623531933,-2.72267697829008E-32,0.419584599500152));
#46654=DIRECTION('center_axis',(-1.22464679915E-16,-1.,-5.47382212627E-48));
#46655=DIRECTION('ref_axis',(1.,-1.22464679915E-16,-6.703498746053E-64));
#46656=DIRECTION('center_axis',(0.382636981165606,-0.0155797766458367,-0.923767401029143));
#46657=DIRECTION('ref_axis',(0.670813900451024,0.692209394753623,0.266185771175894));
#46658=DIRECTION('center_axis',(0.382683425383291,2.34479170719746E-9,-0.923879535403242));
#46659=DIRECTION('ref_axis',(0.653279884842593,0.70710851193395,0.270597384338069));
#46660=DIRECTION('center_axis',(-2.15600582822439E-17,-1.,4.66423576092589E-17));
#46661=DIRECTION('ref_axis',(-0.90771623531933,0.,-0.419584599500153));
#46662=DIRECTION('center_axis',(-0.0335155327516907,4.10446899060886E-18,
0.999438196720723));
#46663=DIRECTION('ref_axis',(0.999438196720723,5.21239906410075E-34,0.0335155327516907));
#46664=DIRECTION('center_axis',(-1.22464679915E-16,-1.,0.));
#46665=DIRECTION('ref_axis',(1.,-1.22464679915E-16,0.));
#46666=DIRECTION('center_axis',(-1.22464679915E-16,-1.,-5.47382212627E-48));
#46667=DIRECTION('ref_axis',(1.,-1.22464679915E-16,-6.703498746053E-64));
#46668=DIRECTION('center_axis',(-0.382683432388042,2.52266547895476E-11,
-0.92387953250178));
#46669=DIRECTION('ref_axis',(0.653281506872114,0.707106754739568,-0.270598060193668));
#46670=DIRECTION('center_axis',(0.854119591553195,0.0486596199953837,-0.517795292279593));
#46671=DIRECTION('ref_axis',(0.492492289235195,0.244264035758894,0.835336115511986));
#46672=DIRECTION('center_axis',(-0.382579843714528,0.0232740187023026,-0.923629245550839));
#46673=DIRECTION('ref_axis',(0.679149393449658,0.684858194219679,-0.264055591092333));
#46674=DIRECTION('center_axis',(0.382579759521302,-0.0232739793740044,-0.923629281415829));
#46675=DIRECTION('ref_axis',(0.679152682329405,0.684854387074657,0.264057006325091));
#46676=DIRECTION('center_axis',(-5.06268119967007E-18,-1.,-2.43796819441885E-17));
#46677=DIRECTION('ref_axis',(-0.979111878581668,0.,0.203322230019931));
#46678=DIRECTION('center_axis',(1.22464679915E-16,1.,5.47382212627E-48));
#46679=DIRECTION('ref_axis',(1.,-1.22464679915E-16,-6.703498746053E-64));
#46680=DIRECTION('center_axis',(0.203322230019931,-2.48997918188915E-17,
0.979111878581668));
#46681=DIRECTION('ref_axis',(0.979111878581668,-1.33094098597294E-33,-0.203322230019931));
#46682=DIRECTION('center_axis',(1.22464679915E-16,1.,5.47382212627E-48));
#46683=DIRECTION('ref_axis',(1.,-1.22464679915E-16,-6.703498746053E-64));
#46684=DIRECTION('center_axis',(-1.22464679915E-16,-1.,0.));
#46685=DIRECTION('ref_axis',(0.,0.,1.));
#46686=DIRECTION('center_axis',(-1.,1.22464679915E-16,-6.12323399574E-17));
#46687=DIRECTION('ref_axis',(-1.22464679915E-16,-1.,-7.49879891332945E-33));
#46688=DIRECTION('center_axis',(-1.22464679915E-16,-1.,-5.47382212627E-48));
#46689=DIRECTION('ref_axis',(1.,-1.22464679915E-16,-6.703498746053E-64));
#46690=DIRECTION('center_axis',(-1.22464679915E-16,-1.,-5.47382212627E-48));
#46691=DIRECTION('ref_axis',(1.,-1.22464679915E-16,-6.703498746053E-64));
#46692=DIRECTION('center_axis',(-5.06268119967007E-18,-1.,-2.43796819441885E-17));
#46693=DIRECTION('ref_axis',(0.979111878581668,0.,-0.203322230019931));
#46694=DIRECTION('center_axis',(-1.22464679915E-16,-1.,-5.47382212627E-48));
#46695=DIRECTION('ref_axis',(1.,-1.22464679915E-16,-6.703498746053E-64));
#46696=DIRECTION('center_axis',(-1.,1.22464679915E-16,-6.12323399574E-17));
#46697=DIRECTION('ref_axis',(-1.22464679915E-16,-1.,-7.49879891332945E-33));
#46698=DIRECTION('center_axis',(-1.22464679915E-16,-1.,-6.16297582204E-33));
#46699=DIRECTION('ref_axis',(1.,-1.22464679915E-16,-7.54746861370013E-49));
#46700=DIRECTION('center_axis',(-1.,1.22464679915E-16,-6.12323399574E-17));
#46701=DIRECTION('ref_axis',(6.12323399574E-17,-7.49879891332945E-33,-1.));
#46702=DIRECTION('',(-1.,0.,0.));
#46703=DIRECTION('',(-1.,0.,0.));
#46704=DIRECTION('center_axis',(-0.923879532523066,-2.50321061818283E-11,
-0.382683432336653));
#46705=DIRECTION('ref_axis',(0.270598059367657,0.707106756803419,-0.653281504980363));
#46706=DIRECTION('center_axis',(0.237817192548205,0.0486596292822717,-0.970090317138874));
#46707=DIRECTION('ref_axis',(0.938916649716559,0.244263330956247,0.242427205641592));
#46708=DIRECTION('center_axis',(-0.923629304634498,0.0232740186304629,-0.382579701078328));
#46709=DIRECTION('ref_axis',(0.293515644570473,0.684858188071701,-0.666946646009654));
#46710=DIRECTION('center_axis',(-0.38257978588401,-0.0232739793753114,-0.923629270496005));
#46711=DIRECTION('ref_axis',(0.66694996580489,0.684854388356,-0.293516966907172));
#46712=DIRECTION('center_axis',(0.970089609818427,0.0486732638221455,-0.237817287662678));
#46713=DIRECTION('ref_axis',(0.242486471652566,-0.239688973466001,0.940079521670536));
#46714=DIRECTION('center_axis',(-0.382683509132997,3.37979830178284E-8,
-0.923879500712974));
#46715=DIRECTION('ref_axis',(0.653293893777471,0.707093332555111,-0.27060322874862));
#46716=DIRECTION('center_axis',(-7.79403475186991E-17,-1.,-5.89087594505755E-17));
#46717=DIRECTION('ref_axis',(-0.602966636474875,0.,0.797766403966835));
#46718=DIRECTION('center_axis',(-1.22464679915E-16,-1.,-5.47382212627E-48));
#46719=DIRECTION('ref_axis',(1.,-1.22464679915E-16,-6.703498746053E-64));
#46720=DIRECTION('center_axis',(-0.797766403966835,9.76982073084798E-17,
-0.602966636474875));
#46721=DIRECTION('ref_axis',(0.602966636474875,6.43171104150991E-32,-0.797766403966835));
#46722=DIRECTION('center_axis',(-1.22464679915E-16,-1.,-5.47382212627E-48));
#46723=DIRECTION('ref_axis',(1.,-1.22464679915E-16,-6.703498746053E-64));
#46724=DIRECTION('center_axis',(-0.585630202615096,7.17190153117117E-17,
-0.810578352650132));
#46725=DIRECTION('ref_axis',(0.810578352650132,6.4321265031143E-32,-0.585630202615096));
#46726=DIRECTION('center_axis',(-1.22464679915E-16,-1.,-5.47382212627E-48));
#46727=DIRECTION('ref_axis',(1.,-1.22464679915E-16,-6.703498746053E-64));
#46728=DIRECTION('center_axis',(-7.79403475186991E-17,-1.,-5.89087594505755E-17));
#46729=DIRECTION('ref_axis',(0.602966636474876,0.,-0.797766403966835));
#46730=DIRECTION('center_axis',(0.734238830876792,-8.99183234042744E-17,
-0.678891257295808));
#46731=DIRECTION('ref_axis',(0.678891257295808,-2.24691316591619E-32,0.734238830876792));
#46732=DIRECTION('center_axis',(1.22464679915E-16,1.,0.));
#46733=DIRECTION('ref_axis',(1.,-1.22464679915E-16,0.));
#46734=DIRECTION('center_axis',(1.22464679915E-16,1.,5.47382212627E-48));
#46735=DIRECTION('ref_axis',(1.,-1.22464679915E-16,-6.703498746053E-64));
#46736=DIRECTION('center_axis',(-0.734238830876792,8.99183234042744E-17,
0.678891257295808));
#46737=DIRECTION('ref_axis',(-0.678891257295808,-1.51038693775819E-31,-0.734238830876792));
#46738=DIRECTION('center_axis',(0.73423883087825,-8.99183234044306E-17,
-0.678891257294231));
#46739=DIRECTION('ref_axis',(0.678891257294231,1.10716302178481E-31,0.73423883087825));
#46740=DIRECTION('',(0.734238830876791,0.,-0.678891257295807));
#46741=DIRECTION('',(0.734238830876791,0.,-0.678891257295807));
#46742=DIRECTION('center_axis',(-6.60215246511763E-17,-1.,6.10447636299848E-17));
#46743=DIRECTION('ref_axis',(0.678891257294231,0.,0.73423883087825));
#46744=DIRECTION('center_axis',(0.581646529321033,-7.12311560368041E-17,
0.813441648140047));
#46745=DIRECTION('ref_axis',(0.813441648140047,-2.80119922649672E-32,-0.581646529321033));
#46746=DIRECTION('center_axis',(1.22464679915E-16,1.,-1.23259516441E-32));
#46747=DIRECTION('ref_axis',(1.,-1.22464679915E-16,1.50949372274247E-48));
#46748=DIRECTION('center_axis',(1.22464679915E-16,1.,5.47382212627E-48));
#46749=DIRECTION('ref_axis',(1.,-1.22464679915E-16,-6.703498746053E-64));
#46750=DIRECTION('center_axis',(-4.14313546884292E-17,-1.,-5.79423889656346E-17));
#46751=DIRECTION('ref_axis',(-0.813441648140047,0.,0.581646529321034));
#46752=DIRECTION('center_axis',(0.142980079684983,-1.75100096927979E-17,
0.98972556641388));
#46753=DIRECTION('ref_axis',(0.98972556641388,3.23015489124122E-33,-0.142980079684983));
#46754=DIRECTION('center_axis',(1.22464679915E-16,1.,5.47382212627E-48));
#46755=DIRECTION('ref_axis',(1.,-1.22464679915E-16,-6.703498746053E-64));
#46756=DIRECTION('center_axis',(1.22464679915E-16,1.,5.47382212627E-48));
#46757=DIRECTION('ref_axis',(1.,-1.22464679915E-16,-6.703498746053E-64));
#46758=DIRECTION('center_axis',(-1.22464679915E-16,-1.,0.));
#46759=DIRECTION('ref_axis',(0.,0.,-1.));
#46760=DIRECTION('center_axis',(1.22464679915E-16,1.,5.47382212627E-48));
#46761=DIRECTION('ref_axis',(1.,-1.22464679915E-16,-6.703498746053E-64));
#46762=DIRECTION('center_axis',(-1.,1.22464679915E-16,-6.12323399574E-17));
#46763=DIRECTION('ref_axis',(-1.22464679915E-16,-1.,-7.49879891332945E-33));
#46764=DIRECTION('center_axis',(1.22464679915E-16,1.,5.47382212627E-48));
#46765=DIRECTION('ref_axis',(1.,-1.22464679915E-16,-6.703498746053E-64));
#46766=DIRECTION('center_axis',(-2.50358258116745E-18,-1.,-1.73301042611612E-17));
#46767=DIRECTION('ref_axis',(-0.98972556641388,0.,0.142980079684983));
#46768=DIRECTION('center_axis',(-1.,1.22464679915E-16,-6.12323399574E-17));
#46769=DIRECTION('ref_axis',(-1.22464679915E-16,-1.,-7.49879891332945E-33));
#46770=DIRECTION('center_axis',(1.22464679915E-16,1.,5.47382212627E-48));
#46771=DIRECTION('ref_axis',(1.,-1.22464679915E-16,-6.703498746053E-64));
#46772=DIRECTION('center_axis',(1.22464679915E-16,1.,5.47382212627E-48));
#46773=DIRECTION('ref_axis',(1.,-1.22464679915E-16,-6.703498746053E-64));
#46774=DIRECTION('center_axis',(-1.,1.22464679915E-16,-6.12323399574E-17));
#46775=DIRECTION('ref_axis',(-1.22464679915E-16,-1.,-7.49879891332945E-33));
#46776=DIRECTION('',(-1.,0.,-2.89652532403E-16));
#46777=DIRECTION('',(-1.,0.,-2.89652532403E-16));
#46778=DIRECTION('center_axis',(-0.734238830876792,8.99183234042744E-17,
0.678891257295808));
#46779=DIRECTION('ref_axis',(0.678891257295808,-2.24691316591619E-32,0.734238830876792));
#46780=DIRECTION('',(-0.734238830876791,0.,0.678891257295807));
#46781=DIRECTION('',(-0.734238830876791,0.,0.678891257295807));
#46782=DIRECTION('center_axis',(-0.734238830876792,8.991832340449E-17,0.678891257295808));
#46783=DIRECTION('ref_axis',(6.6021524650914E-17,1.,-6.10447636300053E-17));
#46784=DIRECTION('',(0.734238830876791,0.,-0.678891257295807));
#46785=DIRECTION('center_axis',(0.734238830881096,6.3373930704663E-12,-0.678891257291153));
#46786=DIRECTION('ref_axis',(6.40968759550252E-12,1.,1.62684680541738E-11));
#46787=DIRECTION('',(0.734238830876791,0.,-0.678891257295807));
#46788=DIRECTION('center_axis',(1.69872863391202E-17,1.,4.23293596334453E-17));
#46789=DIRECTION('ref_axis',(0.928056183869048,0.,-0.37244022283102));
#46790=DIRECTION('center_axis',(1.22464679915E-16,1.,5.47382212627E-48));
#46791=DIRECTION('ref_axis',(1.,-1.22464679915E-16,-6.703498746053E-64));
#46792=DIRECTION('center_axis',(1.22464679915E-16,1.,5.47382212627E-48));
#46793=DIRECTION('ref_axis',(1.,-1.22464679915E-16,-6.703498746053E-64));
#46794=DIRECTION('center_axis',(0.,1.,0.));
#46795=DIRECTION('ref_axis',(0.231145326606897,0.,-0.972919235079557));
#46796=DIRECTION('center_axis',(-0.0335155327516907,4.10446899060886E-18,
0.999438196720723));
#46797=DIRECTION('ref_axis',(0.999438196720723,5.21239906410075E-34,0.0335155327516907));
#46798=DIRECTION('center_axis',(1.22464679915E-16,1.,0.));
#46799=DIRECTION('ref_axis',(1.,-1.22464679915E-16,0.));
#46800=DIRECTION('center_axis',(5.9296278727138E-17,1.,6.12017248415691E-17));
#46801=DIRECTION('ref_axis',(0.718198537785833,0.,-0.695838242928838));
#46802=DIRECTION('center_axis',(-1.22464679915E-16,-1.,-5.47382212627E-48));
#46803=DIRECTION('ref_axis',(1.,-1.22464679915E-16,-6.703498746053E-64));
#46804=DIRECTION('center_axis',(-1.22464679915E-16,-1.,-5.47382212627E-48));
#46805=DIRECTION('ref_axis',(1.,-1.22464679915E-16,-6.703498746053E-64));
#46806=DIRECTION('center_axis',(0.,1.,0.));
#46807=DIRECTION('ref_axis',(-0.776012376688289,0.,0.630717679494236));
#46808=DIRECTION('center_axis',(-1.,1.22464679915E-16,-6.12323399574E-17));
#46809=DIRECTION('ref_axis',(-1.22464679915E-16,-1.,-7.49879891332945E-33));
#46810=DIRECTION('center_axis',(1.22464679915E-16,1.,5.47382212627E-48));
#46811=DIRECTION('ref_axis',(1.,-1.22464679915E-16,-6.703498746053E-64));
#46812=DIRECTION('center_axis',(0.,0.,1.));
#46813=DIRECTION('ref_axis',(1.,0.,0.));
#46814=DIRECTION('center_axis',(-1.,1.22464679915E-16,-6.12323399574E-17));
#46815=DIRECTION('ref_axis',(-1.22464679915E-16,-1.,-7.49879891332945E-33));
#46816=DIRECTION('center_axis',(1.22464679915E-16,1.,6.16297582204E-33));
#46817=DIRECTION('ref_axis',(1.,-1.22464679915E-16,-7.54746861370013E-49));
#46818=DIRECTION('center_axis',(0.,1.,0.));
#46819=DIRECTION('ref_axis',(0.998774211147154,0.,-0.0494982337804088));
#46820=DIRECTION('center_axis',(-0.797766403966835,9.76982073084798E-17,
-0.602966636474875));
#46821=DIRECTION('ref_axis',(0.602966636474875,6.43171104150991E-32,-0.797766403966835));
#46822=DIRECTION('center_axis',(-1.22464679915E-16,-1.,0.));
#46823=DIRECTION('ref_axis',(1.,-1.22464679915E-16,0.));
#46824=DIRECTION('center_axis',(-1.,1.22464679915E-16,-6.12323399574E-17));
#46825=DIRECTION('ref_axis',(-6.12323399574E-17,7.49879891332945E-33,1.));
#46826=DIRECTION('',(1.,0.,4.09734305096E-16));
#46827=DIRECTION('',(1.,0.,0.));
#46828=DIRECTION('center_axis',(5.9296278727138E-17,1.,6.12017248415691E-17));
#46829=DIRECTION('ref_axis',(-0.714690181301574,0.,0.699441166039806));
#46830=DIRECTION('center_axis',(1.22464679915E-16,1.,5.47382212627E-48));
#46831=DIRECTION('ref_axis',(1.,-1.22464679915E-16,-6.703498746053E-64));
#46832=DIRECTION('center_axis',(1.22464679915E-16,1.,5.47382212627E-48));
#46833=DIRECTION('ref_axis',(1.,-1.22464679915E-16,-6.703498746053E-64));
#46834=DIRECTION('center_axis',(-2.68354439599323E-46,-1.,1.81284143127026E-31));
#46835=DIRECTION('ref_axis',(1.,0.,1.97372982155583E-15));
#46836=DIRECTION('center_axis',(-1.22464679915E-16,-1.,-5.47382212627E-48));
#46837=DIRECTION('ref_axis',(1.,-1.22464679915E-16,-6.703498746053E-64));
#46838=DIRECTION('center_axis',(-0.991694064582439,1.21447496192053E-16,
0.128619136492057));
#46839=DIRECTION('ref_axis',(0.128619136492057,-7.10548517584315E-33,0.991694064582438));
#46840=DIRECTION('center_axis',(-1.22464679915E-16,-1.,-5.47382212627E-48));
#46841=DIRECTION('ref_axis',(1.,-1.22464679915E-16,-6.703498746053E-64));
#46842=DIRECTION('center_axis',(-8.38660245249135E-17,-1.,5.68956569482564E-17));
#46843=DIRECTION('ref_axis',(-0.561410669601872,0.,-0.827537346623811));
#46844=DIRECTION('center_axis',(1.22464679915E-16,1.,5.47382212627E-48));
#46845=DIRECTION('ref_axis',(1.,-1.22464679915E-16,-6.703498746053E-64));
#46846=DIRECTION('center_axis',(-0.827537346623811,1.01344096271977E-16,
0.561410669601872));
#46847=DIRECTION('ref_axis',(0.561410669601872,-5.47362952277333E-32,0.827537346623811));
#46848=DIRECTION('center_axis',(1.22464679915E-16,1.,5.47382212627E-48));
#46849=DIRECTION('ref_axis',(1.,-1.22464679915E-16,-6.703498746053E-64));
#46850=DIRECTION('center_axis',(-5.78330237622164E-17,-1.,-6.11379105471829E-17));
#46851=DIRECTION('ref_axis',(-0.726469216974212,0.,0.687199008140201));
#46852=DIRECTION('center_axis',(-0.687199008140201,8.41576065696246E-17,
-0.726469216974212));
#46853=DIRECTION('ref_axis',(0.726469216974212,1.50838013754883E-32,-0.687199008140201));
#46854=DIRECTION('center_axis',(-1.22464679915E-16,-1.,-5.47382212627E-48));
#46855=DIRECTION('ref_axis',(1.,-1.22464679915E-16,-6.703498746053E-64));
#46856=DIRECTION('center_axis',(-1.22464679915E-16,-1.,0.));
#46857=DIRECTION('ref_axis',(1.,-1.22464679915E-16,0.));
#46858=DIRECTION('center_axis',(-8.38660245249135E-17,-1.,5.68956569482564E-17));
#46859=DIRECTION('ref_axis',(0.561410669601872,0.,0.827537346623811));
#46860=DIRECTION('center_axis',(-1.22464679915E-16,-1.,-5.47382212627E-48));
#46861=DIRECTION('ref_axis',(1.,-1.22464679915E-16,-6.703498746053E-64));
#46862=DIRECTION('center_axis',(-0.687199008140201,8.41576065696246E-17,
-0.726469216974212));
#46863=DIRECTION('ref_axis',(0.726469216974212,1.50838013754883E-32,-0.687199008140201));
#46864=DIRECTION('center_axis',(-1.22464679915E-16,-1.,1.23259516441E-32));
#46865=DIRECTION('ref_axis',(1.,-1.22464679915E-16,1.50949372274247E-48));
#46866=DIRECTION('center_axis',(1.,0.,0.));
#46867=DIRECTION('ref_axis',(0.,-1.,0.));
#46868=DIRECTION('center_axis',(0.973274002238674,-1.1919168915396E-16,
0.229646938943923));
#46869=DIRECTION('ref_axis',(0.229646938943923,-2.91124363913666E-32,-0.973274002238674));
#46870=DIRECTION('center_axis',(1.22464679915E-16,1.,-1.23259516441E-32));
#46871=DIRECTION('ref_axis',(1.,-1.22464679915E-16,1.50949372274247E-48));
#46872=DIRECTION('center_axis',(1.22464679914982E-16,1.,7.00298942658309E-29));
#46873=DIRECTION('ref_axis',(0.246934184763054,-3.02407158970066E-17,-0.969032253537211));
#46874=DIRECTION('center_axis',(-1.81298926929756E-20,-0.999999999999994,
1.08984439787114E-7));
#46875=DIRECTION('ref_axis',(0.246934184762501,-1.0560943675131E-7,-0.969032253537346));
#46876=DIRECTION('',(-1.22066246076E-16,-1.,0.));
#46877=DIRECTION('center_axis',(-1.22464679914958E-16,-1.,1.38940690218481E-28));
#46878=DIRECTION('ref_axis',(-0.287097106361984,3.51592552349981E-17,-0.957901483200948));
#46879=DIRECTION('',(-1.13288063737E-16,-1.,0.));
#46880=DIRECTION('center_axis',(1.22464679915E-16,1.,0.));
#46881=DIRECTION('ref_axis',(1.,-1.22464679915E-16,0.));
#46882=DIRECTION('center_axis',(0.,0.,1.));
#46883=DIRECTION('ref_axis',(1.,0.,0.));
#46884=DIRECTION('center_axis',(1.22464679915E-16,1.,0.));
#46885=DIRECTION('ref_axis',(1.,-1.22464679915E-16,0.));
#46886=DIRECTION('center_axis',(1.16436507708486E-16,1.,-2.6493382562289E-17));
#46887=DIRECTION('ref_axis',(-0.221864286407976,0.,-0.975077555077892));
#46888=DIRECTION('center_axis',(1.22464679915E-16,1.,5.47382212627E-48));
#46889=DIRECTION('ref_axis',(1.,-1.22464679915E-16,-6.703498746053E-64));
#46890=DIRECTION('center_axis',(-1.22464679915E-16,-1.,-7.60253073092891E-48));
#46891=DIRECTION('ref_axis',(-1.,1.22464679915E-16,9.3104149250716E-64));
#46892=DIRECTION('center_axis',(1.22464679915E-16,1.,-4.37905770102E-47));
#46893=DIRECTION('ref_axis',(1.,-1.22464679915E-16,5.3627989968473E-63));
#46894=DIRECTION('',(0.,1.,0.));
#46895=DIRECTION('center_axis',(-1.22464679915E-16,-1.,-6.16297582204E-33));
#46896=DIRECTION('ref_axis',(1.,-1.22464679915E-16,-7.54746861370013E-49));
#46897=DIRECTION('',(0.,1.,0.));
#46898=DIRECTION('center_axis',(5.9296278727138E-17,1.,6.12017248415691E-17));
#46899=DIRECTION('ref_axis',(0.718198537785833,0.,-0.695838242928838));
#46900=DIRECTION('center_axis',(1.22464679915E-16,1.,5.47382212627E-48));
#46901=DIRECTION('ref_axis',(1.,-1.22464679915E-16,-6.703498746053E-64));
#46902=DIRECTION('center_axis',(0.981560061088029,-1.66999853996006E-12,
0.191153986296036));
#46903=DIRECTION('ref_axis',(-7.15168665029376E-13,1.,1.24085926718939E-11));
#46904=DIRECTION('center_axis',(1.22464679915E-16,1.,5.47382212627E-48));
#46905=DIRECTION('ref_axis',(1.,-1.22464679915E-16,-6.703498746053E-64));
#46906=DIRECTION('center_axis',(1.22464679915E-16,1.,5.47382212627E-48));
#46907=DIRECTION('ref_axis',(1.,-1.22464679915E-16,0.));
#46908=DIRECTION('center_axis',(-1.22464679915E-16,-1.,6.16297582204E-33));
#46909=DIRECTION('ref_axis',(1.,-1.22464679915E-16,7.54746861370013E-49));
#46910=DIRECTION('center_axis',(1.22464679915E-16,1.,-1.23259516441E-32));
#46911=DIRECTION('ref_axis',(1.,-1.22464679915E-16,-1.1821919162786E-48));
#46912=DIRECTION('center_axis',(-2.24037888703029E-16,-1.,2.20413632410453E-17));
#46913=DIRECTION('ref_axis',(-0.977255721664238,2.19472257881379E-16,0.212064269679052));
#46914=DIRECTION('center_axis',(-0.458332816460024,1.75137682135009E-14,
0.888780641866047));
#46915=DIRECTION('ref_axis',(0.888780641866047,1.15648231731787E-14,0.458332816460024));
#46916=DIRECTION('center_axis',(0.212064269679051,-2.59703829076063E-17,
0.977255721664238));
#46917=DIRECTION('ref_axis',(0.977255721664238,-7.13089940857179E-32,-0.212064269679051));
#46918=DIRECTION('center_axis',(1.22464679915E-16,1.,5.47382212627E-48));
#46919=DIRECTION('ref_axis',(1.,-1.22464679915E-16,5.24998673990483E-64));
#46920=DIRECTION('center_axis',(-1.17653265936146E-16,-1.,-2.37924056871716E-17));
#46921=DIRECTION('ref_axis',(-0.198212453337067,0.,0.980159080630334));
#46922=DIRECTION('center_axis',(0.611236780892201,-7.48549167240244E-17,
0.791447785823259));
#46923=DIRECTION('ref_axis',(0.79144778582326,2.17825094235712E-31,-0.611236780892201));
#46924=DIRECTION('center_axis',(0.980159080630334,5.57379143139189E-15,
0.198212453337067));
#46925=DIRECTION('ref_axis',(0.198212453337067,-2.31296463463575E-14,-0.980159080630334));
#46926=DIRECTION('center_axis',(1.22464679915E-16,1.,5.47382212627E-48));
#46927=DIRECTION('ref_axis',(1.,-1.22464679915E-16,5.63840144221543E-64));
#46928=DIRECTION('center_axis',(-0.923879532511277,1.13142611229034E-16,
-0.382683432365114));
#46929=DIRECTION('ref_axis',(-0.382683432365114,-7.46986778962313E-32,0.923879532511277));
#46930=DIRECTION('center_axis',(-0.923879532511277,1.13142611229034E-16,
-0.382683432365115));
#46931=DIRECTION('ref_axis',(0.382683432365115,-2.77240367868488E-33,-0.923879532511276));
#46932=DIRECTION('',(-0.923879532511277,0.,-0.382683432365114));
#46933=DIRECTION('center_axis',(-0.923879532511277,1.13142611229034E-16,
-0.382683432365115));
#46934=DIRECTION('ref_axis',(0.382683432365115,2.61659610287296E-32,-0.923879532511276));
#46935=DIRECTION('center_axis',(0.923879532511277,-1.13142611229034E-16,
-0.382683432365114));
#46936=DIRECTION('ref_axis',(-0.382683432365114,-7.46986778962313E-32,-0.923879532511277));
#46937=DIRECTION('center_axis',(0.923879532511277,-1.13142611229034E-16,
-0.382683432365115));
#46938=DIRECTION('ref_axis',(0.382683432365115,2.61659610287296E-32,0.923879532511276));
#46939=DIRECTION('',(0.923879532511277,0.,-0.382683432365114));
#46940=DIRECTION('center_axis',(0.923879532511277,-1.13142611229034E-16,
-0.382683432365115));
#46941=DIRECTION('ref_axis',(0.382683432365115,-2.77240367868488E-33,0.923879532511276));
#46942=DIRECTION('center_axis',(-1.79345371456341E-17,-1.,4.32978028118705E-17));
#46943=DIRECTION('ref_axis',(0.923879532511277,0.,0.382683432365114));
#46944=DIRECTION('center_axis',(1.22464679915E-16,1.,5.47382212627E-48));
#46945=DIRECTION('ref_axis',(1.,-1.22464679915E-16,-6.703498746053E-64));
#46946=DIRECTION('center_axis',(0.382683432365114,-4.6865204053314E-17,
-0.923879532511277));
#46947=DIRECTION('ref_axis',(0.923879532511277,-1.59663321827302E-32,0.382683432365114));
#46948=DIRECTION('center_axis',(0.382683432365114,-4.6865204053314E-17,
-0.923879532511277));
#46949=DIRECTION('ref_axis',(-0.923879532511277,1.59663321827302E-32,-0.382683432365114));
#46950=DIRECTION('',(0.382683432365114,0.,-0.923879532511277));
#46951=DIRECTION('center_axis',(0.382683432365114,-4.6865204053314E-17,
-0.923879532511277));
#46952=DIRECTION('ref_axis',(0.923879532511277,-1.59663321827302E-32,0.382683432365114));
#46953=DIRECTION('center_axis',(-1.79345371456341E-17,-1.,-4.32978028118705E-17));
#46954=DIRECTION('ref_axis',(0.923879532511276,0.,-0.382683432365115));
#46955=DIRECTION('center_axis',(1.22464679915E-16,1.,5.47382212627E-48));
#46956=DIRECTION('ref_axis',(1.,-1.22464679915E-16,-6.703498746053E-64));
#46957=DIRECTION('center_axis',(-0.382683432365114,4.6865204053314E-17,
-0.923879532511277));
#46958=DIRECTION('ref_axis',(0.923879532511277,-1.59663321827302E-32,-0.382683432365114));
#46959=DIRECTION('center_axis',(-0.382683432365114,4.6865204053314E-17,
-0.923879532511277));
#46960=DIRECTION('ref_axis',(-0.923879532511277,1.59663321827302E-32,0.382683432365114));
#46961=DIRECTION('',(-0.382683432365114,0.,-0.923879532511277));
#46962=DIRECTION('center_axis',(-0.382683432365114,4.6865204053314E-17,
-0.923879532511277));
#46963=DIRECTION('ref_axis',(0.923879532511277,-1.59663321827302E-32,-0.382683432365114));
#46964=DIRECTION('center_axis',(-1.04530142769366E-16,-1.,-4.32978028118705E-17));
#46965=DIRECTION('ref_axis',(0.382683432365114,0.,-0.923879532511277));
#46966=DIRECTION('center_axis',(1.22464679915E-16,1.,5.47382212627E-48));
#46967=DIRECTION('ref_axis',(1.,-1.22464679915E-16,-6.703498746053E-64));
#46968=DIRECTION('center_axis',(-1.04530142769366E-16,-1.,4.32978028118705E-17));
#46969=DIRECTION('ref_axis',(-0.382683432365115,0.,-0.923879532511276));
#46970=DIRECTION('center_axis',(1.22464679915E-16,1.,5.47382212627E-48));
#46971=DIRECTION('ref_axis',(1.,-1.22464679915E-16,-6.703498746053E-64));
#46972=DIRECTION('center_axis',(-0.923879532511277,1.13142611229034E-16,
0.382683432365115));
#46973=DIRECTION('ref_axis',(0.382683432365115,2.61659610287296E-32,0.923879532511276));
#46974=DIRECTION('center_axis',(0.923879532511277,-1.13142611229013E-16,
-0.382683432365114));
#46975=DIRECTION('ref_axis',(1.22464679915E-16,1.,4.82508167451141E-31));
#46976=DIRECTION('',(-0.923879532511277,0.,0.382683432365114));
#46977=DIRECTION('center_axis',(-0.923879532511277,1.13142611229034E-16,
0.382683432365115));
#46978=DIRECTION('ref_axis',(0.382683432365115,-2.77240367868488E-33,0.923879532511276));
#46979=DIRECTION('center_axis',(-1.04530142769366E-16,-1.,4.32978028118705E-17));
#46980=DIRECTION('ref_axis',(0.382683432365115,0.,0.923879532511276));
#46981=DIRECTION('center_axis',(0.923879532511277,-1.13142611229034E-16,
0.382683432365115));
#46982=DIRECTION('ref_axis',(0.382683432365115,2.61659610287296E-32,-0.923879532511276));
#46983=DIRECTION('center_axis',(1.22464679915E-16,1.,5.47382212627E-48));
#46984=DIRECTION('ref_axis',(1.,-1.22464679915E-16,-6.703498746053E-64));
#46985=DIRECTION('center_axis',(-0.923879532511277,1.13142611229013E-16,
-0.382683432365114));
#46986=DIRECTION('ref_axis',(1.22464679915E-16,1.,-4.82508167451141E-31));
#46987=DIRECTION('center_axis',(0.923879532511277,-1.13142611229034E-16,
0.382683432365115));
#46988=DIRECTION('ref_axis',(0.382683432365115,-2.77240367868488E-33,-0.923879532511276));
#46989=DIRECTION('',(0.923879532511277,0.,0.382683432365114));
#46990=DIRECTION('center_axis',(-1.04530142769366E-16,-1.,-4.32978028118705E-17));
#46991=DIRECTION('ref_axis',(-0.382683432365114,0.,0.923879532511277));
#46992=DIRECTION('center_axis',(0.382683432365114,-4.6865204053314E-17,
0.923879532511277));
#46993=DIRECTION('ref_axis',(0.923879532511277,-1.59663321827302E-32,-0.382683432365114));
#46994=DIRECTION('center_axis',(1.22464679915E-16,1.,5.47382212627E-48));
#46995=DIRECTION('ref_axis',(1.,-1.22464679915E-16,-6.703498746053E-64));
#46996=DIRECTION('center_axis',(-0.382683432365114,4.68652040533673E-17,
-0.923879532511277));
#46997=DIRECTION('ref_axis',(1.79345371456341E-17,1.,4.32978028118705E-17));
#46998=DIRECTION('center_axis',(0.382683432365114,-4.6865204053314E-17,
0.923879532511277));
#46999=DIRECTION('ref_axis',(0.923879532511277,-1.59663321827302E-32,-0.382683432365114));
#47000=DIRECTION('',(0.382683432365114,0.,0.923879532511277));
#47001=DIRECTION('center_axis',(-1.79345371456341E-17,-1.,-4.32978028118705E-17));
#47002=DIRECTION('ref_axis',(-0.923879532511276,0.,0.382683432365115));
#47003=DIRECTION('center_axis',(-0.382683432365114,4.6865204053314E-17,
0.923879532511277));
#47004=DIRECTION('ref_axis',(0.923879532511277,-1.59663321827302E-32,0.382683432365114));
#47005=DIRECTION('center_axis',(1.22464679915E-16,1.,5.47382212627E-48));
#47006=DIRECTION('ref_axis',(1.,-1.22464679915E-16,-6.703498746053E-64));
#47007=DIRECTION('center_axis',(0.382683432365114,-4.68652040533673E-17,
-0.923879532511277));
#47008=DIRECTION('ref_axis',(1.79345371456341E-17,1.,-4.32978028118705E-17));
#47009=DIRECTION('center_axis',(-0.382683432365114,4.6865204053314E-17,
0.923879532511277));
#47010=DIRECTION('ref_axis',(0.923879532511277,-1.59663321827302E-32,0.382683432365114));
#47011=DIRECTION('',(-0.382683432365114,0.,0.923879532511277));
#47012=DIRECTION('center_axis',(-1.79345371456341E-17,-1.,4.32978028118705E-17));
#47013=DIRECTION('ref_axis',(-0.923879532511277,0.,-0.382683432365114));
#47014=DIRECTION('center_axis',(1.22464679915E-16,1.,5.47382212627E-48));
#47015=DIRECTION('ref_axis',(1.,-1.22464679915E-16,-6.703498746053E-64));
#47016=DIRECTION('center_axis',(-1.22464679915E-16,-1.,-5.47382212627E-48));
#47017=DIRECTION('ref_axis',(-1.,1.22464679915E-16,0.));
#47018=DIRECTION('center_axis',(1.22464679915E-16,1.,-1.23259516441E-32));
#47019=DIRECTION('ref_axis',(1.,-1.22464679915E-16,1.50949372274247E-48));
#47020=DIRECTION('',(-2.1862358377E-16,0.,1.));
#47021=DIRECTION('center_axis',(1.22464679915E-16,1.,-4.37905770102E-47));
#47022=DIRECTION('ref_axis',(1.,-1.22464679915E-16,5.3627989968473E-63));
#47023=DIRECTION('',(1.,0.,0.));
#47024=DIRECTION('center_axis',(1.22464679915E-16,1.,-6.16297582204E-33));
#47025=DIRECTION('ref_axis',(1.,-1.22464679915E-16,-5.9109595813834E-49));
#47026=DIRECTION('center_axis',(1.22464679915E-16,1.,1.23259516441E-32));
#47027=DIRECTION('ref_axis',(1.,-1.22464679915E-16,-1.50949372274247E-48));
#47028=DIRECTION('center_axis',(-2.77602545911041E-17,-1.,5.12739598421612E-17));
#47029=DIRECTION('ref_axis',(-0.879386330848967,0.,-0.476108896278982));
#47030=DIRECTION('center_axis',(-5.0552016865731E-17,-1.,-6.02936991345387E-17));
#47031=DIRECTION('ref_axis',(0.766297237624136,0.,-0.642486220560113));
#47032=DIRECTION('center_axis',(-0.642486220560114,-6.75485423398119E-15,
-0.766297237624136));
#47033=DIRECTION('ref_axis',(0.766297237624136,1.12931390012428E-29,-0.642486220560114));
#47034=DIRECTION('center_axis',(1.22464679915E-16,1.,5.47382212627E-48));
#47035=DIRECTION('ref_axis',(1.,-1.22464679915E-16,-6.703498746053E-64));
#47036=DIRECTION('center_axis',(0.980794227872242,7.97285521065847E-12,
0.195045334659643));
#47037=DIRECTION('ref_axis',(-5.58812255727995E-12,1.,-1.27592381105046E-11));
#47038=DIRECTION('center_axis',(-1.2246467991484E-16,-1.,-6.47882833291866E-29));
#47039=DIRECTION('ref_axis',(-0.926909189979645,1.13513637260957E-16,0.375285695878857));
#47040=DIRECTION('center_axis',(1.9201908781E-16,1.,1.71790773243E-16));
#47041=DIRECTION('ref_axis',(1.,-1.9201908781E-16,-3.29871075722954E-32));
#47042=DIRECTION('',(0.,1.,0.));
#47043=DIRECTION('center_axis',(-4.39408528056178E-8,0.99999999999998,1.96572411306371E-7));
#47044=DIRECTION('ref_axis',(-0.926909250500648,-1.14499965064849E-7,0.375285546399425));
#47045=DIRECTION('center_axis',(-0.103350672077944,-0.961332021496742,-0.255263360132284));
#47046=DIRECTION('ref_axis',(-0.360774156658016,0.275391983262014,-0.891067485347048));
#47047=DIRECTION('center_axis',(-0.375285695878857,4.59592426223824E-17,
-0.926909189979645));
#47048=DIRECTION('ref_axis',(0.926909189979645,-3.61589631838611E-32,-0.375285695878857));
#47049=DIRECTION('center_axis',(-4.57540623410157E-17,-1.,-5.92437539213873E-17));
#47050=DIRECTION('ref_axis',(-0.791447868317764,0.,0.611236674075818));
#47051=DIRECTION('center_axis',(-1.22464679915E-16,-1.,0.));
#47052=DIRECTION('ref_axis',(1.,-1.22464679915E-16,0.));
#47053=DIRECTION('center_axis',(-4.57540783324772E-17,-1.,-5.92437580993829E-17));
#47054=DIRECTION('ref_axis',(-0.791447785823259,0.,0.611236780892201));
#47055=DIRECTION('center_axis',(1.22464679915E-16,1.,0.));
#47056=DIRECTION('ref_axis',(1.,-1.22464679915E-16,0.));
#47057=DIRECTION('center_axis',(1.22464679914331E-16,1.,1.45068233549706E-28));
#47058=DIRECTION('ref_axis',(-0.977255721664238,1.19679309148029E-16,0.212064269679051));
#47059=DIRECTION('center_axis',(6.05558773490554E-7,-0.999999999999779,
-2.73579685865623E-7));
#47060=DIRECTION('ref_axis',(-0.0522365709531267,2.41573864176758E-7,-0.998634738357825));
#47061=DIRECTION('center_axis',(-0.522521046689147,2.55431910633826E-7,
0.852626386975452));
#47062=DIRECTION('ref_axis',(0.602897982970372,0.707106794621592,0.36947801440713));
#47063=DIRECTION('center_axis',(3.34362886570006E-17,1.,-5.45598660992754E-17));
#47064=DIRECTION('ref_axis',(-0.852626520482788,0.,-0.52252082883787));
#47065=DIRECTION('center_axis',(-0.496495443044673,-7.53189665075629E-8,
0.868039328046759));
#47066=DIRECTION('ref_axis',(0.613796700774017,0.707106513896531,0.351075473543833));
#47067=DIRECTION('center_axis',(-4.27856751109758E-7,0.999999999999565,
8.29299678606429E-7));
#47068=DIRECTION('ref_axis',(0.900769699186529,7.45562821397678E-7,-0.434297074623873));
#47069=DIRECTION('center_axis',(-0.707141467397435,0.692946912637,-0.140625464812931));
#47070=DIRECTION('ref_axis',(0.32401455277391,0.140799773673971,-0.935515896884752));
#47071=DIRECTION('center_axis',(1.22464679915E-16,1.,-1.23259516441E-32));
#47072=DIRECTION('ref_axis',(1.,-1.22464679915E-16,1.50949372274247E-48));
#47073=DIRECTION('center_axis',(1.22464679914984E-16,1.,7.84281471797691E-29));
#47074=DIRECTION('ref_axis',(0.195045334687923,-2.38861644813906E-17,-0.980794227866618));
#47075=DIRECTION('',(0.,1.,0.));
#47076=DIRECTION('center_axis',(-1.22464679914868E-16,-1.,-1.10428543166843E-28));
#47077=DIRECTION('ref_axis',(-0.766297237624135,9.38443459252164E-17,0.642486220560115));
#47078=DIRECTION('center_axis',(-2.20517453689E-16,-1.,-1.1694814189E-16));
#47079=DIRECTION('ref_axis',(1.,-2.20517453689E-16,-2.57891064632427E-32));
#47080=DIRECTION('',(0.,-1.,0.));
#47081=DIRECTION('center_axis',(1.,-1.22464679915E-16,6.12323399574E-17));
#47082=DIRECTION('ref_axis',(1.22464679915E-16,1.,7.49879891332945E-33));
#47083=DIRECTION('center_axis',(-1.,1.22464679915E-16,5.03301104497E-15));
#47084=DIRECTION('ref_axis',(-1.22464679915E-16,-1.,6.16366086630911E-31));
#47085=DIRECTION('',(1.,0.,3.62521803959E-16));
#47086=DIRECTION('center_axis',(2.17357452795E-16,-2.66186108837E-32,-1.));
#47087=DIRECTION('ref_axis',(0.,-1.,2.66186108837E-32));
#47088=DIRECTION('',(-1.,0.,0.));
#47089=DIRECTION('center_axis',(1.,-1.22464679915E-16,6.12323399574E-17));
#47090=DIRECTION('ref_axis',(-1.22464679915E-16,-1.,-7.49879891332945E-33));
#47091=DIRECTION('center_axis',(-1.,1.22464679915E-16,-9.25185853854E-17));
#47092=DIRECTION('ref_axis',(-1.22464679915E-16,-1.,-1.13302589454116E-32));
#47093=DIRECTION('',(1.,0.,0.));
#47094=DIRECTION('center_axis',(1.1936008304232E-16,1.,1.92500633904415E-17));
#47095=DIRECTION('ref_axis',(-0.159219839565945,0.,0.987243152768655));
#47096=DIRECTION('center_axis',(1.22464679915E-16,1.,5.47382212627E-48));
#47097=DIRECTION('ref_axis',(1.,-1.22464679915E-16,5.63840144221543E-64));
#47098=DIRECTION('center_axis',(0.987243152771461,1.8496896112958E-11,0.159219839548546));
#47099=DIRECTION('ref_axis',(-0.159219839548546,1.48029736616686E-14,0.987243152771461));
#47100=DIRECTION('center_axis',(1.22464679915E-16,1.,5.47382212627E-48));
#47101=DIRECTION('ref_axis',(1.,-1.22464679915E-16,0.));
#47102=DIRECTION('center_axis',(7.52478899174175E-8,0.999999999999997,1.38031989516745E-8));
#47103=DIRECTION('ref_axis',(-0.12861910970648,-4.01023408411311E-9,0.991694068056431));
#47104=DIRECTION('center_axis',(-1.22464679915E-16,-1.,0.));
#47105=DIRECTION('ref_axis',(1.,-1.22464679915E-16,0.));
#47106=DIRECTION('',(-2.19188076492E-16,0.,1.));
#47107=DIRECTION('center_axis',(-1.22464679915E-16,-1.,0.));
#47108=DIRECTION('ref_axis',(1.,-1.22464679915E-16,0.));
#47109=DIRECTION('center_axis',(-1.0413655165592E-9,-1.,-1.26007888238395E-10));
#47110=DIRECTION('ref_axis',(-0.167003259896707,4.96731596649238E-11,0.985956343447251));
#47111=DIRECTION('',(-2.17371312249E-16,0.,1.));
#47112=DIRECTION('center_axis',(0.258465262671631,0.964605492283562,0.0522680805891321));
#47113=DIRECTION('ref_axis',(0.945466832487627,-0.263697258719896,0.191196821127928));
#47114=DIRECTION('center_axis',(-1.22464679915E-16,-1.,-6.16297582204E-33));
#47115=DIRECTION('ref_axis',(1.,-1.22464679915E-16,-7.54746861370013E-49));
#47116=DIRECTION('center_axis',(2.17357452795E-16,-2.66186108837E-32,-1.));
#47117=DIRECTION('ref_axis',(1.,5.7857534586223E-48,2.17357452795E-16));
#47118=DIRECTION('center_axis',(-0.198212453337055,-3.31043063332241E-15,
0.980159080630336));
#47119=DIRECTION('ref_axis',(-0.945466832487629,0.263697258719893,-0.191196821127922));
#47120=DIRECTION('center_axis',(-2.17357452795E-16,2.66186108837E-32,1.));
#47121=DIRECTION('ref_axis',(1.,5.7857534586223E-48,2.17357452795E-16));
#47122=DIRECTION('',(-9.00454292637E-17,0.,1.));
#47123=DIRECTION('center_axis',(-2.17357452795E-16,2.66186108837E-32,1.));
#47124=DIRECTION('ref_axis',(1.,5.7857534586223E-48,2.17357452795E-16));
#47125=DIRECTION('center_axis',(1.22464679914984E-16,1.,8.09446956404351E-29));
#47126=DIRECTION('ref_axis',(-0.198212453337068,2.42740246530083E-17,0.980159080630333));
#47127=DIRECTION('',(0.,-1.,0.));
#47128=DIRECTION('center_axis',(1.,-1.22464679915E-16,6.12323399574E-17));
#47129=DIRECTION('ref_axis',(-1.22464679915E-16,-1.,-6.67366607695787E-50));
#47130=DIRECTION('',(2.17371312249E-16,0.,-1.));
#47131=DIRECTION('center_axis',(-2.17357452795E-16,2.66186108837E-32,1.));
#47132=DIRECTION('ref_axis',(-1.,-5.7857534586223E-48,-2.17357452795E-16));
#47133=DIRECTION('',(-1.29439338185998E-7,0.,0.999999999999992));
#47134=DIRECTION('center_axis',(-0.941574524866053,-0.33680470645719,6.18995477862716E-5));
#47135=DIRECTION('ref_axis',(0.257425227315659,-0.719541941796582,0.644974143929108));
#47136=DIRECTION('center_axis',(3.23815048849E-16,-3.96559063089E-32,-1.));
#47137=DIRECTION('ref_axis',(1.,1.28411792385678E-47,3.23815048849E-16));
#47138=DIRECTION('center_axis',(0.734238830876792,-8.99183234042744E-17,
-0.678891257295808));
#47139=DIRECTION('ref_axis',(-0.678891257295808,-1.51038693775819E-31,-0.734238830876792));
#47140=DIRECTION('',(-0.734238830876791,0.,0.678891257295807));
#47141=DIRECTION('center_axis',(-0.734238830876792,8.99183234042744E-17,
0.678891257295808));
#47142=DIRECTION('ref_axis',(0.678891257295807,3.46311205996404E-31,0.734238830876791));
#47143=DIRECTION('center_axis',(-0.734238830876792,8.99183234042744E-17,
0.678891257295808));
#47144=DIRECTION('ref_axis',(0.678891257295808,1.51038693775819E-31,0.734238830876792));
#47145=DIRECTION('center_axis',(1.,0.,0.));
#47146=DIRECTION('ref_axis',(0.,-1.,0.));
#47147=DIRECTION('center_axis',(-0.790681776842983,9.68305907154979E-17,
-0.612227349738987));
#47148=DIRECTION('ref_axis',(0.612227349738987,1.22226555802243E-31,-0.790681776842983));
#47149=DIRECTION('center_axis',(7.65621835198448E-17,1.,5.92823359275332E-17));
#47150=DIRECTION('ref_axis',(-0.612227349738987,0.,0.790681776842983));
#47151=DIRECTION('center_axis',(-1.22464679915E-16,-1.,-5.47382212627E-48));
#47152=DIRECTION('ref_axis',(1.,-1.22464679915E-16,-6.703498746053E-64));
#47153=DIRECTION('center_axis',(-0.991694064582439,1.21447496192053E-16,
-0.128619136492057));
#47154=DIRECTION('ref_axis',(0.128619136492057,-4.98879909760123E-32,-0.991694064582438));
#47155=DIRECTION('center_axis',(0.,0.,1.));
#47156=DIRECTION('ref_axis',(1.,0.,0.));
#47157=DIRECTION('center_axis',(2.17357452795E-16,-2.66186108837E-32,-1.));
#47158=DIRECTION('ref_axis',(1.,5.7857534586223E-48,2.17357452795E-16));
#47159=DIRECTION('center_axis',(-2.17357452795E-16,2.66186108837E-32,1.));
#47160=DIRECTION('ref_axis',(1.,5.7857534586223E-48,2.17357452795E-16));
#47161=DIRECTION('center_axis',(-1.17036010513E-14,1.43327775659E-30,-1.));
#47162=DIRECTION('ref_axis',(1.,1.98907245817996E-46,-1.17036010513E-14));
#47163=DIRECTION('center_axis',(0.,0.,1.));
#47164=DIRECTION('ref_axis',(1.,0.,0.));
#47165=DIRECTION('center_axis',(0.824331881335686,-1.00951539990962E-16,
0.566106835688784));
#47166=DIRECTION('ref_axis',(0.566106835688784,-1.17683260639136E-31,-0.824331881335686));
#47167=DIRECTION('center_axis',(1.,0.,0.));
#47168=DIRECTION('ref_axis',(0.,-1.,0.));
#47169=DIRECTION('center_axis',(0.99733341416283,-1.22138117333977E-16,
0.0729798670477863));
#47170=DIRECTION('ref_axis',(0.0729798670477863,2.52018738244318E-32,-0.99733341416283));
#47171=DIRECTION('center_axis',(8.32175728849317E-17,1.,5.71493568625004E-17));
#47172=DIRECTION('ref_axis',(-0.566106835688784,0.,0.824331881335686));
#47173=DIRECTION('center_axis',(1.22464679915E-16,1.,5.47382212627E-48));
#47174=DIRECTION('ref_axis',(1.,-1.22464679915E-16,6.49622071350503E-64));
#47175=DIRECTION('center_axis',(1.22464679915E-16,1.,5.47382212627E-48));
#47176=DIRECTION('ref_axis',(1.,-1.22464679915E-16,0.));
#47177=DIRECTION('center_axis',(0.,0.,1.));
#47178=DIRECTION('ref_axis',(1.,0.,0.));
#47179=DIRECTION('center_axis',(-1.,1.22464679915E-16,-6.12323399574E-17));
#47180=DIRECTION('ref_axis',(-6.12323399574E-17,0.,1.));
#47181=DIRECTION('',(1.5105075165E-16,1.,0.));
#47182=DIRECTION('',(-2.28870415168E-16,0.,1.));
#47183=DIRECTION('',(-7.55253758248E-17,-1.,0.));
#47184=DIRECTION('center_axis',(-1.22464679914868E-16,-1.,-1.27704300324719E-28));
#47185=DIRECTION('ref_axis',(0.718198537785833,-8.79539540451795E-17,-0.695838242928838));
#47186=DIRECTION('',(1.5105075165E-16,1.,0.));
#47187=DIRECTION('',(1.5105075165E-16,1.,0.));
#47188=DIRECTION('center_axis',(-1.22464679914988E-16,-1.,-5.97423468748921E-29));
#47189=DIRECTION('ref_axis',(0.191153986297933,-2.34096117463918E-17,-0.981560061087659));
#47190=DIRECTION('',(1.23358113847E-16,1.,0.));
#47191=DIRECTION('center_axis',(7.52094574043E-17,1.,3.8940254264E-17));
#47192=DIRECTION('ref_axis',(1.,-7.52094574043E-17,-2.92867539438092E-33));
#47193=DIRECTION('center_axis',(-1.,1.22464679915E-16,-6.12323399574E-17));
#47194=DIRECTION('ref_axis',(-6.12323399574E-17,0.,1.));
#47195=DIRECTION('',(-1.5105075165E-16,-1.,0.));
#47196=DIRECTION('',(-1.74378361673E-16,0.,1.));
#47197=DIRECTION('center_axis',(-1.22464679915E-16,-1.,3.08148791102006E-33));
#47198=DIRECTION('ref_axis',(1.,-1.22464679915E-16,-5.78241158658936E-15));
#47199=DIRECTION('',(-1.16865581539E-16,-1.,0.));
#47200=DIRECTION('center_axis',(-1.61832416815E-16,-1.,-4.68996881439E-17));
#47201=DIRECTION('ref_axis',(1.,-1.61832416815E-16,-7.58988988019714E-33));
#47202=DIRECTION('center_axis',(-1.22464679915001E-16,-1.,1.11184889946404E-29));
#47203=DIRECTION('ref_axis',(-0.11782622263506,1.44295506406073E-17,0.993034229651503));
#47204=DIRECTION('',(0.,1.,0.));
#47205=DIRECTION('center_axis',(-1.22464679915E-16,-1.,-3.08148791102E-33));
#47206=DIRECTION('ref_axis',(1.,-1.22464679915E-16,-3.77373430685006E-49));
#47207=DIRECTION('center_axis',(-1.224646799149E-16,-1.,1.07603845915075E-28));
#47208=DIRECTION('ref_axis',(-0.678891257295807,8.31402005216763E-17,-0.734238830876792));
#47209=DIRECTION('',(1.23358113847E-16,1.,0.));
#47210=DIRECTION('center_axis',(1.224646799149E-16,1.,-1.07603845915075E-28));
#47211=DIRECTION('ref_axis',(-0.678891257295809,8.31402005216765E-17,-0.73423883087679));
#47212=DIRECTION('',(2.46716227694E-16,1.,0.));
#47213=DIRECTION('center_axis',(0.678891257295808,-8.31402005216763E-17,
0.734238830876792));
#47214=DIRECTION('ref_axis',(-1.22464679914784E-16,-1.,1.83887638005312E-34));
#47215=DIRECTION('center_axis',(-1.22464679915001E-16,-1.,1.11184889946404E-29));
#47216=DIRECTION('ref_axis',(-0.11782622263506,1.44295506406073E-17,0.993034229651503));
#47217=DIRECTION('',(0.,1.,0.));
#47218=DIRECTION('',(0.,1.,0.));
#47219=DIRECTION('center_axis',(1.22464679914738E-16,1.,-8.7827755269459E-30));
#47220=DIRECTION('ref_axis',(0.999438196720723,-1.22395878855966E-16,0.0335155327516906));
#47221=DIRECTION('',(0.,1.,0.));
#47222=DIRECTION('center_axis',(-1.22464679914868E-16,-1.,-1.27704300324719E-28));
#47223=DIRECTION('ref_axis',(0.718198537785833,-8.79539540451795E-17,-0.695838242928838));
#47224=DIRECTION('',(0.,1.,0.));
#47225=DIRECTION('center_axis',(-1.22464679915E-16,-1.,-1.94567767731298E-44));
#47226=DIRECTION('ref_axis',(-2.38276793969895E-60,-1.94567767731298E-44,
1.));
#47227=DIRECTION('',(0.,1.,0.));
#47228=DIRECTION('center_axis',(1.22464679915E-16,1.,6.39482694638668E-33));
#47229=DIRECTION('ref_axis',(2.89120579329468E-15,-3.60465418990613E-31,
1.));
#47230=DIRECTION('',(0.,1.,0.));
#47231=DIRECTION('center_axis',(-2.17357452795E-16,2.66186108837E-32,1.));
#47232=DIRECTION('ref_axis',(1.,2.56447231488414E-65,2.17357452795E-16));
#47233=DIRECTION('center_axis',(-1.22464679914868E-16,-1.,-1.27704300324719E-28));
#47234=DIRECTION('ref_axis',(-0.714687205042302,8.7523939804668E-17,0.699444207173683));
#47235=DIRECTION('',(0.,-1.,0.));
#47236=DIRECTION('',(0.,1.,0.));
#47237=DIRECTION('center_axis',(-1.22464679914919E-16,-1.,-1.07732241244701E-28));
#47238=DIRECTION('ref_axis',(0.602966636474876,-7.38421161351848E-17,-0.797766403966835));
#47239=DIRECTION('',(-2.46716227694E-16,-1.,0.));
#47240=DIRECTION('center_axis',(0.678891257295808,-8.31402005216763E-17,
0.734238830876792));
#47241=DIRECTION('ref_axis',(-1.22464679914784E-16,-1.,1.83887638005312E-34));
#47242=DIRECTION('',(0.,-1.,0.));
#47243=DIRECTION('center_axis',(1.22464679914841E-16,1.,1.13501471389221E-28));
#47244=DIRECTION('ref_axis',(-0.813441648140047,9.96178710688057E-17,0.581646529321034));
#47245=DIRECTION('',(0.,-1.,0.));
#47246=DIRECTION('center_axis',(-1.16236097357E-16,-1.,-6.09147290561E-17));
#47247=DIRECTION('ref_axis',(1.,-1.16236097357E-16,-7.08049037704012E-33));
#47248=DIRECTION('center_axis',(-1.22464679915001E-16,-1.,1.11184889946404E-29));
#47249=DIRECTION('ref_axis',(-0.11782622263506,1.44295506406073E-17,0.993034229651503));
#47250=DIRECTION('',(0.,-1.,0.));
#47251=DIRECTION('center_axis',(-1.22464679915E-16,-1.,-3.08148791102E-33));
#47252=DIRECTION('ref_axis',(1.,-1.22464679915E-16,-3.77373430685006E-49));
#47253=DIRECTION('center_axis',(-1.22464679915E-16,-1.,-1.94567767731298E-44));
#47254=DIRECTION('ref_axis',(2.38276793969895E-60,1.94567767731298E-44,
-1.));
#47255=DIRECTION('center_axis',(9.4593208002E-17,1.,5.4521376634E-17));
#47256=DIRECTION('ref_axis',(1.,-9.4593208002E-17,-5.15735192049534E-33));
#47257=DIRECTION('',(0.,1.,0.));
#47258=DIRECTION('center_axis',(-1.22464679914423E-16,-1.,-8.33007499390688E-29));
#47259=DIRECTION('ref_axis',(-0.98972556641388,1.21206424693985E-16,0.142980079684982));
#47260=DIRECTION('',(0.,-1.,0.));
#47261=DIRECTION('center_axis',(-2.61334043E-16,-1.,-1.20249303974E-16));
#47262=DIRECTION('ref_axis',(1.,-2.61334043E-16,-3.14252367754614E-32));
#47263=DIRECTION('center_axis',(-2.17357452795E-16,2.66186108837E-32,1.));
#47264=DIRECTION('ref_axis',(1.,2.56447231488414E-65,2.17357452795E-16));
#47265=DIRECTION('',(1.,0.,0.));
#47266=DIRECTION('center_axis',(0.,1.,0.));
#47267=DIRECTION('ref_axis',(-0.10172047258397,0.,0.994813020349701));
#47268=DIRECTION('center_axis',(0.581646529321033,-7.12311560368041E-17,
0.813441648140047));
#47269=DIRECTION('ref_axis',(0.813441648140047,-2.80119922649672E-32,-0.581646529321033));
#47270=DIRECTION('center_axis',(1.69872863391202E-17,1.,4.23293596334453E-17));
#47271=DIRECTION('ref_axis',(-0.927892968287493,0.,0.372846670097274));
#47272=DIRECTION('center_axis',(-1.22464679915E-16,-1.,-5.47382212627E-48));
#47273=DIRECTION('ref_axis',(1.,-1.22464679915E-16,-6.703498746053E-64));
#47274=DIRECTION('center_axis',(0.,0.,1.));
#47275=DIRECTION('ref_axis',(1.,0.,0.));
#47276=DIRECTION('center_axis',(1.,-1.22464679915E-16,6.12323399574E-17));
#47277=DIRECTION('ref_axis',(-1.22464679915E-16,-1.,-7.49879891332945E-33));
#47278=DIRECTION('center_axis',(0.,0.,1.));
#47279=DIRECTION('ref_axis',(1.,0.,0.));
#47280=DIRECTION('center_axis',(-1.,1.22464679915E-16,-6.12323399574E-17));
#47281=DIRECTION('ref_axis',(-1.22464679915E-16,-1.,-7.49879891332945E-33));
#47282=DIRECTION('center_axis',(-1.,1.22464679915E-16,-6.12323399574E-17));
#47283=DIRECTION('ref_axis',(1.22464679915E-16,1.,7.49879891332945E-33));
#47284=DIRECTION('',(1.,0.,2.89652532403E-16));
#47285=DIRECTION('center_axis',(1.22464679915E-16,1.,5.47382212627E-48));
#47286=DIRECTION('ref_axis',(1.,-1.22464679915E-16,0.));
#47287=DIRECTION('center_axis',(-1.22464679915E-16,-1.,-3.08148791102E-33));
#47288=DIRECTION('ref_axis',(1.,-1.22464679915E-16,-3.77373430685006E-49));
#47289=DIRECTION('',(-1.74378361673E-16,0.,1.));
#47290=DIRECTION('center_axis',(-0.62218556523187,0.249390626342792,-0.742084522079155));
#47291=DIRECTION('ref_axis',(0.160230040961959,0.968402971645766,0.191107348055953));
#47292=DIRECTION('center_axis',(0.,1.,0.));
#47293=DIRECTION('ref_axis',(0.751205410155072,0.,0.660068505349066));
#47294=DIRECTION('center_axis',(-0.991694064582439,1.21447496192053E-16,
0.128619136492057));
#47295=DIRECTION('ref_axis',(0.128619136492057,-4.98879909760123E-32,0.991694064582438));
#47296=DIRECTION('center_axis',(-2.17357452795E-16,2.66186108837E-32,1.));
#47297=DIRECTION('ref_axis',(1.,5.7857534586223E-48,2.17357452795E-16));
#47298=DIRECTION('center_axis',(1.22464679915E-16,1.,5.47382212627E-48));
#47299=DIRECTION('ref_axis',(1.,-1.22464679915E-16,-6.703498746053E-64));
#47300=DIRECTION('center_axis',(1.22464679915E-16,1.,5.47382212627E-48));
#47301=DIRECTION('ref_axis',(1.,-1.22464679915E-16,0.));
#47302=DIRECTION('center_axis',(1.22464679915E-16,1.,5.47382212627E-48));
#47303=DIRECTION('ref_axis',(1.,-1.22464679915E-16,0.));
#47304=DIRECTION('center_axis',(-1.22464679915E-16,-1.,-7.60253073092891E-48));
#47305=DIRECTION('ref_axis',(1.,-1.22464679915E-16,-9.3104149250716E-64));
#47306=DIRECTION('',(1.16865581539E-16,1.,0.));
#47307=DIRECTION('center_axis',(1.22464679915E-16,1.,1.94578320706031E-44));
#47308=DIRECTION('ref_axis',(-2.38289717636624E-60,-1.94578320706031E-44,
1.));
#47309=DIRECTION('center_axis',(-1.22464679915E-16,-1.,6.16297582204E-33));
#47310=DIRECTION('ref_axis',(1.,-1.22464679915E-16,7.54746861370013E-49));
#47311=DIRECTION('center_axis',(0.,0.,1.));
#47312=DIRECTION('ref_axis',(1.,0.,0.));
#47313=DIRECTION('center_axis',(-2.17357452795E-16,2.66186108837E-32,1.));
#47314=DIRECTION('ref_axis',(1.,5.7857534586223E-48,2.17357452795E-16));
#47315=DIRECTION('center_axis',(1.69872863391202E-17,1.,4.23293596334453E-17));
#47316=DIRECTION('ref_axis',(0.928056183869048,0.,-0.37244022283102));
#47317=DIRECTION('center_axis',(1.22464679914985E-16,1.,-5.43497430306078E-29));
#47318=DIRECTION('ref_axis',(-0.269603455472075,3.30169008783092E-17,-0.962971430935268));
#47319=DIRECTION('center_axis',(0.,-1.,0.));
#47320=DIRECTION('ref_axis',(-0.269603444240349,0.,-0.962971434079818));
#47321=DIRECTION('center_axis',(2.17357452795E-16,-2.66186108836794E-32,
-1.));
#47322=DIRECTION('ref_axis',(5.78575345861782E-48,1.,-2.66186108836794E-32));
#47323=DIRECTION('center_axis',(-2.17357452795E-16,2.66186108837E-32,1.));
#47324=DIRECTION('ref_axis',(1.,5.7857534586223E-48,2.17357452795E-16));
#47325=DIRECTION('',(0.,0.,1.));
#47326=DIRECTION('center_axis',(0.,1.,0.));
#47327=DIRECTION('ref_axis',(0.642923934113106,0.,0.765930032669124));
#47328=DIRECTION('center_axis',(9.19369336238712E-17,1.,5.29776121060009E-17));
#47329=DIRECTION('ref_axis',(-0.499277443708891,0.,0.86644217014381));
#47330=DIRECTION('center_axis',(-4.29367103357466E-45,-1.,7.25136572506882E-31));
#47331=DIRECTION('ref_axis',(-1.,0.,-5.9211894646675E-15));
#47332=DIRECTION('center_axis',(1.,0.,0.));
#47333=DIRECTION('ref_axis',(0.,-1.,0.));
#47334=DIRECTION('center_axis',(-0.687199008140201,8.41576065696246E-17,
-0.726469216974212));
#47335=DIRECTION('ref_axis',(0.726469216974212,1.50838013754883E-32,-0.687199008140201));
#47336=DIRECTION('center_axis',(-0.827537346623811,1.01344096271977E-16,
0.561410669601872));
#47337=DIRECTION('ref_axis',(0.561410669601872,-5.47362952277333E-32,0.827537346623811));
#47338=DIRECTION('center_axis',(1.22464679915E-16,1.,-1.23259516441E-32));
#47339=DIRECTION('ref_axis',(1.,-1.22464679915E-16,1.50949372274247E-48));
#47340=DIRECTION('center_axis',(1.22464679914912E-16,1.,8.35596805204809E-29));
#47341=DIRECTION('ref_axis',(-0.726469216974212,8.89668201247259E-17,0.687199008140201));
#47342=DIRECTION('',(0.,1.,0.));
#47343=DIRECTION('',(0.,1.,0.));
#47344=DIRECTION('center_axis',(-1.22464679914998E-16,-1.,-1.73663083545565E-29));
#47345=DIRECTION('ref_axis',(-0.095298509688002,1.16707014853003E-17,0.99544874004202));
#47346=DIRECTION('center_axis',(1.22464679915E-16,1.,0.));
#47347=DIRECTION('ref_axis',(1.,-1.22464679915E-16,0.));
#47348=DIRECTION('center_axis',(1.68490994230906E-17,1.,4.21844451941189E-17));
#47349=DIRECTION('ref_axis',(0.928663912412966,0.,-0.370922279974987));
#47350=DIRECTION('center_axis',(1.22464679915E-16,1.,5.47382212627E-48));
#47351=DIRECTION('ref_axis',(1.,-1.22464679915E-16,-6.703498746053E-64));
#47352=DIRECTION('center_axis',(-2.17357452795E-16,2.66186108837E-32,1.));
#47353=DIRECTION('ref_axis',(1.,5.7857534586223E-48,2.17357452795E-16));
#47354=DIRECTION('',(0.,0.,-1.));
#47355=DIRECTION('center_axis',(2.17357452795E-16,-5.59737441582E-15,-1.));
#47356=DIRECTION('ref_axis',(1.,1.21663104536254E-30,2.17357452795E-16));
#47357=DIRECTION('center_axis',(3.17795218513E-15,-3.89186897136E-31,-1.));
#47358=DIRECTION('ref_axis',(1.,1.11597938503332E-46,3.17795218513E-15));
#47359=DIRECTION('center_axis',(2.68354439599323E-46,1.,1.81284143127026E-31));
#47360=DIRECTION('ref_axis',(-1.,0.,1.97372982155583E-15));
#47361=DIRECTION('center_axis',(-1.22464679915E-16,-1.,-5.47382212627E-48));
#47362=DIRECTION('ref_axis',(1.,-1.22464679915E-16,-6.703498746053E-64));
#47363=DIRECTION('center_axis',(-0.904759192693671,1.1080104493296E-16,
0.425923471102845));
#47364=DIRECTION('ref_axis',(0.425923471102845,3.65487816993661E-32,0.904759192693671));
#47365=DIRECTION('center_axis',(1.0293130162049E-16,1.,-4.48396705262131E-17));
#47366=DIRECTION('ref_axis',(-0.399377187820903,0.,-0.916786704663777));
#47367=DIRECTION('center_axis',(1.22464679915E-16,1.,5.47382212627E-48));
#47368=DIRECTION('ref_axis',(1.,-1.22464679915E-16,-6.703498746053E-64));
#47369=DIRECTION('center_axis',(-0.916786704663777,1.12273990336973E-16,
0.399377187820903));
#47370=DIRECTION('ref_axis',(0.399377187820903,3.93858763528754E-32,0.916786704663777));
#47371=DIRECTION('center_axis',(1.0293130162049E-16,1.,-4.48396705262131E-17));
#47372=DIRECTION('ref_axis',(0.399377187820903,0.,0.916786704663777));
#47373=DIRECTION('center_axis',(-1.22464679915E-16,-1.,-5.47382212627E-48));
#47374=DIRECTION('ref_axis',(1.,-1.22464679915E-16,-6.703498746053E-64));
#47375=DIRECTION('center_axis',(-2.17357452795E-16,2.66186108837E-32,1.));
#47376=DIRECTION('ref_axis',(1.,5.7857534586223E-48,2.17357452795E-16));
#47377=DIRECTION('center_axis',(-2.17357452795E-16,2.66186108835898E-32,
1.));
#47378=DIRECTION('ref_axis',(5.78575345859834E-48,1.,-2.66186108835898E-32));
#47379=DIRECTION('',(0.,0.,1.));
#47380=DIRECTION('center_axis',(-3.47250861231E-16,-5.79129605623E-15,1.));
#47381=DIRECTION('ref_axis',(1.,-2.01103254316956E-30,3.47250861231E-16));
#47382=DIRECTION('center_axis',(1.22464679915E-16,1.,5.47382212627E-48));
#47383=DIRECTION('ref_axis',(1.,-1.22464679915E-16,0.));
#47384=DIRECTION('center_axis',(1.22464679915E-16,1.,0.));
#47385=DIRECTION('ref_axis',(1.,-1.22464679915E-16,0.));
#47386=DIRECTION('',(-0.687199008140201,0.,-0.726469216974212));
#47387=DIRECTION('center_axis',(1.22464679915E-16,1.,0.));
#47388=DIRECTION('ref_axis',(1.,-1.22464679915E-16,0.));
#47389=DIRECTION('center_axis',(0.,0.957608642877659,-0.288072364321897));
#47390=DIRECTION('ref_axis',(0.,-0.288072364321899,-0.957608642877659));
#47391=DIRECTION('center_axis',(-0.890715300400791,1.09081164158974E-16,
0.454561605980893));
#47392=DIRECTION('ref_axis',(0.454561605980893,-9.65132779741589E-32,0.890715300400791));
#47393=DIRECTION('center_axis',(-1.22464679915E-16,-1.,-5.47382212627E-48));
#47394=DIRECTION('ref_axis',(1.,-1.22464679915E-16,-6.703498746053E-64));
#47395=DIRECTION('center_axis',(-1.,1.2919345348203E-16,-3.88645861503935E-17));
#47396=DIRECTION('ref_axis',(0.,0.288072364321903,0.957608642877657));
#47397=DIRECTION('center_axis',(1.178693242477E-16,1.,-2.32734068666895E-17));
#47398=DIRECTION('ref_axis',(-0.193710935823942,0.,-0.981058649287703));
#47399=DIRECTION('center_axis',(1.22464679915E-16,1.,5.47382212627E-48));
#47400=DIRECTION('ref_axis',(1.,-1.22464679915E-16,6.22660996643423E-64));
#47401=DIRECTION('center_axis',(-0.684308456885095,0.684308456885093,0.25188066950658));
#47402=DIRECTION('ref_axis',(-0.178106529457909,0.178106529457906,-0.967758300573505));
#47403=DIRECTION('center_axis',(0.938446715307966,-1.14926576606996E-16,
-0.345424032932987));
#47404=DIRECTION('ref_axis',(0.345424032932987,5.96953449650393E-32,0.938446715307966));
#47405=DIRECTION('center_axis',(1.22464679915E-16,1.,3.08148791102E-33));
#47406=DIRECTION('ref_axis',(1.,-1.22464679915E-16,-3.77373430685006E-49));
#47407=DIRECTION('center_axis',(1.178693242477E-16,1.,-2.32734068666895E-17));
#47408=DIRECTION('ref_axis',(-0.193710935823942,0.,-0.981058649287703));
#47409=DIRECTION('center_axis',(1.22464679915E-16,1.,5.47382212627E-48));
#47410=DIRECTION('ref_axis',(1.,-1.22464679915E-16,6.22660996643423E-64));
#47411=DIRECTION('center_axis',(1.22464679915E-16,1.,7.60253073092891E-48));
#47412=DIRECTION('ref_axis',(1.,-1.22464679915E-16,-9.3104149250716E-64));
#47413=DIRECTION('',(-1.38777878078E-16,-1.,0.));
#47414=DIRECTION('center_axis',(-1.22464679914586E-16,-1.,-1.3947821589454E-28));
#47415=DIRECTION('ref_axis',(-0.947590338356885,1.16046347476986E-16,0.319487950715961));
#47416=DIRECTION('',(0.,-1.,0.));
#47417=DIRECTION('center_axis',(-1.22464679914973E-16,-1.,1.28029659727041E-28));
#47418=DIRECTION('ref_axis',(-0.207931718074914,2.54642912980895E-17,-0.978143343594595));
#47419=DIRECTION('',(1.42793958151E-16,1.,0.));
#47420=DIRECTION('center_axis',(-1.22464679914586E-16,-1.,-1.3947821589454E-28));
#47421=DIRECTION('ref_axis',(-0.947590338356885,1.16046347476986E-16,0.319487950715961));
#47422=DIRECTION('center_axis',(1.22464679914899E-16,1.,-1.21650294976139E-28));
#47423=DIRECTION('ref_axis',(-0.638858327474962,7.82375805850953E-17,-0.769324403236954));
#47424=DIRECTION('center_axis',(-6.13428128073E-17,-1.,3.67652253532E-18));
#47425=DIRECTION('ref_axis',(1.,-6.13428128073E-17,2.25528233665955E-34));
#47426=DIRECTION('',(0.,-1.,0.));
#47427=DIRECTION('center_axis',(0.,1.,0.));
#47428=DIRECTION('ref_axis',(-0.998195841446114,0.,-0.0600421695118078));
#47429=DIRECTION('center_axis',(0.687199008140201,-8.41576065696246E-17,
0.726469216974212));
#47430=DIRECTION('ref_axis',(0.726469216974212,1.50838013754883E-32,-0.687199008140201));
#47431=DIRECTION('center_axis',(0.687199008140201,-8.41576065697951E-17,
0.726469216974212));
#47432=DIRECTION('ref_axis',(5.78330237622164E-17,1.,6.11379105471828E-17));
#47433=DIRECTION('',(-0.687199008140201,0.,-0.726469216974212));
#47434=DIRECTION('center_axis',(-0.726469216974212,8.89668201247259E-17,
0.687199008140201));
#47435=DIRECTION('ref_axis',(1.22464679914833E-16,1.,-2.7960247294612E-34));
#47436=DIRECTION('',(-0.687199008140201,0.,-0.726469216974212));
#47437=DIRECTION('center_axis',(0.687199008140201,-8.41576065697951E-17,
0.726469216974212));
#47438=DIRECTION('ref_axis',(-5.78330237622164E-17,-1.,-6.11379105471828E-17));
#47439=DIRECTION('',(-0.687199008140201,0.,-0.726469216974212));
#47440=DIRECTION('center_axis',(0.678892491799354,-1.68130604497259E-6,
0.734237689427366));
#47441=DIRECTION('ref_axis',(0.519185258239941,0.70710677855387,-0.480048613527311));
#47442=DIRECTION('center_axis',(0.734238830876792,-8.99183234042744E-17,
-0.678891257295808));
#47443=DIRECTION('ref_axis',(0.678891257295808,1.51038693775819E-31,0.734238830876792));
#47444=DIRECTION('',(0.734238830876791,0.,-0.678891257295807));
#47445=DIRECTION('center_axis',(0.734238830876792,-8.99183234042744E-17,
-0.678891257295808));
#47446=DIRECTION('ref_axis',(0.678891257295808,1.51038693775819E-31,0.734238830876792));
#47447=DIRECTION('center_axis',(-6.60215246509141E-17,-1.,6.10447636300053E-17));
#47448=DIRECTION('ref_axis',(-0.678891257295808,0.,-0.734238830876791));
#47449=DIRECTION('center_axis',(-1.22464679915E-16,-1.,-5.47382212627E-48));
#47450=DIRECTION('ref_axis',(1.,-1.22464679915E-16,-6.703498746053E-64));
#47451=DIRECTION('center_axis',(0.790681776842983,-9.68305907154979E-17,
0.612227349738987));
#47452=DIRECTION('ref_axis',(0.612227349738987,1.22226555802243E-31,-0.790681776842983));
#47453=DIRECTION('center_axis',(-1.20438761132693E-16,-1.,-1.56204720894266E-17));
#47454=DIRECTION('ref_axis',(-0.128619136492057,0.,0.991694064582438));
#47455=DIRECTION('center_axis',(1.22464679915E-16,1.,5.47382212627E-48));
#47456=DIRECTION('ref_axis',(1.,-1.22464679915E-16,-6.703498746053E-64));
#47457=DIRECTION('center_axis',(0.991694064582439,-1.21447496192053E-16,
0.128619136492057));
#47458=DIRECTION('ref_axis',(0.128619136492057,-7.10548517584315E-33,-0.991694064582438));
#47459=DIRECTION('center_axis',(-1.20438761132693E-16,-1.,-1.56204720894266E-17));
#47460=DIRECTION('ref_axis',(0.128619136492057,0.,-0.991694064582438));
#47461=DIRECTION('center_axis',(-1.22464679915E-16,-1.,-5.47382212627E-48));
#47462=DIRECTION('ref_axis',(1.,-1.22464679915E-16,-6.703498746053E-64));
#47463=DIRECTION('center_axis',(-2.17357452795E-16,2.66186108837E-32,1.));
#47464=DIRECTION('ref_axis',(1.,5.7857534586223E-48,2.17357452795E-16));
#47465=DIRECTION('center_axis',(-2.17357452795E-16,2.66186108837E-32,1.));
#47466=DIRECTION('ref_axis',(-1.,-5.7857534586223E-48,-2.17357452795E-16));
#47467=DIRECTION('',(-5.89048887673E-17,0.,1.));
#47468=DIRECTION('center_axis',(5.70383201187E-15,-6.98517961621E-31,1.));
#47469=DIRECTION('ref_axis',(1.,-5.48892443580096E-47,-5.70383201187E-15));
#47470=DIRECTION('center_axis',(-0.734238830876792,8.99183234042744E-17,
0.678891257295808));
#47471=DIRECTION('ref_axis',(0.678891257295807,3.46311205996404E-31,0.734238830876791));
#47472=DIRECTION('center_axis',(-8.32175728849317E-17,-1.,-5.71493568625004E-17));
#47473=DIRECTION('ref_axis',(-0.566106835688784,0.,0.824331881335687));
#47474=DIRECTION('center_axis',(-0.824331881335686,1.00951539990962E-16,
-0.566106835688784));
#47475=DIRECTION('ref_axis',(0.566106835688784,-1.17683260639136E-31,-0.824331881335686));
#47476=DIRECTION('center_axis',(-1.22464679915E-16,-1.,-5.47382212627E-48));
#47477=DIRECTION('ref_axis',(1.,-1.22464679915E-16,-6.703498746053E-64));
#47478=DIRECTION('center_axis',(-1.07341775839004E-43,-1.,3.62568286252829E-30));
#47479=DIRECTION('ref_axis',(1.,0.,2.96059473233375E-14));
#47480=DIRECTION('center_axis',(-1.22464679915E-16,-1.,-5.47382212627E-48));
#47481=DIRECTION('ref_axis',(1.,-1.22464679915E-16,-6.703498746053E-64));
#47482=DIRECTION('center_axis',(-0.99733341416283,1.22138117333977E-16,
-0.0729798670477863));
#47483=DIRECTION('ref_axis',(0.0729798670477863,2.52018738244318E-32,-0.99733341416283));
#47484=DIRECTION('center_axis',(-1.21812425560124E-16,-1.,-8.91362356450131E-18));
#47485=DIRECTION('ref_axis',(-0.0729798670477876,0.,0.99733341416283));
#47486=DIRECTION('center_axis',(-1.22464679915E-16,-1.,-5.47382212627E-48));
#47487=DIRECTION('ref_axis',(1.,-1.22464679915E-16,5.9677926224237E-64));
#47488=DIRECTION('center_axis',(-7.91623497736024E-17,-1.,-5.85483919904324E-17));
#47489=DIRECTION('ref_axis',(0.594634643326775,0.,-0.803996045360696));
#47490=DIRECTION('center_axis',(-1.22464679915E-16,-1.,-5.47382212627E-48));
#47491=DIRECTION('ref_axis',(1.,-1.22464679915E-16,-6.703498746053E-64));
#47492=DIRECTION('center_axis',(0.803996045360697,-9.84611183477626E-17,
0.594634643326775));
#47493=DIRECTION('ref_axis',(0.594634643326775,4.97302608069436E-32,-0.803996045360697));
#47494=DIRECTION('center_axis',(-7.91623497736024E-17,-1.,-5.85483919904324E-17));
#47495=DIRECTION('ref_axis',(-0.594634643326775,0.,0.803996045360696));
#47496=DIRECTION('center_axis',(1.22464679915E-16,1.,5.47382212627E-48));
#47497=DIRECTION('ref_axis',(1.,-1.22464679915E-16,-6.703498746053E-64));
#47498=DIRECTION('center_axis',(0.766648861207372,2.15189723830724E-8,0.642066603717589));
#47499=DIRECTION('ref_axis',(-0.454009649462123,-0.707106763017885,0.542102632247482));
#47500=DIRECTION('center_axis',(-0.204326481649494,0.26766241396516,-0.941598386281052));
#47501=DIRECTION('ref_axis',(-0.591685618293079,0.732523927752735,0.336625644262053));
#47502=DIRECTION('center_axis',(-0.198845429179661,-2.66706420366427E-7,
-0.980030864460036));
#47503=DIRECTION('ref_axis',(0.692986505330404,-0.707106783433054,-0.140604766110239));
#47504=DIRECTION('center_axis',(-0.988161317760145,-0.0726194459501342,
-0.135142984103609));
#47505=DIRECTION('ref_axis',(0.140217557783907,-0.0700183990770855,-0.987641868431973));
#47506=DIRECTION('center_axis',(0.734238830876792,-8.991832340449E-17,-0.678891257295808));
#47507=DIRECTION('ref_axis',(6.6021524650914E-17,1.,-6.10447636300053E-17));
#47508=DIRECTION('',(-0.734238830876791,0.,0.678891257295807));
#47509=DIRECTION('center_axis',(-0.734238784116523,6.88429683969821E-8,
0.678891307868266));
#47510=DIRECTION('ref_axis',(0.480048418882853,-0.707107065263036,0.519185047726887));
#47511=DIRECTION('center_axis',(0.911344426846927,1.14523576333168E-7,-0.411644671598009));
#47512=DIRECTION('ref_axis',(0.291076971310159,-0.707106395458268,0.644418142416025));
#47513=DIRECTION('center_axis',(-2.17357452795E-16,2.66186108837E-32,1.));
#47514=DIRECTION('ref_axis',(1.,5.7857534586223E-48,2.17357452795E-16));
#47515=DIRECTION('',(0.,0.,-1.));
#47516=DIRECTION('center_axis',(-0.815922427322792,1.0845679086032E-6,-0.578161389743822));
#47517=DIRECTION('ref_axis',(0.408841377131885,-0.707071904207434,-0.576973180161242));
#47518=DIRECTION('center_axis',(0.734238830876792,-8.99183234042744E-17,
-0.678891257295808));
#47519=DIRECTION('ref_axis',(-0.678891257295808,-1.51038693775819E-31,-0.734238830876792));
#47520=DIRECTION('',(-0.734238830876791,0.,0.678891257295807));
#47521=DIRECTION('center_axis',(-2.19931778314037E-16,-1.,1.97757654230408E-17));
#47522=DIRECTION('ref_axis',(-0.980030917502135,2.19472257881379E-16,0.198845167756028));
#47523=DIRECTION('center_axis',(-1.22464679915E-16,-1.,-5.47382212627E-48));
#47524=DIRECTION('ref_axis',(1.,-1.22464679915E-16,5.24998673990483E-64));
#47525=DIRECTION('center_axis',(-1.00613328137095E-16,-1.,-4.6888561789305E-17));
#47526=DIRECTION('ref_axis',(4.11834732982896E-10,0.,1.));
#47527=DIRECTION('center_axis',(1.22464679915E-16,1.,5.47382212627E-48));
#47528=DIRECTION('ref_axis',(1.,-1.22464679915E-16,5.63840144221543E-64));
#47529=DIRECTION('center_axis',(-0.923879532511277,1.13142611229013E-16,
-0.382683432365114));
#47530=DIRECTION('ref_axis',(-1.22464679915E-16,-1.,-1.95419172973166E-31));
#47531=DIRECTION('center_axis',(0.923879532511277,-1.13142611229034E-16,
0.382683432365115));
#47532=DIRECTION('ref_axis',(0.382683432365115,2.61659610287296E-32,-0.923879532511276));
#47533=DIRECTION('',(0.923879532511277,0.,0.382683432365114));
#47534=DIRECTION('center_axis',(0.923879532511277,-1.13142611229034E-16,
0.382683432365115));
#47535=DIRECTION('ref_axis',(0.382683432365115,-2.77240367868488E-33,-0.923879532511276));
#47536=DIRECTION('center_axis',(0.923879532511277,-1.13142611229013E-16,
-0.382683432365114));
#47537=DIRECTION('ref_axis',(-1.22464679915E-16,-1.,1.95419172973166E-31));
#47538=DIRECTION('',(-0.923879532511277,0.,0.382683432365114));
#47539=DIRECTION('center_axis',(-0.923879532511277,1.13142611229034E-16,
0.382683432365115));
#47540=DIRECTION('ref_axis',(0.382683432365115,2.61659610287296E-32,0.923879532511276));
#47541=DIRECTION('center_axis',(0.382683432365114,-4.68652040533673E-17,
-0.923879532511277));
#47542=DIRECTION('ref_axis',(-1.79345371456341E-17,-1.,4.32978028118705E-17));
#47543=DIRECTION('',(-0.382683432365114,0.,0.923879532511277));
#47544=DIRECTION('center_axis',(-0.382683432365114,4.68652040533673E-17,
-0.923879532511277));
#47545=DIRECTION('ref_axis',(-1.79345371456341E-17,-1.,-4.32978028118705E-17));
#47546=DIRECTION('center_axis',(0.382683432365114,-4.6865204053314E-17,
0.923879532511277));
#47547=DIRECTION('ref_axis',(0.923879532511277,-1.59663321827302E-32,-0.382683432365114));
#47548=DIRECTION('',(0.382683432365114,0.,0.923879532511277));
#47549=DIRECTION('center_axis',(-1.04530142769366E-16,-1.,-4.32978028118705E-17));
#47550=DIRECTION('ref_axis',(0.382683432365114,0.,-0.923879532511277));
#47551=DIRECTION('center_axis',(-1.22464679915E-16,-1.,-5.47382212627E-48));
#47552=DIRECTION('ref_axis',(1.,-1.22464679915E-16,-6.703498746053E-64));
#47553=DIRECTION('center_axis',(-1.04530142769366E-16,-1.,4.32978028118705E-17));
#47554=DIRECTION('ref_axis',(-0.382683432365115,0.,-0.923879532511276));
#47555=DIRECTION('center_axis',(0.923879532511277,-1.13142611229034E-16,
-0.382683432365115));
#47556=DIRECTION('ref_axis',(0.382683432365115,2.61659610287296E-32,0.923879532511276));
#47557=DIRECTION('center_axis',(-1.22464679915E-16,-1.,-5.47382212627E-48));
#47558=DIRECTION('ref_axis',(1.,-1.22464679915E-16,-6.703498746053E-64));
#47559=DIRECTION('center_axis',(0.923879532511277,-1.13142611229034E-16,
-0.382683432365114));
#47560=DIRECTION('ref_axis',(0.382683432365114,7.46986778962313E-32,0.923879532511277));
#47561=DIRECTION('center_axis',(0.923879532511277,-1.13142611229034E-16,
-0.382683432365115));
#47562=DIRECTION('ref_axis',(0.382683432365115,-2.77240367868488E-33,0.923879532511276));
#47563=DIRECTION('',(0.923879532511277,0.,-0.382683432365114));
#47564=DIRECTION('center_axis',(-1.04530142769366E-16,-1.,4.32978028118705E-17));
#47565=DIRECTION('ref_axis',(0.382683432365115,0.,0.923879532511276));
#47566=DIRECTION('center_axis',(-1.22464679915E-16,-1.,-5.47382212627E-48));
#47567=DIRECTION('ref_axis',(1.,-1.22464679915E-16,-6.703498746053E-64));
#47568=DIRECTION('center_axis',(-0.923879532511277,1.13142611229034E-16,
-0.382683432365115));
#47569=DIRECTION('ref_axis',(0.382683432365115,2.61659610287296E-32,-0.923879532511276));
#47570=DIRECTION('center_axis',(-0.923879532511277,1.13142611229034E-16,
-0.382683432365114));
#47571=DIRECTION('ref_axis',(0.382683432365114,7.46986778962313E-32,-0.923879532511277));
#47572=DIRECTION('',(-0.923879532511277,0.,-0.382683432365114));
#47573=DIRECTION('center_axis',(-0.382683432365114,4.6865204053314E-17,
-0.923879532511277));
#47574=DIRECTION('ref_axis',(0.923879532511277,-1.59663321827302E-32,-0.382683432365114));
#47575=DIRECTION('',(-0.382683432365114,0.,-0.923879532511277));
#47576=DIRECTION('center_axis',(0.382683432365114,-4.6865204053314E-17,
-0.923879532511277));
#47577=DIRECTION('ref_axis',(0.923879532511277,-1.59663321827302E-32,0.382683432365114));
#47578=DIRECTION('',(0.382683432365114,0.,-0.923879532511277));
#47579=DIRECTION('center_axis',(0.382683432365114,-4.6865204053314E-17,
-0.923879532511277));
#47580=DIRECTION('ref_axis',(0.923879532511277,-1.59663321827302E-32,0.382683432365114));
#47581=DIRECTION('center_axis',(-1.79345371456341E-17,-1.,4.32978028118705E-17));
#47582=DIRECTION('ref_axis',(-0.923879532511277,0.,-0.382683432365114));
#47583=DIRECTION('center_axis',(-1.22464679915E-16,-1.,-5.47382212627E-48));
#47584=DIRECTION('ref_axis',(1.,-1.22464679915E-16,-6.703498746053E-64));
#47585=DIRECTION('center_axis',(-1.22464679915E-16,-1.,-5.47382212627E-48));
#47586=DIRECTION('ref_axis',(-1.,1.22464679915E-16,0.));
#47587=DIRECTION('',(-0.734238830876791,0.,0.678891257295807));
#47588=DIRECTION('center_axis',(-1.22464679915E-16,-1.,0.));
#47589=DIRECTION('ref_axis',(1.,-1.22464679915E-16,0.));
#47590=DIRECTION('center_axis',(1.22464679915E-16,1.,1.23259516441E-32));
#47591=DIRECTION('ref_axis',(1.,-1.22464679915E-16,-1.50949372274247E-48));
#47592=DIRECTION('center_axis',(-1.22464679915E-16,-1.,0.));
#47593=DIRECTION('ref_axis',(1.,-1.22464679915E-16,0.));
#47594=DIRECTION('',(1.,0.,4.75520106567E-17));
#47595=DIRECTION('center_axis',(-1.22464679915E-16,-1.,1.54074395551E-33));
#47596=DIRECTION('ref_axis',(1.,-1.22464679915E-16,1.88686715342503E-49));
#47597=DIRECTION('center_axis',(-1.22464679915E-16,-1.,0.));
#47598=DIRECTION('ref_axis',(1.,-1.22464679915E-16,0.));
#47599=DIRECTION('center_axis',(-5.46401789901627E-17,-1.,-6.08764557973899E-17));
#47600=DIRECTION('ref_axis',(-0.744196935834912,0.,0.667960268798922));
#47601=DIRECTION('center_axis',(-1.22464679915E-16,-1.,0.));
#47602=DIRECTION('ref_axis',(1.,-1.22464679915E-16,0.));
#47603=DIRECTION('center_axis',(-1.24261220950731E-7,-0.999999999999986,
-1.11355973133144E-7));
#47604=DIRECTION('ref_axis',(0.721616554826204,-1.66759910844075E-7,0.692292963853261));
#47605=DIRECTION('center_axis',(-0.884316205578325,-0.0178356349302338,
-0.466547681033985));
#47606=DIRECTION('ref_axis',(0.0157873708942533,-0.999840932052135,0.00829876577361474));
#47607=DIRECTION('center_axis',(-1.14444500362894E-17,-1.,-3.5644992269101E-17));
#47608=DIRECTION('ref_axis',(-0.952128653909774,0.,0.305697606146927));
#47609=DIRECTION('center_axis',(0.110668766458005,-1.35530150608006E-17,
-0.993857345966041));
#47610=DIRECTION('ref_axis',(0.993857345966041,-5.87811925404552E-33,0.110668766458005));
#47611=DIRECTION('center_axis',(-1.22464679915E-16,-1.,-5.47382212627E-48));
#47612=DIRECTION('ref_axis',(1.,-1.22464679915E-16,6.22660996643423E-64));
#47613=DIRECTION('center_axis',(-1.49989545857296E-18,-1.,1.34697635782315E-17));
#47614=DIRECTION('ref_axis',(-0.993857345966041,0.,-0.110668766458005));
#47615=DIRECTION('center_axis',(1.,-1.22464679915E-16,6.12323399574E-17));
#47616=DIRECTION('ref_axis',(1.22464679915E-16,1.,7.49879891332945E-33));
#47617=DIRECTION('center_axis',(-1.22464679915E-16,-1.,3.08148791102E-33));
#47618=DIRECTION('ref_axis',(1.,-1.22464679915E-16,3.77373430685006E-49));
#47619=DIRECTION('center_axis',(1.,-1.22464679915E-16,6.12323399574E-17));
#47620=DIRECTION('ref_axis',(-6.12323399574E-17,7.49879891332945E-33,1.));
#47621=DIRECTION('center_axis',(1.,-1.22464679915E-16,6.12323399574E-17));
#47622=DIRECTION('ref_axis',(-1.22464679915E-16,-1.,-7.49879891332945E-33));
#47623=DIRECTION('',(1.,0.,2.65024142098E-16));
#47624=DIRECTION('center_axis',(-1.22464679915E-16,-1.,-1.81284143127026E-30));
#47625=DIRECTION('ref_axis',(1.57898385724467E-14,0.,-1.));
#47626=DIRECTION('center_axis',(0.106117864373042,-1.29956902936052E-17,
0.994353558278395));
#47627=DIRECTION('ref_axis',(0.994353558278395,-3.91187297993902E-33,-0.106117864373042));
#47628=DIRECTION('center_axis',(-1.22464679915E-16,-1.,-5.47382212627E-48));
#47629=DIRECTION('ref_axis',(1.,-1.22464679915E-16,-6.703498746053E-64));
#47630=DIRECTION('center_axis',(-4.52327322274045E-17,-1.,-5.91050929206098E-17));
#47631=DIRECTION('ref_axis',(-0.794132678900969,0.,0.607744426795977));
#47632=DIRECTION('center_axis',(0.607744426795977,-7.44272266974971E-17,
0.794132678900969));
#47633=DIRECTION('ref_axis',(0.794132678900969,-3.80543459761737E-32,-0.607744426795977));
#47634=DIRECTION('center_axis',(1.22464679915E-16,1.,5.47382212627E-48));
#47635=DIRECTION('ref_axis',(1.,-1.22464679915E-16,-6.703498746053E-64));
#47636=DIRECTION('center_axis',(-4.52327322274045E-17,-1.,-5.91050929206098E-17));
#47637=DIRECTION('ref_axis',(0.794132678900969,0.,-0.607744426795977));
#47638=DIRECTION('center_axis',(-0.734238830876792,8.99183234042744E-17,
0.678891257295808));
#47639=DIRECTION('ref_axis',(0.678891257295808,1.51038693775819E-31,0.734238830876792));
#47640=DIRECTION('center_axis',(-1.22464679915E-16,-1.,-1.23259516441E-32));
#47641=DIRECTION('ref_axis',(1.,-1.22464679915E-16,-1.50949372274247E-48));
#47642=DIRECTION('center_axis',(-0.540714503083014,0.0890998529400356,0.836474173158833));
#47643=DIRECTION('ref_axis',(0.803860483463198,0.347724019666725,0.482593337369186));
#47644=DIRECTION('center_axis',(0.757497881302333,-0.120607621490521,0.641600156998793));
#47645=DIRECTION('ref_axis',(0.519185231994408,0.707106824013922,-0.480048574950346));
#47646=DIRECTION('center_axis',(0.734238830876792,-8.991832340449E-17,-0.678891257295808));
#47647=DIRECTION('ref_axis',(-6.6021524650914E-17,-1.,6.10447636300053E-17));
#47648=DIRECTION('',(-0.734238830876791,0.,0.678891257295807));
#47649=DIRECTION('center_axis',(-1.2246467991486E-16,-1.,-1.56475089353662E-28));
#47650=DIRECTION('ref_axis',(-0.667272304480808,8.17172891841765E-17,0.744813850349785));
#47651=DIRECTION('',(0.,-1.,0.));
#47652=DIRECTION('center_axis',(-1.22464679915E-16,-1.,0.));
#47653=DIRECTION('ref_axis',(1.,-1.22464679915E-16,0.));
#47654=DIRECTION('',(0.,1.,0.));
#47655=DIRECTION('center_axis',(1.22464679915011E-16,1.,-3.67929656575737E-30));
#47656=DIRECTION('ref_axis',(-0.952128653909774,1.16602130838972E-16,0.305697606146927));
#47657=DIRECTION('',(-2.85587916301E-16,-1.,0.));
#47658=DIRECTION('center_axis',(-1.22464679915E-16,-1.,0.));
#47659=DIRECTION('ref_axis',(1.,-1.22464679915E-16,0.));
#47660=DIRECTION('center_axis',(-1.22464679914586E-16,-1.,-1.3947821589454E-28));
#47661=DIRECTION('ref_axis',(-0.947590338356885,1.16046347476986E-16,0.319487950715961));
#47662=DIRECTION('center_axis',(-1.22464679915E-16,-1.,6.16297582204E-33));
#47663=DIRECTION('ref_axis',(1.,-1.22464679915E-16,-7.0105395811531E-49));
#47664=DIRECTION('center_axis',(-1.22464679914997E-16,-1.,-3.04211334326766E-29));
#47665=DIRECTION('ref_axis',(-0.111333411199055,1.36344105663067E-17,0.993783110920478));
#47666=DIRECTION('',(-2.77555756156E-16,-1.,0.));
#47667=DIRECTION('center_axis',(-2.96428448085E-16,-1.,-1.50904692324E-15));
#47668=DIRECTION('ref_axis',(1.,-2.96428448085E-16,-4.47324437543477E-31));
#47669=DIRECTION('center_axis',(-1.22464679914586E-16,-1.,-1.3947821589454E-28));
#47670=DIRECTION('ref_axis',(-0.947590338356885,1.16046347476986E-16,0.319487950715961));
#47671=DIRECTION('',(0.,1.,0.));
#47672=DIRECTION('center_axis',(-1.22464679915E-16,-1.,6.16297582204E-33));
#47673=DIRECTION('ref_axis',(1.,-1.22464679915E-16,-7.0105395811531E-49));
#47674=DIRECTION('center_axis',(1.22464679915E-16,1.,-5.21020650422465E-33));
#47675=DIRECTION('ref_axis',(-6.38066271830923E-49,-5.21020650422465E-33,
-1.));
#47676=DIRECTION('',(0.,1.,0.));
#47677=DIRECTION('center_axis',(-3.04677329401E-20,1.,-1.36892417294E-16));
#47678=DIRECTION('ref_axis',(1.,3.04677329401E-20,-4.17080161163832E-36));
#47679=DIRECTION('center_axis',(-2.17357452795E-16,2.66186108837E-32,1.));
#47680=DIRECTION('ref_axis',(1.,2.56447231488414E-65,2.17357452795E-16));
#47681=DIRECTION('',(0.,1.,0.));
#47682=DIRECTION('',(1.,0.,1.09790153833E-16));
#47683=DIRECTION('center_axis',(-1.22464679915E-16,-1.,-1.94567767731298E-44));
#47684=DIRECTION('ref_axis',(2.38276793969895E-60,1.94567767731298E-44,
-1.));
#47685=DIRECTION('',(0.,1.,0.));
#47686=DIRECTION('center_axis',(2.45272844836E-16,1.,-1.36611674972E-16));
#47687=DIRECTION('ref_axis',(1.,-2.45272844836E-16,3.35071341581934E-32));
#47688=DIRECTION('center_axis',(-1.22464679914998E-16,-1.,-1.73663083545565E-29));
#47689=DIRECTION('ref_axis',(-0.095298509688002,1.16707014853003E-17,0.99544874004202));
#47690=DIRECTION('',(0.,1.,0.));
#47691=DIRECTION('center_axis',(1.22464679915E-16,1.,0.));
#47692=DIRECTION('ref_axis',(1.,-1.22464679915E-16,0.));
#47693=DIRECTION('center_axis',(1.224646799149E-16,1.,-1.07586726537792E-28));
#47694=DIRECTION('ref_axis',(0.678891257295809,-8.31402005216765E-17,0.73423883087679));
#47695=DIRECTION('',(0.,1.,0.));
#47696=DIRECTION('center_axis',(6.14568728566E-17,1.,-5.23898221099E-18));
#47697=DIRECTION('ref_axis',(1.,-6.14568728566E-17,3.21971463638802E-34));
#47698=DIRECTION('center_axis',(0.678891257295808,-8.31402005216763E-17,
0.734238830876792));
#47699=DIRECTION('ref_axis',(-1.22464679914784E-16,-1.,1.83887638005312E-34));
#47700=DIRECTION('',(0.,1.,0.));
#47701=DIRECTION('',(-0.734238830876791,0.,0.678891257295807));
#47702=DIRECTION('center_axis',(-1.224646799149E-16,-1.,1.07603845915075E-28));
#47703=DIRECTION('ref_axis',(0.67889125729581,-8.31402005216767E-17,0.734238830876789));
#47704=DIRECTION('center_axis',(-1.22365143363E-16,-1.,-6.12322590562E-17));
#47705=DIRECTION('ref_axis',(1.,-1.22365143363E-16,-7.49269415785227E-33));
#47706=DIRECTION('center_axis',(0.,1.,0.));
#47707=DIRECTION('ref_axis',(-0.00162555525320111,0.,0.999998678784187));
#47708=DIRECTION('center_axis',(0.734238830876792,-8.99183234042744E-17,
-0.678891257295808));
#47709=DIRECTION('ref_axis',(0.678891257295807,3.46311205996404E-31,0.734238830876791));
#47710=DIRECTION('center_axis',(0.732027802944257,-8.96475505763315E-17,
0.68127475787424));
#47711=DIRECTION('ref_axis',(0.68127475787424,-1.91888914560603E-31,-0.732027802944257));
#47712=DIRECTION('center_axis',(5.46401789901627E-17,1.,6.08764557973899E-17));
#47713=DIRECTION('ref_axis',(-0.744196935834912,0.,0.667960268798922));
#47714=DIRECTION('center_axis',(-0.667960268798921,8.18015405141904E-17,
-0.744196935834913));
#47715=DIRECTION('ref_axis',(0.744196935834913,-3.15837441223295E-32,-0.667960268798921));
#47716=DIRECTION('center_axis',(-1.22464679915E-16,-1.,-5.47382212627E-48));
#47717=DIRECTION('ref_axis',(1.,-1.22464679915E-16,6.49622071350503E-64));
#47718=DIRECTION('center_axis',(1.14444500362894E-17,1.,3.5644992269101E-17));
#47719=DIRECTION('ref_axis',(-0.952128653909774,0.,0.305697606146927));
#47720=DIRECTION('center_axis',(-0.305697606146928,3.74371594874912E-17,
-0.952128653909774));
#47721=DIRECTION('ref_axis',(0.952128653909774,-6.76944606262743E-33,-0.305697606146928));
#47722=DIRECTION('center_axis',(-1.22464679915E-16,-1.,-5.47382212627E-48));
#47723=DIRECTION('ref_axis',(1.,-1.22464679915E-16,-6.703498746053E-64));
#47724=DIRECTION('center_axis',(-0.222411493783323,0.670605060062733,-0.707687770737441));
#47725=DIRECTION('ref_axis',(-0.848579081651793,0.224251763465943,0.479191703564883));
#47726=DIRECTION('center_axis',(0.734238830876792,-8.99183234042744E-17,
-0.678891257295808));
#47727=DIRECTION('ref_axis',(0.678891257295807,3.46311205996404E-31,0.734238830876791));
#47728=DIRECTION('center_axis',(-0.299820876204079,3.67174676361097E-17,
-0.953995514765252));
#47729=DIRECTION('ref_axis',(0.953995514765252,-6.3869078326472E-32,-0.299820876204079));
#47730=DIRECTION('center_axis',(2.41898181523141E-16,1.,-1.1741867647411E-17));
#47731=DIRECTION('ref_axis',(0.99520202856178,-2.41886400693281E-16,-0.0978413120645785));
#47732=DIRECTION('center_axis',(-1.22464679915E-16,-1.,-5.47382212627E-48));
#47733=DIRECTION('ref_axis',(1.,-1.22464679915E-16,6.49622071350503E-64));
#47734=DIRECTION('center_axis',(-0.962126872935794,0.250387400346799,-0.107786966384449));
#47735=DIRECTION('ref_axis',(0.248830769651925,0.968145727536702,0.0278764834019926));
#47736=DIRECTION('center_axis',(0.152411459643054,-1.86650206205066E-17,
0.988317128744349));
#47737=DIRECTION('ref_axis',(0.988317128744349,-1.89428554374595E-32,-0.152411459643054));
#47738=DIRECTION('center_axis',(-0.993783110920478,1.2170333058406E-16,
-0.111333411199054));
#47739=DIRECTION('ref_axis',(0.111333411199054,1.57725565511394E-32,-0.993783110920478));
#47740=DIRECTION('center_axis',(2.41898181523141E-16,1.,-1.1741867647411E-17));
#47741=DIRECTION('ref_axis',(-0.999778332126524,2.41886400693281E-16,0.0210543727122351));
#47742=DIRECTION('center_axis',(0.110668766460438,2.4072234423934E-12,-0.99385734596577));
#47743=DIRECTION('ref_axis',(2.68725782367101E-10,1.,3.2344497450746E-11));
#47744=DIRECTION('center_axis',(-1.22464679915E-16,-1.,-5.47382212627E-48));
#47745=DIRECTION('ref_axis',(1.,-1.22464679915E-16,6.49622071350503E-64));
#47746=DIRECTION('center_axis',(0.,1.,0.));
#47747=DIRECTION('ref_axis',(-0.666832525280057,0.,-0.745207610823066));
#47748=DIRECTION('center_axis',(1.,-1.22464679915E-16,6.12323399574E-17));
#47749=DIRECTION('ref_axis',(1.22464679915E-16,1.,7.49879891332945E-33));
#47750=DIRECTION('center_axis',(1.,-1.22464679915E-16,6.12323399574E-17));
#47751=DIRECTION('ref_axis',(6.12323399574E-17,-7.49879891332945E-33,-1.));
#47752=DIRECTION('center_axis',(1.,0.,0.));
#47753=DIRECTION('ref_axis',(0.,1.,3.70074341541721E-15));
#47754=DIRECTION('',(1.,0.,2.65024142098E-16));
#47755=DIRECTION('center_axis',(0.,1.,0.));
#47756=DIRECTION('ref_axis',(0.66853651195256,0.,-0.743679320800507));
#47757=DIRECTION('center_axis',(0.106117864373042,-1.29956902936052E-17,
0.994353558278395));
#47758=DIRECTION('ref_axis',(0.994353558278395,-3.91187297993902E-33,-0.106117864373042));
#47759=DIRECTION('center_axis',(1.68490994230906E-17,1.,4.21844451941189E-17));
#47760=DIRECTION('ref_axis',(-0.928750804671078,0.,0.370704657136683));
#47761=DIRECTION('center_axis',(0.607744426797546,-1.7991646764781E-12,
0.794132678899768));
#47762=DIRECTION('ref_axis',(-4.46309655899322E-12,1.,5.68064114266551E-12));
#47763=DIRECTION('center_axis',(1.22464679915E-16,1.,5.47382212627E-48));
#47764=DIRECTION('ref_axis',(1.,-1.22464679915E-16,-6.703498746053E-64));
#47765=DIRECTION('center_axis',(0.,0.,1.));
#47766=DIRECTION('ref_axis',(1.,0.,0.));
#47767=DIRECTION('center_axis',(-0.734238830876792,8.99183234042744E-17,
0.678891257295808));
#47768=DIRECTION('ref_axis',(0.678891257295808,1.51038693775819E-31,0.734238830876792));
#47769=DIRECTION('center_axis',(0.734238830876792,-8.991832340449E-17,-0.678891257295808));
#47770=DIRECTION('ref_axis',(6.6021524650914E-17,1.,-6.10447636300053E-17));
#47771=DIRECTION('',(-0.734238830876791,0.,0.678891257295807));
#47772=DIRECTION('center_axis',(0.734238830876792,-8.99183234042744E-17,
-0.678891257295808));
#47773=DIRECTION('ref_axis',(-0.678891257295807,-3.46311205996404E-31,-0.734238830876791));
#47774=DIRECTION('center_axis',(0.734238830876792,-8.99183234042744E-17,
-0.678891257295808));
#47775=DIRECTION('ref_axis',(0.678891257295807,3.46311205996404E-31,0.734238830876791));
#47776=DIRECTION('',(0.734238830876791,0.,-0.678891257295807));
#47777=DIRECTION('center_axis',(6.60215246509141E-17,1.,-6.10447636300053E-17));
#47778=DIRECTION('ref_axis',(0.678891257295808,0.,0.734238830876791));
#47779=DIRECTION('center_axis',(-0.613815420645987,7.51707090161983E-17,
-0.789449573675983));
#47780=DIRECTION('ref_axis',(0.789449573675983,7.34020703099417E-32,-0.613815420645987));
#47781=DIRECTION('center_axis',(1.22464679915E-16,1.,5.47382212627E-48));
#47782=DIRECTION('ref_axis',(1.,-1.22464679915E-16,-6.703498746053E-64));
#47783=DIRECTION('center_axis',(3.85062311351295E-17,1.,5.68588026119494E-17));
#47784=DIRECTION('ref_axis',(-0.827993213361104,0.,0.560738119471071));
#47785=DIRECTION('center_axis',(-0.560738119471071,6.86706143170087E-17,
-0.827993213361104));
#47786=DIRECTION('ref_axis',(0.827993213361104,-2.38131063616686E-32,-0.560738119471071));
#47787=DIRECTION('center_axis',(-1.22464679915E-16,-1.,-5.47382212627E-48));
#47788=DIRECTION('ref_axis',(1.,-1.22464679915E-16,-6.703498746053E-64));
#47789=DIRECTION('center_axis',(3.85062311351295E-17,1.,5.68588026119494E-17));
#47790=DIRECTION('ref_axis',(0.827993213361104,0.,-0.560738119471072));
#47791=DIRECTION('center_axis',(1.22464679915E-16,1.,5.47382212627E-48));
#47792=DIRECTION('ref_axis',(1.,-1.22464679915E-16,-6.703498746053E-64));
#47793=DIRECTION('center_axis',(1.22464679915E-16,1.,5.47382212627E-48));
#47794=DIRECTION('ref_axis',(1.,-1.22464679915E-16,0.));
#85187=CARTESIAN_POINT('',(0.,0.,0.));
#85188=CARTESIAN_POINT('Origin',(8.21591479143,-23.2742356128,11.6886688365));
#85189=CARTESIAN_POINT('',(7.99564314217,-23.4742356128,11.4850014593));
#85190=CARTESIAN_POINT('',(8.01224741424,-22.8742356128,11.9089404858));
#85191=CARTESIAN_POINT('Ctrl Pts',(7.99564314217,-23.4742356128,11.4850014593));
#85192=CARTESIAN_POINT('Ctrl Pts',(7.98964252128,-23.4742356128,11.4914912894));
#85193=CARTESIAN_POINT('Ctrl Pts',(7.97859188254,-23.4732430341,11.5041738872));
#85194=CARTESIAN_POINT('Ctrl Pts',(7.97506561416,-23.4709827428,11.5096523074));
#85195=CARTESIAN_POINT('Ctrl Pts',(7.96049908281,-23.4651088112,11.5297325584));
#85196=CARTESIAN_POINT('Ctrl Pts',(7.94999449773,-23.4537301075,11.5494738265));
#85197=CARTESIAN_POINT('Ctrl Pts',(7.9432480685,-23.4460266432,11.5624437668));
#85198=CARTESIAN_POINT('Ctrl Pts',(7.93181038161,-23.4257772831,11.589727728));
#85199=CARTESIAN_POINT('Ctrl Pts',(7.92449811306,-23.4017307742,11.6153459759));
#85200=CARTESIAN_POINT('Ctrl Pts',(7.92150726931,-23.3879026248,11.6287650914));
#85201=CARTESIAN_POINT('Ctrl Pts',(7.91677660432,-23.3563766548,11.6571003353));
#85202=CARTESIAN_POINT('Ctrl Pts',(7.91547477954,-23.3227166577,11.6832984902));
#85203=CARTESIAN_POINT('Ctrl Pts',(7.9155846643,-23.3039994083,11.6969647216));
#85204=CARTESIAN_POINT('Ctrl Pts',(7.91959338184,-23.2114810387,11.7607695014));
#85205=CARTESIAN_POINT('Ctrl Pts',(7.93828028322,-23.1128615217,11.8131880532));
#85206=CARTESIAN_POINT('Ctrl Pts',(7.95813278234,-23.0338190575,11.8499462819));
#85207=CARTESIAN_POINT('Ctrl Pts',(7.9829584197,-22.9540055384,11.8818593216));
#85208=CARTESIAN_POINT('Ctrl Pts',(8.01224741424,-22.8742356128,11.9089404858));
#85209=CARTESIAN_POINT('',(8.03752439844,-23.4742356128,11.4474700229));
#85210=CARTESIAN_POINT('Origin',(8.21591479143,-23.4742356128,11.6886688365));
#85211=CARTESIAN_POINT('',(8.03752439844,-25.4742356128,11.4474700229));
#85212=CARTESIAN_POINT('',(8.03752439844,-22.6642356128,11.4474700229));
#85213=CARTESIAN_POINT('',(8.01224741424,-25.4742356128,11.9089404858));
#85214=CARTESIAN_POINT('Origin',(8.21591479143,-25.4742356128,11.6886688365));
#85215=CARTESIAN_POINT('',(8.01224741424,-24.1742356128,11.9089404858));
#85216=CARTESIAN_POINT('Origin',(7.16045579301E-17,-22.6642356128,0.580061096523));
#85217=CARTESIAN_POINT('',(8.73611663980898,-23.4697909663899,10.8942572011661));
#85218=CARTESIAN_POINT('',(8.73611663424,-25.4742356128,10.8942572059));
#85219=CARTESIAN_POINT('',(8.73611663424,-23.2742356128,10.8942572059));
#85220=CARTESIAN_POINT('Origin',(-1.62597327472E-14,-25.4742356128,0.580061096523));
#85221=CARTESIAN_POINT('',(8.67864985337,-23.4742356128,10.942657873));
#85222=CARTESIAN_POINT('Origin',(2.30650470794E-14,-23.4742356128,0.580061096523));
#85223=CARTESIAN_POINT('Origin',(8.65818093366798,-22.8777633816448,10.9233631052074));
#85224=CARTESIAN_POINT('Origin',(8.93001206801,-23.2742356128,11.1231776304));
#85225=CARTESIAN_POINT('',(9.1336794452,-22.8742356128,10.9029059811));
#85226=CARTESIAN_POINT('Ctrl Pts',(9.1336794452,-22.8742356128,10.9029059811));
#85227=CARTESIAN_POINT('Ctrl Pts',(9.12864186713826,-22.887974922811,10.8982344510715));
#85228=CARTESIAN_POINT('Ctrl Pts',(9.12335771886472,-22.9019293773381,10.8936712120832));
#85229=CARTESIAN_POINT('Ctrl Pts',(9.11787226943502,-22.9159664885182,10.8892648795277));
#85230=CARTESIAN_POINT('Ctrl Pts',(9.11216771025498,-22.9305642954016,10.8846825412613));
#85231=CARTESIAN_POINT('Ctrl Pts',(9.10624538901133,-22.9452518966254,10.8802696612691));
#85232=CARTESIAN_POINT('Ctrl Pts',(9.10013711659066,-22.9599342922501,10.8760617975029));
#85233=CARTESIAN_POINT('Ctrl Pts',(9.09343775296072,-22.9760374881251,10.8714467431089));
#85234=CARTESIAN_POINT('Ctrl Pts',(9.0865147798379,-22.9921346475642,10.8670780600761));
#85235=CARTESIAN_POINT('Ctrl Pts',(9.07938726585101,-23.0081598565969,10.8629836574886));
#85236=CARTESIAN_POINT('Ctrl Pts',(9.07426631747019,-23.0196735861245,10.8600419271266));
#85237=CARTESIAN_POINT('Ctrl Pts',(9.06903926975429,-23.0311515307987,10.8572413388931));
#85238=CARTESIAN_POINT('Ctrl Pts',(9.0637068507804,-23.0425837055347,10.8545884512405));
#85239=CARTESIAN_POINT('Ctrl Pts',(9.05410828995007,-23.0631620631552,10.8498131506434));
#85240=CARTESIAN_POINT('Ctrl Pts',(9.04417029772133,-23.0835899275873,10.8455159152366));
#85241=CARTESIAN_POINT('Ctrl Pts',(9.03386350882102,-23.1038677787328,10.8417281569271));
#85242=CARTESIAN_POINT('Ctrl Pts',(9.0241092043464,-23.1230586572963,10.8381434373616));
#85243=CARTESIAN_POINT('Ctrl Pts',(9.01402344674499,-23.1421190687442,10.8350133981201));
#85244=CARTESIAN_POINT('Ctrl Pts',(9.00355723569183,-23.1610637443997,10.8323801860489));
#85245=CARTESIAN_POINT('Ctrl Pts',(8.99509378474724,-23.1763832647359,10.830250851844));
#85246=CARTESIAN_POINT('Ctrl Pts',(8.98638093349722,-23.1916281008454,10.8284463322577));
#85247=CARTESIAN_POINT('Ctrl Pts',(8.97738730234821,-23.2067889067296,10.8270074448473));
#85248=CARTESIAN_POINT('Ctrl Pts',(8.96872247513198,-23.2213954389821,10.8256211626452));
#85249=CARTESIAN_POINT('Ctrl Pts',(8.95979676807654,-23.2359248322128,10.8245739094458));
#85250=CARTESIAN_POINT('Ctrl Pts',(8.95058185178658,-23.2503385870446,10.823924671162));
#85251=CARTESIAN_POINT('Ctrl Pts',(8.94184683855384,-23.2640016888274,10.8233092445188));
#85252=CARTESIAN_POINT('Ctrl Pts',(8.93285178149626,-23.2775613698534,10.8230512852217));
#85253=CARTESIAN_POINT('Ctrl Pts',(8.92357530042097,-23.2909480014561,10.82322518767));
#85254=CARTESIAN_POINT('Ctrl Pts',(8.91488039725482,-23.3034953741679,10.8233881875119));
#85255=CARTESIAN_POINT('Ctrl Pts',(8.90593815285812,-23.3158909022145,10.8239305650324));
#85256=CARTESIAN_POINT('Ctrl Pts',(8.89673528370321,-23.3280395843762,10.8249366440998));
#85257=CARTESIAN_POINT('Ctrl Pts',(8.88802059732318,-23.3395438178048,10.8258893538904));
#85258=CARTESIAN_POINT('Ctrl Pts',(8.87907214142089,-23.3508268089755,10.8272578606624));
#85259=CARTESIAN_POINT('Ctrl Pts',(8.86988374445289,-23.361770917696,10.8291354703124));
#85260=CARTESIAN_POINT('Ctrl Pts',(8.86073527603326,-23.3726674683521,10.8310049207342));
#85261=CARTESIAN_POINT('Ctrl Pts',(8.85134885107335,-23.3832284587279,10.8333788805503));
#85262=CARTESIAN_POINT('Ctrl Pts',(8.84172478760057,-23.3932960776091,10.8363732226571));
#85263=CARTESIAN_POINT('Ctrl Pts',(8.83247645671033,-23.4029706470832,10.8392506628029));
#85264=CARTESIAN_POINT('Ctrl Pts',(8.82300864068946,-23.4121896919426,10.8427009774483));
#85265=CARTESIAN_POINT('Ctrl Pts',(8.81332846159939,-23.4207716836739,10.8468501500846));
#85266=CARTESIAN_POINT('Ctrl Pts',(8.80383668759135,-23.4291866443162,10.8509185674783));
#85267=CARTESIAN_POINT('Ctrl Pts',(8.79414068539646,-23.4369892804721,10.8556588323708));
#85268=CARTESIAN_POINT('Ctrl Pts',(8.78425456845438,-23.4439657681908,10.8612131542089));
#85269=CARTESIAN_POINT('Ctrl Pts',(8.77462998987335,-23.4507576921243,10.8666205358237));
#85270=CARTESIAN_POINT('Ctrl Pts',(8.76482519042245,-23.4567666850184,10.8727994450304));
#85271=CARTESIAN_POINT('Ctrl Pts',(8.75486086381769,-23.4617528149732,10.8799042056571));
#85272=CARTESIAN_POINT('Ctrl Pts',(8.74867197648696,-23.4648497223439,10.8843170039098));
#85273=CARTESIAN_POINT('Ctrl Pts',(8.74242170151348,-23.4675511927818,10.889087426161));
#85274=CARTESIAN_POINT('Ctrl Pts',(8.73611663424,-23.4697908757,10.8942572059));
#85275=CARTESIAN_POINT('',(9.1336794452,-25.4742356128,10.9029059811));
#85276=CARTESIAN_POINT('',(9.1336794452,-24.1742356128,10.9029059811));
#85277=CARTESIAN_POINT('Origin',(8.93001206801,-25.4742356128,11.1231776304));
#85278=CARTESIAN_POINT('Origin',(10.806321674,-23.2742356128,10.0787147334));
#85279=CARTESIAN_POINT('',(11.0909930576,-25.4742356128,10.1733836478));
#85280=CARTESIAN_POINT('',(11.0909930576,-22.9538972343,10.1733836478));
#85281=CARTESIAN_POINT('',(11.0909930576,-22.6642356128,10.1733836478));
#85282=CARTESIAN_POINT('',(11.031648508,-25.4742356128,10.2767748704));
#85283=CARTESIAN_POINT('Origin',(10.806321674,-25.4742356128,10.0787147334));
#85284=CARTESIAN_POINT('',(11.031648508,-22.9538972343,10.2767748704));
#85285=CARTESIAN_POINT('',(11.031648508,-22.6642356128,10.2767748704));
#85286=CARTESIAN_POINT('Ctrl Pts',(11.0316485080236,-22.9538972342712,10.2767748704012));
#85287=CARTESIAN_POINT('Ctrl Pts',(11.0362618244719,-22.9574629735615,10.2715264443151));
#85288=CARTESIAN_POINT('Ctrl Pts',(11.0409289539567,-22.9603378044225,10.2658423505117));
#85289=CARTESIAN_POINT('Ctrl Pts',(11.0497741877589,-22.9645897469489,10.2541599678227));
#85290=CARTESIAN_POINT('Ctrl Pts',(11.0539505572373,-22.9660452016239,10.2482245763534));
#85291=CARTESIAN_POINT('Ctrl Pts',(11.0609089320228,-22.9675632436939,10.2375072647136));
#85292=CARTESIAN_POINT('Ctrl Pts',(11.0637741673946,-22.9678862078995,10.2328198127542));
#85293=CARTESIAN_POINT('Ctrl Pts',(11.0665081104589,-22.9678862078995,10.2280566842471));
#85294=CARTESIAN_POINT('Ctrl Pts',(11.0691844131435,-22.9678862078995,10.2233939779248));
#85295=CARTESIAN_POINT('Ctrl Pts',(11.0717346751094,-22.9675767047451,10.2186592052973));
#85296=CARTESIAN_POINT('Ctrl Pts',(11.0773589468691,-22.9661256456956,10.2075161455921));
#85297=CARTESIAN_POINT('Ctrl Pts',(11.0803172029966,-22.9647393225438,10.2010842541412));
#85298=CARTESIAN_POINT('Ctrl Pts',(11.0860358359614,-22.9605581903024,10.1874436600315));
#85299=CARTESIAN_POINT('Ctrl Pts',(11.0887021061436,-22.9576018392337,10.1802725862398));
#85300=CARTESIAN_POINT('Ctrl Pts',(11.0909930576014,-22.9538972342539,10.1733836478253));
#85301=CARTESIAN_POINT('Origin',(10.8795671881,-23.2742356128,9.85222376962));
#85302=CARTESIAN_POINT('',(11.0832345653,-25.4742356128,9.63195212036));
#85303=CARTESIAN_POINT('',(11.0832345653,-21.0742356128,9.63195212036));
#85304=CARTESIAN_POINT('',(11.0832345653,-23.2742356128,9.63195212036));
#85305=CARTESIAN_POINT('',(11.1657658425,-25.4742356128,9.94217003248));
#85306=CARTESIAN_POINT('Origin',(10.8795671881,-25.4742356128,9.85222376962));
#85307=CARTESIAN_POINT('',(11.1657658425,-21.0742356128,9.94217003248));
#85308=CARTESIAN_POINT('',(11.1657658425,-22.6642356128,9.94217003248));
#85309=CARTESIAN_POINT('Origin',(10.8795671881,-21.0742356128,9.85222376962));
#85310=CARTESIAN_POINT('Origin',(11.221722051,-23.1742356128,9.76000029674));
#85311=CARTESIAN_POINT('',(10.7039554837,-21.0742356128,9.28126343203));
#85312=CARTESIAN_POINT('',(10.7039554837,-25.4742356128,9.28126343203));
#85313=CARTESIAN_POINT('',(10.7039554837,-23.2742356128,9.28126343203));
#85314=CARTESIAN_POINT('',(11.080905232,-25.4742356128,9.62979837427));
#85315=CARTESIAN_POINT('',(9.20983954971,-21.0742356128,7.89977528084));
#85316=CARTESIAN_POINT('Origin',(10.9076228609,-23.2742356128,9.06099178277));
#85317=CARTESIAN_POINT('',(10.6707879888,-21.0742356128,8.87684715658));
#85318=CARTESIAN_POINT('Origin',(10.9076228609,-21.0742356128,9.06099178277));
#85319=CARTESIAN_POINT('',(10.6707879888,-25.4742356128,8.87684715658));
#85320=CARTESIAN_POINT('',(10.6707879888,-22.6642356128,8.87684715658));
#85321=CARTESIAN_POINT('Origin',(10.9076228609,-25.4742356128,9.06099178277));
#85322=CARTESIAN_POINT('Origin',(7.16045579301E-17,-22.6642356128,0.580061096523));
#85323=CARTESIAN_POINT('',(11.1917725091,-21.0742356128,8.1594148509));
#85324=CARTESIAN_POINT('',(11.1917725091,-25.4742356128,8.1594148509));
#85325=CARTESIAN_POINT('',(11.1917725091,-23.2742356128,8.1594148509));
#85326=CARTESIAN_POINT('Origin',(2.10437608802E-14,-25.4742356128,0.580061096523));
#85327=CARTESIAN_POINT('Origin',(-5.06274711921E-15,-21.0742356128,0.580061096523));
#85328=CARTESIAN_POINT('Origin',(11.4401704731,-23.2742356128,8.32763628675));
#85329=CARTESIAN_POINT('',(11.4067704497,-21.0742356128,8.02950135347));
#85330=CARTESIAN_POINT('Origin',(11.4401704731,-21.0742356128,8.32763628675));
#85331=CARTESIAN_POINT('',(11.4067704324828,-22.8742356736053,8.02950135644609));
#85332=CARTESIAN_POINT('',(11.4067704497,-23.1237854196,8.02950135347));
#85333=CARTESIAN_POINT('',(11.6438378494077,-23.4645367062672,8.107364636655));
#85334=CARTESIAN_POINT('Ctrl Pts',(11.4067704240483,-22.8742356736211,8.02950135948828));
#85335=CARTESIAN_POINT('Ctrl Pts',(11.406804630593,-22.8931971151233,8.02949752860505));
#85336=CARTESIAN_POINT('Ctrl Pts',(11.4072793786485,-22.9119159973912,8.02944297070681));
#85337=CARTESIAN_POINT('Ctrl Pts',(11.4081636215115,-22.9303682802508,8.02934885100158));
#85338=CARTESIAN_POINT('Ctrl Pts',(11.4093015847953,-22.9541151729595,8.02922772503799));
#85339=CARTESIAN_POINT('Ctrl Pts',(11.4111181074154,-22.9774225569164,8.02904008763942));
#85340=CARTESIAN_POINT('Ctrl Pts',(11.4136025576223,-23.0003019569523,8.02882283063887));
#85341=CARTESIAN_POINT('Ctrl Pts',(11.4158839595366,-23.0213114772456,8.0286233295438));
#85342=CARTESIAN_POINT('Ctrl Pts',(11.4187306210101,-23.041963354936,8.02839868544617));
#85343=CARTESIAN_POINT('Ctrl Pts',(11.4221516301857,-23.0622661414509,8.02819479359798));
#85344=CARTESIAN_POINT('Ctrl Pts',(11.4255161960669,-23.0822339519104,8.02799426576521));
#85345=CARTESIAN_POINT('Ctrl Pts',(11.4294208422657,-23.1018555855848,8.02781470906328));
#85346=CARTESIAN_POINT('Ctrl Pts',(11.433865073085,-23.121150855687,8.02771826496776));
#85347=CARTESIAN_POINT('Ctrl Pts',(11.4378046064153,-23.1382549087334,8.02763277329456));
#85348=CARTESIAN_POINT('Ctrl Pts',(11.4421665723171,-23.1550964914925,8.02761253148517));
#85349=CARTESIAN_POINT('Ctrl Pts',(11.4469532894184,-23.171677434704,8.02771668501094));
#85350=CARTESIAN_POINT('Ctrl Pts',(11.4493343026855,-23.1799251428787,8.02776849315448));
#85351=CARTESIAN_POINT('Ctrl Pts',(11.45182061247,-23.1881086229785,8.02785134438343));
#85352=CARTESIAN_POINT('Ctrl Pts',(11.4544133388932,-23.1962268038527,8.02797457619187));
#85353=CARTESIAN_POINT('Ctrl Pts',(11.4560833706917,-23.2014559017182,8.02805395249506));
#85354=CARTESIAN_POINT('Ctrl Pts',(11.4577973958969,-23.2066571892584,8.02815006675177));
#85355=CARTESIAN_POINT('Ctrl Pts',(11.4595579723806,-23.21182985295,8.02826447101687));
#85356=CARTESIAN_POINT('Ctrl Pts',(11.4608371058657,-23.215588012505,8.02834759056758));
#85357=CARTESIAN_POINT('Ctrl Pts',(11.4619902680251,-23.2188887018161,8.02842958664865));
#85358=CARTESIAN_POINT('Ctrl Pts',(11.4632664251937,-23.2224651114436,8.02852793871659));
#85359=CARTESIAN_POINT('Ctrl Pts',(11.4642974173963,-23.2253544502573,8.02860739618285));
#85360=CARTESIAN_POINT('Ctrl Pts',(11.4654089415283,-23.2284235612494,8.02869756181277));
#85361=CARTESIAN_POINT('Ctrl Pts',(11.4667526561535,-23.2320483579825,8.02881620022717));
#85362=CARTESIAN_POINT('Ctrl Pts',(11.4716505862419,-23.2452609856118,8.02924864521855));
#85363=CARTESIAN_POINT('Ctrl Pts',(11.476723057138,-23.2578514126002,8.02981125418537));
#85364=CARTESIAN_POINT('Ctrl Pts',(11.4819567085306,-23.2698805438842,8.03053293688576));
#85365=CARTESIAN_POINT('Ctrl Pts',(11.4891125155748,-23.2863275969878,8.031519670958));
#85366=CARTESIAN_POINT('Ctrl Pts',(11.4965676819051,-23.3017228895861,8.03280495670992));
#85367=CARTESIAN_POINT('Ctrl Pts',(11.5042645117035,-23.3161285879357,8.03446701167399));
#85368=CARTESIAN_POINT('Ctrl Pts',(11.5134123496989,-23.333250051988,8.03644239763791));
#85369=CARTESIAN_POINT('Ctrl Pts',(11.5228989659229,-23.3489714733738,8.03894962022515));
#85370=CARTESIAN_POINT('Ctrl Pts',(11.5326485135102,-23.3633433251174,8.04211213354388));
#85371=CARTESIAN_POINT('Ctrl Pts',(11.5413937056095,-23.3762346519401,8.04494885865768));
#85372=CARTESIAN_POINT('Ctrl Pts',(11.5503523954545,-23.3880408749711,8.04831209101017));
#85373=CARTESIAN_POINT('Ctrl Pts',(11.5594844411486,-23.3987638621671,8.0522969369301));
#85374=CARTESIAN_POINT('Ctrl Pts',(11.5675484360139,-23.4082327278062,8.0558157297738));
#85375=CARTESIAN_POINT('Ctrl Pts',(11.5757495248873,-23.4168566128402,8.05981987129089));
#85376=CARTESIAN_POINT('Ctrl Pts',(11.5840455773726,-23.4246048038136,8.06437911997429));
#85377=CARTESIAN_POINT('Ctrl Pts',(11.5912704990814,-23.4313526002225,8.06834970897998));
#85378=CARTESIAN_POINT('Ctrl Pts',(11.5985685290852,-23.4374349566399,8.07274238219416));
#85379=CARTESIAN_POINT('Ctrl Pts',(11.6058815281764,-23.4428171841118,8.07759494346571));
#85380=CARTESIAN_POINT('Ctrl Pts',(11.6122904881892,-23.4475340561116,8.08184762704481));
#85381=CARTESIAN_POINT('Ctrl Pts',(11.6187115020277,-23.4517117790196,8.08645452510614));
#85382=CARTESIAN_POINT('Ctrl Pts',(11.6250704319617,-23.4553328841096,8.09142084227157));
#85383=CARTESIAN_POINT('Ctrl Pts',(11.6303453144621,-23.4583366762679,8.0955405196039));
#85384=CARTESIAN_POINT('Ctrl Pts',(11.6355773644057,-23.4609566494751,8.09990789774777));
#85385=CARTESIAN_POINT('Ctrl Pts',(11.6406968626537,-23.4632004596753,8.10450322745316));
#85386=CARTESIAN_POINT('Ctrl Pts',(11.6417489768831,-23.4636615878026,8.10544761917633));
#85387=CARTESIAN_POINT('Ctrl Pts',(11.6427962324924,-23.4641069212813,8.10640153774678));
#85388=CARTESIAN_POINT('Ctrl Pts',(11.6438378503,-23.4645366935,8.10736463748));
#85389=CARTESIAN_POINT('',(11.6438378503,-25.4742356128,8.10736463748));
#85390=CARTESIAN_POINT('',(11.6438378503,-24.4693861731,8.10736463748));
#85391=CARTESIAN_POINT('Origin',(11.4401704731,-25.4742356128,8.32763628675));
#85392=CARTESIAN_POINT('Origin',(12.8942551175,-23.1742356128,9.2635243433));
#85393=CARTESIAN_POINT('',(12.7478394283,-25.4742356128,9.12814559847));
#85394=CARTESIAN_POINT('',(12.7478394285276,-23.4742356127672,9.12814559867721));
#85395=CARTESIAN_POINT('',(12.7478394283,-22.5760378048,9.12814559847));
#85396=CARTESIAN_POINT('',(12.1510854644,-25.4742356128,8.57637547707));
#85397=CARTESIAN_POINT('',(11.7384871149,-23.4742356128,8.19487915673));
#85398=CARTESIAN_POINT('Origin',(11.7384707086266,-22.6130235696614,8.19486399662491));
#85399=CARTESIAN_POINT('',(6.46706166421,-23.4742356128,3.32081842676));
#85400=CARTESIAN_POINT('Origin',(8.92072771219,-25.4742356128,12.3403523349));
#85401=CARTESIAN_POINT('',(9.18405109086,-25.4742356128,12.9924125631));
#85402=CARTESIAN_POINT('',(9.38771846805,-25.7742356128,12.7721409138));
#85403=CARTESIAN_POINT('Ctrl Pts',(9.18405109085604,-25.4742356128,12.9924125631043));
#85404=CARTESIAN_POINT('Ctrl Pts',(9.18405109085603,-25.4915889699708,12.9924125631043));
#85405=CARTESIAN_POINT('Ctrl Pts',(9.18506704327817,-25.5091509586982,12.9912971565068));
#85406=CARTESIAN_POINT('Ctrl Pts',(9.18716742200737,-25.5266577240362,12.989007694918));
#85407=CARTESIAN_POINT('Ctrl Pts',(9.18920364301532,-25.5436297314494,12.9867881667352));
#85408=CARTESIAN_POINT('Ctrl Pts',(9.19225937615859,-25.5605494747294,12.9834648633035));
#85409=CARTESIAN_POINT('Ctrl Pts',(9.19637109291018,-25.577145193568,12.9790123784317));
#85410=CARTESIAN_POINT('Ctrl Pts',(9.19702801738436,-25.5797966733586,12.9783010098088));
#85411=CARTESIAN_POINT('Ctrl Pts',(9.19771183581985,-25.582439822218,12.9775608837574));
#85412=CARTESIAN_POINT('Ctrl Pts',(9.19842262451815,-25.5850734653017,12.976791975009));
#85413=CARTESIAN_POINT('Ctrl Pts',(9.20271106230882,-25.6009631587567,12.9721528785487));
#85414=CARTESIAN_POINT('Ctrl Pts',(9.20798244683343,-25.6165082390736,12.966462002305));
#85415=CARTESIAN_POINT('Ctrl Pts',(9.21422564722063,-25.6314368687755,12.9597255814124));
#85416=CARTESIAN_POINT('Ctrl Pts',(9.21507861227714,-25.6334764636448,12.9588052310679));
#85417=CARTESIAN_POINT('Ctrl Pts',(9.21594966634115,-25.6355045241066,12.9578654196439));
#85418=CARTESIAN_POINT('Ctrl Pts',(9.21683873157363,-25.6375203320718,12.9569062165261));
#85419=CARTESIAN_POINT('Ctrl Pts',(9.22053698036576,-25.6459054978619,12.9529162148453));
#85420=CARTESIAN_POINT('Ctrl Pts',(9.22454701548163,-25.6540787107173,12.9485902011535));
#85421=CARTESIAN_POINT('Ctrl Pts',(9.22885958309505,-25.6619871955642,12.9439349706664));
#85422=CARTESIAN_POINT('Ctrl Pts',(9.23101586690176,-25.6659414379876,12.9416073554228));
#85423=CARTESIAN_POINT('Ctrl Pts',(9.2332477536728,-25.6698295357845,12.9391974685992));
#85424=CARTESIAN_POINT('Ctrl Pts',(9.23555354594216,-25.6736446998774,12.9367065617839));
#85425=CARTESIAN_POINT('Ctrl Pts',(9.23661514745997,-25.6754012258428,12.9355597323444));
#85426=CARTESIAN_POINT('Ctrl Pts',(9.23786437853895,-25.6774206517901,12.9342097543335));
#85427=CARTESIAN_POINT('Ctrl Pts',(9.23906757488256,-25.6793122990687,12.9329092711513));
#85428=CARTESIAN_POINT('Ctrl Pts',(9.24047771393935,-25.6815292985829,12.9313851124903));
#85429=CARTESIAN_POINT('Ctrl Pts',(9.24182444870364,-25.6835705571029,12.929929124854));
#85430=CARTESIAN_POINT('Ctrl Pts',(9.24269077028947,-25.6848647673463,12.9289922005395));
#85431=CARTESIAN_POINT('Ctrl Pts',(9.24702851674015,-25.6913449889886,12.9243009401738));
#85432=CARTESIAN_POINT('Ctrl Pts',(9.25189294570965,-25.6980495816226,12.919007545773));
#85433=CARTESIAN_POINT('Ctrl Pts',(9.25736979554345,-25.7047927115736,12.9130403476632));
#85434=CARTESIAN_POINT('Ctrl Pts',(9.26273984236593,-25.7114043450244,12.9071895147536));
#85435=CARTESIAN_POINT('Ctrl Pts',(9.26869935366587,-25.7180531264771,12.9006901484567));
#85436=CARTESIAN_POINT('Ctrl Pts',(9.27531632190389,-25.7245165097648,12.8934885636304));
#85437=CARTESIAN_POINT('Ctrl Pts',(9.28152670348966,-25.7305827435909,12.8867294878444));
#85438=CARTESIAN_POINT('Ctrl Pts',(9.28831672104179,-25.7364852360521,12.8793513061525));
#85439=CARTESIAN_POINT('Ctrl Pts',(9.29572291972933,-25.7420008228083,12.8713309055222));
#85440=CARTESIAN_POINT('Ctrl Pts',(9.29620779517355,-25.7423619220295,12.870805818972));
#85441=CARTESIAN_POINT('Ctrl Pts',(9.29669530270517,-25.7427213495874,12.8702779894634));
#85442=CARTESIAN_POINT('Ctrl Pts',(9.29718544861305,-25.7430790373084,12.8697474147999));
#85443=CARTESIAN_POINT('Ctrl Pts',(9.30425747107762,-25.7482398997328,12.8620920699751));
#85444=CARTESIAN_POINT('Ctrl Pts',(9.31188552467293,-25.7530410399209,12.8538658250417));
#85445=CARTESIAN_POINT('Ctrl Pts',(9.32005647568179,-25.7572618964892,12.8450655815725));
#85446=CARTESIAN_POINT('Ctrl Pts',(9.32798270924704,-25.7613563397148,12.8365289026605));
#85447=CARTESIAN_POINT('Ctrl Pts',(9.33642017572173,-25.7649041797592,12.8274516947767));
#85448=CARTESIAN_POINT('Ctrl Pts',(9.34532707567636,-25.7676848145053,12.8178633707713));
#85449=CARTESIAN_POINT('Ctrl Pts',(9.35386441150747,-25.7703500754572,12.808672884462));
#85450=CARTESIAN_POINT('Ctrl Pts',(9.36283322025893,-25.7723098092211,12.7990126145978));
#85451=CARTESIAN_POINT('Ctrl Pts',(9.37216502621645,-25.7733606539579,12.7889427107013));
#85452=CARTESIAN_POINT('Ctrl Pts',(9.37724758285781,-25.7739329952519,12.7834581499249));
#85453=CARTESIAN_POINT('Ctrl Pts',(9.38243724338762,-25.7742356128009,12.7778526977998));
#85454=CARTESIAN_POINT('Ctrl Pts',(9.38771846805,-25.7742356128,12.7721409138));
#85455=CARTESIAN_POINT('',(8.59814925255,-25.4742356128,12.4506765244));
#85456=CARTESIAN_POINT('',(8.21591479143,-25.7742356128,11.6886688365));
#85457=CARTESIAN_POINT('Origin',(8.21591479143,-25.4742356128,11.6886688365));
#85458=CARTESIAN_POINT('',(8.80181662974,-25.7742356128,12.2304048752));
#85459=CARTESIAN_POINT('Origin',(8.21591479143,-25.4742356128,11.6886688365));
#85460=CARTESIAN_POINT('Origin',(8.21591479143,-25.4742356128,11.6886688365));
#85461=CARTESIAN_POINT('Origin',(-1.62597327472E-14,-25.4742356128,0.580061096523));
#85462=CARTESIAN_POINT('',(8.93001206801,-25.7742356128,11.1231776304));
#85463=CARTESIAN_POINT('Origin',(-3.09260596606E-16,-25.7742356128,0.580061096523));
#85464=CARTESIAN_POINT('Origin',(8.93001206801,-25.4742356128,11.1231776304));
#85465=CARTESIAN_POINT('Origin',(8.93001206801,-25.4742356128,11.1231776304));
#85466=CARTESIAN_POINT('Origin',(8.93001206801,-25.4742356128,11.1231776304));
#85467=CARTESIAN_POINT('Origin',(9.58357319026,-25.4742356128,11.7274727362));
#85468=CARTESIAN_POINT('',(9.39452601497,-25.7742356128,11.5526761045));
#85469=CARTESIAN_POINT('',(9.16226904149,-25.7742356128,11.3379268674));
#85470=CARTESIAN_POINT('',(9.59819339216,-25.4742356128,11.3324044552));
#85471=CARTESIAN_POINT('',(9.36593641868,-25.4742356128,11.1176552182));
#85472=CARTESIAN_POINT('Origin',(9.39452601497,-25.4742356128,11.5526761045));
#85473=CARTESIAN_POINT('Origin',(9.80186076935,-25.4742356128,11.1121328059));
#85474=CARTESIAN_POINT('',(10.2106256241,-25.7742356128,11.5513494877));
#85475=CARTESIAN_POINT('Origin',(9.80186076935,-25.7742356128,11.1121328059));
#85476=CARTESIAN_POINT('',(10.0062431967,-25.4742356128,11.3317411468));
#85477=CARTESIAN_POINT('Origin',(9.80186076935,-25.4742356128,11.1121328059));
#85478=CARTESIAN_POINT('Origin',(10.2106256241,-25.4742356128,11.5513494877));
#85479=CARTESIAN_POINT('Origin',(3.28019248617E-15,-25.4742356128,0.580061096523));
#85480=CARTESIAN_POINT('',(11.256975342,-25.7742356128,10.4748350074));
#85481=CARTESIAN_POINT('Origin',(8.59564264812E-16,-25.7742356128,0.580061096523));
#85482=CARTESIAN_POINT('Origin',(-2.72521192632E-16,-25.4742356128,0.580061096523));
#85483=CARTESIAN_POINT('Origin',(11.256975342,-25.4742356128,10.4748350074));
#85484=CARTESIAN_POINT('Origin',(10.806321674,-25.4742356128,10.0787147334));
#85485=CARTESIAN_POINT('',(11.3756644412,-25.7742356128,10.2680525622));
#85486=CARTESIAN_POINT('Origin',(10.806321674,-25.7742356128,10.0787147334));
#85487=CARTESIAN_POINT('Origin',(11.3756644412,-25.4742356128,10.2680525622));
#85488=CARTESIAN_POINT('Origin',(-2.84607155346,-25.4742356128,5.53854202767));
#85489=CARTESIAN_POINT('',(11.4519644969,-25.7742356128,10.0321162953));
#85490=CARTESIAN_POINT('Origin',(-2.84607155346,-25.7742356128,5.53854202767));
#85491=CARTESIAN_POINT('Origin',(-2.84607155346,-25.4742356128,5.53854202767));
#85492=CARTESIAN_POINT('Origin',(11.4519644969,-25.4742356128,10.0321162953));
#85493=CARTESIAN_POINT('Origin',(10.8795671881,-25.4742356128,9.85222376962));
#85494=CARTESIAN_POINT('',(11.2869019425,-25.7742356128,9.4116804711));
#85495=CARTESIAN_POINT('Origin',(10.8795671881,-25.7742356128,9.85222376962));
#85496=CARTESIAN_POINT('Origin',(11.2869019425,-25.4742356128,9.4116804711));
#85497=CARTESIAN_POINT('Origin',(11.2845726092,-25.4742356128,9.409526725));
#85498=CARTESIAN_POINT('',(10.9076228609,-25.7742356128,9.06099178277));
#85499=CARTESIAN_POINT('',(11.0972624017,-25.7742356128,9.23633612693));
#85500=CARTESIAN_POINT('Origin',(10.9076228609,-25.4742356128,9.06099178277));
#85501=CARTESIAN_POINT('Origin',(10.9076228609,-25.4742356128,9.06099178277));
#85502=CARTESIAN_POINT('Origin',(10.9076228609,-25.4742356128,9.06099178277));
#85503=CARTESIAN_POINT('Origin',(2.10437608802E-14,-25.4742356128,0.580061096523));
#85504=CARTESIAN_POINT('',(11.4401704731,-25.7742356128,8.32763628675));
#85505=CARTESIAN_POINT('Origin',(-3.09260596606E-16,-25.7742356128,0.580061096523));
#85506=CARTESIAN_POINT('Origin',(11.4401704731,-25.4742356128,8.32763628675));
#85507=CARTESIAN_POINT('Origin',(11.4401704731,-25.4742356128,8.32763628675));
#85508=CARTESIAN_POINT('Origin',(11.4401704731,-25.4742356128,8.32763628675));
#85509=CARTESIAN_POINT('Origin',(11.9474180872,-25.4742356128,8.79664712633));
#85510=CARTESIAN_POINT('',(12.5441720511,-25.7742356128,9.34841724773));
#85511=CARTESIAN_POINT('Ctrl Pts',(12.5441720511,-25.7742356128,9.34841724773));
#85512=CARTESIAN_POINT('Ctrl Pts',(12.5539822763409,-25.7742356128001,9.33780722995768));
#85513=CARTESIAN_POINT('Ctrl Pts',(12.5634456430601,-25.7731910200537,9.3275154089535));
#85514=CARTESIAN_POINT('Ctrl Pts',(12.5724911176183,-25.7713070166777,9.31765005053512));
#85515=CARTESIAN_POINT('Ctrl Pts',(12.5817733359601,-25.7693737039942,9.30752648982309));
#85516=CARTESIAN_POINT('Ctrl Pts',(12.590615701935,-25.7665572829415,9.29785179003076));
#85517=CARTESIAN_POINT('Ctrl Pts',(12.5989798508501,-25.7630785008082,9.28870141850777));
#85518=CARTESIAN_POINT('Ctrl Pts',(12.6077176009545,-25.7594443320175,9.27914232761384));
#85519=CARTESIAN_POINT('Ctrl Pts',(12.6159336998732,-25.7550880979871,9.27015519076182));
#85520=CARTESIAN_POINT('Ctrl Pts',(12.623622484751,-25.7502477283811,9.26178486645217));
#85521=CARTESIAN_POINT('Ctrl Pts',(12.6283279817392,-25.7472854469589,9.25666227082029));
#85522=CARTESIAN_POINT('Ctrl Pts',(12.6328367078553,-25.7441415029729,9.2517699072643));
#85523=CARTESIAN_POINT('Ctrl Pts',(12.6371532053515,-25.7408663583315,9.24711174163293));
#85524=CARTESIAN_POINT('Ctrl Pts',(12.6446891080961,-25.7351484883423,9.23897934188115));
#85525=CARTESIAN_POINT('Ctrl Pts',(12.6516265314871,-25.7290305922244,9.23154438354611));
#85526=CARTESIAN_POINT('Ctrl Pts',(12.6579848548716,-25.7227419730146,9.22475891729431));
#85527=CARTESIAN_POINT('Ctrl Pts',(12.662046954928,-25.7187244044039,9.22042393129609));
#85528=CARTESIAN_POINT('Ctrl Pts',(12.665873268387,-25.714636311481,9.2163534156184));
#85529=CARTESIAN_POINT('Ctrl Pts',(12.6694732315878,-25.710528583226,9.21253012695852));
#85530=CARTESIAN_POINT('Ctrl Pts',(12.6740906881256,-25.7052598469562,9.2076262242703));
#85531=CARTESIAN_POINT('Ctrl Pts',(12.6783349748146,-25.6999590815914,9.20312778888616));
#85532=CARTESIAN_POINT('Ctrl Pts',(12.6822277695392,-25.6947156622293,9.19898775635845));
#85533=CARTESIAN_POINT('Ctrl Pts',(12.6841741669014,-25.6920939525483,9.1969177400946));
#85534=CARTESIAN_POINT('Ctrl Pts',(12.6860327378614,-25.6894862802653,9.19493721400768));
#85535=CARTESIAN_POINT('Ctrl Pts',(12.6878063838999,-25.6869020998827,9.19303982266937));
#85536=CARTESIAN_POINT('Ctrl Pts',(12.6887246962375,-25.6855641301432,9.19205744070731));
#85537=CARTESIAN_POINT('Ctrl Pts',(12.6894223110675,-25.6845279385757,9.19131139879719));
#85538=CARTESIAN_POINT('Ctrl Pts',(12.6902095492152,-25.6833392669281,9.19046563803261));
#85539=CARTESIAN_POINT('Ctrl Pts',(12.6909427979048,-25.6822321153875,9.18967788025659));
#85540=CARTESIAN_POINT('Ctrl Pts',(12.6917542381505,-25.6809931412886,9.18880313678734));
#85541=CARTESIAN_POINT('Ctrl Pts',(12.6928755092835,-25.6792284128773,9.18759052905043));
#85542=CARTESIAN_POINT('Ctrl Pts',(12.7010717825987,-25.6663285923428,9.17872660297269));
#85543=CARTESIAN_POINT('Ctrl Pts',(12.7083456542452,-25.6525959016894,9.17086003188428));
#85544=CARTESIAN_POINT('Ctrl Pts',(12.7146889305147,-25.6382910415628,9.16399975905503));
#85545=CARTESIAN_POINT('Ctrl Pts',(12.7215940637009,-25.6227191256968,9.15653183623932));
#85546=CARTESIAN_POINT('Ctrl Pts',(12.7273969802182,-25.6064695638937,9.15025579407772));
#85547=CARTESIAN_POINT('Ctrl Pts',(12.7321138526963,-25.5898298670075,9.14515424664999));
#85548=CARTESIAN_POINT('Ctrl Pts',(12.737124295717,-25.5721545421994,9.13973518713073));
#85549=CARTESIAN_POINT('Ctrl Pts',(12.7409100277816,-25.5540387942889,9.13564058265248));
#85550=CARTESIAN_POINT('Ctrl Pts',(12.7435088166785,-25.5357731503047,9.13282971245183));
#85551=CARTESIAN_POINT('Ctrl Pts',(12.746416898406,-25.5153336349699,9.12968430872993));
#85552=CARTESIAN_POINT('Ctrl Pts',(12.7478394282971,-25.4947060095316,9.12814559847313));
#85553=CARTESIAN_POINT('Ctrl Pts',(12.7478394282971,-25.4742356128,9.12814559847313));
#85554=CARTESIAN_POINT('',(11.9921712621,-25.7742356128,8.83802676724));
#85555=CARTESIAN_POINT('Origin',(-3.18408167778E-16,-25.7742356128,0.729452270839));
#85556=CARTESIAN_POINT('',(12.1784264826,-25.7742356128,9.98548488886));
#85557=CARTESIAN_POINT('Origin',(10.0415172382,-25.7742356128,8.33514586886));
#85558=CARTESIAN_POINT('Origin',(-3.09260596606E-16,-25.7742356128,0.580061096523));
#85559=CARTESIAN_POINT('Origin',(3.39394702409,-23.1742356128,-9.39793292047));
#85560=CARTESIAN_POINT('',(3.39394702409,-21.0742356128,-7.0794205347));
#85561=CARTESIAN_POINT('',(3.39394702409,-25.4742356128,-7.0794205347));
#85562=CARTESIAN_POINT('',(3.39394702409,-23.2742356128,-7.0794205347));
#85563=CARTESIAN_POINT('',(3.39394702409,-25.4742356128,-9.19678210318));
#85564=CARTESIAN_POINT('',(3.39394702409,-25.4742356128,-8.58812386759));
#85565=CARTESIAN_POINT('',(3.39394702409,-23.4742356128,-9.19678210416077));
#85566=CARTESIAN_POINT('',(3.39394702409,-23.2742356128,-9.19678210318));
#85567=CARTESIAN_POINT('',(3.39394702409,-23.4742356128,-7.94679080481));
#85568=CARTESIAN_POINT('',(3.39394702409,-23.4742356128,3.39628270998));
#85569=CARTESIAN_POINT('',(3.39394702409,-22.8742356071,-7.27665075406));
#85570=CARTESIAN_POINT('Ctrl Pts',(3.39394702409,-22.8742356071,-7.27665075406));
#85571=CARTESIAN_POINT('Ctrl Pts',(3.39394702409,-22.8963796807801,-7.27665075202916));
#85572=CARTESIAN_POINT('Ctrl Pts',(3.39394702409,-22.9185266226574,-7.27803164667852));
#85573=CARTESIAN_POINT('Ctrl Pts',(3.39394702409019,-22.9404763729725,-7.28076880448012));
#85574=CARTESIAN_POINT('Ctrl Pts',(3.39394702409038,-22.9635612306701,-7.28364751141022));
#85575=CARTESIAN_POINT('Ctrl Pts',(3.39394702409077,-22.9864277437381,-7.28802596271889));
#85576=CARTESIAN_POINT('Ctrl Pts',(3.39394702409072,-23.0088766193784,-7.29382800372885));
#85577=CARTESIAN_POINT('Ctrl Pts',(3.3939470240907,-23.0181604618048,-7.29622746619418));
#85578=CARTESIAN_POINT('Ctrl Pts',(3.39394702409061,-23.0273732778489,-7.29886989897477));
#85579=CARTESIAN_POINT('Ctrl Pts',(3.39394702409046,-23.0365026587174,-7.30174800896343));
#85580=CARTESIAN_POINT('Ctrl Pts',(3.39394702409007,-23.0599555275722,-7.30914171255472));
#85581=CARTESIAN_POINT('Ctrl Pts',(3.39394702409004,-23.0828466467018,-7.31809082810804));
#85582=CARTESIAN_POINT('Ctrl Pts',(3.39394702409001,-23.1049940708735,-7.32844271008414));
#85583=CARTESIAN_POINT('Ctrl Pts',(3.39394702408999,-23.1281264931002,-7.33925498797506));
#85584=CARTESIAN_POINT('Ctrl Pts',(3.39394702409,-23.1504472805791,-7.35159636510977));
#85585=CARTESIAN_POINT('Ctrl Pts',(3.39394702409,-23.1717995438951,-7.36526779521605));
#85586=CARTESIAN_POINT('Ctrl Pts',(3.39394702409,-23.1802621945299,-7.37068626233385));
#85587=CARTESIAN_POINT('Ctrl Pts',(3.39394702409,-23.1885732730389,-7.37631349194848));
#85588=CARTESIAN_POINT('Ctrl Pts',(3.39394702409,-23.1967252289902,-7.38213675751289));
#85589=CARTESIAN_POINT('Ctrl Pts',(3.39394702409,-23.216964154042,-7.39659422465562));
#85590=CARTESIAN_POINT('Ctrl Pts',(3.39394702409,-23.2362264780343,-7.41226456121671));
#85591=CARTESIAN_POINT('Ctrl Pts',(3.39394702409,-23.2544248664386,-7.42895825046336));
#85592=CARTESIAN_POINT('Ctrl Pts',(3.39394702409,-23.2663051018241,-7.43985619116538));
#85593=CARTESIAN_POINT('Ctrl Pts',(3.39394702409,-23.2777329032204,-7.45119035077379));
#85594=CARTESIAN_POINT('Ctrl Pts',(3.39394702409,-23.2886950564466,-7.46291290030111));
#85595=CARTESIAN_POINT('Ctrl Pts',(3.39394702409,-23.3092436284265,-7.48488683624042));
#85596=CARTESIAN_POINT('Ctrl Pts',(3.39394702407267,-23.3281539933134,-7.5082252168758));
#85597=CARTESIAN_POINT('Ctrl Pts',(3.39394702415533,-23.3453669419493,-7.53263177580096));
#85598=CARTESIAN_POINT('Ctrl Pts',(3.39394702418428,-23.351396654865,-7.54118141750917));
#85599=CARTESIAN_POINT('Ctrl Pts',(3.39394702422707,-23.3572183823464,-7.54986251226728));
#85600=CARTESIAN_POINT('Ctrl Pts',(3.39394702429189,-23.3628304875723,-7.55866347490331));
#85601=CARTESIAN_POINT('Ctrl Pts',(3.39394702449706,-23.3805929863697,-7.58651881295321));
#85602=CARTESIAN_POINT('Ctrl Pts',(3.39394702467124,-23.3962633147006,-7.61557726389403));
#85603=CARTESIAN_POINT('Ctrl Pts',(3.39394702467555,-23.4098082144408,-7.64551044052));
#85604=CARTESIAN_POINT('Ctrl Pts',(3.39394702468063,-23.4257384366872,-7.68071499465771));
#85605=CARTESIAN_POINT('Ctrl Pts',(3.39394702450576,-23.4387297283905,-7.71712955274666));
#85606=CARTESIAN_POINT('Ctrl Pts',(3.3939470243646,-23.448763496914,-7.75428420736052));
#85607=CARTESIAN_POINT('Ctrl Pts',(3.39394702420207,-23.4603148681498,-7.79705848579653));
#85608=CARTESIAN_POINT('Ctrl Pts',(3.39394702411207,-23.4679503272946,-7.84081579026664));
#85609=CARTESIAN_POINT('Ctrl Pts',(3.39394702409605,-23.4716451363039,-7.88490127919122));
#85610=CARTESIAN_POINT('Ctrl Pts',(3.39394702408857,-23.4733699118574,-7.90548084727437));
#85611=CARTESIAN_POINT('Ctrl Pts',(3.39394702409,-23.4742356128,-7.92613251437262));
#85612=CARTESIAN_POINT('Ctrl Pts',(3.39394702409,-23.4742356128,-7.94679080481));
#85613=CARTESIAN_POINT('',(3.39394702409,-21.0742356128,-7.27665075431));
#85614=CARTESIAN_POINT('',(3.39394702409,-23.1223803511,-7.27665075431));
#85615=CARTESIAN_POINT('',(3.39394702409,-21.0742356128,-6.14889144395));
#85616=CARTESIAN_POINT('Origin',(3.09394702409,-23.2742356128,-7.0794205347));
#85617=CARTESIAN_POINT('',(2.96616998276,-21.0742356128,-6.8079927769));
#85618=CARTESIAN_POINT('Origin',(3.09394702409,-21.0742356128,-7.0794205347));
#85619=CARTESIAN_POINT('',(2.96616998276,-25.4742356128,-6.8079927769));
#85620=CARTESIAN_POINT('',(2.96616998276,-22.6642356128,-6.8079927769));
#85621=CARTESIAN_POINT('Origin',(3.09394702409,-25.4742356128,-7.0794205347));
#85622=CARTESIAN_POINT('Origin',(-2.84607155346,-22.6642356128,5.53854202767));
#85623=CARTESIAN_POINT('',(2.60391380109,-21.0742356128,-6.97212274247));
#85624=CARTESIAN_POINT('',(2.60391380109,-25.4742356128,-6.97212274247));
#85625=CARTESIAN_POINT('',(2.60391380109,-23.2742356128,-6.97212274247));
#85626=CARTESIAN_POINT('Origin',(-2.84607155346,-25.4742356128,5.53854202767));
#85627=CARTESIAN_POINT('Origin',(-2.84607155346,-21.0742356128,5.53854202767));
#85628=CARTESIAN_POINT('Origin',(2.72372695744,-23.2742356128,-7.24715875387));
#85629=CARTESIAN_POINT('',(2.42372695744,-21.0742356128,-7.24715875387));
#85630=CARTESIAN_POINT('Origin',(2.72372695744,-21.0742356128,-7.24715875387));
#85631=CARTESIAN_POINT('',(2.42372695744,-25.4742356128,-7.24715875387));
#85632=CARTESIAN_POINT('',(2.42372695744,-23.2742356128,-7.24715875387));
#85633=CARTESIAN_POINT('Origin',(2.72372695744,-25.4742356128,-7.24715875387));
#85634=CARTESIAN_POINT('Origin',(2.42372695744,-23.1742356128,-8.1710440518));
#85635=CARTESIAN_POINT('',(2.42372695744,-21.0742356128,-7.96338790087));
#85636=CARTESIAN_POINT('',(2.42372695744,-21.0742356128,-6.11170048962));
#85637=CARTESIAN_POINT('',(2.42372695744,-25.4742356128,-7.96338790087));
#85638=CARTESIAN_POINT('',(2.42372695744,-23.2742356128,-7.96338790087));
#85639=CARTESIAN_POINT('',(2.42372695744,-25.4742356128,-8.58812386759));
#85640=CARTESIAN_POINT('Origin',(2.12372695744,-23.2742356128,-7.96338790087));
#85641=CARTESIAN_POINT('',(2.22735416732,-25.4742356128,-8.24492191546));
#85642=CARTESIAN_POINT('',(2.22735416732,-21.0742356128,-8.24492191546));
#85643=CARTESIAN_POINT('',(2.22735416732,-22.6642356128,-8.24492191546));
#85644=CARTESIAN_POINT('Origin',(2.12372695744,-25.4742356128,-7.96338790087));
#85645=CARTESIAN_POINT('Ctrl Pts',(2.22735416732076,-21.0742356128,-8.24492191546207));
#85646=CARTESIAN_POINT('Ctrl Pts',(2.24108151060133,-21.0742356128001,-8.23986914666857));
#85647=CARTESIAN_POINT('Ctrl Pts',(2.25402468097048,-21.0741856837446,-8.2339643074798));
#85648=CARTESIAN_POINT('Ctrl Pts',(2.26612777278258,-21.0741202589394,-8.22743715345324));
#85649=CARTESIAN_POINT('Ctrl Pts',(2.27875418582157,-21.0740520052548,-8.22062777416504));
#85650=CARTESIAN_POINT('Ctrl Pts',(2.29046668928501,-21.0739668868197,-8.21314184239419));
#85651=CARTESIAN_POINT('Ctrl Pts',(2.30125680627737,-21.0739039993993,-8.20522080345313));
#85652=CARTESIAN_POINT('Ctrl Pts',(2.31096366691234,-21.0738474254599,-8.19809498441526));
#85653=CARTESIAN_POINT('Ctrl Pts',(2.31992518748148,-21.0738088429042,-8.19061695362599));
#85654=CARTESIAN_POINT('Ctrl Pts',(2.32816585676089,-21.0738167151887,-8.1829436715627));
#85655=CARTESIAN_POINT('Ctrl Pts',(2.33583411214787,-21.0738240406482,-8.17580339150502));
#85656=CARTESIAN_POINT('Ctrl Pts',(2.34299563004193,-21.0738628977486,-8.16837895699461));
#85657=CARTESIAN_POINT('Ctrl Pts',(2.34958037155088,-21.0739142203341,-8.16084735325064));
#85658=CARTESIAN_POINT('Ctrl Pts',(2.35632821361967,-21.0739668141528,-8.15312919567072));
#85659=CARTESIAN_POINT('Ctrl Pts',(2.36247022703321,-21.0740324986314,-8.14529944422524));
#85660=CARTESIAN_POINT('Ctrl Pts',(2.36798314853736,-21.0740907554554,-8.13756859185097));
#85661=CARTESIAN_POINT('Ctrl Pts',(2.37385294559234,-21.0741527834987,-8.12933728754802));
#85662=CARTESIAN_POINT('Ctrl Pts',(2.3790097036189,-21.0742063911124,-8.12121921958259));
#85663=CARTESIAN_POINT('Ctrl Pts',(2.38348457893087,-21.0742268117467,-8.11347446948094));
#85664=CARTESIAN_POINT('Ctrl Pts',(2.38470841967809,-21.0742323966183,-8.11135634549074));
#85665=CARTESIAN_POINT('Ctrl Pts',(2.38588156616565,-21.074235499182,-8.10926612248979));
#85666=CARTESIAN_POINT('Ctrl Pts',(2.38700529704613,-21.0742356128,-8.10720902551531));
#85667=CARTESIAN_POINT('Ctrl Pts',(2.39285425271468,-21.0742362041755,-8.09650195212366));
#85668=CARTESIAN_POINT('Ctrl Pts',(2.39788657480719,-21.0742365265271,-8.08574567897341));
#85669=CARTESIAN_POINT('Ctrl Pts',(2.40220661886468,-21.0742366716414,-8.07496333800916));
#85670=CARTESIAN_POINT('Ctrl Pts',(2.4067318406694,-21.0742368236478,-8.06366889661274));
#85671=CARTESIAN_POINT('Ctrl Pts',(2.41047617380133,-21.0742367811817,-8.05234499029572));
#85672=CARTESIAN_POINT('Ctrl Pts',(2.41351966652779,-21.0742366497387,-8.04097775690518));
#85673=CARTESIAN_POINT('Ctrl Pts',(2.4166090583842,-21.0742365163134,-8.02943909346062));
#85674=CARTESIAN_POINT('Ctrl Pts',(2.41897665741814,-21.0742362912073,-8.0178546901109));
#85675=CARTESIAN_POINT('Ctrl Pts',(2.42065864862612,-21.0742360847615,-8.00618475553654));
#85676=CARTESIAN_POINT('Ctrl Pts',(2.42234140953528,-21.0742358782212,-7.9945094806475));
#85677=CARTESIAN_POINT('Ctrl Pts',(2.42333809291483,-21.0742356903582,-7.98274747425376));
#85678=CARTESIAN_POINT('Ctrl Pts',(2.42363412571554,-21.0742356316651,-7.97085050208861));
#85679=CARTESIAN_POINT('Ctrl Pts',(2.42369587368949,-21.0742356194226,-7.96836897326607));
#85680=CARTESIAN_POINT('Ctrl Pts',(2.42372695744,-21.0742356128,-7.96588157712267));
#85681=CARTESIAN_POINT('Ctrl Pts',(2.42372695744,-21.0742356128,-7.96338790087));
#85682=CARTESIAN_POINT('Origin',(3.09394702409,-23.2742356128,-9.19678210318));
#85683=CARTESIAN_POINT('',(3.20611083607784,-23.4742356128,-9.47502535777846));
#85684=CARTESIAN_POINT('Origin',(3.09394702409,-23.4742356128,-9.19678210318));
#85685=CARTESIAN_POINT('',(3.20611081633,-25.4742356128,-9.47502531282));
#85686=CARTESIAN_POINT('Origin',(3.09394702409,-25.4742356128,-9.19678210318));
#85687=CARTESIAN_POINT('',(3.20611081633,-20.0742356128,-9.47502531282));
#85688=CARTESIAN_POINT('Origin',(3.09394702409,-25.4742356128,-8.58812386759));
#85689=CARTESIAN_POINT('',(3.09394702409,-25.7742356128,-7.0794205347));
#85690=CARTESIAN_POINT('',(3.09394702409,-25.7742356128,-9.19678210318));
#85691=CARTESIAN_POINT('',(3.09394702409,-25.7742356128,-8.13810131894));
#85692=CARTESIAN_POINT('Origin',(3.09394702409,-25.4742356128,-9.19678210318));
#85693=CARTESIAN_POINT('Origin',(3.09394702409,-25.4742356128,-7.0794205347));
#85694=CARTESIAN_POINT('Origin',(3.09394702409,-25.4742356128,-7.0794205347));
#85695=CARTESIAN_POINT('Origin',(3.09394702409,-25.4742356128,-7.0794205347));
#85696=CARTESIAN_POINT('Origin',(-2.84607155346,-25.4742356128,5.53854202767));
#85697=CARTESIAN_POINT('',(2.72372695744,-25.7742356128,-7.24715875387));
#85698=CARTESIAN_POINT('Origin',(-2.84607155346,-25.7742356128,5.53854202767));
#85699=CARTESIAN_POINT('Origin',(2.72372695744,-25.4742356128,-7.24715875387));
#85700=CARTESIAN_POINT('Origin',(2.72372695744,-25.4742356128,-7.24715875387));
#85701=CARTESIAN_POINT('Origin',(2.72372695744,-25.4742356128,-7.24715875387));
#85702=CARTESIAN_POINT('Origin',(2.72372695744,-25.4742356128,-8.58812386759));
#85703=CARTESIAN_POINT('',(2.72372695744,-25.7742356128,-7.96338790087));
#85704=CARTESIAN_POINT('',(2.72372695744,-25.7742356128,-7.60527332737));
#85705=CARTESIAN_POINT('Origin',(2.72372695744,-25.4742356128,-7.96338790087));
#85706=CARTESIAN_POINT('Origin',(2.12372695744,-25.4742356128,-7.96338790087));
#85707=CARTESIAN_POINT('',(2.3309813772,-25.7742356128,-8.52645593005));
#85708=CARTESIAN_POINT('Origin',(2.12372695744,-25.7742356128,-7.96338790087));
#85709=CARTESIAN_POINT('Origin',(2.3309813772,-25.4742356128,-8.52645593005));
#85710=CARTESIAN_POINT('Origin',(-2.84607155346,-25.4742356128,5.53854202767));
#85711=CARTESIAN_POINT('',(-2.3573467526E-14,-25.7742356128,-9.1762777575));
#85712=CARTESIAN_POINT('',(0.207931717439474,-25.4742356128,-8.82796732002595));
#85713=CARTESIAN_POINT('Ctrl Pts',(-2.3573467526E-14,-25.7742356128,-9.1762777575));
#85714=CARTESIAN_POINT('Ctrl Pts',(0.0543179010637,-25.7751862689,-9.07845703679));
#85715=CARTESIAN_POINT('Ctrl Pts',(0.109343357832,-25.7400248661,-8.98386898437));
#85716=CARTESIAN_POINT('Ctrl Pts',(0.16325179783,-25.6940006666,-8.89703057892));
#85717=CARTESIAN_POINT('Ctrl Pts',(0.208904902043,-25.586489454,-8.82655958228));
#85718=CARTESIAN_POINT('Ctrl Pts',(0.207931718075,-25.4742356128,-8.82796731988));
#85719=CARTESIAN_POINT('Origin',(-2.84607155346,-25.7742356128,5.53854202767));
#85720=CARTESIAN_POINT('Origin',(-2.84607155346,-25.4742356128,5.53854202767));
#85721=CARTESIAN_POINT('Origin',(3.09394702409,-25.4742356128,-9.19678210318));
#85722=CARTESIAN_POINT('Origin',(3.09394702409,-25.4742356128,-9.19678210318));
#85723=CARTESIAN_POINT('Origin',(-2.84607155346,-25.4742356128,5.53854202767));
#85724=CARTESIAN_POINT('',(-3.64520546117E-14,-25.7742356128,-10.0919881826));
#85725=CARTESIAN_POINT('',(0.647446102181,-25.4742356128,-10.2675153591));
#85726=CARTESIAN_POINT('Ctrl Pts',(2.77555756156289E-16,-25.7742356128,
-10.0919881826));
#85727=CARTESIAN_POINT('Ctrl Pts',(0.0127666947406751,-25.7742356128,-10.0968936681105));
#85728=CARTESIAN_POINT('Ctrl Pts',(0.0271180838392129,-25.7739854886413,
-10.1023205735565));
#85729=CARTESIAN_POINT('Ctrl Pts',(0.0431487367547728,-25.773293591676,
-10.1082196250995));
#85730=CARTESIAN_POINT('Ctrl Pts',(0.05389738199205,-25.7728296707701,-10.1121749731822));
#85731=CARTESIAN_POINT('Ctrl Pts',(0.065400894022011,-25.7721663394268,
-10.1163419506036));
#85732=CARTESIAN_POINT('Ctrl Pts',(0.0776850226532396,-25.7712351361557,
-10.1206985310685));
#85733=CARTESIAN_POINT('Ctrl Pts',(0.0929874322081948,-25.7700751308952,
-10.1261255483634));
#85734=CARTESIAN_POINT('Ctrl Pts',(0.109500172992918,-25.7684996343647,
-10.1318460369282));
#85735=CARTESIAN_POINT('Ctrl Pts',(0.127205102846768,-25.7663646795551,
-10.1377881312263));
#85736=CARTESIAN_POINT('Ctrl Pts',(0.136057567773693,-25.7652972021504,
-10.1407591783753));
#85737=CARTESIAN_POINT('Ctrl Pts',(0.144896818651612,-25.7641306876289,
-10.1436826499001));
#85738=CARTESIAN_POINT('Ctrl Pts',(0.154175043372714,-25.7627912803035,
-10.1467024954506));
#85739=CARTESIAN_POINT('Ctrl Pts',(0.163453268093816,-25.761451872978,-10.1497223410011));
#85740=CARTESIAN_POINT('Ctrl Pts',(0.173170690817713,-25.7599402451658,
-10.1528388311902));
#85741=CARTESIAN_POINT('Ctrl Pts',(0.183778538386152,-25.7581340314033,
-10.1561762498561));
#85742=CARTESIAN_POINT('Ctrl Pts',(0.201065198147305,-25.7551906064939,
-10.161614942351));
#85743=CARTESIAN_POINT('Ctrl Pts',(0.217387269440654,-25.7520155315348,
-10.1666030373977));
#85744=CARTESIAN_POINT('Ctrl Pts',(0.232709678556698,-25.7487351314624,
-10.1711799585317));
#85745=CARTESIAN_POINT('Ctrl Pts',(0.249222845736503,-25.7451998000141,
-10.1761125682331));
#85746=CARTESIAN_POINT('Ctrl Pts',(0.264575283226697,-25.7415419604595,
-10.1805680336023));
#85747=CARTESIAN_POINT('Ctrl Pts',(0.278780403189311,-25.7379006349803,
-10.1845847080561));
#85748=CARTESIAN_POINT('Ctrl Pts',(0.283747727460943,-25.7366273163121,
-10.1859892808128));
#85749=CARTESIAN_POINT('Ctrl Pts',(0.288575211171245,-25.7353558696552,
-10.1873400786056));
#85750=CARTESIAN_POINT('Ctrl Pts',(0.293264740388737,-25.7340918048577,
-10.1886383529592));
#85751=CARTESIAN_POINT('Ctrl Pts',(0.306688881619296,-25.7304733213002,
-10.1923547640251));
#85752=CARTESIAN_POINT('Ctrl Pts',(0.318964875652885,-25.7269134297011,
-10.1956507029994));
#85753=CARTESIAN_POINT('Ctrl Pts',(0.330098484404839,-25.7235154506728,
-10.1985807972922));
#85754=CARTESIAN_POINT('Ctrl Pts',(0.33163100564525,-25.7230477249649,-10.1989841195069));
#85755=CARTESIAN_POINT('Ctrl Pts',(0.333141857760913,-25.7225830413197,
-10.1993804990849));
#85756=CARTESIAN_POINT('Ctrl Pts',(0.334630964292926,-25.7221216340532,
-10.1997700635937));
#85757=CARTESIAN_POINT('Ctrl Pts',(0.340784620245485,-25.7202148923185,
-10.2013799188375));
#85758=CARTESIAN_POINT('Ctrl Pts',(0.34656837976259,-25.7183638800075,-10.2028735271497));
#85759=CARTESIAN_POINT('Ctrl Pts',(0.35198311466046,-25.7165836270321,-10.2042604508819));
#85760=CARTESIAN_POINT('Ctrl Pts',(0.354690482109395,-25.7156935005444,
-10.2049539127479));
#85761=CARTESIAN_POINT('Ctrl Pts',(0.35730559201964,-25.7148210565333,-10.2056206967166));
#85762=CARTESIAN_POINT('Ctrl Pts',(0.359828577161451,-25.7139680222366,
-10.2062620182685));
#85763=CARTESIAN_POINT('Ctrl Pts',(0.361090069732355,-25.7135415050882,
-10.2065826790445));
#85764=CARTESIAN_POINT('Ctrl Pts',(0.362323886515271,-25.7131202917207,
-10.2068973089369));
#85765=CARTESIAN_POINT('Ctrl Pts',(0.363535529846051,-25.7127040568142,
-10.2072056663922));
#85766=CARTESIAN_POINT('Ctrl Pts',(0.364650472969556,-25.712321041256,-10.2074894141054));
#85767=CARTESIAN_POINT('Ctrl Pts',(0.364770803899085,-25.7122807741327,
-10.2075203139685));
#85768=CARTESIAN_POINT('Ctrl Pts',(0.366590937652134,-25.7116489007287,
-10.2079818068637));
#85769=CARTESIAN_POINT('Ctrl Pts',(0.366748799795484,-25.7115940976738,
-10.2080218326351));
#85770=CARTESIAN_POINT('Ctrl Pts',(0.366919439077047,-25.7115348150142,
-10.2080650866454));
#85771=CARTESIAN_POINT('Ctrl Pts',(0.367104605833077,-25.7114704193595,
-10.2081120060478));
#85772=CARTESIAN_POINT('Ctrl Pts',(0.389501333108037,-25.7036814838767,
-10.2137871125346));
#85773=CARTESIAN_POINT('Ctrl Pts',(0.410401281874009,-25.6955112103493,
-10.2188521723151));
#85774=CARTESIAN_POINT('Ctrl Pts',(0.429803208558037,-25.6871592795531,
-10.2233953578027));
#85775=CARTESIAN_POINT('Ctrl Pts',(0.442559404690514,-25.6816681307071,
-10.2263823686336));
#85776=CARTESIAN_POINT('Ctrl Pts',(0.454670476409811,-25.6760980541835,
-10.2291439086179));
#85777=CARTESIAN_POINT('Ctrl Pts',(0.466122175642957,-25.6704997865415,
-10.2316997585462));
#85778=CARTESIAN_POINT('Ctrl Pts',(0.480556931371571,-25.6634432245178,
-10.2349213825727));
#85779=CARTESIAN_POINT('Ctrl Pts',(0.493936616845627,-25.6563383359936,
-10.2378216347637));
#85780=CARTESIAN_POINT('Ctrl Pts',(0.506275616356922,-25.649249086395,-10.2404322659966));
#85781=CARTESIAN_POINT('Ctrl Pts',(0.512445116112571,-25.6457044615957,
-10.2417375816131));
#85782=CARTESIAN_POINT('Ctrl Pts',(0.518354491225542,-25.6421636198033,
-10.2429701357078));
#85783=CARTESIAN_POINT('Ctrl Pts',(0.524003849100926,-25.638633533667,-10.2441336784079));
#85784=CARTESIAN_POINT('Ctrl Pts',(0.526235482565565,-25.6372390639717,
-10.2445933060124));
#85785=CARTESIAN_POINT('Ctrl Pts',(0.52842660556555,-25.6358463010662,-10.2450421307954));
#85786=CARTESIAN_POINT('Ctrl Pts',(0.53057705908913,-25.6344556231107,-10.2454804579075));
#85787=CARTESIAN_POINT('Ctrl Pts',(0.531148531397364,-25.6340860573738,
-10.2455969411534));
#85788=CARTESIAN_POINT('Ctrl Pts',(0.53171713188043,-25.6337166391242,-10.2457126830695));
#85789=CARTESIAN_POINT('Ctrl Pts',(0.532282888338958,-25.6333473964984,
-10.2458276940714));
#85790=CARTESIAN_POINT('Ctrl Pts',(0.533630238942648,-25.6324680441423,
-10.2461015930973));
#85791=CARTESIAN_POINT('Ctrl Pts',(0.534961368822432,-25.6315896547556,
-10.2463713913334));
#85792=CARTESIAN_POINT('Ctrl Pts',(0.536274157225102,-25.630712658771,-10.2466376811725));
#85793=CARTESIAN_POINT('Ctrl Pts',(0.537260883005261,-25.6300534858644,
-10.2468378315157));
#85794=CARTESIAN_POINT('Ctrl Pts',(0.537698506461127,-25.6297596128986,
-10.2469265405115));
#85795=CARTESIAN_POINT('Ctrl Pts',(0.538805038270017,-25.6290097214713,
-10.2471504943624));
#85796=CARTESIAN_POINT('Ctrl Pts',(0.539170690684045,-25.6287619205419,
-10.2472244997056));
#85797=CARTESIAN_POINT('Ctrl Pts',(0.539609233626648,-25.6284640898016,
-10.2473132167283));
#85798=CARTESIAN_POINT('Ctrl Pts',(0.540163859237224,-25.6280854254163,
-10.2474252657462));
#85799=CARTESIAN_POINT('Ctrl Pts',(0.547924623835747,-25.6227868508452,
-10.2489931451136));
#85800=CARTESIAN_POINT('Ctrl Pts',(0.555251731899524,-25.6174552869425,
-10.2504479415432));
#85801=CARTESIAN_POINT('Ctrl Pts',(0.562169842897244,-25.6120958381659,
-10.2518022325599));
#85802=CARTESIAN_POINT('Ctrl Pts',(0.573305111815716,-25.6034693643494,
-10.2539820753912));
#85803=CARTESIAN_POINT('Ctrl Pts',(0.583378449603745,-25.5947641147587,
-10.2559016411584));
#85804=CARTESIAN_POINT('Ctrl Pts',(0.592367203409916,-25.5859391051817,
-10.2575864731877));
#85805=CARTESIAN_POINT('Ctrl Pts',(0.600561704306696,-25.5778938799534,
-10.2591224322174));
#85806=CARTESIAN_POINT('Ctrl Pts',(0.607850336182629,-25.569747293597,-10.2604624417005));
#85807=CARTESIAN_POINT('Ctrl Pts',(0.614214632612605,-25.5615083372879,
-10.2616195565446));
#85808=CARTESIAN_POINT('Ctrl Pts',(0.621304560947548,-25.5523300077696,
-10.2629086010464));
#85809=CARTESIAN_POINT('Ctrl Pts',(0.627247118265407,-25.5430378679536,
-10.2639706364414));
#85810=CARTESIAN_POINT('Ctrl Pts',(0.632051116031981,-25.5337020589155,
-10.2648221979346));
#85811=CARTESIAN_POINT('Ctrl Pts',(0.637187967973039,-25.5237194004904,
-10.2657327614949));
#85812=CARTESIAN_POINT('Ctrl Pts',(0.641026239505504,-25.5136885666782,
-10.266403109198));
#85813=CARTESIAN_POINT('Ctrl Pts',(0.643589723141555,-25.5037325098279,
-10.266848622649));
#85814=CARTESIAN_POINT('Ctrl Pts',(0.64583883367469,-25.4949974151249,-10.2672395005081));
#85815=CARTESIAN_POINT('Ctrl Pts',(0.64710868213128,-25.4863197852285,-10.2674574760169));
#85816=CARTESIAN_POINT('Ctrl Pts',(0.647387572639472,-25.4777990118003,
-10.2675053229145));
#85817=CARTESIAN_POINT('Ctrl Pts',(0.647426555016346,-25.4766080067597,
-10.2675120107929));
#85818=CARTESIAN_POINT('Ctrl Pts',(0.647446102180999,-25.4754201027178,
-10.2675153591));
#85819=CARTESIAN_POINT('Ctrl Pts',(0.647446102181,-25.4742356128,-10.2675153591));
#85820=CARTESIAN_POINT('Origin',(-2.84607155346,-25.4742356128,5.53854202767));
#85821=CARTESIAN_POINT('Origin',(-2.84607155346,-25.7742356128,5.53854202767));
#85822=CARTESIAN_POINT('Origin',(7.06664156103,-21.0742356128,-3.23658091327));
#85823=CARTESIAN_POINT('',(7.64099403241,-21.0742356128,-4.28030970457));
#85824=CARTESIAN_POINT('',(5.92940140951,-21.0742356128,-2.47090756951));
#85825=CARTESIAN_POINT('',(6.78519772096,-21.0742356128,-3.37560863704));
#85826=CARTESIAN_POINT('',(7.85893479751,-20.7742356128,-4.07415000213));
#85827=CARTESIAN_POINT('Ctrl Pts',(7.85893479751,-20.7742356128,-4.07415000213));
#85828=CARTESIAN_POINT('Ctrl Pts',(7.85183926652127,-20.7742356127998,-4.08086197525167));
#85829=CARTESIAN_POINT('Ctrl Pts',(7.84533191258089,-20.7747094757886,-4.08700495036613));
#85830=CARTESIAN_POINT('Ctrl Pts',(7.83943039491049,-20.7754368206059,-4.09255817936291));
#85831=CARTESIAN_POINT('Ctrl Pts',(7.83330363186861,-20.7761919262575,-4.09832336047068));
#85832=CARTESIAN_POINT('Ctrl Pts',(7.82782908140359,-20.7772197128011,-4.10345363014837));
#85833=CARTESIAN_POINT('Ctrl Pts',(7.82300251618872,-20.7783191472933,-4.10794846284614));
#85834=CARTESIAN_POINT('Ctrl Pts',(7.82041781215545,-20.7789079123134,-4.11035551873072));
#85835=CARTESIAN_POINT('Ctrl Pts',(7.81801860696792,-20.7795180417377,-4.11258065655733));
#85836=CARTESIAN_POINT('Ctrl Pts',(7.81580268710095,-20.7801243597889,-4.11462527537135));
#85837=CARTESIAN_POINT('Ctrl Pts',(7.8115806647721,-20.7812795858371,-4.11852091546893));
#85838=CARTESIAN_POINT('Ctrl Pts',(7.80802846205607,-20.7824184098577,-4.12177047634116));
#85839=CARTESIAN_POINT('Ctrl Pts',(7.80513688118672,-20.783408983068,-4.12440799958011));
#85840=CARTESIAN_POINT('Ctrl Pts',(7.80448775989285,-20.7836313535266,-4.12500008832839));
#85841=CARTESIAN_POINT('Ctrl Pts',(7.80387192759621,-20.7838464613465,-4.12556133630691));
#85842=CARTESIAN_POINT('Ctrl Pts',(7.80328928645214,-20.7840531729096,-4.12609212275007));
#85843=CARTESIAN_POINT('Ctrl Pts',(7.80170024694699,-20.7846169381762,-4.1275397387236));
#85844=CARTESIAN_POINT('Ctrl Pts',(7.80035804175691,-20.785117756612,-4.12876088185069));
#85845=CARTESIAN_POINT('Ctrl Pts',(7.79926085691167,-20.7855373871536,-4.12976226790216));
#85846=CARTESIAN_POINT('Ctrl Pts',(7.79871226448904,-20.7857472024244,-4.13026296092789));
#85847=CARTESIAN_POINT('Ctrl Pts',(7.79853440088772,-20.7858158360464,-4.13042047045815));
#85848=CARTESIAN_POINT('Ctrl Pts',(7.79826256025366,-20.7859215662924,-4.13066808561332));
#85849=CARTESIAN_POINT('Ctrl Pts',(7.7979907196196,-20.7860272965384,-4.13091570076849));
#85850=CARTESIAN_POINT('Ctrl Pts',(7.79762464761794,-20.7861689844856,-4.13125366213504));
#85851=CARTESIAN_POINT('Ctrl Pts',(7.79670305211903,-20.7865412504096,-4.13211202964214));
#85852=CARTESIAN_POINT('Ctrl Pts',(7.79077432765017,-20.7889360777444,-4.13763400153611));
#85853=CARTESIAN_POINT('Ctrl Pts',(7.78442746797871,-20.791913998756,-4.14376377093566));
#85854=CARTESIAN_POINT('Ctrl Pts',(7.77769431332228,-20.7956726711726,-4.15032683375898));
#85855=CARTESIAN_POINT('Ctrl Pts',(7.77605434143871,-20.7965881583992,-4.15192537694558));
#85856=CARTESIAN_POINT('Ctrl Pts',(7.77439162408683,-20.7975500115351,-4.15354946303284));
#85857=CARTESIAN_POINT('Ctrl Pts',(7.77270696753313,-20.7985611469581,-4.15519624304362));
#85858=CARTESIAN_POINT('Ctrl Pts',(7.76840633206434,-20.8011424000059,-4.15940018627946));
#85859=CARTESIAN_POINT('Ctrl Pts',(7.76396141066586,-20.8040448037012,-4.16375080512166));
#85860=CARTESIAN_POINT('Ctrl Pts',(7.75938461841096,-20.8073139488897,-4.16818508401255));
#85861=CARTESIAN_POINT('Ctrl Pts',(7.75745526485453,-20.8086920618877,-4.17005436084921));
#85862=CARTESIAN_POINT('Ctrl Pts',(7.75529472619584,-20.810286165269,-4.17213333375864));
#85863=CARTESIAN_POINT('Ctrl Pts',(7.753170537234,-20.8119177521571,-4.17416630948157));
#85864=CARTESIAN_POINT('Ctrl Pts',(7.75095089065221,-20.8136226599238,-4.17629064384886));
#85865=CARTESIAN_POINT('Ctrl Pts',(7.74877121181608,-20.8153685032777,-4.17836449142159));
#85866=CARTESIAN_POINT('Ctrl Pts',(7.74691494002475,-20.8168980893368,-4.18011674479675));
#85867=CARTESIAN_POINT('Ctrl Pts',(7.74633359759334,-20.8173771211698,-4.18066551100778));
#85868=CARTESIAN_POINT('Ctrl Pts',(7.74578381270852,-20.8178345854507,-4.18118288870584));
#85869=CARTESIAN_POINT('Ctrl Pts',(7.7452739071026,-20.8182617746731,-4.18166091416508));
#85870=CARTESIAN_POINT('Ctrl Pts',(7.73623209499571,-20.8258368329543,-4.1901374171386));
#85871=CARTESIAN_POINT('Ctrl Pts',(7.72791609663171,-20.8340692187894,-4.19800215501873));
#85872=CARTESIAN_POINT('Ctrl Pts',(7.72029634619406,-20.8427229030516,-4.20522725952926));
#85873=CARTESIAN_POINT('Ctrl Pts',(7.71545651995509,-20.8482194515934,-4.20981641906612));
#85874=CARTESIAN_POINT('Ctrl Pts',(7.71089683958716,-20.8538864976655,-4.21414823283737));
#85875=CARTESIAN_POINT('Ctrl Pts',(7.70660331641012,-20.8596698009706,-4.2182216252992));
#85876=CARTESIAN_POINT('Ctrl Pts',(7.70107672530996,-20.8671140259712,-4.22346486577998));
#85877=CARTESIAN_POINT('Ctrl Pts',(7.69599298422546,-20.8747513212587,-4.22828368619705));
#85878=CARTESIAN_POINT('Ctrl Pts',(7.69132291127602,-20.8824884583873,-4.23270372921761));
#85879=CARTESIAN_POINT('Ctrl Pts',(7.68931388380915,-20.8858169119628,-4.23460519583906));
#85880=CARTESIAN_POINT('Ctrl Pts',(7.68727656376502,-20.8893444390518,-4.23653209982262));
#85881=CARTESIAN_POINT('Ctrl Pts',(7.68534941494104,-20.8928381851489,-4.23835441195482));
#85882=CARTESIAN_POINT('Ctrl Pts',(7.68331638715091,-20.8965238802124,-4.24027684324861));
#85883=CARTESIAN_POINT('Ctrl Pts',(7.68140611510582,-20.9001715874312,-4.2420827359796));
#85884=CARTESIAN_POINT('Ctrl Pts',(7.67974560486613,-20.9034727800355,-4.2436530646065));
#85885=CARTESIAN_POINT('Ctrl Pts',(7.67932124059199,-20.904316441321,-4.24405438183538));
#85886=CARTESIAN_POINT('Ctrl Pts',(7.67891301835769,-20.9051373252889,-4.24444047509348));
#85887=CARTESIAN_POINT('Ctrl Pts',(7.67852273949611,-20.9059300251566,-4.24480965903291));
#85888=CARTESIAN_POINT('Ctrl Pts',(7.67352497797012,-20.9160810358573,-4.24953728707039));
#85889=CARTESIAN_POINT('Ctrl Pts',(7.66914206979505,-20.9263164258937,-4.25368328847564));
#85890=CARTESIAN_POINT('Ctrl Pts',(7.66528975762001,-20.9365851464252,-4.25732736873421));
#85891=CARTESIAN_POINT('Ctrl Pts',(7.66128653682442,-20.9472561288658,-4.2611142004366));
#85892=CARTESIAN_POINT('Ctrl Pts',(7.65785582893469,-20.9579639028255,-4.26435945938395));
#85893=CARTESIAN_POINT('Ctrl Pts',(7.65492517216004,-20.9686982280599,-4.26713169346425));
#85894=CARTESIAN_POINT('Ctrl Pts',(7.65187006261451,-20.9798883953195,-4.27002165276431));
#85895=CARTESIAN_POINT('Ctrl Pts',(7.64935794570938,-20.9911083156681,-4.27239796652737));
#85896=CARTESIAN_POINT('Ctrl Pts',(7.64733735079348,-21.0023832268463,-4.27430932661769));
#85897=CARTESIAN_POINT('Ctrl Pts',(7.64522595759957,-21.0141647920359,-4.2763065763653));
#85898=CARTESIAN_POINT('Ctrl Pts',(7.64365080122791,-21.026007495695,-4.27779657458376));
#85899=CARTESIAN_POINT('Ctrl Pts',(7.64259285259056,-21.0379639184472,-4.27879732574037));
#85900=CARTESIAN_POINT('Ctrl Pts',(7.64153490395321,-21.0499203411994,-4.27979807689698));
#85901=CARTESIAN_POINT('Ctrl Pts',(7.64099403240862,-21.0619917936591,-4.28030970457131));
#85902=CARTESIAN_POINT('Ctrl Pts',(7.64099403240862,-21.0742356128,-4.28030970457131));
#85903=CARTESIAN_POINT('',(6.1473421746,-20.7742356128,-2.26474786707));
#85904=CARTESIAN_POINT('',(7.00313848605,-20.7742356128,-3.1694489346));
#85905=CARTESIAN_POINT('Ctrl Pts',(5.92940140950644,-21.0742356128,-2.47090756951336));
#85906=CARTESIAN_POINT('Ctrl Pts',(5.92940140950644,-21.0620465213214,-2.47090756951336));
#85907=CARTESIAN_POINT('Ctrl Pts',(5.92995101839846,-21.0500039028176,-2.47041394631259));
#85908=CARTESIAN_POINT('Ctrl Pts',(5.93101943002766,-21.0380655608985,-2.46943347772656));
#85909=CARTESIAN_POINT('Ctrl Pts',(5.9320858573139,-21.0261493918611,-2.46845483014835));
#85910=CARTESIAN_POINT('Ctrl Pts',(5.93366928149062,-21.0143359647724,-2.46699103089334));
#85911=CARTESIAN_POINT('Ctrl Pts',(5.93577611680437,-21.0025880055739,-2.46501377374376));
#85912=CARTESIAN_POINT('Ctrl Pts',(5.93693874668391,-20.9961050458956,-2.46392264990193));
#85913=CARTESIAN_POINT('Ctrl Pts',(5.93826141371168,-20.9896422032718,-2.46267455482446));
#85914=CARTESIAN_POINT('Ctrl Pts',(5.93974980292276,-20.9831957720588,-2.46126037362452));
#85915=CARTESIAN_POINT('Ctrl Pts',(5.94256096536312,-20.9710202166559,-2.45858936993573));
#85916=CARTESIAN_POINT('Ctrl Pts',(5.94596922600863,-20.9589055034122,-2.45533644285574));
#85917=CARTESIAN_POINT('Ctrl Pts',(5.95004731874438,-20.9468901927177,-2.45145053613956));
#85918=CARTESIAN_POINT('Ctrl Pts',(5.95096515538695,-20.9441859647508,-2.45057595387651));
#85919=CARTESIAN_POINT('Ctrl Pts',(5.95191701489044,-20.9414869353962,-2.44966922051427));
#85920=CARTESIAN_POINT('Ctrl Pts',(5.95290388063803,-20.9387938528556,-2.44872960814046));
#85921=CARTESIAN_POINT('Ctrl Pts',(5.95558971347156,-20.9314644166798,-2.44617237908421));
#85922=CARTESIAN_POINT('Ctrl Pts',(5.95853458616578,-20.9241793796473,-2.44337210772868));
#85923=CARTESIAN_POINT('Ctrl Pts',(5.96175683895069,-20.9169637237193,-2.44031448175405));
#85924=CARTESIAN_POINT('Ctrl Pts',(5.96319285476145,-20.9137480244278,-2.43895183284472));
#85925=CARTESIAN_POINT('Ctrl Pts',(5.96478214034198,-20.9103349058105,-2.43744524137443));
#85926=CARTESIAN_POINT('Ctrl Pts',(5.96640032087268,-20.9070148772088,-2.43591232356138));
#85927=CARTESIAN_POINT('Ctrl Pts',(5.96807093993496,-20.9035872602254,-2.43432973022842));
#85928=CARTESIAN_POINT('Ctrl Pts',(5.96977220807806,-20.9002591791179,-2.43271921754394));
#85929=CARTESIAN_POINT('Ctrl Pts',(5.97133259130416,-20.8973175679299,-2.43124300810494));
#85930=CARTESIAN_POINT('Ctrl Pts',(5.97165222026851,-20.8967150081729,-2.43094062130261));
#85931=CARTESIAN_POINT('Ctrl Pts',(5.97196583563394,-20.8961285551134,-2.43064396641428));
#85932=CARTESIAN_POINT('Ctrl Pts',(5.97227182042976,-20.8955605161796,-2.43035457266878));
#85933=CARTESIAN_POINT('Ctrl Pts',(5.97602931122008,-20.8885850027176,-2.42680081984083));
#85934=CARTESIAN_POINT('Ctrl Pts',(5.98019629816105,-20.8813245480512,-2.42269456354623));
#85935=CARTESIAN_POINT('Ctrl Pts',(5.98491790960405,-20.8738972008456,-2.41798939022611));
#85936=CARTESIAN_POINT('Ctrl Pts',(5.98946154888746,-20.866749813361,-2.41346156946182));
#85937=CARTESIAN_POINT('Ctrl Pts',(5.99451930907194,-20.8594475486382,-2.40837863946706));
#85938=CARTESIAN_POINT('Ctrl Pts',(6.00022051682109,-20.8521423476661,-2.40269924115795));
#85939=CARTESIAN_POINT('Ctrl Pts',(6.00560265299428,-20.8452459867309,-2.39733769384615));
#85940=CARTESIAN_POINT('Ctrl Pts',(6.01155875634439,-20.8383470065419,-2.39144407574847));
#85941=CARTESIAN_POINT('Ctrl Pts',(6.01819022591929,-20.8316177623016,-2.38499059670732));
#85942=CARTESIAN_POINT('Ctrl Pts',(6.02246370269338,-20.8272812772068,-2.38083182126803));
#85943=CARTESIAN_POINT('Ctrl Pts',(6.02701749468084,-20.8230161860919,-2.37644068965293));
#85944=CARTESIAN_POINT('Ctrl Pts',(6.03187524669176,-20.8188792073734,-2.37181306735779));
#85945=CARTESIAN_POINT('Ctrl Pts',(6.03904491973146,-20.8127733409732,-2.36498304830108));
#85946=CARTESIAN_POINT('Ctrl Pts',(6.04690540802277,-20.8069436641881,-2.35765851382944));
#85947=CARTESIAN_POINT('Ctrl Pts',(6.05541988710496,-20.8016210284865,-2.34979781381991));
#85948=CARTESIAN_POINT('Ctrl Pts',(6.06364317348351,-20.796480425375,-2.34220594746024));
#85949=CARTESIAN_POINT('Ctrl Pts',(6.07247680878188,-20.7918134067092,-2.33411365367724));
#85950=CARTESIAN_POINT('Ctrl Pts',(6.08185538094852,-20.7878447886848,-2.32551390647897));
#85951=CARTESIAN_POINT('Ctrl Pts',(6.09099832383897,-20.7839758790783,-2.31713022118987));
#85952=CARTESIAN_POINT('Ctrl Pts',(6.10065940586829,-20.7807714248902,-2.30826403339204));
#85953=CARTESIAN_POINT('Ctrl Pts',(6.11074267212237,-20.7784463041617,-2.29894227287215));
#85954=CARTESIAN_POINT('Ctrl Pts',(6.12050826794062,-20.7761944357004,-2.2899141917665));
#85955=CARTESIAN_POINT('Ctrl Pts',(6.13066992045268,-20.7747681118582,-2.28045873909444));
#85956=CARTESIAN_POINT('Ctrl Pts',(6.14110482235127,-20.774358224677,-2.27063409101451));
#85957=CARTESIAN_POINT('Ctrl Pts',(6.14317369217154,-20.7742769586309,-2.26868621281644));
#85958=CARTESIAN_POINT('Ctrl Pts',(6.14525318677249,-20.7742356128,-2.26672393202862));
#85959=CARTESIAN_POINT('Ctrl Pts',(6.1473421746,-20.7742356128,-2.26474786707));
#85960=CARTESIAN_POINT('Origin',(0.00234331738835,-21.0742356128,3.08191746407));
#85961=CARTESIAN_POINT('',(8.05349668264,-20.7742356128,1.84629187045));
#85962=CARTESIAN_POINT('Origin',(0.00234331738835,-20.7742356128,3.08191746407));
#85963=CARTESIAN_POINT('',(7.75696851341,-21.0742356128,1.89180060423));
#85964=CARTESIAN_POINT('Ctrl Pts',(7.75696851340708,-21.0742356128,1.89180060423045));
#85965=CARTESIAN_POINT('Ctrl Pts',(7.75696851340708,-21.0616661584389,1.89180060423045));
#85966=CARTESIAN_POINT('Ctrl Pts',(7.75774249257575,-21.0492324960412,1.89166508636217));
#85967=CARTESIAN_POINT('Ctrl Pts',(7.75926820201175,-21.0369022993968,1.8914120010612));
#85968=CARTESIAN_POINT('Ctrl Pts',(7.76078851625566,-21.0246157046192,1.89115981071688));
#85969=CARTESIAN_POINT('Ctrl Pts',(7.76305543403818,-21.0124306480291,1.89079084973378));
#85970=CARTESIAN_POINT('Ctrl Pts',(7.76609704294065,-21.0003208010519,1.8903152156623));
#85971=CARTESIAN_POINT('Ctrl Pts',(7.76767607380167,-20.9940340552169,1.89006829342426));
#85972=CARTESIAN_POINT('Ctrl Pts',(7.76946470014536,-20.9877677810365,1.88979249855927));
#85973=CARTESIAN_POINT('Ctrl Pts',(7.7714719062634,-20.9815205326532,1.88948847860383));
#85974=CARTESIAN_POINT('Ctrl Pts',(7.77423444354622,-20.9729223840033,1.88907005298523));
#85975=CARTESIAN_POINT('Ctrl Pts',(7.77736366142895,-20.9644930346671,1.88859926473075));
#85976=CARTESIAN_POINT('Ctrl Pts',(7.78090592895025,-20.9561289601266,1.88806630410627));
#85977=CARTESIAN_POINT('Ctrl Pts',(7.78438936162325,-20.9479038076336,1.88754219562447));
#85978=CARTESIAN_POINT('Ctrl Pts',(7.78827253241698,-20.939741062644,1.8869579179785));
#85979=CARTESIAN_POINT('Ctrl Pts',(7.79264235226126,-20.9315661910541,1.88629756027545));
#85980=CARTESIAN_POINT('Ctrl Pts',(7.79681578785701,-20.9237587066955,1.88566687973438));
#85981=CARTESIAN_POINT('Ctrl Pts',(7.80143350528879,-20.915939583347,1.88496674416322));
#85982=CARTESIAN_POINT('Ctrl Pts',(7.80660547580603,-20.9080749321963,1.88417801872099));
#85983=CARTESIAN_POINT('Ctrl Pts',(7.80995423788519,-20.9029827056549,1.88366733254384));
#85984=CARTESIAN_POINT('Ctrl Pts',(7.81353604563579,-20.897872017984,1.88311940119982));
#85985=CARTESIAN_POINT('Ctrl Pts',(7.81738779919566,-20.892743072491,1.88252794322287));
#85986=CARTESIAN_POINT('Ctrl Pts',(7.82462310241973,-20.8831086357898,1.88141692255628));
#85987=CARTESIAN_POINT('Ctrl Pts',(7.83271540665919,-20.8735443563726,1.88019259901566));
#85988=CARTESIAN_POINT('Ctrl Pts',(7.84175563150046,-20.8642171343037,1.87881827297348));
#85989=CARTESIAN_POINT('Ctrl Pts',(7.84668640059003,-20.8591298296098,1.87806868051459));
#85990=CARTESIAN_POINT('Ctrl Pts',(7.85189894556063,-20.854113854674,1.87727449378871));
#85991=CARTESIAN_POINT('Ctrl Pts',(7.8574054894449,-20.8492024317588,1.87643010692974));
#85992=CARTESIAN_POINT('Ctrl Pts',(7.86520669548291,-20.8422443428183,1.8752338509839));
#85993=CARTESIAN_POINT('Ctrl Pts',(7.8735979524252,-20.8354966552672,1.87393871427795));
#85994=CARTESIAN_POINT('Ctrl Pts',(7.8825978759917,-20.8290738365449,1.87254643281156));
#85995=CARTESIAN_POINT('Ctrl Pts',(7.88709783777494,-20.8258624271837,1.87185029207836));
#85996=CARTESIAN_POINT('Ctrl Pts',(7.89174968103352,-20.822732539534,1.87113009993202));
#85997=CARTESIAN_POINT('Ctrl Pts',(7.89655375328037,-20.8197001322686,1.87038764109567));
#85998=CARTESIAN_POINT('Ctrl Pts',(7.89870392181544,-20.8183429114875,1.87005533726124));
#85999=CARTESIAN_POINT('Ctrl Pts',(7.901185677847,-20.8168201497101,1.86967235116843));
#86000=CARTESIAN_POINT('Ctrl Pts',(7.90359907289843,-20.8153894858188,1.86930032870983));
#86001=CARTESIAN_POINT('Ctrl Pts',(7.90623217468787,-20.8138285794724,1.86889443867501));
#86002=CARTESIAN_POINT('Ctrl Pts',(7.90878358936557,-20.8123773614406,1.86850164745361));
#86003=CARTESIAN_POINT('Ctrl Pts',(7.91070059863892,-20.8113116696728,1.86820712823749));
#86004=CARTESIAN_POINT('Ctrl Pts',(7.9109522801952,-20.8111717564411,1.86816846120771));
#86005=CARTESIAN_POINT('Ctrl Pts',(7.91119299389188,-20.8110384236042,1.86813149309831));
#86006=CARTESIAN_POINT('Ctrl Pts',(7.91142146587712,-20.8109122481099,1.86809642019366));
#86007=CARTESIAN_POINT('Ctrl Pts',(7.91772242298953,-20.8074324937851,1.86712915557353));
#86008=CARTESIAN_POINT('Ctrl Pts',(7.92487299159786,-20.8037803081172,1.86603160716374));
#86009=CARTESIAN_POINT('Ctrl Pts',(7.93293913642026,-20.800148831898,1.86479361588198));
#86010=CARTESIAN_POINT('Ctrl Pts',(7.94056676519282,-20.7967147809225,1.86362292800955));
#86011=CARTESIAN_POINT('Ctrl Pts',(7.9490140035596,-20.7932995377014,1.86232651780251));
#86012=CARTESIAN_POINT('Ctrl Pts',(7.95831982767407,-20.7901088517458,1.86089837350558));
#86013=CARTESIAN_POINT('Ctrl Pts',(7.96730267214303,-20.7870289057532,1.85951979618231));
#86014=CARTESIAN_POINT('Ctrl Pts',(7.97708639509304,-20.7841585184049,1.85801833885613));
#86015=CARTESIAN_POINT('Ctrl Pts',(7.98767748349669,-20.7817192873822,1.85639297870789));
#86016=CARTESIAN_POINT('Ctrl Pts',(7.99768726647839,-20.7794139366714,1.85485682852852));
#86017=CARTESIAN_POINT('Ctrl Pts',(8.00841878677286,-20.7774942736015,1.85320991650343));
#86018=CARTESIAN_POINT('Ctrl Pts',(8.01984167864081,-20.7761741033989,1.85145687957012));
#86019=CARTESIAN_POINT('Ctrl Pts',(8.03048065196714,-20.7749445324868,1.84982414826274));
#86020=CARTESIAN_POINT('Ctrl Pts',(8.04171959731026,-20.7742356128001,1.84809932180418));
#86021=CARTESIAN_POINT('Ctrl Pts',(8.05349668264,-20.7742356128,1.84629187045));
#86022=CARTESIAN_POINT('',(5.92101866809,-21.0742356128,-2.06782739988));
#86023=CARTESIAN_POINT('Origin',(0.00234331738835,-21.0742356128,3.08191746407));
#86024=CARTESIAN_POINT('Origin',(6.14734217460299,-21.0742356128,-2.26474786707535));
#86025=CARTESIAN_POINT('Origin',(-8.59172680003,-21.0742356128,1.84629187045));
#86026=CARTESIAN_POINT('',(11.0596214465,-20.7742356128,1.84629187045));
#86027=CARTESIAN_POINT('',(9.55655906459,-20.7742356128,1.84629187045));
#86028=CARTESIAN_POINT('',(11.0596214465,-21.0742356128,2.14629187045));
#86029=CARTESIAN_POINT('Ctrl Pts',(11.0596214465,-20.7742356128,1.84629187045));
#86030=CARTESIAN_POINT('Ctrl Pts',(11.0596214514713,-20.7742356128,1.86570125826323));
#86031=CARTESIAN_POINT('Ctrl Pts',(11.059621456438,-20.7761238547456,1.88504253295737));
#86032=CARTESIAN_POINT('Ctrl Pts',(11.0596214756218,-20.7798335852751,1.90397589067421));
#86033=CARTESIAN_POINT('Ctrl Pts',(11.0596214903527,-20.7826822310291,1.91851452862674));
#86034=CARTESIAN_POINT('Ctrl Pts',(11.059621513363,-20.786621837117,1.93289102969955));
#86035=CARTESIAN_POINT('Ctrl Pts',(11.0596215459651,-20.7916084043232,1.94689933055417));
#86036=CARTESIAN_POINT('Ctrl Pts',(11.0596215513868,-20.7924376650847,1.94922889591513));
#86037=CARTESIAN_POINT('Ctrl Pts',(11.0596215570631,-20.7932957658107,1.95154830433926));
#86038=CARTESIAN_POINT('Ctrl Pts',(11.0596215629872,-20.7941823691093,1.95385664488059));
#86039=CARTESIAN_POINT('Ctrl Pts',(11.0596215996861,-20.7996747577981,1.9681565053698));
#86040=CARTESIAN_POINT('Ctrl Pts',(11.0596216464123,-20.8062505351596,1.98200383104242));
#86041=CARTESIAN_POINT('Ctrl Pts',(11.0596217085961,-20.8138429039508,1.99527387331651));
#86042=CARTESIAN_POINT('Ctrl Pts',(11.0596217625585,-20.8204314682786,2.00678945291488));
#86043=CARTESIAN_POINT('Ctrl Pts',(11.0596218281764,-20.8277896556534,2.01787429563428));
#86044=CARTESIAN_POINT('Ctrl Pts',(11.0596219124487,-20.835846848425,2.02842038831454));
#86045=CARTESIAN_POINT('Ctrl Pts',(11.059621983873,-20.842675656481,2.03735864320007));
#86046=CARTESIAN_POINT('Ctrl Pts',(11.0596220686938,-20.8500054114903,2.04590963456982));
#86047=CARTESIAN_POINT('Ctrl Pts',(11.0596221745448,-20.8577913720448,2.05402220199404));
#86048=CARTESIAN_POINT('Ctrl Pts',(11.0596222613442,-20.8641759739613,2.06067462633664));
#86049=CARTESIAN_POINT('Ctrl Pts',(11.0596223622858,-20.8708674013712,2.06703237410384));
#86050=CARTESIAN_POINT('Ctrl Pts',(11.0596224948845,-20.8778366192505,2.07306804938344));
#86051=CARTESIAN_POINT('Ctrl Pts',(11.0596225983655,-20.8832754459947,2.07777833290419));
#86052=CARTESIAN_POINT('Ctrl Pts',(11.0596227211269,-20.8888833845846,2.08229251640741));
#86053=CARTESIAN_POINT('Ctrl Pts',(11.0596228734679,-20.8946459379248,2.0865990669219));
#86054=CARTESIAN_POINT('Ctrl Pts',(11.0596229829271,-20.8987864179635,2.0896933873365));
#86055=CARTESIAN_POINT('Ctrl Pts',(11.0596231076574,-20.9030067046001,2.09268053834455));
#86056=CARTESIAN_POINT('Ctrl Pts',(11.0596233102948,-20.9073012235333,2.09555660858332));
#86057=CARTESIAN_POINT('Ctrl Pts',(11.0596234335262,-20.9099128823873,2.09730565531492));
#86058=CARTESIAN_POINT('Ctrl Pts',(11.05962358557,-20.9125519917939,2.09901362387901));
#86059=CARTESIAN_POINT('Ctrl Pts',(11.0596238053652,-20.9152170612572,2.10067956720373));
#86060=CARTESIAN_POINT('Ctrl Pts',(11.0596238835097,-20.9161645813609,2.10127186500815));
#86061=CARTESIAN_POINT('Ctrl Pts',(11.0596239702182,-20.9171153822968,2.10185885195));
#86062=CARTESIAN_POINT('Ctrl Pts',(11.0596243586793,-20.9180695616141,2.10244058594263));
#86063=CARTESIAN_POINT('Ctrl Pts',(11.0596295564672,-20.9308369188505,2.1102244537817));
#86064=CARTESIAN_POINT('Ctrl Pts',(11.0596887741995,-20.9442101040438,2.11706359965047));
#86065=CARTESIAN_POINT('Ctrl Pts',(11.0597786773667,-20.958006572114,2.12286154590208));
#86066=CARTESIAN_POINT('Ctrl Pts',(11.0598685819633,-20.971803259534,2.12865958433516));
#86067=CARTESIAN_POINT('Ctrl Pts',(11.0599892148189,-20.986027642207,2.13342149132777));
#86068=CARTESIAN_POINT('Ctrl Pts',(11.0600749747649,-21.0005419751008,2.13709943925585));
#86069=CARTESIAN_POINT('Ctrl Pts',(11.0601461047687,-21.0125802820666,2.14014995948896));
#86070=CARTESIAN_POINT('Ctrl Pts',(11.0601932330123,-21.0248049323751,2.14245042568098));
#86071=CARTESIAN_POINT('Ctrl Pts',(11.0601138668724,-21.0371032668211,2.14398457510411));
#86072=CARTESIAN_POINT('Ctrl Pts',(11.0600344938244,-21.0494026717346,2.14551885806216));
#86073=CARTESIAN_POINT('Ctrl Pts',(11.0598278725422,-21.0618265078302,2.14629187045));
#86074=CARTESIAN_POINT('Ctrl Pts',(11.0596214465,-21.0742356128,2.14629187045));
#86075=CARTESIAN_POINT('',(8.05349668264,-21.0742356128,2.14629187045));
#86076=CARTESIAN_POINT('',(9.55655906459,-21.0742356128,2.14629187045));
#86077=CARTESIAN_POINT('Origin',(8.05349668264,-21.0742356128,1.84629187045));
#86078=CARTESIAN_POINT('Origin',(-2.84607155346,-21.0742356128,5.53854202767));
#86079=CARTESIAN_POINT('',(11.3495744826,-21.0742356128,1.76930332028));
#86080=CARTESIAN_POINT('',(8.08214906615,-21.0742356128,-4.27458799822));
#86081=CARTESIAN_POINT('Origin',(-2.84607155346,-21.0742356128,5.53854202767));
#86082=CARTESIAN_POINT('Ctrl Pts',(11.0596214465,-20.7742356128,1.84629187045));
#86083=CARTESIAN_POINT('Ctrl Pts',(11.070799043927,-20.7742356127963,1.84332398630273));
#86084=CARTESIAN_POINT('Ctrl Pts',(11.0812745407999,-20.7749023807717,1.84056790739039));
#86085=CARTESIAN_POINT('Ctrl Pts',(11.090984392949,-20.7759944024526,1.83801248606312));
#86086=CARTESIAN_POINT('Ctrl Pts',(11.0983251775274,-20.7768199861785,1.83608055165439));
#86087=CARTESIAN_POINT('Ctrl Pts',(11.105229605784,-20.7778890057565,1.83426296451625));
#86088=CARTESIAN_POINT('Ctrl Pts',(11.1116861224859,-20.7791077535672,1.83255059549683));
#86089=CARTESIAN_POINT('Ctrl Pts',(11.1191844845229,-20.7805231626395,1.83056191283071));
#86090=CARTESIAN_POINT('Ctrl Pts',(11.1260816354282,-20.7821401240567,1.82871994583986));
#86091=CARTESIAN_POINT('Ctrl Pts',(11.1323879808919,-20.7838325871391,1.82702746924725));
#86092=CARTESIAN_POINT('Ctrl Pts',(11.1355411536237,-20.7846788186803,1.82618123095095));
#86093=CARTESIAN_POINT('Ctrl Pts',(11.1385469425801,-20.7855442815937,1.82537246668409));
#86094=CARTESIAN_POINT('Ctrl Pts',(11.1414081485161,-20.7864153809969,1.82460200663818));
#86095=CARTESIAN_POINT('Ctrl Pts',(11.1428387514841,-20.7868509306985,1.82421677661523));
#86096=CARTESIAN_POINT('Ctrl Pts',(11.1437160692069,-20.7871263827825,1.82398021955917));
#86097=CARTESIAN_POINT('Ctrl Pts',(11.1448178401921,-20.7874771225719,1.8236833995488));
#86098=CARTESIAN_POINT('Ctrl Pts',(11.1457920700905,-20.7877872606986,1.82342093944374));
#86099=CARTESIAN_POINT('Ctrl Pts',(11.1469421037944,-20.7881554945431,1.82311127916004));
#86100=CARTESIAN_POINT('Ctrl Pts',(11.1487960782264,-20.7887760313561,1.82261250308688));
#86101=CARTESIAN_POINT('Ctrl Pts',(11.14903879087,-20.7888572687927,1.82254720593001));
#86102=CARTESIAN_POINT('Ctrl Pts',(11.1492935454941,-20.788942900769,1.82247867357926));
#86103=CARTESIAN_POINT('Ctrl Pts',(11.1495615021919,-20.7890334389009,1.82240659421726));
#86104=CARTESIAN_POINT('Ctrl Pts',(11.1563279211354,-20.7913196998364,1.82058645251367));
#86105=CARTESIAN_POINT('Ctrl Pts',(11.1625769168139,-20.7937252051572,1.81886794431943));
#86106=CARTESIAN_POINT('Ctrl Pts',(11.1680845579708,-20.7960314016393,1.81734032689293));
#86107=CARTESIAN_POINT('Ctrl Pts',(11.1757232918988,-20.7992299435943,1.8152216225815));
#86108=CARTESIAN_POINT('Ctrl Pts',(11.1819360774177,-20.8022315964258,1.81347008282657));
#86109=CARTESIAN_POINT('Ctrl Pts',(11.186205818646,-20.8043814218725,1.81230297902011));
#86110=CARTESIAN_POINT('Ctrl Pts',(11.1872827793046,-20.8049236742727,1.81200859938046));
#86111=CARTESIAN_POINT('Ctrl Pts',(11.1882363244331,-20.8054118612248,1.81175134962557));
#86112=CARTESIAN_POINT('Ctrl Pts',(11.1890582182961,-20.8058362808762,1.8115347011105));
#86113=CARTESIAN_POINT('Ctrl Pts',(11.191620679814,-20.8071595162392,1.81085924469486));
#86114=CARTESIAN_POINT('Ctrl Pts',(11.1950125808572,-20.8089466794886,1.81003220731266));
#86115=CARTESIAN_POINT('Ctrl Pts',(11.1991539097921,-20.8112879294087,1.80901917411934));
#86116=CARTESIAN_POINT('Ctrl Pts',(11.2002083640929,-20.8118840523168,1.80876123826724));
#86117=CARTESIAN_POINT('Ctrl Pts',(11.2013112466889,-20.8125163047139,1.80849128555073));
#86118=CARTESIAN_POINT('Ctrl Pts',(11.2024608971286,-20.8131865820199,1.80820883669898));
#86119=CARTESIAN_POINT('Ctrl Pts',(11.2052933264132,-20.814837964914,1.80751295874215));
#86120=CARTESIAN_POINT('Ctrl Pts',(11.208409451306,-20.8167196829706,1.80674007759016));
#86121=CARTESIAN_POINT('Ctrl Pts',(11.2117758887729,-20.8188620521781,1.80587689222197));
#86122=CARTESIAN_POINT('Ctrl Pts',(11.2135389634822,-20.8199840563754,1.805424823735));
#86123=CARTESIAN_POINT('Ctrl Pts',(11.2156745716249,-20.8213772323699,1.80486375185293));
#86124=CARTESIAN_POINT('Ctrl Pts',(11.217695862772,-20.8227376815279,1.80432438855134));
#86125=CARTESIAN_POINT('Ctrl Pts',(11.2195340508706,-20.8239748914441,1.80383388464586));
#86126=CARTESIAN_POINT('Ctrl Pts',(11.221278205261,-20.8251839540792,1.8033611982393));
#86127=CARTESIAN_POINT('Ctrl Pts',(11.2225827407332,-20.8261038737532,1.80299917840933));
#86128=CARTESIAN_POINT('Ctrl Pts',(11.2311650483049,-20.8321558621824,1.80061751413563));
#86129=CARTESIAN_POINT('Ctrl Pts',(11.2388722047358,-20.8382890404485,1.79847325067937));
#86130=CARTESIAN_POINT('Ctrl Pts',(11.2458190592394,-20.8443217970411,1.79659127395651));
#86131=CARTESIAN_POINT('Ctrl Pts',(11.2477404719851,-20.8459903817801,1.79607074282109));
#86132=CARTESIAN_POINT('Ctrl Pts',(11.2496037920806,-20.8476515874104,1.79557025959013));
#86133=CARTESIAN_POINT('Ctrl Pts',(11.2514115713214,-20.8493022441783,1.79509032176336));
#86134=CARTESIAN_POINT('Ctrl Pts',(11.2555834676177,-20.8531115416307,1.79398274690199));
#86135=CARTESIAN_POINT('Ctrl Pts',(11.2594601534398,-20.856864462399,1.79298521059919));
#86136=CARTESIAN_POINT('Ctrl Pts',(11.2630756862055,-20.8605294332295,1.79210639261045));
#86137=CARTESIAN_POINT('Ctrl Pts',(11.2647550735698,-20.8622317841974,1.79169818836465));
#86138=CARTESIAN_POINT('Ctrl Pts',(11.2668542955939,-20.8644074833757,1.79118402619731));
#86139=CARTESIAN_POINT('Ctrl Pts',(11.2689933712148,-20.8667099173455,1.79064579654053));
#86140=CARTESIAN_POINT('Ctrl Pts',(11.2710430014965,-20.868916075155,1.79013007292968));
#86141=CARTESIAN_POINT('Ctrl Pts',(11.2731287735226,-20.8712386651904,1.78959237040092));
#86142=CARTESIAN_POINT('Ctrl Pts',(11.2749530779121,-20.8733356323948,1.78909495732801));
#86143=CARTESIAN_POINT('Ctrl Pts',(11.2753237759261,-20.8737617353974,1.78899388316553));
#86144=CARTESIAN_POINT('Ctrl Pts',(11.2756838044323,-20.8741784050093,1.78889443889188));
#86145=CARTESIAN_POINT('Ctrl Pts',(11.2760308487974,-20.8745826066336,1.78879709845521));
#86146=CARTESIAN_POINT('Ctrl Pts',(11.2786809486211,-20.8776691706615,1.78805378751286));
#86147=CARTESIAN_POINT('Ctrl Pts',(11.280819351248,-20.8802900091605,1.78742118467707));
#86148=CARTESIAN_POINT('Ctrl Pts',(11.2826709372862,-20.8826174977141,1.78686578086445));
#86149=CARTESIAN_POINT('Ctrl Pts',(11.2847855319977,-20.8852755945482,1.78623148467696));
#86150=CARTESIAN_POINT('Ctrl Pts',(11.2865255819466,-20.8875519570998,1.78569800051693));
#86151=CARTESIAN_POINT('Ctrl Pts',(11.2881757877891,-20.8897516108374,1.78522881404554));
#86152=CARTESIAN_POINT('Ctrl Pts',(11.2892652516828,-20.8912038195644,1.78491905770677));
#86153=CARTESIAN_POINT('Ctrl Pts',(11.2903146411927,-20.8926234410485,1.78463756969843));
#86154=CARTESIAN_POINT('Ctrl Pts',(11.2913968729573,-20.8941058380151,1.78437624402163));
#86155=CARTESIAN_POINT('Ctrl Pts',(11.2934752969568,-20.896952778507,1.78387436856746));
#86156=CARTESIAN_POINT('Ctrl Pts',(11.2959003782589,-20.9003586644651,1.78334317638522));
#86157=CARTESIAN_POINT('Ctrl Pts',(11.2985721795118,-20.9043476305441,1.78272589006414));
#86158=CARTESIAN_POINT('Ctrl Pts',(11.2997437831322,-20.9060968201946,1.78245520567554));
#86159=CARTESIAN_POINT('Ctrl Pts',(11.3011892265232,-20.9083082281453,1.78210362596708));
#86160=CARTESIAN_POINT('Ctrl Pts',(11.3025914362365,-20.9105281754296,1.78175149746585));
#86161=CARTESIAN_POINT('Ctrl Pts',(11.3040652188877,-20.9128614353999,1.78138139528274));
#86162=CARTESIAN_POINT('Ctrl Pts',(11.3054908542077,-20.9152040706641,1.78101078849584));
#86163=CARTESIAN_POINT('Ctrl Pts',(11.3065530473484,-20.9169938461998,1.78071892298188));
#86164=CARTESIAN_POINT('Ctrl Pts',(11.3067849034257,-20.9173845193448,1.78065521442402));
#86165=CARTESIAN_POINT('Ctrl Pts',(11.3069996179879,-20.917748743027,1.78059521109814));
#86166=CARTESIAN_POINT('Ctrl Pts',(11.307194142963,-20.9180805322724,1.78053967587823));
#86167=CARTESIAN_POINT('Ctrl Pts',(11.3144962577439,-20.930535298823,1.77845498443932));
#86168=CARTESIAN_POINT('Ctrl Pts',(11.3208213488539,-20.9432998130216,1.77679228846964));
#86169=CARTESIAN_POINT('Ctrl Pts',(11.3262029546748,-20.9562949396764,1.77540952966746));
#86170=CARTESIAN_POINT('Ctrl Pts',(11.3265215026431,-20.9570641471085,1.7753276814196));
#86171=CARTESIAN_POINT('Ctrl Pts',(11.3268367370717,-20.9578341751543,1.77524681580918));
#86172=CARTESIAN_POINT('Ctrl Pts',(11.3271486618196,-20.958605011926,1.77516690410521));
#86173=CARTESIAN_POINT('Ctrl Pts',(11.3290483249791,-20.9632995102861,1.77468023121025));
#86174=CARTESIAN_POINT('Ctrl Pts',(11.3309150432156,-20.9682576704015,1.77420483690388));
#86175=CARTESIAN_POINT('Ctrl Pts',(11.3326433989493,-20.9732472551659,1.77376348769531));
#86176=CARTESIAN_POINT('Ctrl Pts',(11.334434517243,-20.9784180289684,1.7733061115742));
#86177=CARTESIAN_POINT('Ctrl Pts',(11.3360766368962,-20.9836221559145,1.77288540523271));
#86178=CARTESIAN_POINT('Ctrl Pts',(11.337506302503,-20.9885816823008,1.77251239450797));
#86179=CARTESIAN_POINT('Ctrl Pts',(11.3387505506701,-20.9928979934623,1.77218776061571));
#86180=CARTESIAN_POINT('Ctrl Pts',(11.3398351802698,-20.9970284406791,1.77189890714644));
#86181=CARTESIAN_POINT('Ctrl Pts',(11.3407487906881,-21.0007831501905,1.77164502091652));
#86182=CARTESIAN_POINT('Ctrl Pts',(11.3431127849098,-21.0104985731009,1.77098808272004));
#86183=CARTESIAN_POINT('Ctrl Pts',(11.3449694913004,-21.0201442238305,1.77048932883145));
#86184=CARTESIAN_POINT('Ctrl Pts',(11.3463686089709,-21.0298042582066,1.77012153108541));
#86185=CARTESIAN_POINT('Ctrl Pts',(11.3477748237025,-21.03951329336,1.76975186767566));
#86186=CARTESIAN_POINT('Ctrl Pts',(11.3487188980331,-21.0492377497457,1.76951446321259));
#86187=CARTESIAN_POINT('Ctrl Pts',(11.3492020949561,-21.0590740018403,1.76939470728942));
#86188=CARTESIAN_POINT('Ctrl Pts',(11.3494487174911,-21.0640944010007,1.76933358415731));
#86189=CARTESIAN_POINT('Ctrl Pts',(11.3495744826921,-21.0691440165458,1.76930332025556));
#86190=CARTESIAN_POINT('Ctrl Pts',(11.3495744826921,-21.0742356128,1.76930332025556));
#86191=CARTESIAN_POINT('Origin',(-2.84607155346,-20.7742356128,5.53854202767));
#86192=CARTESIAN_POINT('Origin',(7.85893479754359,-21.0742356128,-4.07415000216138));
#86193=CARTESIAN_POINT('Origin',(7.85893479751,-21.0742356128,-4.07415000213));
#86194=CARTESIAN_POINT('Origin',(7.85893479751,-21.0742356128,-4.07415000213));
#86195=CARTESIAN_POINT('Origin',(7.86219292935,-23.1742356128,-4.51414908377));
#86196=CARTESIAN_POINT('',(7.64099403241,-22.8742356128,-4.28030970457));
#86197=CARTESIAN_POINT('',(5.92940140951,-22.8742356128,-2.47090756951));
#86198=CARTESIAN_POINT('',(6.88866980649,-22.8742356128,-3.48499366825));
#86199=CARTESIAN_POINT('',(7.64099403241,-22.1242356128,-4.28030970457));
#86200=CARTESIAN_POINT('',(5.92940140951,-22.1242356128,-2.47090756951));
#86201=CARTESIAN_POINT('Origin',(6.1473421746,-21.0742356128,-2.26474786707));
#86202=CARTESIAN_POINT('Origin',(6.1473421746,-21.0742356128,-2.26474786707));
#86203=CARTESIAN_POINT('Origin',(0.00234331738835,-21.2742356128,3.08191746407));
#86204=CARTESIAN_POINT('',(5.92101866809,-22.8742356128,-2.06782739988));
#86205=CARTESIAN_POINT('',(7.75696851341,-22.8742356128,1.89180060423));
#86206=CARTESIAN_POINT('Origin',(0.00234331738837,-22.8742356128,3.08191746407));
#86207=CARTESIAN_POINT('',(5.92101866809,-22.1242356128,-2.06782739988));
#86208=CARTESIAN_POINT('',(7.75696851341,-22.1242356128,1.89180060423));
#86209=CARTESIAN_POINT('Origin',(8.05349668264,-21.0742356128,1.84629187045));
#86210=CARTESIAN_POINT('Origin',(8.05349668264,-21.0742356128,1.84629187045));
#86211=CARTESIAN_POINT('Origin',(-11.4443506127,-23.1742356128,2.14629187045));
#86212=CARTESIAN_POINT('',(8.05349668264,-22.8742356128,2.14629187045));
#86213=CARTESIAN_POINT('',(8.05349668264,-22.1242356128,2.14629187045));
#86214=CARTESIAN_POINT('',(11.0596214465,-22.8742356128,2.14629187045));
#86215=CARTESIAN_POINT('',(11.0596214465,-22.1242356128,2.14629187045));
#86216=CARTESIAN_POINT('',(-6.6707290414,-22.8742356128,2.14629187045));
#86217=CARTESIAN_POINT('Origin',(11.0596214465,-21.0742356128,1.84629187045));
#86218=CARTESIAN_POINT('Origin',(11.0596214465,-21.0742356128,1.84629187045));
#86219=CARTESIAN_POINT('Origin',(-2.84607155346,-21.2742356128,5.53854202767));
#86220=CARTESIAN_POINT('',(11.3495744826,-22.8742356128,1.76930332028));
#86221=CARTESIAN_POINT('',(11.3495744826,-22.1242356128,1.76930332028));
#86222=CARTESIAN_POINT('',(8.08214906615,-22.8742356128,-4.27458799822));
#86223=CARTESIAN_POINT('',(8.08214906615,-22.1242356128,-4.27458799822));
#86224=CARTESIAN_POINT('Origin',(-2.84607155346,-22.8742356128,5.53854202767));
#86225=CARTESIAN_POINT('Origin',(7.85893479751,-22.1242356128,-4.07415000213));
#86226=CARTESIAN_POINT('Origin',(7.85893479751,-22.8742356128,-4.07415000213));
#86227=CARTESIAN_POINT('Origin',(6.6707290414,-22.8742356128,-3.69115337069));
#86228=CARTESIAN_POINT('',(5.71146064442,-23.1742356128,-2.67706727196));
#86229=CARTESIAN_POINT('Origin',(5.71146064442,-22.8742356128,-2.67706727196));
#86230=CARTESIAN_POINT('',(7.42305326732,-23.1742356128,-4.48646940701));
#86231=CARTESIAN_POINT('',(6.56725695587,-23.1742356128,-3.58176833949));
#86232=CARTESIAN_POINT('Origin',(7.42305326732,-22.8742356128,-4.48646940701));
#86233=CARTESIAN_POINT('Origin',(6.1473421746,-22.1242356128,-2.26474786707));
#86234=CARTESIAN_POINT('Origin',(6.1473421746,-22.8742356128,-2.26474786707));
#86235=CARTESIAN_POINT('Origin',(0.00234331738837,-22.8742356128,3.08191746407));
#86236=CARTESIAN_POINT('',(7.46044034417,-23.1742356128,1.93730933801));
#86237=CARTESIAN_POINT('Origin',(7.46044034417,-22.8742356128,1.93730933801));
#86238=CARTESIAN_POINT('',(5.69469516158,-23.1742356128,-1.87090693268));
#86239=CARTESIAN_POINT('Origin',(0.00234331738835,-23.1742356128,3.08191746407));
#86240=CARTESIAN_POINT('Origin',(5.69469516158,-22.8742356128,-1.87090693268));
#86241=CARTESIAN_POINT('Origin',(8.05349668264,-22.1242356128,1.84629187045));
#86242=CARTESIAN_POINT('Origin',(8.05349668264,-22.8742356128,1.84629187045));
#86243=CARTESIAN_POINT('Origin',(-6.6707290414,-22.8742356128,2.44629187045));
#86244=CARTESIAN_POINT('',(11.0596214465,-23.1742356128,2.44629187045));
#86245=CARTESIAN_POINT('Origin',(11.0596214465,-22.8742356128,2.44629187045));
#86246=CARTESIAN_POINT('',(8.05349668264,-23.1742356128,2.44629187045));
#86247=CARTESIAN_POINT('',(9.55655906459,-23.1742356128,2.44629187045));
#86248=CARTESIAN_POINT('Origin',(8.05349668264,-22.8742356128,2.44629187045));
#86249=CARTESIAN_POINT('Origin',(11.0596214465,-22.1242356128,1.84629187045));
#86250=CARTESIAN_POINT('Origin',(11.0596214465,-22.8742356128,1.84629187045));
#86251=CARTESIAN_POINT('Origin',(-2.84607155346,-22.8742356128,5.53854202767));
#86252=CARTESIAN_POINT('',(8.30536333479,-23.1742356128,-4.4750259943));
#86253=CARTESIAN_POINT('Origin',(8.30536333479,-22.8742356128,-4.4750259943));
#86254=CARTESIAN_POINT('',(11.6395275187,-23.1742356128,1.69231477012));
#86255=CARTESIAN_POINT('Origin',(-2.84607155346,-23.1742356128,5.53854202767));
#86256=CARTESIAN_POINT('Origin',(11.6395275187,-22.8742356128,1.69231477012));
#86257=CARTESIAN_POINT('Origin',(7.85893479751,-22.8742356128,-4.07415000213));
#86258=CARTESIAN_POINT('Origin',(7.85893479751,-23.1742356128,-4.07415000213));
#86259=CARTESIAN_POINT('Origin',(3.41821282746,-21.0742356128,8.06979469543));
#86260=CARTESIAN_POINT('',(3.62188020465,-21.0742356128,7.84952304616));
#86261=CARTESIAN_POINT('',(3.58772315463,-21.0742356128,8.31731489457));
#86262=CARTESIAN_POINT('Origin',(3.41821282746,-21.0742356128,8.06979469543));
#86263=CARTESIAN_POINT('',(3.41821282746,-20.7742356128,8.06979469543));
#86264=CARTESIAN_POINT('Origin',(3.41821282746,-21.0742356128,8.06979469543));
#86265=CARTESIAN_POINT('Origin',(3.41821282746,-21.0742356128,8.06979469543));
#86266=CARTESIAN_POINT('Origin',(6.1473421746,-22.8742356128,-2.26474786707));
#86267=CARTESIAN_POINT('Origin',(6.1473421746,-23.1742356128,-2.26474786707));
#86268=CARTESIAN_POINT('Origin',(8.05349668264,-22.8742356128,1.84629187045));
#86269=CARTESIAN_POINT('Origin',(8.05349668264,-23.1742356128,1.84629187045));
#86270=CARTESIAN_POINT('Origin',(11.0596214465,-22.8742356128,1.84629187045));
#86271=CARTESIAN_POINT('Origin',(11.0596214465,-23.1742356128,1.84629187045));
#86272=CARTESIAN_POINT('Origin',(-2.84607155346,-22.8742356128,5.53854202767));
#86273=CARTESIAN_POINT('',(0.246934184019208,-22.8742356128,-6.59919549797773));
#86274=CARTESIAN_POINT('',(2.37995077076E-13,-23.1742356128,-6.35119542306));
#86275=CARTESIAN_POINT('Ctrl Pts',(0.246934184763,-22.8742356128,-6.59919549778));
#86276=CARTESIAN_POINT('Ctrl Pts',(0.247420066333,-22.976056074,-6.59957097409));
#86277=CARTESIAN_POINT('Ctrl Pts',(0.206909891011,-23.0789305063,-6.56242231995));
#86278=CARTESIAN_POINT('Ctrl Pts',(0.139040717811,-23.1404071843,-6.49840377124));
#86279=CARTESIAN_POINT('Ctrl Pts',(0.0693760469986,-23.1744148412,-6.42641803012));
#86280=CARTESIAN_POINT('Ctrl Pts',(2.37995077076E-13,-23.1742356128,-6.35119542306));
#86281=CARTESIAN_POINT('',(0.530881036642,-22.8742356128,-6.52327988851));
#86282=CARTESIAN_POINT('Origin',(-2.84607155346,-22.8742356128,5.53854202767));
#86283=CARTESIAN_POINT('',(0.45,-23.1742356128,-6.23438845923));
#86284=CARTESIAN_POINT('Origin',(0.45,-22.8742356128,-6.23438845923));
#86285=CARTESIAN_POINT('Origin',(-2.84607155346,-23.1742356128,5.53854202767));
#86286=CARTESIAN_POINT('Origin',(2.93915231795E-16,-20.7742356128,0.729452270839));
#86287=CARTESIAN_POINT('Ctrl Pts',(3.39394702409,-22.8742356071,-7.27665075406));
#86288=CARTESIAN_POINT('Ctrl Pts',(3.3939470242,-22.8742356096,-7.39921133184));
#86289=CARTESIAN_POINT('Ctrl Pts',(3.45653492108,-22.8742356121,-7.52177190961));
#86290=CARTESIAN_POINT('Ctrl Pts',(3.58353228733,-22.8742356136,-7.59954001295));
#86291=CARTESIAN_POINT('Ctrl Pts',(3.72114892405,-22.8742356136,-7.59957667728));
#86292=CARTESIAN_POINT('Ctrl Pts',(3.83031550589,-22.8742356125,-7.54386534431));
#86293=CARTESIAN_POINT('Ctrl Pts',(3.39394702409,-22.9689887672,-7.27665074537));
#86294=CARTESIAN_POINT('Ctrl Pts',(3.3939470273,-22.9472590608,-7.39921132275));
#86295=CARTESIAN_POINT('Ctrl Pts',(3.45653492596,-22.9255293543,-7.52177190012));
#86296=CARTESIAN_POINT('Ctrl Pts',(3.5835322914,-22.9117412055,-7.59954000419));
#86297=CARTESIAN_POINT('Ctrl Pts',(3.72114892639,-22.9117347492,-7.59957667094));
#86298=CARTESIAN_POINT('Ctrl Pts',(3.83031550688,-22.9216122395,-7.54386534051));
#86299=CARTESIAN_POINT('Ctrl Pts',(3.39394702409,-23.0638368546,-7.29765903263));
#86300=CARTESIAN_POINT('Ctrl Pts',(3.39394703709,-23.0202773024,-7.41438252872));
#86301=CARTESIAN_POINT('Ctrl Pts',(3.45551763217,-22.9767177502,-7.53110602482));
#86302=CARTESIAN_POINT('Ctrl Pts',(3.58040884259,-22.9491120295,-7.6059738358));
#86303=CARTESIAN_POINT('Ctrl Pts',(3.71667793436,-22.9491723593,-7.60786209828));
#86304=CARTESIAN_POINT('Ctrl Pts',(3.82588511173,-22.969036255,-7.55663051616));
#86305=CARTESIAN_POINT('Ctrl Pts',(3.39394702409,-23.1509380315,-7.33965594802));
#86306=CARTESIAN_POINT('Ctrl Pts',(3.39394697957,-23.0896047046,-7.44484208723));
#86307=CARTESIAN_POINT('Ctrl Pts',(3.45348987378,-23.0282713776,-7.55002822643));
#86308=CARTESIAN_POINT('Ctrl Pts',(3.57418338496,-22.9885124598,-7.61911093785));
#86309=CARTESIAN_POINT('Ctrl Pts',(3.70775302124,-22.9865706365,-7.62456986686));
#86310=CARTESIAN_POINT('Ctrl Pts',(3.81702777332,-23.0125868459,-7.58214937101));
#86311=CARTESIAN_POINT('Ctrl Pts',(3.39394702409,-23.3144960216,-7.46222952989));
#86312=CARTESIAN_POINT('Ctrl Pts',(3.39394707642,-23.2249734796,-7.53850326899));
#86313=CARTESIAN_POINT('Ctrl Pts',(3.4480237922,-23.1354509376,-7.6147770081));
#86314=CARTESIAN_POINT('Ctrl Pts',(3.55743149517,-23.0743105508,-7.66795137089));
#86315=CARTESIAN_POINT('Ctrl Pts',(3.68302539363,-23.0640733183,-7.67932532721));
#86316=CARTESIAN_POINT('Ctrl Pts',(3.79142259861,-23.0943657893,-7.65641303197));
#86317=CARTESIAN_POINT('Ctrl Pts',(3.39394702409,-23.4183511293,-7.6347947685));
#86318=CARTESIAN_POINT('Ctrl Pts',(3.39394696259,-23.319135779,-7.67899068739));
#86319=CARTESIAN_POINT('Ctrl Pts',(3.44128745287,-23.2199204287,-7.72318660628));
#86320=CARTESIAN_POINT('Ctrl Pts',(3.53685705407,-23.1477285443,-7.75602607095));
#86321=CARTESIAN_POINT('Ctrl Pts',(3.65117651028,-23.1252941134,-7.76773938497));
#86322=CARTESIAN_POINT('Ctrl Pts',(3.75606800489,-23.1462934039,-7.76036589659));
#86323=CARTESIAN_POINT('Ctrl Pts',(3.39394702409,-23.4554260016,-7.73594528854));
#86324=CARTESIAN_POINT('Ctrl Pts',(3.39394732526,-23.3552502828,-7.7641726908));
#86325=CARTESIAN_POINT('Ctrl Pts',(3.43768548772,-23.255074564,-7.79240009306));
#86326=CARTESIAN_POINT('Ctrl Pts',(3.52588291425,-23.1798234897,-7.81406109398));
#86327=CARTESIAN_POINT('Ctrl Pts',(3.63360843235,-23.151042617,-7.82338875536));
#86328=CARTESIAN_POINT('Ctrl Pts',(3.73562880641,-23.1648309328,-7.82105608415));
#86329=CARTESIAN_POINT('Ctrl Pts',(3.39394702409,-23.4742356128,-7.84128512581));
#86330=CARTESIAN_POINT('Ctrl Pts',(3.39394702409,-23.3758453918,-7.85470223468));
#86331=CARTESIAN_POINT('Ctrl Pts',(3.43421150493,-23.2774551707,-7.86811934354));
#86332=CARTESIAN_POINT('Ctrl Pts',(3.51532352314,-23.2014862199,-7.87872422454));
#86333=CARTESIAN_POINT('Ctrl Pts',(3.61626901029,-23.167728681,-7.88399310977));
#86334=CARTESIAN_POINT('Ctrl Pts',(3.71465923135,-23.1742356128,-7.88399310977));
#86335=CARTESIAN_POINT('Ctrl Pts',(3.39394702409,-23.4742356128,-7.94679080481));
#86336=CARTESIAN_POINT('Ctrl Pts',(3.39394702409,-23.3799878332,-7.94679080481));
#86337=CARTESIAN_POINT('Ctrl Pts',(3.4309580406,-23.2857400536,-7.94679080481));
#86338=CARTESIAN_POINT('Ctrl Pts',(3.50545146488,-23.2112466293,-7.94679080481));
#86339=CARTESIAN_POINT('Ctrl Pts',(3.59969924449,-23.1742356128,-7.94679080481));
#86340=CARTESIAN_POINT('Ctrl Pts',(3.69394702409,-23.1742356128,-7.94679080481));
#86341=CARTESIAN_POINT('',(3.8303155059,-22.8742356128,-7.54386534442));
#86342=CARTESIAN_POINT('Ctrl Pts',(3.8303155059,-22.8742356128,-7.54386534442));
#86343=CARTESIAN_POINT('Ctrl Pts',(3.72114892405,-22.8742356145701,-7.59957667728));
#86344=CARTESIAN_POINT('Ctrl Pts',(3.58353228733,-22.8742356145703,-7.59954001295));
#86345=CARTESIAN_POINT('Ctrl Pts',(3.45653492108,-22.874235613427,-7.52177190961));
#86346=CARTESIAN_POINT('Ctrl Pts',(3.3939470242,-22.8742356114892,-7.39921133184));
#86347=CARTESIAN_POINT('Ctrl Pts',(3.39394702409,-22.8742356071,-7.27665075406));
#86348=CARTESIAN_POINT('',(3.69394702409,-23.1742356128,-7.94679080481));
#86349=CARTESIAN_POINT('Origin',(3.69182568282636,-23.4721142715478,-7.94679080481));
#86350=CARTESIAN_POINT('Ctrl Pts',(3.8303155058534,-22.8742356128,-7.54386534432868));
#86351=CARTESIAN_POINT('Ctrl Pts',(3.83031550576691,-22.8891836981438,-7.54386534335005));
#86352=CARTESIAN_POINT('Ctrl Pts',(3.82971372840363,-22.9043888182403,-7.54543077875052));
#86353=CARTESIAN_POINT('Ctrl Pts',(3.82852226081592,-22.9196429501145,-7.54866017859));
#86354=CARTESIAN_POINT('Ctrl Pts',(3.82728294903626,-22.9355096220367,-7.5520192571781));
#86355=CARTESIAN_POINT('Ctrl Pts',(3.8254052437601,-22.9514301757083,-7.55717821794454));
#86356=CARTESIAN_POINT('Ctrl Pts',(3.82292523898896,-22.9671744194393,-7.56419691331168));
#86357=CARTESIAN_POINT('Ctrl Pts',(3.821706622318,-22.9749107746696,-7.56764573699232));
#86358=CARTESIAN_POINT('Ctrl Pts',(3.82034295925121,-22.982604531287,-7.57154287310375));
#86359=CARTESIAN_POINT('Ctrl Pts',(3.81884079211807,-22.9902275607281,-7.5758915167602));
#86360=CARTESIAN_POINT('Ctrl Pts',(3.81607775040317,-23.0042491352088,-7.58389028304987));
#86361=CARTESIAN_POINT('Ctrl Pts',(3.8128308557735,-23.0180209455026,-7.59342190599612));
#86362=CARTESIAN_POINT('Ctrl Pts',(3.80908417075911,-23.031335083101,-7.60449227138444));
#86363=CARTESIAN_POINT('Ctrl Pts',(3.80774703235729,-23.0360867087652,-7.60844312677423));
#86364=CARTESIAN_POINT('Ctrl Pts',(3.80634639550617,-23.0407798967205,-7.61258949584727));
#86365=CARTESIAN_POINT('Ctrl Pts',(3.80488200217345,-23.0454049053476,-7.61693019755438));
#86366=CARTESIAN_POINT('Ctrl Pts',(3.80209817773717,-23.0541970868923,-7.62518190917649));
#86367=CARTESIAN_POINT('Ctrl Pts',(3.79908193039014,-23.0627426525445,-7.63413739357837));
#86368=CARTESIAN_POINT('Ctrl Pts',(3.79582238365986,-23.0709722301392,-7.64378448429961));
#86369=CARTESIAN_POINT('Ctrl Pts',(3.79441196867438,-23.0745331913784,-7.64795880743269));
#86370=CARTESIAN_POINT('Ctrl Pts',(3.79294260755751,-23.0780316640683,-7.65226591558948));
#86371=CARTESIAN_POINT('Ctrl Pts',(3.79142613720875,-23.0814652617517,-7.65670050231454));
#86372=CARTESIAN_POINT('Ctrl Pts',(3.79119028429884,-23.0819992807688,-7.65739020269952));
#86373=CARTESIAN_POINT('Ctrl Pts',(3.79095329160658,-23.082531731389,-7.65808298900307));
#86374=CARTESIAN_POINT('Ctrl Pts',(3.79071520419736,-23.0830626037977,-7.65877884160525));
#86375=CARTESIAN_POINT('Ctrl Pts',(3.78990694113206,-23.0848648182104,-7.66114113350075));
#86376=CARTESIAN_POINT('Ctrl Pts',(3.78898629334184,-23.086868580809,-7.66383305214407));
#86377=CARTESIAN_POINT('Ctrl Pts',(3.78808966118208,-23.0887663855061,-7.6664561297899));
#86378=CARTESIAN_POINT('Ctrl Pts',(3.78710763895836,-23.0908449261523,-7.66932901418814));
#86379=CARTESIAN_POINT('Ctrl Pts',(3.78615456208163,-23.0927963606278,-7.67211893756012));
#86380=CARTESIAN_POINT('Ctrl Pts',(3.78542392434147,-23.0942650558611,-7.67425848985647));
#86381=CARTESIAN_POINT('Ctrl Pts',(3.78536167208538,-23.0943901925558,-7.67444078533636));
#86382=CARTESIAN_POINT('Ctrl Pts',(3.78530104061487,-23.0945118473466,-7.67461834086054));
#86383=CARTESIAN_POINT('Ctrl Pts',(3.78524215234058,-23.0946298108357,-7.67479079697391));
#86384=CARTESIAN_POINT('Ctrl Pts',(3.7815169251505,-23.1020920909291,-7.68570023880042));
#86385=CARTESIAN_POINT('Ctrl Pts',(3.77739994333826,-23.109525749538,-7.69775930932877));
#86386=CARTESIAN_POINT('Ctrl Pts',(3.772875551567,-23.1167109360701,-7.71103970318222));
#86387=CARTESIAN_POINT('Ctrl Pts',(3.77069040030985,-23.1201811747624,-7.71745375191882));
#86388=CARTESIAN_POINT('Ctrl Pts',(3.76841042757223,-23.1235929863598,-7.72415214818587));
#86389=CARTESIAN_POINT('Ctrl Pts',(3.76603516262184,-23.1269190542052,-7.73113960412645));
#86390=CARTESIAN_POINT('Ctrl Pts',(3.76238851748999,-23.1320254273341,-7.74186715356705));
#86391=CARTESIAN_POINT('Ctrl Pts',(3.75852730260589,-23.1369322492204,-7.75327548212248));
#86392=CARTESIAN_POINT('Ctrl Pts',(3.75444904890525,-23.1415316798466,-7.76537128242619));
#86393=CARTESIAN_POINT('Ctrl Pts',(3.75240992205494,-23.1438313951596,-7.77141918257805));
#86394=CARTESIAN_POINT('Ctrl Pts',(3.75031641641447,-23.1460540871329,-7.77763873481617));
#86395=CARTESIAN_POINT('Ctrl Pts',(3.74816743160474,-23.1481853204141,-7.78402931127238));
#86396=CARTESIAN_POINT('Ctrl Pts',(3.74709293919988,-23.1492509370547,-7.78722459950048));
#86397=CARTESIAN_POINT('Ctrl Pts',(3.74600457707861,-23.1502936881539,-7.79046264393566));
#86398=CARTESIAN_POINT('Ctrl Pts',(3.74490214245977,-23.1513117086285,-7.79374324293244));
#86399=CARTESIAN_POINT('Ctrl Pts',(3.74435092515035,-23.1518207188659,-7.79538354243082));
#86400=CARTESIAN_POINT('Ctrl Pts',(3.74379618970325,-23.1523235465235,-7.79703448054263));
#86401=CARTESIAN_POINT('Ctrl Pts',(3.74323790853073,-23.1528199569261,-7.79869602771192));
#86402=CARTESIAN_POINT('Ctrl Pts',(3.74281599488497,-23.153195112552,-7.79995172010905));
#86403=CARTESIAN_POINT('Ctrl Pts',(3.7421707340011,-23.1537585415559,-7.80187200933954));
#86404=CARTESIAN_POINT('Ctrl Pts',(3.74180381131037,-23.154074114798,-7.80296414761389));
#86405=CARTESIAN_POINT('Ctrl Pts',(3.74168521751671,-23.1541761118369,-7.8033171397412));
#86406=CARTESIAN_POINT('Ctrl Pts',(3.74159574384263,-23.1542526471401,-7.80358346296994));
#86407=CARTESIAN_POINT('Ctrl Pts',(3.74155239904321,-23.1542897009319,-7.80371246452033));
#86408=CARTESIAN_POINT('Ctrl Pts',(3.7404152624986,-23.1552617949622,-7.80709677772983));
#86409=CARTESIAN_POINT('Ctrl Pts',(3.73888225575716,-23.1565394420993,-7.81166442353252));
#86410=CARTESIAN_POINT('Ctrl Pts',(3.73694415193971,-23.158023736641,-7.81744798511014));
#86411=CARTESIAN_POINT('Ctrl Pts',(3.73500913445982,-23.1595056675146,-7.82322233664276));
#86412=CARTESIAN_POINT('Ctrl Pts',(3.73267003716621,-23.1611935991109,-7.83020952169269));
#86413=CARTESIAN_POINT('Ctrl Pts',(3.72991761188174,-23.1629377834524,-7.83844583282956));
#86414=CARTESIAN_POINT('Ctrl Pts',(3.72723730229835,-23.1646362687963,-7.84646634615521));
#86415=CARTESIAN_POINT('Ctrl Pts',(3.72416473685366,-23.1663879276109,-7.85567229785107));
#86416=CARTESIAN_POINT('Ctrl Pts',(3.72069556429772,-23.1680073125115,-7.86608830518644));
#86417=CARTESIAN_POINT('Ctrl Pts',(3.71735496001881,-23.1695666826613,-7.87611829306183));
#86418=CARTESIAN_POINT('Ctrl Pts',(3.71364632450648,-23.1710032445205,-7.88727117149701));
#86419=CARTESIAN_POINT('Ctrl Pts',(3.70957386674216,-23.1721096345942,-7.89954781998661));
#86420=CARTESIAN_POINT('Ctrl Pts',(3.705781791046,-23.1731398515176,-7.91097924127122));
#86421=CARTESIAN_POINT('Ctrl Pts',(3.70167409659488,-23.1738836084695,-7.92338559552355));
#86422=CARTESIAN_POINT('Ctrl Pts',(3.69726432338169,-23.1741393298497,-7.93673921986036));
#86423=CARTESIAN_POINT('Ctrl Pts',(3.69617676356291,-23.1742023971062,-7.94003255594855));
#86424=CARTESIAN_POINT('Ctrl Pts',(3.69507088830591,-23.1742356128,-7.9433833416931));
#86425=CARTESIAN_POINT('Ctrl Pts',(3.69394702409,-23.1742356128,-7.94679080481));
#86426=CARTESIAN_POINT('Origin',(-2.84607155346,-22.8742356128,5.53854202767));
#86427=CARTESIAN_POINT('',(6.72883656293,-23.1742356128,-5.99173026574));
#86428=CARTESIAN_POINT('Origin',(-2.84607155346,-23.1742356128,5.53854202767));
#86429=CARTESIAN_POINT('',(6.53717906469,-22.8742356128,-5.76093294477));
#86430=CARTESIAN_POINT('Origin',(6.72883656293,-22.8742356128,-5.99173026574));
#86431=CARTESIAN_POINT('Origin',(-2.84607155346,-22.8742356128,5.53854202767));
#86432=CARTESIAN_POINT('Origin',(3.1295913978,-23.1742356128,-2.83309600707));
#86433=CARTESIAN_POINT('',(3.32093311398,-19.4742356128,-2.75383967318));
#86434=CARTESIAN_POINT('',(0.11480502971,-19.4742356128,-4.08186140839));
#86435=CARTESIAN_POINT('',(-0.0382683432365,-19.4742356128,-4.14526647551));
#86436=CARTESIAN_POINT('',(0.11480502971,-23.0742356128,-4.08186140839));
#86437=CARTESIAN_POINT('',(0.11480502971,-21.2742356128,-4.08186140839));
#86438=CARTESIAN_POINT('',(3.32093311398,-23.0742356128,-2.75383967318));
#86439=CARTESIAN_POINT('',(-0.0382683432365,-23.0742356128,-4.14526647551));
#86440=CARTESIAN_POINT('',(3.32093311398,-21.2742356128,-2.75383967318));
#86441=CARTESIAN_POINT('Origin',(-2.84607155346,-20.0742356128,5.53854202767));
#86442=CARTESIAN_POINT('',(0.647446102181,-19.6742356128,-10.2675153591));
#86443=CARTESIAN_POINT('',(10.575526102,-19.6742356128,-3.51114482323));
#86444=CARTESIAN_POINT('Origin',(-2.84607155346,-19.6742356128,5.53854202767));
#86445=CARTESIAN_POINT('',(10.5755260956339,-22.0742355256,-3.51114483719302));
#86446=CARTESIAN_POINT('',(10.575526102,-21.2742356128,-3.51114482323));
#86447=CARTESIAN_POINT('',(10.9558455155,-22.6742356128,-2.9197793747));
#86448=CARTESIAN_POINT('Ctrl Pts',(10.5755260924509,-22.0742355256,-3.51114484417453));
#86449=CARTESIAN_POINT('Ctrl Pts',(10.5755260822369,-22.1031469614448,-3.51114486448172));
#86450=CARTESIAN_POINT('Ctrl Pts',(10.5767677418046,-22.1320579213261,-3.50930400549703));
#86451=CARTESIAN_POINT('Ctrl Pts',(10.5792325785806,-22.1606355884888,-3.50564573524642));
#86452=CARTESIAN_POINT('Ctrl Pts',(10.5800163561132,-22.1697228163623,-3.50448246550852));
#86453=CARTESIAN_POINT('Ctrl Pts',(10.5809235534889,-22.1787763809613,-3.50313572368826));
#86454=CARTESIAN_POINT('Ctrl Pts',(10.5819528553846,-22.1877857466703,-3.50160709265196));
#86455=CARTESIAN_POINT('Ctrl Pts',(10.5851501398811,-22.2157712244254,-3.49685875950131));
#86456=CARTESIAN_POINT('Ctrl Pts',(10.5895274155016,-22.2433280808744,-3.49035326238203));
#86457=CARTESIAN_POINT('Ctrl Pts',(10.5950216821739,-22.2701519594831,-3.48216748914416));
#86458=CARTESIAN_POINT('Ctrl Pts',(10.6005159488462,-22.2969758380917,-3.47398171590629));
#86459=CARTESIAN_POINT('Ctrl Pts',(10.6071270982676,-22.3230660301722,-3.46411560723739));
#86460=CARTESIAN_POINT('Ctrl Pts',(10.6147618810049,-22.3481448348233,-3.45268519075675));
#86461=CARTESIAN_POINT('Ctrl Pts',(10.622080654927,-22.3721856108078,-3.44172788693612));
#86462=CARTESIAN_POINT('Ctrl Pts',(10.6303374421656,-22.3952935640886,-3.42933684581244));
#86463=CARTESIAN_POINT('Ctrl Pts',(10.6394305448136,-22.4172536196383,-3.41564103111456));
#86464=CARTESIAN_POINT('Ctrl Pts',(10.6482304239307,-22.4385055335037,-3.40238686271701));
#86465=CARTESIAN_POINT('Ctrl Pts',(10.6578134256327,-22.458682025422,-3.38791074678196));
#86466=CARTESIAN_POINT('Ctrl Pts',(10.6680658047926,-22.4776185689884,-3.37236187144577));
#86467=CARTESIAN_POINT('Ctrl Pts',(10.669564024975,-22.4803858400105,-3.37008965360445));
#86468=CARTESIAN_POINT('Ctrl Pts',(10.6710765029369,-22.4831266918783,-3.36779458436634));
#86469=CARTESIAN_POINT('Ctrl Pts',(10.6726028459052,-22.4858406750051,-3.36547718891772));
#86470=CARTESIAN_POINT('Ctrl Pts',(10.6822657120498,-22.5030221710496,-3.35080638262524));
#86471=CARTESIAN_POINT('Ctrl Pts',(10.6924829158915,-22.5191257906813,-3.33524243824077));
#86472=CARTESIAN_POINT('Ctrl Pts',(10.7031594665192,-22.5340498367433,-3.31891032579951));
#86473=CARTESIAN_POINT('Ctrl Pts',(10.7138348392274,-22.5489722362692,-3.30258001524305));
#86474=CARTESIAN_POINT('Ctrl Pts',(10.7249691157714,-22.5627148211697,-3.28548218570652));
#86475=CARTESIAN_POINT('Ctrl Pts',(10.7364505099692,-22.5752141494242,-3.26777236884616));
#86476=CARTESIAN_POINT('Ctrl Pts',(10.7411978244337,-22.5803823581624,-3.2604497329104));
#86477=CARTESIAN_POINT('Ctrl Pts',(10.7460043143161,-22.5853385080984,-3.2530227890494));
#86478=CARTESIAN_POINT('Ctrl Pts',(10.7508614475812,-22.5900803309822,-3.24550376429458));
#86479=CARTESIAN_POINT('Ctrl Pts',(10.7627069683827,-22.6016446341505,-3.22716645311171));
#86480=CARTESIAN_POINT('Ctrl Pts',(10.7748560071437,-22.6119277933076,-3.20827751126037));
#86481=CARTESIAN_POINT('Ctrl Pts',(10.7871852725812,-22.620935663889,-3.18901744575809));
#86482=CARTESIAN_POINT('Ctrl Pts',(10.7903745404317,-22.6232657712415,-3.18403535594778));
#86483=CARTESIAN_POINT('Ctrl Pts',(10.7935758339048,-22.6255107998843,-3.17902851552711));
#86484=CARTESIAN_POINT('Ctrl Pts',(10.7967869569923,-22.6276714019374,-3.17400020894282));
#86485=CARTESIAN_POINT('Ctrl Pts',(10.8086005850894,-22.6356201938167,-3.15550121580945));
#86486=CARTESIAN_POINT('Ctrl Pts',(10.8205463051744,-22.6424216610541,-3.1367127417122));
#86487=CARTESIAN_POINT('Ctrl Pts',(10.8325097037303,-22.6481359064699,-3.11780970742614));
#86488=CARTESIAN_POINT('Ctrl Pts',(10.836369413317,-22.6499794735557,-3.11171108734659));
#86489=CARTESIAN_POINT('Ctrl Pts',(10.8402309498401,-22.65171026809,-3.10560060707827));
#86490=CARTESIAN_POINT('Ctrl Pts',(10.8440904541677,-22.6533314735688,-3.09948429558307));
#86491=CARTESIAN_POINT('Ctrl Pts',(10.8558666365666,-22.658278122103,-3.08082210643566));
#86492=CARTESIAN_POINT('Ctrl Pts',(10.8676229787536,-22.6621918852187,-3.06210658929104));
#86493=CARTESIAN_POINT('Ctrl Pts',(10.8792423341283,-22.6652063814963,-3.04352515477538));
#86494=CARTESIAN_POINT('Ctrl Pts',(10.8901782818038,-22.6680435762027,-3.02603661181894));
#86495=CARTESIAN_POINT('Ctrl Pts',(10.9009927099858,-22.6700845210861,-3.00866714751033));
#86496=CARTESIAN_POINT('Ctrl Pts',(10.9115939386224,-22.6714920197301,-2.99156911371205));
#86497=CARTESIAN_POINT('Ctrl Pts',(10.9122564291068,-22.6715799769368,-2.99050062579605));
#86498=CARTESIAN_POINT('Ctrl Pts',(10.9129180895068,-22.671665477032,-2.98943319573186));
#86499=CARTESIAN_POINT('Ctrl Pts',(10.9135788984978,-22.6717485664354,-2.98836685977345));
#86500=CARTESIAN_POINT('Ctrl Pts',(10.9246016135353,-22.6731345506286,-2.97057969651869));
#86501=CARTESIAN_POINT('Ctrl Pts',(10.9353804297876,-22.6738503295624,-2.95310776326211));
#86502=CARTESIAN_POINT('Ctrl Pts',(10.9458478020495,-22.6741130911883,-2.93607201666154));
#86503=CARTESIAN_POINT('Ctrl Pts',(10.9492132620403,-22.6741975740669,-2.93059469893907));
#86504=CARTESIAN_POINT('Ctrl Pts',(10.9525465530167,-22.6742356128,-2.92516247667493));
#86505=CARTESIAN_POINT('Ctrl Pts',(10.9558455155,-22.6742356128,-2.9197793747));
#86506=CARTESIAN_POINT('',(11.2053401891,-22.6742356128,-2.49849372966));
#86507=CARTESIAN_POINT('Origin',(-2.84607155346,-22.6742356128,5.53854202767));
#86508=CARTESIAN_POINT('',(11.5410915433775,-22.0742358826999,-1.880733914433));
#86509=CARTESIAN_POINT('Ctrl Pts',(11.2053401891,-22.6742356128,-2.49849372966));
#86510=CARTESIAN_POINT('Ctrl Pts',(11.2150383685076,-22.6742356128,-2.48153808629711));
#86511=CARTESIAN_POINT('Ctrl Pts',(11.2249897894519,-22.6738663548581,-2.46406918052205));
#86512=CARTESIAN_POINT('Ctrl Pts',(11.2351241182894,-22.6729000605474,-2.44619729884691));
#86513=CARTESIAN_POINT('Ctrl Pts',(11.2369260237553,-22.6727282513405,-2.44301963984323));
#86514=CARTESIAN_POINT('Ctrl Pts',(11.2387336971335,-22.6725376931046,-2.43982928294016));
#86515=CARTESIAN_POINT('Ctrl Pts',(11.2405467261739,-22.6723272624817,-2.43662689819009));
#86516=CARTESIAN_POINT('Ctrl Pts',(11.2503196279632,-22.6711929630497,-2.41936485166077));
#86517=CARTESIAN_POINT('Ctrl Pts',(11.2602458476986,-22.6694750423375,-2.40175690044939));
#86518=CARTESIAN_POINT('Ctrl Pts',(11.2702378606974,-22.6669990989714,-2.38395208224529));
#86519=CARTESIAN_POINT('Ctrl Pts',(11.2725244303702,-22.6664325047313,-2.37987763224816));
#86520=CARTESIAN_POINT('Ctrl Pts',(11.2748144198167,-22.665826417789,-2.37579294242994));
#86521=CARTESIAN_POINT('Ctrl Pts',(11.2771067403129,-22.6651791086157,-2.37169991214447));
#86522=CARTESIAN_POINT('Ctrl Pts',(11.2875627511759,-22.6622265233383,-2.35303028492714));
#86523=CARTESIAN_POINT('Ctrl Pts',(11.2980683420681,-22.658419074168,-2.33418470244293));
#86524=CARTESIAN_POINT('Ctrl Pts',(11.3085232390998,-22.6536382160094,-2.31534181654695));
#86525=CARTESIAN_POINT('Ctrl Pts',(11.311982469164,-22.6520563651097,-2.30910723793846));
#86526=CARTESIAN_POINT('Ctrl Pts',(11.3154361566497,-22.6503683749809,-2.30287299222311));
#86527=CARTESIAN_POINT('Ctrl Pts',(11.3188807244952,-22.6485711953677,-2.29664559899274));
#86528=CARTESIAN_POINT('Ctrl Pts',(11.3296723127873,-22.6429407583018,-2.27713561489883));
#86529=CARTESIAN_POINT('Ctrl Pts',(11.3403771745526,-22.6362330411102,-2.25768738349784));
#86530=CARTESIAN_POINT('Ctrl Pts',(11.350894153497,-22.6283844511168,-2.23848952894692));
#86531=CARTESIAN_POINT('Ctrl Pts',(11.3538790481232,-22.6261568899304,-2.23304085654893));
#86532=CARTESIAN_POINT('Ctrl Pts',(11.356848858058,-22.6238377439721,-2.22761230160938));
#86533=CARTESIAN_POINT('Ctrl Pts',(11.3598014066801,-22.6214262928633,-2.22220802156407));
#86534=CARTESIAN_POINT('Ctrl Pts',(11.3700755207974,-22.6130350597113,-2.20340250910257));
#86535=CARTESIAN_POINT('Ctrl Pts',(11.380144070066,-22.6035189145293,-2.18488415807147));
#86536=CARTESIAN_POINT('Ctrl Pts',(11.3899200358009,-22.5928768230476,-2.16682324106742));
#86537=CARTESIAN_POINT('Ctrl Pts',(11.3995284381226,-22.582417140672,-2.1490718943892));
#86538=CARTESIAN_POINT('Ctrl Pts',(11.4088538998602,-22.5708701456172,-2.13176302103624));
#86539=CARTESIAN_POINT('Ctrl Pts',(11.4178296800987,-22.5582763477247,-2.11503479986363));
#86540=CARTESIAN_POINT('Ctrl Pts',(11.41987788432,-22.5554025396189,-2.11121754806936));
#86541=CARTESIAN_POINT('Ctrl Pts',(11.4219079567884,-22.5524743831754,-2.10743041339639));
#86542=CARTESIAN_POINT('Ctrl Pts',(11.4239192477556,-22.5494926390321,-2.1036748141767));
#86543=CARTESIAN_POINT('Ctrl Pts',(11.43417381845,-22.5342902110344,-2.08452688464914));
#86544=CARTESIAN_POINT('Ctrl Pts',(11.4439376612349,-22.5176830774906,-2.06620306707214));
#86545=CARTESIAN_POINT('Ctrl Pts',(11.4531160015901,-22.4997822076498,-2.04890684167093));
#86546=CARTESIAN_POINT('Ctrl Pts',(11.4604919004757,-22.4853967086597,-2.03500724711187));
#86547=CARTESIAN_POINT('Ctrl Pts',(11.4674900183935,-22.4701767234614,-2.02177078277232));
#86548=CARTESIAN_POINT('Ctrl Pts',(11.4740689030204,-22.4541987893081,-2.00928995557508));
#86549=CARTESIAN_POINT('Ctrl Pts',(11.4825434750249,-22.4336168576976,-1.99321281260074));
#86550=CARTESIAN_POINT('Ctrl Pts',(11.490322094781,-22.4117772815337,-1.97839019854048));
#86551=CARTESIAN_POINT('Ctrl Pts',(11.497328194312,-22.388875007061,-1.96499799149759));
#86552=CARTESIAN_POINT('Ctrl Pts',(11.5044353732041,-22.3656423137493,-1.95141257056642));
#86553=CARTESIAN_POINT('Ctrl Pts',(11.5107475618039,-22.3413165292408,-1.93929939008369));
#86554=CARTESIAN_POINT('Ctrl Pts',(11.516202430633,-22.3161381940112,-1.92880681486341));
#86555=CARTESIAN_POINT('Ctrl Pts',(11.5217404470366,-22.2905760699918,-1.91815430322522));
#86556=CARTESIAN_POINT('Ctrl Pts',(11.5263947864914,-22.2641357626773,-1.90917247603084));
#86557=CARTESIAN_POINT('Ctrl Pts',(11.5301185510954,-22.2370988916848,-1.90197624996427));
#86558=CARTESIAN_POINT('Ctrl Pts',(11.5312011327901,-22.2292386683008,-1.89988414602147));
#86559=CARTESIAN_POINT('Ctrl Pts',(11.5322051805355,-22.2213281837172,-1.89794268745646));
#86560=CARTESIAN_POINT('Ctrl Pts',(11.5331298302645,-22.2133747150666,-1.8961540158936));
#86561=CARTESIAN_POINT('Ctrl Pts',(11.5363534362541,-22.18564654041,-1.88991817092117));
#86562=CARTESIAN_POINT('Ctrl Pts',(11.538610065403,-22.1573952246849,-1.88554404014394));
#86563=CARTESIAN_POINT('Ctrl Pts',(11.5398768288808,-22.1289373239018,-1.88308865866385));
#86564=CARTESIAN_POINT('Ctrl Pts',(11.5406859896255,-22.1107594899229,-1.88152025355765));
#86565=CARTESIAN_POINT('Ctrl Pts',(11.5410916389492,-22.0924976615588,-1.88073379444023));
#86566=CARTESIAN_POINT('Ctrl Pts',(11.5410916355629,-22.0742358827,-1.88073379476507));
#86567=CARTESIAN_POINT('',(11.5410914269,-19.6742356128,-1.88073402204));
#86568=CARTESIAN_POINT('',(11.5410914269,-21.2742356128,-1.88073402204));
#86569=CARTESIAN_POINT('',(12.9732844032,-19.6742356128,8.9713386779));
#86570=CARTESIAN_POINT('Origin',(-2.84607155346,-19.6742356128,5.53854202767));
#86571=CARTESIAN_POINT('',(12.9732844032,-22.9031898545,8.97133867789999));
#86572=CARTESIAN_POINT('',(12.9732844032,-21.2742356128,8.9713386779));
#86573=CARTESIAN_POINT('',(13.018207968,-22.8742356128,8.75735407375));
#86574=CARTESIAN_POINT('Origin',(12.9922058324069,-23.4864244001328,8.73196264121582));
#86575=CARTESIAN_POINT('',(3.81744045688,-22.8742356128,-9.21387212773));
#86576=CARTESIAN_POINT('Origin',(-2.84607155346,-22.8742356128,5.53854202767));
#86577=CARTESIAN_POINT('Ctrl Pts',(3.81744045688,-22.8742356128,-9.21387212773));
#86578=CARTESIAN_POINT('Ctrl Pts',(3.78438300100211,-22.8742356128,-9.22880383666651));
#86579=CARTESIAN_POINT('Ctrl Pts',(3.75125472648156,-22.876873984767,-9.24363320588492));
#86580=CARTESIAN_POINT('Ctrl Pts',(3.71838012225711,-22.8821739340745,-9.25821762563378));
#86581=CARTESIAN_POINT('Ctrl Pts',(3.6865095776919,-22.8873120117665,-9.27235660648325));
#86582=CARTESIAN_POINT('Ctrl Pts',(3.65487745148123,-22.8949539427161,-9.28626544525872));
#86583=CARTESIAN_POINT('Ctrl Pts',(3.62382288627738,-22.9051278862397,-9.29980564138486));
#86584=CARTESIAN_POINT('Ctrl Pts',(3.59982416043969,-22.9129902304622,-9.31026939936978));
#86585=CARTESIAN_POINT('Ctrl Pts',(3.57617118781195,-22.9223651478789,-9.32051284720793));
#86586=CARTESIAN_POINT('Ctrl Pts',(3.55303923210181,-22.9332555735994,-9.33046796299208));
#86587=CARTESIAN_POINT('Ctrl Pts',(3.52731510523081,-22.9453663824053,-9.34153865086025));
#86588=CARTESIAN_POINT('Ctrl Pts',(3.50223264779224,-22.9593502627365,-9.35225383201401));
#86589=CARTESIAN_POINT('Ctrl Pts',(3.47806004814019,-22.9751863932197,-9.36251314034884));
#86590=CARTESIAN_POINT('Ctrl Pts',(3.45499124406393,-22.990299397063,-9.37230397697133));
#86591=CARTESIAN_POINT('Ctrl Pts',(3.43275123888764,-23.0070999540256,-9.38167960517042));
#86592=CARTESIAN_POINT('Ctrl Pts',(3.41159767393858,-23.0255307665745,-9.39054653772574));
#86593=CARTESIAN_POINT('Ctrl Pts',(3.39154598669303,-23.0430015281129,-9.39895159658247));
#86594=CARTESIAN_POINT('Ctrl Pts',(3.37247065010445,-23.061937444689,-9.40689954920998));
#86595=CARTESIAN_POINT('Ctrl Pts',(3.35461163146646,-23.0822474209105,-9.41430534116002));
#86596=CARTESIAN_POINT('Ctrl Pts',(3.34903427425971,-23.0885902102061,-9.41661816405032));
#86597=CARTESIAN_POINT('Ctrl Pts',(3.34357569434173,-23.0950666709068,-9.41887806947029));
#86598=CARTESIAN_POINT('Ctrl Pts',(3.33824360900109,-23.1016730489955,-9.42108235584647));
#86599=CARTESIAN_POINT('Ctrl Pts',(3.32258626090874,-23.1210722811451,-9.42755511029096));
#86600=CARTESIAN_POINT('Ctrl Pts',(3.30801838438582,-23.1415942623807,-9.43354874753964));
#86601=CARTESIAN_POINT('Ctrl Pts',(3.29472253386083,-23.1631172221777,-9.43900011480726));
#86602=CARTESIAN_POINT('Ctrl Pts',(3.28136620602029,-23.1847380810018,-9.44447627808608));
#86603=CARTESIAN_POINT('Ctrl Pts',(3.26929464819255,-23.2073686497991,-9.44940485150287));
#86604=CARTESIAN_POINT('Ctrl Pts',(3.25868404771759,-23.2308337864388,-9.45372543317535));
#86605=CARTESIAN_POINT('Ctrl Pts',(3.24835603008727,-23.253673996612,-9.45793094857403));
#86606=CARTESIAN_POINT('Ctrl Pts',(3.23941312735556,-23.2773043321175,-9.46156012110628));
#86607=CARTESIAN_POINT('Ctrl Pts',(3.23199421260798,-23.3015220020268,-9.46456562543563));
#86608=CARTESIAN_POINT('Ctrl Pts',(3.22751779279442,-23.3161344434833,-9.46637908462574));
#86609=CARTESIAN_POINT('Ctrl Pts',(3.22359568701309,-23.3309599547749,-9.46796566933521));
#86610=CARTESIAN_POINT('Ctrl Pts',(3.22025193761968,-23.3459477027596,-9.46931721244178));
#86611=CARTESIAN_POINT('Ctrl Pts',(3.21506416160153,-23.3692009644169,-9.47141411089046));
#86612=CARTESIAN_POINT('Ctrl Pts',(3.21127189271638,-23.3928404899255,-9.47294403759531));
#86613=CARTESIAN_POINT('Ctrl Pts',(3.20893196554164,-23.4166584893515,-9.47388782994456));
#86614=CARTESIAN_POINT('Ctrl Pts',(3.20705389182888,-23.4357753059324,-9.47464533710999));
#86615=CARTESIAN_POINT('Ctrl Pts',(3.20611087685479,-23.4550065968702,-9.47502544136242));
#86616=CARTESIAN_POINT('Ctrl Pts',(3.20611087388,-23.4742356128,-9.47502544833));
#86617=CARTESIAN_POINT('',(0.647446102181,-22.5742356128,-10.2675153591));
#86618=CARTESIAN_POINT('Origin',(0.306146745892,-23.1742356128,5.46150961618));
#86619=CARTESIAN_POINT('',(0.11480502971,-19.4742356128,5.54076595007));
#86620=CARTESIAN_POINT('',(3.32093311398,-19.4742356128,4.21274421486));
#86621=CARTESIAN_POINT('',(-0.0382683432365,-19.4742356128,5.60417101718));
#86622=CARTESIAN_POINT('',(3.32093311415531,-23.073803734,4.21274421517325));
#86623=CARTESIAN_POINT('',(3.32093311398,-21.2742356128,4.21274421486));
#86624=CARTESIAN_POINT('',(3.28628881313932,-23.0742356036667,4.22709435412836));
#86625=CARTESIAN_POINT('Origin',(3.00255805893453,-22.7188049298779,4.34461947511254));
#86626=CARTESIAN_POINT('',(0.11480502971,-23.0742356128,5.54076595007));
#86627=CARTESIAN_POINT('',(-0.0382683432365,-23.0742356128,5.60417101718));
#86628=CARTESIAN_POINT('',(0.11480502971,-21.2742356128,5.54076595007));
#86629=CARTESIAN_POINT('Origin',(3.20612808427,-21.2742356128,3.93558035511));
#86630=CARTESIAN_POINT('',(3.48329194402,-19.4742356128,4.05038538482));
#86631=CARTESIAN_POINT('Origin',(3.20612808427,-19.4742356128,3.93558035511));
#86632=CARTESIAN_POINT('',(3.48329194400887,-23.0738037252489,4.05038538484686));
#86633=CARTESIAN_POINT('',(3.48329194402,-21.2742356128,4.05038538482));
#86634=CARTESIAN_POINT('Ctrl Pts',(3.48329194397624,-23.0738037279964,4.05038538492565));
#86635=CARTESIAN_POINT('Ctrl Pts',(3.48098634454964,-23.0736167153402,4.05595159432511));
#86636=CARTESIAN_POINT('Ctrl Pts',(3.4784307715636,-23.0733915443397,4.06163651831605));
#86637=CARTESIAN_POINT('Ctrl Pts',(3.47568621500459,-23.0731489780744,4.06724958582579));
#86638=CARTESIAN_POINT('Ctrl Pts',(3.47295007607425,-23.0729071557663,4.07284543790675));
#86639=CARTESIAN_POINT('Ctrl Pts',(3.47002625698439,-23.0726490502738,4.07836908794044));
#86640=CARTESIAN_POINT('Ctrl Pts',(3.46702586138249,-23.0723930177292,4.08364288587821));
#86641=CARTESIAN_POINT('Ctrl Pts',(3.46391091293507,-23.0721272100547,4.08911803345138));
#86642=CARTESIAN_POINT('Ctrl Pts',(3.46071410686951,-23.0718642230652,4.0943231709983));
#86643=CARTESIAN_POINT('Ctrl Pts',(3.45760867737687,-23.0716094471801,4.09908381872732));
#86644=CARTESIAN_POINT('Ctrl Pts',(3.45706037627568,-23.071564463419,4.09992436860887));
#86645=CARTESIAN_POINT('Ctrl Pts',(3.4565150238358,-23.0715196889556,4.10075113425691));
#86646=CARTESIAN_POINT('Ctrl Pts',(3.45597369050821,-23.0714750936175,4.10156324898665));
#86647=CARTESIAN_POINT('Ctrl Pts',(3.45121228376426,-23.0710828463037,4.10870636830695));
#86648=CARTESIAN_POINT('Ctrl Pts',(3.44576580670688,-23.0707659119886,4.11621427685738));
#86649=CARTESIAN_POINT('Ctrl Pts',(3.43950871638769,-23.0705320441909,4.12394678367705));
#86650=CARTESIAN_POINT('Ctrl Pts',(3.43696673293655,-23.0704370338839,4.12708816463349));
#86651=CARTESIAN_POINT('Ctrl Pts',(3.43413272839561,-23.0703508111332,4.13045538474554));
#86652=CARTESIAN_POINT('Ctrl Pts',(3.4311823830913,-23.0702865717675,4.13379961336395));
#86653=CARTESIAN_POINT('Ctrl Pts',(3.42822610199249,-23.0702222031588,4.13715057022999));
#86654=CARTESIAN_POINT('Ctrl Pts',(3.42515323237904,-23.070180117365,4.14047778426316));
#86655=CARTESIAN_POINT('Ctrl Pts',(3.42218199664131,-23.0701613237193,4.1435627393036));
#86656=CARTESIAN_POINT('Ctrl Pts',(3.42127115978427,-23.0701555624985,4.14450843698671));
#86657=CARTESIAN_POINT('Ctrl Pts',(3.42037014466647,-23.0701518952376,4.14543162551489));
#86658=CARTESIAN_POINT('Ctrl Pts',(3.41948589011018,-23.0701501102534,4.14632668871697));
#86659=CARTESIAN_POINT('Ctrl Pts',(3.41902952637369,-23.0701491890231,4.14678863079506));
#86660=CARTESIAN_POINT('Ctrl Pts',(3.41857813528195,-23.0701487673843,4.14724258288722));
#86661=CARTESIAN_POINT('Ctrl Pts',(3.4181311520111,-23.0701488062869,4.14768934682833));
#86662=CARTESIAN_POINT('Ctrl Pts',(3.40995185158464,-23.0701495181617,4.15586463376247));
#86663=CARTESIAN_POINT('Ctrl Pts',(3.40130199341124,-23.0703088319828,4.16357700165279));
#86664=CARTESIAN_POINT('Ctrl Pts',(3.392239298764,-23.0706029962599,4.17076819388485));
#86665=CARTESIAN_POINT('Ctrl Pts',(3.38355096748122,-23.0708850091479,4.17766233109926));
#86666=CARTESIAN_POINT('Ctrl Pts',(3.37448324687743,-23.0712911996594,4.18407710913278));
#86667=CARTESIAN_POINT('Ctrl Pts',(3.3650882824239,-23.0717548501856,4.18996630671111));
#86668=CARTESIAN_POINT('Ctrl Pts',(3.35653925662874,-23.072176752826,4.19532523087298));
#86669=CARTESIAN_POINT('Ctrl Pts',(3.34771933557013,-23.0726463371389,4.20024856543282));
#86670=CARTESIAN_POINT('Ctrl Pts',(3.33866815976237,-23.0730726361156,4.20471093107887));
#86671=CARTESIAN_POINT('Ctrl Pts',(3.33284862738816,-23.0733467287583,4.20758004796427));
#86672=CARTESIAN_POINT('Ctrl Pts',(3.32693351063594,-23.073602143823,4.21025877484239));
#86673=CARTESIAN_POINT('Ctrl Pts',(3.32093311468,-23.073803734,4.21274421611));
#86674=CARTESIAN_POINT('Origin',(3.56254827791,-23.1742356128,3.85904366864));
#86675=CARTESIAN_POINT('',(4.81131367923,-19.4742356128,0.844257300549));
#86676=CARTESIAN_POINT('',(4.02322090503,-19.4742356128,2.74688156443));
#86677=CARTESIAN_POINT('',(4.81131367968088,-23.0738037377,0.844257300670363));
#86678=CARTESIAN_POINT('',(4.81131367923,-21.2742356128,0.844257300549));
#86679=CARTESIAN_POINT('',(4.7969635399687,-23.0742356036667,0.878901601387461));
#86680=CARTESIAN_POINT('Origin',(4.67943816259639,-22.718804315054,1.16263295713764));
#86681=CARTESIAN_POINT('',(3.49764206635,-23.0742356128,4.01574112487));
#86682=CARTESIAN_POINT('',(3.72150316839,-23.0742356128,3.47529261624));
#86683=CARTESIAN_POINT('Origin',(3.6188764873545,-22.7074964989808,3.72305533773425));
#86684=CARTESIAN_POINT('Origin',(4.53414981948,-21.2742356128,0.729452270839));
#86685=CARTESIAN_POINT('',(4.81131367923,-19.4742356128,0.614647241129));
#86686=CARTESIAN_POINT('Origin',(4.53414981948,-19.4742356128,0.729452270839));
#86687=CARTESIAN_POINT('',(4.81131367923,-23.073803728,0.614647241129));
#86688=CARTESIAN_POINT('',(4.81131367923,-21.2742356128,0.614647241129));
#86689=CARTESIAN_POINT('Ctrl Pts',(4.81131367923,-23.073803728,0.614647241129));
#86690=CARTESIAN_POINT('Ctrl Pts',(4.81361941635584,-23.0736167041411,0.620213782969603));
#86691=CARTESIAN_POINT('Ctrl Pts',(4.81583231216333,-23.0733915202761,0.626041017783809));
#86692=CARTESIAN_POINT('Ctrl Pts',(4.81786074302077,-23.0731489400806,0.631951065709471));
#86693=CARTESIAN_POINT('Ctrl Pts',(4.81988294684359,-23.0729071045767,0.637842970510925));
#86694=CARTESIAN_POINT('Ctrl Pts',(4.82172136423803,-23.07264898495,0.643816521943502));
#86695=CARTESIAN_POINT('Ctrl Pts',(4.82332894451412,-23.072392936172,0.649667543460664));
#86696=CARTESIAN_POINT('Ctrl Pts',(4.82499787516201,-23.072127115759,0.655741858551897));
#86697=CARTESIAN_POINT('Ctrl Pts',(4.8264179869893,-23.0718641136417,0.66168312794498));
#86698=CARTESIAN_POINT('Ctrl Pts',(4.82758840454674,-23.0716093169037,0.667245496676535));
#86699=CARTESIAN_POINT('Ctrl Pts',(4.82779483941714,-23.0715643765905,0.668226571217771));
#86700=CARTESIAN_POINT('Ctrl Pts',(4.82799362825734,-23.0715196449537,0.669195839033689));
#86701=CARTESIAN_POINT('Ctrl Pts',(4.82818491470393,-23.0714750919041,0.670151934751179));
#86702=CARTESIAN_POINT('Ctrl Pts',(4.82986909518099,-23.0710828248214,0.678569874288066));
#86703=CARTESIAN_POINT('Ctrl Pts',(4.83132678694503,-23.0707658746989,0.687730166613046));
#86704=CARTESIAN_POINT('Ctrl Pts',(4.83237008382055,-23.070531995008,0.697622452530011));
#86705=CARTESIAN_POINT('Ctrl Pts',(4.83279391590162,-23.0704369830144,0.701641124707754));
#86706=CARTESIAN_POINT('Ctrl Pts',(4.83317095257545,-23.0703507579002,0.706025977439678));
#86707=CARTESIAN_POINT('Ctrl Pts',(4.83344946883151,-23.0702865157832,0.710476836880151));
#86708=CARTESIAN_POINT('Ctrl Pts',(4.83372854583356,-23.0702221443254,0.714936657383202));
#86709=CARTESIAN_POINT('Ctrl Pts',(4.83390839562994,-23.0701800553783,0.719462128784709));
#86710=CARTESIAN_POINT('Ctrl Pts',(4.83398881030789,-23.0701612585932,0.72374442753318));
#86711=CARTESIAN_POINT('Ctrl Pts',(4.83401346873702,-23.0701554947302,0.725057555470943));
#86712=CARTESIAN_POINT('Ctrl Pts',(4.83402915073398,-23.070151826053,0.726347808314679));
#86713=CARTESIAN_POINT('Ctrl Pts',(4.83403679243025,-23.0701500406831,0.727606300447712));
#86714=CARTESIAN_POINT('Ctrl Pts',(4.83404073492145,-23.0701491195781,0.728255579612234));
#86715=CARTESIAN_POINT('Ctrl Pts',(4.8340425442249,-23.0701486979849,0.728895692950971));
#86716=CARTESIAN_POINT('Ctrl Pts',(4.83404238791158,-23.0701487368575,0.729527607238744));
#86717=CARTESIAN_POINT('Ctrl Pts',(4.83403952722203,-23.0701494482644,0.741092268194386));
#86718=CARTESIAN_POINT('Ctrl Pts',(4.83337656821033,-23.0703087716981,0.752662286883749));
#86719=CARTESIAN_POINT('Ctrl Pts',(4.83205314158895,-23.070602953119,0.764155702040393));
#86720=CARTESIAN_POINT('Ctrl Pts',(4.83078440495958,-23.070884977629,0.775174157140385));
#86721=CARTESIAN_POINT('Ctrl Pts',(4.82890844194233,-23.0712911827742,0.786121930299115));
#86722=CARTESIAN_POINT('Ctrl Pts',(4.82642944014751,-23.0717548494332,0.796929483802132));
#86723=CARTESIAN_POINT('Ctrl Pts',(4.82417372918903,-23.0721767523,0.806763569812917));
#86724=CARTESIAN_POINT('Ctrl Pts',(4.82141849079573,-23.0726463352063,0.816481229255217));
#86725=CARTESIAN_POINT('Ctrl Pts',(4.81817380824922,-23.0730726323263,0.826036466393276));
#86726=CARTESIAN_POINT('Ctrl Pts',(4.81608756260042,-23.0733467301768,0.832180232884085));
#86727=CARTESIAN_POINT('Ctrl Pts',(4.81379910625625,-23.0736021493999,0.838256961933748));
#86728=CARTESIAN_POINT('Ctrl Pts',(4.81131368103,-23.0738037377,0.844257301033));
#86729=CARTESIAN_POINT('Origin',(4.73205734534,-23.1742356128,0.423305524947));
#86730=CARTESIAN_POINT('',(3.48329194402,-19.4742356128,-2.59148084314));
#86731=CARTESIAN_POINT('',(5.72621658766,-19.4742356128,2.8234182509));
#86732=CARTESIAN_POINT('',(3.48329194402,-23.0742356128,-2.59148084314));
#86733=CARTESIAN_POINT('',(3.48329194402,-21.2742356128,-2.59148084314));
#86734=CARTESIAN_POINT('',(4.79748445122,-23.0742356128,0.581260531297));
#86735=CARTESIAN_POINT('',(6.0279343243,-23.0742356128,3.55182930271));
#86736=CARTESIAN_POINT('',(4.80666892690046,-23.074039392286,0.603433817058651));
#86737=CARTESIAN_POINT('Ctrl Pts',(4.79748445122,-23.0742356128,0.581260531297));
#86738=CARTESIAN_POINT('Ctrl Pts',(4.79932022595,-23.0742356128,0.585692483551));
#86739=CARTESIAN_POINT('Ctrl Pts',(4.80115669118,-23.0742141429,0.590126102828));
#86740=CARTESIAN_POINT('Ctrl Pts',(4.80299369795,-23.0741730643,0.594561029481));
#86741=CARTESIAN_POINT('Ctrl Pts',(4.80483113724,-23.0741142107,0.598997000343));
#86742=CARTESIAN_POINT('Ctrl Pts',(4.80666892681,-23.0740393771,0.60343381684));
#86743=CARTESIAN_POINT('Origin',(4.6587912950397,-22.5974864729216,0.246425719139891));
#86744=CARTESIAN_POINT('Origin',(3.20612808427,-21.2742356128,-2.47667581343));
#86745=CARTESIAN_POINT('Origin',(3.20612808427,-19.4742356128,-2.47667581343));
#86746=CARTESIAN_POINT('Origin',(3.20612808427,-23.0742356128,-2.47667581343));
#86747=CARTESIAN_POINT('Origin',(9.38771846805,-25.4742356128,12.7721409138));
#86748=CARTESIAN_POINT('',(9.57074430825,-25.4742356128,13.0098414435));
#86749=CARTESIAN_POINT('Origin',(9.38771846805,-25.4742356128,12.7721409138));
#86750=CARTESIAN_POINT('Origin',(9.38771846805,-25.4742356128,12.7721409138));
#86751=CARTESIAN_POINT('Origin',(-2.72521192632E-16,-25.4742356128,0.580061096523));
#86752=CARTESIAN_POINT('',(12.4158608431,-25.4742356128,10.1688558911));
#86753=CARTESIAN_POINT('Origin',(12.1784264826,-25.4742356128,9.98548488886));
#86754=CARTESIAN_POINT('Origin',(-2.72521192632E-16,-25.4742356128,0.580061096523));
#86755=CARTESIAN_POINT('Origin',(9.38771846805,-22.5741587422,12.7721409138));
#86756=CARTESIAN_POINT('',(9.18405109086,-23.4742356128,12.9924125631));
#86757=CARTESIAN_POINT('',(9.18405109086,-24.4742356128,12.9924125631));
#86758=CARTESIAN_POINT('',(9.57074430825,-23.4742356128,13.0098414435));
#86759=CARTESIAN_POINT('',(9.57074430825,-21.2742356128,13.0098414435));
#86760=CARTESIAN_POINT('Origin',(9.38760641356428,-23.4742356128,12.7746270588514));
#86761=CARTESIAN_POINT('Origin',(3.88971125292,-23.1742356128,8.09716475273));
#86762=CARTESIAN_POINT('',(8.78908955148,-23.4742356128,12.6272235745));
#86763=CARTESIAN_POINT('',(6.87439641858,-23.4742356128,10.8568617063));
#86764=CARTESIAN_POINT('',(8.34854625295,-22.8742356128,12.2198888201));
#86765=CARTESIAN_POINT('Origin',(8.78908955139227,-22.8742356128972,12.627223574425));
#86766=CARTESIAN_POINT('',(8.34854625295,-21.0742356128,12.2198888201));
#86767=CARTESIAN_POINT('',(8.34854625295,-21.9742356128,12.2198888201));
#86768=CARTESIAN_POINT('',(5.19285862192,-21.0742356128,9.30207971851));
#86769=CARTESIAN_POINT('',(6.71750298683,-21.0742356128,10.7117950404));
#86770=CARTESIAN_POINT('',(5.19285862192,-22.8742356128,9.30207971851));
#86771=CARTESIAN_POINT('',(5.19285862192,-21.9742356128,9.30207971851));
#86772=CARTESIAN_POINT('',(6.46706166421,-22.8742356128,10.4802322066));
#86773=CARTESIAN_POINT('Origin',(4.98919124473,-21.9742356128,9.52235136777));
#86774=CARTESIAN_POINT('',(4.80552303981,-21.0742356128,9.28514683472));
#86775=CARTESIAN_POINT('Origin',(4.98919124473,-21.0742356128,9.52235136777));
#86776=CARTESIAN_POINT('',(4.80552303981,-22.8742356128,9.28514683472));
#86777=CARTESIAN_POINT('',(4.80552303981,-21.2742356128,9.28514683472));
#86778=CARTESIAN_POINT('Origin',(4.98919124473,-22.8742356128,9.52235136777));
#86779=CARTESIAN_POINT('Origin',(0.00234331738835,-21.2742356128,3.08191746407));
#86780=CARTESIAN_POINT('',(1.01141425905,-22.8742356128,10.8621723381));
#86781=CARTESIAN_POINT('Origin',(0.00234331738803,-22.8742356128,3.08191746407));
#86782=CARTESIAN_POINT('',(1.01141425905,-21.0742356128,10.8621723381));
#86783=CARTESIAN_POINT('Origin',(0.00234331738803,-21.0742356128,3.08191746407));
#86784=CARTESIAN_POINT('',(1.01141425905,-21.9742356128,10.8621723381));
#86785=CARTESIAN_POINT('Origin',(1.05,-21.9742356128,11.1596805575));
#86786=CARTESIAN_POINT('',(0.75,-21.0742356128,11.1596805575));
#86787=CARTESIAN_POINT('Origin',(1.05,-21.0742356128,11.1596805575));
#86788=CARTESIAN_POINT('',(0.75,-22.8742356128,11.1596805575));
#86789=CARTESIAN_POINT('',(0.75,-21.9742356128,11.1596805575));
#86790=CARTESIAN_POINT('Origin',(1.05,-22.8742356128,11.1596805575));
#86791=CARTESIAN_POINT('Origin',(0.75,-23.1742356128,-8.70195642562));
#86792=CARTESIAN_POINT('',(0.75,-22.8742356128,14.92922515));
#86793=CARTESIAN_POINT('',(0.75,-22.8742356128,2.93538176615));
#86794=CARTESIAN_POINT('',(0.75,-21.0742356128,14.92922515));
#86795=CARTESIAN_POINT('',(0.75,-21.0742356128,12.1167294155));
#86796=CARTESIAN_POINT('',(0.75,-21.9742356128,14.92922515));
#86797=CARTESIAN_POINT('Origin',(8.14487887576,-21.9742356128,12.4401604693));
#86798=CARTESIAN_POINT('',(8.31471092647,-21.0742356128,12.6874600337));
#86799=CARTESIAN_POINT('',(8.31471092647,-22.8742356128,12.6874600337));
#86800=CARTESIAN_POINT('',(8.31471092647,-22.5742356128,12.6874600337));
#86801=CARTESIAN_POINT('Origin',(8.14487887576,-21.0742356128,12.4401604693));
#86802=CARTESIAN_POINT('Ctrl Pts',(8.31471092647,-22.8742356128,12.6874600337));
#86803=CARTESIAN_POINT('Ctrl Pts',(8.40342053421,-22.8742356128,12.6265390425));
#86804=CARTESIAN_POINT('Ctrl Pts',(8.4651120838,-22.8742356128,12.5258960706));
#86805=CARTESIAN_POINT('Ctrl Pts',(8.47411942559,-22.8742356128,12.4014233916));
#86806=CARTESIAN_POINT('Ctrl Pts',(8.4275605919,-22.8742356128,12.2929469882));
#86807=CARTESIAN_POINT('Ctrl Pts',(8.34854625295,-22.8742356128,12.2198888201));
#86808=CARTESIAN_POINT('Origin',(1.05,-21.9742356128,14.92922515));
#86809=CARTESIAN_POINT('',(1.07189396011,-21.0742356128,15.2284251743));
#86810=CARTESIAN_POINT('Origin',(1.05,-21.0742356128,14.92922515));
#86811=CARTESIAN_POINT('',(1.07189396011,-22.8742356128,15.2284251743));
#86812=CARTESIAN_POINT('',(1.07189396011,-22.5742356128,15.2284251743));
#86813=CARTESIAN_POINT('Origin',(1.05,-22.8742356128,14.92922515));
#86814=CARTESIAN_POINT('Origin',(2.4183046301E-16,-21.2742356128,0.580061096523));
#86815=CARTESIAN_POINT('Origin',(2.04268023839E-15,-21.0742356128,0.580061096523));
#86816=CARTESIAN_POINT('Origin',(-2.61864828395E-15,-22.8742356128,0.580061096523));
#86817=CARTESIAN_POINT('Origin',(0.45,-22.8742356128,2.93538176615));
#86818=CARTESIAN_POINT('',(0.75,-22.8742356128,-6.23438845923));
#86819=CARTESIAN_POINT('',(0.75,-22.8742356128,-4.99584562937));
#86820=CARTESIAN_POINT('',(0.75,-22.8742356128,-5.6151170443));
#86821=CARTESIAN_POINT('',(0.45,-23.1742356128,-4.99584562937));
#86822=CARTESIAN_POINT('Origin',(0.45,-22.8742356128,-4.99584562937));
#86823=CARTESIAN_POINT('',(0.45,-23.1742356128,-5.6151170443));
#86824=CARTESIAN_POINT('Origin',(0.45,-22.8742356128,-6.23438845923));
#86825=CARTESIAN_POINT('Origin',(8.13895521212E-16,-22.8742356128,0.729452270839));
#86826=CARTESIAN_POINT('',(0.935307608221,-23.1742356128,5.53218022249));
#86827=CARTESIAN_POINT('',(1.12365184404,-23.1742356128,5.49163692002));
#86828=CARTESIAN_POINT('Origin',(3.42702565972E-16,-23.1742356128,0.729452270839));
#86829=CARTESIAN_POINT('',(1.19254592572,-22.8742356128,5.78361912069));
#86830=CARTESIAN_POINT('Origin',(1.12365184404,-22.8742356128,5.49163692002));
#86831=CARTESIAN_POINT('',(0.992653804111,-22.8742356128,5.82664824081));
#86832=CARTESIAN_POINT('Origin',(3.67394039744E-17,-22.8742356128,0.729452270839));
#86833=CARTESIAN_POINT('Origin',(0.935307608221,-22.8742356128,5.53218022249));
#86834=CARTESIAN_POINT('Origin',(1.05,-22.8742356128,6.12111625914));
#86835=CARTESIAN_POINT('',(0.45,-23.1742356128,6.12111625914));
#86836=CARTESIAN_POINT('Origin',(1.05,-23.1742356128,6.12111625914));
#86837=CARTESIAN_POINT('',(0.75,-22.8742356128,6.12111625914));
#86838=CARTESIAN_POINT('Origin',(1.05,-22.8742356128,6.12111625914));
#86839=CARTESIAN_POINT('Origin',(0.45,-22.8742356128,6.12111625914));
#86840=CARTESIAN_POINT('Origin',(0.45,-22.8742356128,2.93538176615));
#86841=CARTESIAN_POINT('',(0.45,-23.1742356128,9.0358656718));
#86842=CARTESIAN_POINT('',(0.45,-23.1742356128,7.57849096547));
#86843=CARTESIAN_POINT('',(0.75,-22.8742356128,9.0358656718));
#86844=CARTESIAN_POINT('',(0.75,-22.8742356128,7.57849096547));
#86845=CARTESIAN_POINT('Origin',(0.45,-22.8742356128,9.0358656718));
#86846=CARTESIAN_POINT('Origin',(1.05,-22.8742356128,9.0358656718));
#86847=CARTESIAN_POINT('',(1.15397857793,-23.1742356128,9.62678737163));
#86848=CARTESIAN_POINT('Origin',(1.05,-23.1742356128,9.0358656718));
#86849=CARTESIAN_POINT('',(1.10198928897,-22.8742356128,9.33132652171));
#86850=CARTESIAN_POINT('Origin',(1.05,-22.8742356128,9.0358656718));
#86851=CARTESIAN_POINT('Origin',(1.15397857793,-22.8742356128,9.62678737163));
#86852=CARTESIAN_POINT('Origin',(0.00234331738835,-22.8742356128,3.08191746407));
#86853=CARTESIAN_POINT('',(3.7572334818,-23.1742356128,8.56483509371));
#86854=CARTESIAN_POINT('Origin',(0.00234331738835,-23.1742356128,3.08191746407));
#86855=CARTESIAN_POINT('',(3.58772315463,-22.8742356128,8.31731489457));
#86856=CARTESIAN_POINT('Origin',(0.00234331738835,-22.8742356128,3.08191746407));
#86857=CARTESIAN_POINT('Origin',(3.7572334818,-22.8742356128,8.56483509371));
#86858=CARTESIAN_POINT('Origin',(1.2614400074,-22.8742356128,6.07560132137));
#86859=CARTESIAN_POINT('',(1.66877476178,-23.1742356128,5.63505802284));
#86860=CARTESIAN_POINT('Origin',(1.2614400074,-23.1742356128,6.07560132137));
#86861=CARTESIAN_POINT('',(1.46510738459,-22.8742356128,5.8553296721));
#86862=CARTESIAN_POINT('Origin',(1.66877476178,-22.8742356128,5.63505802284));
#86863=CARTESIAN_POINT('Origin',(1.2614400074,-22.8742356128,6.07560132137));
#86864=CARTESIAN_POINT('Origin',(3.41821282746,-22.8742356128,8.06979469543));
#86865=CARTESIAN_POINT('',(3.82554758184,-23.1742356128,7.6292513969));
#86866=CARTESIAN_POINT('Origin',(3.41821282746,-23.1742356128,8.06979469543));
#86867=CARTESIAN_POINT('',(3.62188020465,-22.8742356128,7.84952304616));
#86868=CARTESIAN_POINT('Origin',(3.41821282746,-22.8742356128,8.06979469543));
#86869=CARTESIAN_POINT('Origin',(3.82554758184,-22.8742356128,7.6292513969));
#86870=CARTESIAN_POINT('Origin',(6.6707290414,-22.8742356128,10.2599605573));
#86871=CARTESIAN_POINT('',(2.74716117181,-23.1742356128,6.63215470987));
#86872=CARTESIAN_POINT('',(2.54349379462,-22.8742356128,6.85242635913));
#86873=CARTESIAN_POINT('Origin',(0.00234331738835,-22.8742356128,3.08191746407));
#86874=CARTESIAN_POINT('',(6.21380646358,-22.8742356128,1.78497474518));
#86875=CARTESIAN_POINT('',(5.76218263052,-22.8742356128,0.419477620705));
#86876=CARTESIAN_POINT('Origin',(0.00234331738835,-22.8742356128,3.08191746407));
#86877=CARTESIAN_POINT('',(6.03449750111,-23.1742356128,0.293602240855));
#86878=CARTESIAN_POINT('Origin',(6.03449750111,-22.8742356128,0.293602240855));
#86879=CARTESIAN_POINT('',(6.50747329887,-23.1742356128,1.72365761992));
#86880=CARTESIAN_POINT('Origin',(0.00234331738835,-23.1742356128,3.08191746407));
#86881=CARTESIAN_POINT('Origin',(6.50747329887,-22.8742356128,1.72365761992));
#86882=CARTESIAN_POINT('Ctrl Pts',(4.90348290416,-23.1739412926,0.565017054665));
#86883=CARTESIAN_POINT('Ctrl Pts',(4.87372566569,-23.1752779987,0.577365446817));
#86884=CARTESIAN_POINT('Ctrl Pts',(4.8433931743,-23.1636304197,0.589733130986));
#86885=CARTESIAN_POINT('Ctrl Pts',(4.81906109907,-23.1385222588,0.599388343724));
#86886=CARTESIAN_POINT('Ctrl Pts',(4.80686116456,-23.1062808154,0.603897954914));
#86887=CARTESIAN_POINT('Ctrl Pts',(4.80666892681,-23.0740393771,0.60343381684));
#86888=CARTESIAN_POINT('Ctrl Pts',(4.90080268812,-23.1740535365,0.560642186752));
#86889=CARTESIAN_POINT('Ctrl Pts',(4.87118078695,-23.1751250633,0.572926200655));
#86890=CARTESIAN_POINT('Ctrl Pts',(4.84109884961,-23.1633367321,0.585221262381));
#86891=CARTESIAN_POINT('Ctrl Pts',(4.81703621353,-23.138278721,0.59483800517));
#86892=CARTESIAN_POINT('Ctrl Pts',(4.80498960977,-23.1061964638,0.5993796148));
#86893=CARTESIAN_POINT('Ctrl Pts',(4.80483113724,-23.0741142107,0.598997000343));
#86894=CARTESIAN_POINT('Ctrl Pts',(4.89810075797,-23.174141808,0.556252600105));
#86895=CARTESIAN_POINT('Ctrl Pts',(4.86861969578,-23.1749465698,0.568471513776));
#86896=CARTESIAN_POINT('Ctrl Pts',(4.83879402141,-23.1630185285,0.580695452156));
#86897=CARTESIAN_POINT('Ctrl Pts',(4.81500555152,-23.1380131826,0.59027755579));
#86898=CARTESIAN_POINT('Ctrl Pts',(4.80311602073,-23.1060931221,0.594856360919));
#86899=CARTESIAN_POINT('Ctrl Pts',(4.80299369795,-23.0741730643,0.594561029481));
#86900=CARTESIAN_POINT('Ctrl Pts',(4.89537785067,-23.1742034158,0.551847890098));
#86901=CARTESIAN_POINT('Ctrl Pts',(4.86604324142,-23.1747403351,0.564001283399));
#86902=CARTESIAN_POINT('Ctrl Pts',(4.83647936267,-23.162674027,0.576155883108));
#86903=CARTESIAN_POINT('Ctrl Pts',(4.81296943337,-23.1377239686,0.585707321132));
#86904=CARTESIAN_POINT('Ctrl Pts',(4.80124051889,-23.1059690552,0.590328488331));
#86905=CARTESIAN_POINT('Ctrl Pts',(4.80115669118,-23.0742141429,0.590126102828));
#86906=CARTESIAN_POINT('Ctrl Pts',(4.89263477146,-23.1742356128,0.547427786194));
#86907=CARTESIAN_POINT('Ctrl Pts',(4.86345231855,-23.1745041136,0.559515553974));
#86908=CARTESIAN_POINT('Ctrl Pts',(4.83415555361,-23.1623013592,0.571602872333));
#86909=CARTESIAN_POINT('Ctrl Pts',(4.81092823343,-23.1374093317,0.581127733296));
#86910=CARTESIAN_POINT('Ctrl Pts',(4.79936326115,-23.1058224723,0.585796379724));
#86911=CARTESIAN_POINT('Ctrl Pts',(4.79932022595,-23.0742356128,0.585692483551));
#86912=CARTESIAN_POINT('Ctrl Pts',(4.88987240447,-23.1742356128,0.542992188061));
#86913=CARTESIAN_POINT('Ctrl Pts',(4.86084787295,-23.1742356128,0.555014542658));
#86914=CARTESIAN_POINT('Ctrl Pts',(4.83182334143,-23.1618986073,0.567036897256));
#86915=CARTESIAN_POINT('Ctrl Pts',(4.80888235809,-23.1370674659,0.576539363687));
#86916=CARTESIAN_POINT('Ctrl Pts',(4.79748445122,-23.1056515394,0.581260531297));
#86917=CARTESIAN_POINT('Ctrl Pts',(4.79748445122,-23.0742356128,0.581260531297));
#86918=CARTESIAN_POINT('',(4.88987240447,-23.1742356128,0.542992188061));
#86919=CARTESIAN_POINT('Origin',(4.8892191319917,-23.074942709897,0.543262782382199));
#86920=CARTESIAN_POINT('',(4.90348290262634,-23.1739412930696,0.565017052852735));
#86921=CARTESIAN_POINT('Ctrl Pts',(4.88987240447,-23.1742356128,0.542992188061));
#86922=CARTESIAN_POINT('Ctrl Pts',(4.89447634935402,-23.1742356128,0.550384851456529));
#86923=CARTESIAN_POINT('Ctrl Pts',(4.89901587678319,-23.1741283657784,0.557725607105687));
#86924=CARTESIAN_POINT('Ctrl Pts',(4.90348290292941,-23.1739412926515,0.565017052656334));
#86925=CARTESIAN_POINT('Origin',(4.89839481331612,-23.0747913371752,0.565452395094602));
#86926=CARTESIAN_POINT('Origin',(5.48986775992,-22.8742356128,0.545353000555));
#86927=CARTESIAN_POINT('Origin',(5.48986775992,-23.1742356128,0.545353000555));
#86928=CARTESIAN_POINT('',(5.1900363009,-22.8742356128,0.55540766038));
#86929=CARTESIAN_POINT('Origin',(5.48986775992,-22.8742356128,0.545353000555));
#86930=CARTESIAN_POINT('Origin',(4.89020484189,-22.8742356128,0.565462320206));
#86931=CARTESIAN_POINT('Ctrl Pts',(4.88935150261,-23.1742356021,0.91716994496));
#86932=CARTESIAN_POINT('Ctrl Pts',(4.86032696478,-23.1742356,0.905147589619));
#86933=CARTESIAN_POINT('Ctrl Pts',(4.83130242791,-23.1618985927,0.893125234378));
#86934=CARTESIAN_POINT('Ctrl Pts',(4.80836144191,-23.1370674502,0.883622767727));
#86935=CARTESIAN_POINT('Ctrl Pts',(4.79696353608,-23.1056515239,0.878901600531));
#86936=CARTESIAN_POINT('Ctrl Pts',(4.79696353997,-23.0742355991,0.878901601388));
#86937=CARTESIAN_POINT('Ctrl Pts',(4.89352277618,-23.1742356053,0.910289082657));
#86938=CARTESIAN_POINT('Ctrl Pts',(4.86427270861,-23.1746190551,0.898173309533));
#86939=CARTESIAN_POINT('Ctrl Pts',(4.83486220494,-23.1624737743,0.886051376935));
#86940=CARTESIAN_POINT('Ctrl Pts',(4.81151797125,-23.1375556797,0.876503237567));
#86941=CARTESIAN_POINT('Ctrl Pts',(4.79988864887,-23.1058956405,0.871839755064));
#86942=CARTESIAN_POINT('Ctrl Pts',(4.7998343674,-23.0742356024,0.871970810865));
#86943=CARTESIAN_POINT('Ctrl Pts',(4.89770025261,-23.1741720972,0.903404272608));
#86944=CARTESIAN_POINT('Ctrl Pts',(4.86823093749,-23.1749477738,0.8911929985));
#86945=CARTESIAN_POINT('Ctrl Pts',(4.8384337256,-23.1630030812,0.878969713281));
#86946=CARTESIAN_POINT('Ctrl Pts',(4.81468031581,-23.138001656,0.869376268272));
#86947=CARTESIAN_POINT('Ctrl Pts',(4.80281540183,-23.1060974603,0.864773950955));
#86948=CARTESIAN_POINT('Ctrl Pts',(4.80270499263,-23.0741932655,0.865040508505));
#86949=CARTESIAN_POINT('Ctrl Pts',(4.90188362001,-23.1740438599,0.896515941201));
#86950=CARTESIAN_POINT('Ctrl Pts',(4.87220170104,-23.1752205531,0.884206882396));
#86951=CARTESIAN_POINT('Ctrl Pts',(4.84201719325,-23.1634855096,0.871880308931));
#86952=CARTESIAN_POINT('Ctrl Pts',(4.81784851738,-23.1384045129,0.862241927592));
#86953=CARTESIAN_POINT('Ctrl Pts',(4.80574369007,-23.1062561443,0.85770444106));
#86954=CARTESIAN_POINT('Ctrl Pts',(4.80557522399,-23.074107776,0.858111157027));
#86955=CARTESIAN_POINT('Ctrl Pts',(4.90607254573,-23.1738495698,0.889624547672));
#86956=CARTESIAN_POINT('Ctrl Pts',(4.87618505232,-23.1754360753,0.877215197865));
#86957=CARTESIAN_POINT('Ctrl Pts',(4.84561282186,-23.1639199594,0.864783222044));
#86958=CARTESIAN_POINT('Ctrl Pts',(4.82102262893,-23.1387632939,0.855100274339));
#86959=CARTESIAN_POINT('Ctrl Pts',(4.80867340462,-23.1063707724,0.850631487337));
#86960=CARTESIAN_POINT('Ctrl Pts',(4.80844485738,-23.0739782508,0.851183249168));
#86961=CARTESIAN_POINT('Ctrl Pts',(4.91026668047,-23.1735877856,0.88273057755));
#86962=CARTESIAN_POINT('Ctrl Pts',(4.88018105717,-23.1755928932,0.870218178851));
#86963=CARTESIAN_POINT('Ctrl Pts',(4.84922086665,-23.1643052014,0.857678479765));
#86964=CARTESIAN_POINT('Ctrl Pts',(4.82420271933,-23.1390769393,0.847951335568));
#86965=CARTESIAN_POINT('Ctrl Pts',(4.81160443804,-23.1064403336,0.843555346692));
#86966=CARTESIAN_POINT('Ctrl Pts',(4.81131367923,-23.073803728,0.844257300549));
#86967=CARTESIAN_POINT('',(4.91026667615,-23.1735877859,0.882730584254));
#86968=CARTESIAN_POINT('Origin',(4.90303610744803,-23.074577514893,0.882230480615193));
#86969=CARTESIAN_POINT('',(4.88935150281824,-23.17423560745,0.917169942276108));
#86970=CARTESIAN_POINT('Origin',(4.78463428057749,-22.695072482409,1.13494583768666));
#86971=CARTESIAN_POINT('Origin',(4.88869822348194,-23.0749427242252,0.916899342539095));
#86972=CARTESIAN_POINT('Ctrl Pts',(4.91032402632243,-23.1735838337648,0.882801288663071));
#86973=CARTESIAN_POINT('Ctrl Pts',(4.88022665094269,-23.1756159833063,0.870279796156956));
#86974=CARTESIAN_POINT('Ctrl Pts',(4.84924391018748,-23.1643432866006,0.857726457153785));
#86975=CARTESIAN_POINT('Ctrl Pts',(4.82420253417771,-23.1391098958492,0.847986322123972));
#86976=CARTESIAN_POINT('Ctrl Pts',(4.81159274228477,-23.1064572908804,0.8435837999636));
#86977=CARTESIAN_POINT('Ctrl Pts',(4.8113020121647,-23.0738046836214,0.844285468079136));
#86978=CARTESIAN_POINT('Ctrl Pts',(4.94434678643153,-23.1714537954251,0.826899603928996));
#86979=CARTESIAN_POINT('Ctrl Pts',(4.91067754612114,-23.1770054612896,0.818105977984605));
#86980=CARTESIAN_POINT('Ctrl Pts',(4.87457563392111,-23.1676522550584,0.809243170339568));
#86981=CARTESIAN_POINT('Ctrl Pts',(4.84456167258553,-23.1418126359453,0.802686041110078));
#86982=CARTESIAN_POINT('Ctrl Pts',(4.82932405322906,-23.1071018168935,0.800487598287962));
#86983=CARTESIAN_POINT('Ctrl Pts',(4.82875103516455,-23.072390977125,0.802171963194603));
#86984=CARTESIAN_POINT('Ctrl Pts',(4.96420701657059,-23.1658533501376,0.763668324381971));
#86985=CARTESIAN_POINT('Ctrl Pts',(4.92841400152884,-23.1744320422292,0.760047974352074));
#86986=CARTESIAN_POINT('Ctrl Pts',(4.88880843425898,-23.167036746932,0.75637324615978));
#86987=CARTESIAN_POINT('Ctrl Pts',(4.85536678488683,-23.1410190286572,0.753869397878117));
#86988=CARTESIAN_POINT('Ctrl Pts',(4.83885676622638,-23.104840908069,0.753537697803965));
#86989=CARTESIAN_POINT('Ctrl Pts',(4.83896173895554,-23.0686627522125,0.754909330181028));
#86990=CARTESIAN_POINT('Ctrl Pts',(4.96420960733232,-23.1658532166256,0.695240215931854));
#86991=CARTESIAN_POINT('Ctrl Pts',(4.92841570207977,-23.1744322004681,0.698860297638863));
#86992=CARTESIAN_POINT('Ctrl Pts',(4.88880908546722,-23.1670368247264,0.702534748596797));
#86993=CARTESIAN_POINT('Ctrl Pts',(4.85536672756385,-23.1410185335977,0.705038288754641));
#86994=CARTESIAN_POINT('Ctrl Pts',(4.83885679345067,-23.1048397903563,0.705369584679646));
#86995=CARTESIAN_POINT('Ctrl Pts',(4.83896246818167,-23.0686613287168,0.703997574618044));
#86996=CARTESIAN_POINT('Ctrl Pts',(4.94434696413387,-23.1714537954603,0.632005245990061));
#86997=CARTESIAN_POINT('Ctrl Pts',(4.91067766676893,-23.1770054791343,0.640798851452071));
#86998=CARTESIAN_POINT('Ctrl Pts',(4.87457568728806,-23.167652266686,0.649661638070962));
#86999=CARTESIAN_POINT('Ctrl Pts',(4.8445616776457,-23.1418126091363,0.65621874298175));
#87000=CARTESIAN_POINT('Ctrl Pts',(4.82932406284209,-23.1071017495619,0.658417158281277));
#87001=CARTESIAN_POINT('Ctrl Pts',(4.82875108823279,-23.0723908897367,0.656732768578983));
#87002=CARTESIAN_POINT('Ctrl Pts',(4.91032403084861,-23.1735838343689,0.576103259411724));
#87003=CARTESIAN_POINT('Ctrl Pts',(4.88022665064079,-23.1756159843951,0.58862475168427));
#87004=CARTESIAN_POINT('Ctrl Pts',(4.84924390460287,-23.1643432860911,0.601178090382025));
#87005=CARTESIAN_POINT('Ctrl Pts',(4.82420252556862,-23.1391098913619,0.610918224408618));
#87006=CARTESIAN_POINT('Ctrl Pts',(4.81159273532899,-23.1064572826193,0.615320744486395));
#87007=CARTESIAN_POINT('Ctrl Pts',(4.81130201028653,-23.073804673977,0.614619073855797));
#87008=CARTESIAN_POINT('',(4.91026667801796,-23.1735877850581,0.576173964176449));
#87009=CARTESIAN_POINT('Origin',(4.90303610342538,-23.0745775186776,0.576674063713962));
#87010=CARTESIAN_POINT('Ctrl Pts',(4.91026667829262,-23.1735877856817,0.576173964033033));
#87011=CARTESIAN_POINT('Ctrl Pts',(4.91879478395542,-23.1730554892432,0.590191754493607));
#87012=CARTESIAN_POINT('Ctrl Pts',(4.92622882474333,-23.1722658877838,0.604789479073382));
#87013=CARTESIAN_POINT('Ctrl Pts',(4.93243370799892,-23.1714622149877,0.619819256633221));
#87014=CARTESIAN_POINT('Ctrl Pts',(4.93811287037115,-23.1707266349428,0.633575606860094));
#87015=CARTESIAN_POINT('Ctrl Pts',(4.94276367114871,-23.169980088222,0.647693656938457));
#87016=CARTESIAN_POINT('Ctrl Pts',(4.94629890408633,-23.1693713285753,0.662053029204814));
#87017=CARTESIAN_POINT('Ctrl Pts',(4.94857426938964,-23.1689795154748,0.671295084257086));
#87018=CARTESIAN_POINT('Ctrl Pts',(4.95038777030555,-23.1686439942748,0.680636981774246));
#87019=CARTESIAN_POINT('Ctrl Pts',(4.95171673385527,-23.1683928076863,0.690045471846521));
#87020=CARTESIAN_POINT('Ctrl Pts',(4.95361415108075,-23.168034178016,0.703478369334758));
#87021=CARTESIAN_POINT('Ctrl Pts',(4.95454008117551,-23.1678467304298,0.717033448149962));
#87022=CARTESIAN_POINT('Ctrl Pts',(4.95448640970839,-23.1678573287494,0.730585086546251));
#87023=CARTESIAN_POINT('Ctrl Pts',(4.95447403946633,-23.1678597714585,0.733708478850725));
#87024=CARTESIAN_POINT('Ctrl Pts',(4.95440960372007,-23.1678725183262,0.736831685519014));
#87025=CARTESIAN_POINT('Ctrl Pts',(4.95429295109091,-23.1678955066979,0.739953164503366));
#87026=CARTESIAN_POINT('Ctrl Pts',(4.95376672469149,-23.1679992085021,0.754034327171142));
#87027=CARTESIAN_POINT('Ctrl Pts',(4.95214771891704,-23.1683223664373,0.768061308831125));
#87028=CARTESIAN_POINT('Ctrl Pts',(4.94950130935781,-23.1688045279757,0.781917200280443));
#87029=CARTESIAN_POINT('Ctrl Pts',(4.94672033804524,-23.1693112059394,0.796477621019677));
#87030=CARTESIAN_POINT('Ctrl Pts',(4.94280411815531,-23.1699929254357,0.810849003605565));
#87031=CARTESIAN_POINT('Ctrl Pts',(4.93782602638737,-23.1707197504248,0.82489992093009));
#87032=CARTESIAN_POINT('Ctrl Pts',(4.93251851625825,-23.1714946720558,0.839880638341444));
#87033=CARTESIAN_POINT('Ctrl Pts',(4.92600261331167,-23.1723201180346,0.854496854361639));
#87034=CARTESIAN_POINT('Ctrl Pts',(4.91838074795892,-23.1729821955269,0.86859655447077));
#87035=CARTESIAN_POINT('Ctrl Pts',(4.91580097596841,-23.1732062888284,0.873368878532235));
#87036=CARTESIAN_POINT('Ctrl Pts',(4.91309470690581,-23.1734112694024,0.878082103809534));
#87037=CARTESIAN_POINT('Ctrl Pts',(4.91026667614405,-23.1735877858095,0.882730584253814));
#87038=CARTESIAN_POINT('Ctrl Pts',(4.91026667737,-23.1735877838,0.576173964303));
#87039=CARTESIAN_POINT('Ctrl Pts',(4.88018105555,-23.1755928914,0.588686362769));
#87040=CARTESIAN_POINT('Ctrl Pts',(4.84922086633,-23.1643052,0.60122606158));
#87041=CARTESIAN_POINT('Ctrl Pts',(4.8242027202,-23.1390769384,0.610953205678));
#87042=CARTESIAN_POINT('Ctrl Pts',(4.81160443883,-23.1064403334,0.615349194696));
#87043=CARTESIAN_POINT('Ctrl Pts',(4.81131367923,-23.073803728,0.614647241116));
#87044=CARTESIAN_POINT('Ctrl Pts',(4.90856932846,-23.173693728,0.573384000981));
#87045=CARTESIAN_POINT('Ctrl Pts',(4.87856388841,-23.175529429,0.585854696056));
#87046=CARTESIAN_POINT('Ctrl Pts',(4.84776070495,-23.1641492947,0.59835079987));
#87047=CARTESIAN_POINT('Ctrl Pts',(4.82291574931,-23.138950008,0.608060057838));
#87048=CARTESIAN_POINT('Ctrl Pts',(4.81041826051,-23.1064121826,0.612485507872));
#87049=CARTESIAN_POINT('Ctrl Pts',(4.81015267804,-23.073874357,0.611844336315));
#87050=CARTESIAN_POINT('Ctrl Pts',(4.90687289735,-23.1737878802,0.570594502155));
#87051=CARTESIAN_POINT('Ctrl Pts',(4.87694893964,-23.1754557109,0.583023975772));
#87052=CARTESIAN_POINT('Ctrl Pts',(4.8463027189,-23.1639847944,0.595476889953));
#87053=CARTESIAN_POINT('Ctrl Pts',(4.82162983017,-23.138815193,0.605168197316));
#87054=CARTESIAN_POINT('Ctrl Pts',(4.80923231893,-23.1063761589,0.609622392402));
#87055=CARTESIAN_POINT('Ctrl Pts',(4.80899154105,-23.0739371247,0.609041103626));
#87056=CARTESIAN_POINT('Ctrl Pts',(4.90517741318,-23.173870363,0.567805508191));
#87057=CARTESIAN_POINT('Ctrl Pts',(4.87533620313,-23.1753718603,0.580194220924));
#87058=CARTESIAN_POINT('Ctrl Pts',(4.84484688747,-23.1638118024,0.59260433356));
#87059=CARTESIAN_POINT('Ctrl Pts',(4.82034495602,-23.1386725836,0.602277625735));
#87060=CARTESIAN_POINT('Ctrl Pts',(4.80804662282,-23.1063323483,0.606759869239));
#87061=CARTESIAN_POINT('Ctrl Pts',(4.80783028602,-23.0739921129,0.606237585981));
#87062=CARTESIAN_POINT('Ctrl Pts',(4.90348289858,-23.1739412934,0.56501704892));
#87063=CARTESIAN_POINT('Ctrl Pts',(4.87372566819,-23.1752779933,0.577365441412));
#87064=CARTESIAN_POINT('Ctrl Pts',(4.84339318703,-23.163630415,0.589733124619));
#87065=CARTESIAN_POINT('Ctrl Pts',(4.81906111697,-23.138522264,0.599388336927));
#87066=CARTESIAN_POINT('Ctrl Pts',(4.80686117717,-23.106280832,0.603897950258));
#87067=CARTESIAN_POINT('Ctrl Pts',(4.80666892643,-23.0740393999,0.603433815923));
#87068=CARTESIAN_POINT('Origin',(4.75289906745657,-22.5762659927124,0.262522382627455));
#87069=CARTESIAN_POINT('Origin',(3.67394039744E-17,-22.8742356128,0.729452270839));
#87070=CARTESIAN_POINT('',(5.08448267152,-22.8742356128,1.78529520144));
#87071=CARTESIAN_POINT('Origin',(3.67394039744E-17,-22.8742356128,0.729452270839));
#87072=CARTESIAN_POINT('',(4.79074910795,-23.1742356128,1.72429853244));
#87073=CARTESIAN_POINT('Origin',(4.79074910795,-22.8742356128,1.72429853244));
#87074=CARTESIAN_POINT('Origin',(3.42702565972E-16,-23.1742356128,0.729452270839));
#87075=CARTESIAN_POINT('Origin',(5.92013962829,-22.8742356128,1.84629187045));
#87076=CARTESIAN_POINT('',(5.92013962829,-22.8742356128,2.14629187045));
#87077=CARTESIAN_POINT('Origin',(5.92013962829,-22.8742356128,1.84629187045));
#87078=CARTESIAN_POINT('',(5.92013962829,-23.1742356128,2.44629187045));
#87079=CARTESIAN_POINT('Origin',(5.92013962829,-23.1742356128,1.84629187045));
#87080=CARTESIAN_POINT('Origin',(5.92013962829,-22.8742356128,2.44629187045));
#87081=CARTESIAN_POINT('Origin',(5.3782162351,-22.8742356128,1.84629187045));
#87082=CARTESIAN_POINT('',(5.3782162351,-22.8742356128,2.14629187045));
#87083=CARTESIAN_POINT('Origin',(5.3782162351,-22.8742356128,1.84629187045));
#87084=CARTESIAN_POINT('',(5.3782162351,-23.1742356128,2.44629187045));
#87085=CARTESIAN_POINT('Origin',(5.3782162351,-22.8742356128,2.44629187045));
#87086=CARTESIAN_POINT('Origin',(5.3782162351,-23.1742356128,1.84629187045));
#87087=CARTESIAN_POINT('Origin',(-6.6707290414,-22.8742356128,2.44629187045));
#87088=CARTESIAN_POINT('',(5.6491779317,-22.8742356128,2.14629187045));
#87089=CARTESIAN_POINT('',(5.6491779317,-23.1742356128,2.44629187045));
#87090=CARTESIAN_POINT('Ctrl Pts',(3.32455716278,-23.1742356021,4.31948231426));
#87091=CARTESIAN_POINT('Ctrl Pts',(3.31253480425,-23.1742356,4.29045777775));
#87092=CARTESIAN_POINT('Ctrl Pts',(3.30051244632,-23.1618985927,4.26143324199));
#87093=CARTESIAN_POINT('Ctrl Pts',(3.29100997816,-23.1370674502,4.23849225662));
#87094=CARTESIAN_POINT('Ctrl Pts',(3.286288811,-23.1056515239,4.22709435078));
#87095=CARTESIAN_POINT('Ctrl Pts',(3.28628881314,-23.0742355991,4.22709435413));
#87096=CARTESIAN_POINT('Ctrl Pts',(3.33237220301,-23.1742356053,4.31756634569));
#87097=CARTESIAN_POINT('Ctrl Pts',(3.32025642721,-23.1746190551,4.28831627923));
#87098=CARTESIAN_POINT('Ctrl Pts',(3.30803156137,-23.1624737743,4.2589484119));
#87099=CARTESIAN_POINT('Ctrl Pts',(3.29827624952,-23.1375556797,4.23568999186));
#87100=CARTESIAN_POINT('Ctrl Pts',(3.29335065691,-23.1058956405,4.22416923905));
#87101=CARTESIAN_POINT('Ctrl Pts',(3.29321960366,-23.0742356024,4.2242235267));
#87102=CARTESIAN_POINT('Ctrl Pts',(3.34019442079,-23.1741720972,4.31565197173));
#87103=CARTESIAN_POINT('Ctrl Pts',(3.32799114296,-23.1749477738,4.28617934444));
#87104=CARTESIAN_POINT('Ctrl Pts',(3.31556450024,-23.1630030812,4.25646636599));
#87105=CARTESIAN_POINT('Ctrl Pts',(3.30555189312,-23.138001656,4.23288657883));
#87106=CARTESIAN_POINT('Ctrl Pts',(3.30041646177,-23.1060974603,4.22124248791));
#87107=CARTESIAN_POINT('Ctrl Pts',(3.30014990602,-23.0741932655,4.22135290147));
#87108=CARTESIAN_POINT('Ctrl Pts',(3.3480232941,-23.1740438599,4.31373927334));
#87109=CARTESIAN_POINT('Ctrl Pts',(3.33573882686,-23.1752205531,4.28404716821));
#87110=CARTESIAN_POINT('Ctrl Pts',(3.3231113604,-23.1634855096,4.25398729437));
#87111=CARTESIAN_POINT('Ctrl Pts',(3.3128368906,-23.1384045129,4.23008209497));
#87112=CARTESIAN_POINT('Ctrl Pts',(3.30748597263,-23.1062561443,4.218314202));
#87113=CARTESIAN_POINT('Ctrl Pts',(3.3070792575,-23.074107776,4.21848267011));
#87114=CARTESIAN_POINT('Ctrl Pts',(3.35585826297,-23.1738495698,4.31182834003));
#87115=CARTESIAN_POINT('Ctrl Pts',(3.34349934911,-23.1754360753,4.28191995536));
#87116=CARTESIAN_POINT('Ctrl Pts',(3.33067225204,-23.1639199594,4.25151138948));
#87117=CARTESIAN_POINT('Ctrl Pts',(3.32013123785,-23.1387632939,4.22727661933));
#87118=CARTESIAN_POINT('Ctrl Pts',(3.31455892719,-23.1063707724,4.21538448948));
#87119=CARTESIAN_POINT('Ctrl Pts',(3.31400716536,-23.0739782508,4.21561303671));
#87120=CARTESIAN_POINT('Ctrl Pts',(3.36369873711,-23.1735877856,4.30991926812));
#87121=CARTESIAN_POINT('Ctrl Pts',(3.35127259083,-23.1755928932,4.2797979179));
#87122=CARTESIAN_POINT('Ctrl Pts',(3.33824733642,-23.1643052014,4.24903885097));
#87123=CARTESIAN_POINT('Ctrl Pts',(3.32743496442,-23.1390769393,4.22447021973));
#87124=CARTESIAN_POINT('Ctrl Pts',(3.32163506784,-23.1064403336,4.21245345605));
#87125=CARTESIAN_POINT('Ctrl Pts',(3.32093311398,-23.073803728,4.21274421486));
#87126=CARTESIAN_POINT('',(3.36369873258,-23.1735877857,4.30991926955));
#87127=CARTESIAN_POINT('Origin',(3.35893957337299,-23.074577514808,4.30445285837843));
#87128=CARTESIAN_POINT('',(3.32455716483031,-23.17423560745,4.3194823125052));
#87129=CARTESIAN_POINT('Origin',(3.09652469257192,-22.6950826646314,4.39942546521357));
#87130=CARTESIAN_POINT('Origin',(3.32428656951706,-23.0749427241466,4.31882903140108));
#87131=CARTESIAN_POINT('Ctrl Pts',(3.36368929336556,-23.1735838355436,4.3100097843108));
#87132=CARTESIAN_POINT('Ctrl Pts',(3.35126126667731,-23.1756159753277,4.27987369799882));
#87133=CARTESIAN_POINT('Ctrl Pts',(3.33822971249265,-23.1643432723425,4.24908904885602));
#87134=CARTESIAN_POINT('Ctrl Pts',(3.32741010276691,-23.1391098819976,4.22449481546317));
#87135=CARTESIAN_POINT('Ctrl Pts',(3.32160668783934,-23.1064572814787,4.21246529856621));
#87136=CARTESIAN_POINT('Ctrl Pts',(3.3209049569083,-23.0738046795702,4.21275587774604));
#87137=CARTESIAN_POINT('Ctrl Pts',(3.42727587068037,-23.1714537891356,4.29453895824509));
#87138=CARTESIAN_POINT('Ctrl Pts',(3.40968612110659,-23.1770054655411,4.26451318049342));
#87139=CARTESIAN_POINT('Ctrl Pts',(3.39042512741839,-23.1676522631102,4.23271832267249));
#87140=CARTESIAN_POINT('Ctrl Pts',(3.3738386086957,-23.1418126390217,4.20685865723294));
#87141=CARTESIAN_POINT('Ctrl Pts',(3.36461849949685,-23.1071018108388,4.19452950363387));
#87142=CARTESIAN_POINT('Ctrl Pts',(3.36302228471092,-23.0723909633791,4.1953153506082));
#87143=CARTESIAN_POINT('Ctrl Pts',(3.48602780500958,-23.1658533405815,4.26387171240888));
#87144=CARTESIAN_POINT('Ctrl Pts',(3.46327855666835,-23.1744319191555,4.23600234342951));
#87145=CARTESIAN_POINT('Ctrl Pts',(3.43787192065916,-23.1670366207478,4.20539868415393));
#87146=CARTESIAN_POINT('Ctrl Pts',(3.41599585681065,-23.1410190434613,4.1799814558232));
#87147=CARTESIAN_POINT('Ctrl Pts',(3.40455618145493,-23.1048410962315,4.16807249384115));
#87148=CARTESIAN_POINT('Ctrl Pts',(3.40366050713365,-23.068663043311,4.16911644023449));
#87149=CARTESIAN_POINT('Ctrl Pts',(3.53441735913858,-23.1658531413152,4.21548783590638));
#87150=CARTESIAN_POINT('Ctrl Pts',(3.50654749801918,-23.1744321561296,4.19273743139755));
#87151=CARTESIAN_POINT('Ctrl Pts',(3.47594318930563,-23.1670368001775,4.16732946763638));
#87152=CARTESIAN_POINT('Ctrl Pts',(3.45052561848652,-23.1410185073567,4.14545234848626));
#87153=CARTESIAN_POINT('Ctrl Pts',(3.43861708176451,-23.1048397492347,4.13401229478962));
#87154=CARTESIAN_POINT('Ctrl Pts',(3.43966196606321,-23.0686612727428,4.1331168715304));
#87155=CARTESIAN_POINT('Ctrl Pts',(3.56508656734137,-23.1714537839891,4.15672855586756));
#87156=CARTESIAN_POINT('Ctrl Pts',(3.53506076659917,-23.1770054815344,4.13913874792724));
#87157=CARTESIAN_POINT('Ctrl Pts',(3.50326587807461,-23.1676522759815,4.11987768748972));
#87158=CARTESIAN_POINT('Ctrl Pts',(3.47740619605725,-23.1418126154361,4.10329111307365));
#87159=CARTESIAN_POINT('Ctrl Pts',(3.46507706381281,-23.1071017471307,4.09407098400021));
#87160=CARTESIAN_POINT('Ctrl Pts',(3.46586295657012,-23.0723908784742,4.09247478015265));
#87161=CARTESIAN_POINT('Ctrl Pts',(3.58055751223848,-23.1735838358499,4.09314156852285));
#87162=CARTESIAN_POINT('Ctrl Pts',(3.55042142397976,-23.1756159758171,4.08071353967926));
#87163=CARTESIAN_POINT('Ctrl Pts',(3.51963677274451,-23.1643432719327,4.06768198311457));
#87164=CARTESIAN_POINT('Ctrl Pts',(3.495042538531,-23.13910987911,4.05686237170097));
#87165=CARTESIAN_POINT('Ctrl Pts',(3.48301302329125,-23.1064572763175,4.05105895662086));
#87166=CARTESIAN_POINT('Ctrl Pts',(3.48330360576356,-23.0738046736254,4.05035722683515));
#87167=CARTESIAN_POINT('',(3.58046699021159,-23.1735877810644,4.09315100260664));
#87168=CARTESIAN_POINT('Origin',(3.5750005834412,-23.0745775165868,4.08839183728771));
#87169=CARTESIAN_POINT('Ctrl Pts',(3.58046699304039,-23.1735877859444,4.09315100345836));
#87170=CARTESIAN_POINT('Ctrl Pts',(3.57658526578705,-23.1730554985274,4.10909309137931));
#87171=CARTESIAN_POINT('Ctrl Pts',(3.57151986290398,-23.1722659160818,4.1246716419425));
#87172=CARTESIAN_POINT('Ctrl Pts',(3.5652798453657,-23.1714622614676,4.13968656724023));
#87173=CARTESIAN_POINT('Ctrl Pts',(3.55956845646456,-23.170726689169,4.15342948978343));
#87174=CARTESIAN_POINT('Ctrl Pts',(3.55287415413697,-23.1699801491101,4.16670101052127));
#87175=CARTESIAN_POINT('Ctrl Pts',(3.5452204080535,-23.1693713921876,4.17935434371679));
#87176=CARTESIAN_POINT('Ctrl Pts',(3.54029406542148,-23.1689795650814,4.18749867644987));
#87177=CARTESIAN_POINT('Ctrl Pts',(3.53497051338374,-23.1686440328199,4.19538699940324));
#87178=CARTESIAN_POINT('Ctrl Pts',(3.52925723559328,-23.1683928406018,4.20297976398894));
#87179=CARTESIAN_POINT('Ctrl Pts',(3.52110035296887,-23.1680342118927,4.2138200017284));
#87180=CARTESIAN_POINT('Ctrl Pts',(3.51217014253913,-23.1678467659713,4.22405966720967));
#87181=CARTESIAN_POINT('Ctrl Pts',(3.50254971355978,-23.1678573637056,4.2336041965472));
#87182=CARTESIAN_POINT('Ctrl Pts',(3.50033236766523,-23.1678598063038,4.23580404886016));
#87183=CARTESIAN_POINT('Ctrl Pts',(3.49807833812036,-23.1678725531436,4.2379669522243));
#87184=CARTESIAN_POINT('Ctrl Pts',(3.4957886085378,-23.1678955415342,4.24009170920016));
#87185=CARTESIAN_POINT('Ctrl Pts',(3.48545965182566,-23.1679992420294,4.24967647545144));
#87186=CARTESIAN_POINT('Ctrl Pts',(3.47439638442631,-23.1683223884004,4.25845019369705));
#87187=CARTESIAN_POINT('Ctrl Pts',(3.46272764401182,-23.1688045362578,4.26637644567551));
#87188=CARTESIAN_POINT('Ctrl Pts',(3.45046583703957,-23.1693111893969,4.27470555133053));
#87189=CARTESIAN_POINT('Ctrl Pts',(3.43753502135603,-23.1699928747773,4.28209828027822));
#87190=CARTESIAN_POINT('Ctrl Pts',(3.42407993887611,-23.170719673524,4.28851360926196));
#87191=CARTESIAN_POINT('Ctrl Pts',(3.40973489722923,-23.1714945449011,4.29535326718213));
#87192=CARTESIAN_POINT('Ctrl Pts',(3.39479315367958,-23.1723199471667,4.30108085339101));
#87193=CARTESIAN_POINT('Ctrl Pts',(3.37943451815742,-23.1729820221765,4.30566133260555));
#87194=CARTESIAN_POINT('Ctrl Pts',(3.374234505679,-23.1732061826046,4.30721215715884));
#87195=CARTESIAN_POINT('Ctrl Pts',(3.36898679610344,-23.1734112234077,4.30863168405366));
#87196=CARTESIAN_POINT('Ctrl Pts',(3.36369873257884,-23.1735877856743,4.30991926954876));
#87197=CARTESIAN_POINT('Ctrl Pts',(3.58046698701,-23.1735877712,4.09315099924));
#87198=CARTESIAN_POINT('Ctrl Pts',(3.55034564212,-23.1755928789,4.0807248569));
#87199=CARTESIAN_POINT('Ctrl Pts',(3.51958658051,-23.1643051888,4.06769960633));
#87200=CARTESIAN_POINT('Ctrl Pts',(3.49501795255,-23.13907693,4.05688723684));
#87201=CARTESIAN_POINT('Ctrl Pts',(3.48300118847,-23.1064403276,4.05108734042));
#87202=CARTESIAN_POINT('Ctrl Pts',(3.48329194402,-23.073803724,4.05038538482));
#87203=CARTESIAN_POINT('Ctrl Pts',(3.58237609938,-23.1738495633,4.08531036606));
#87204=CARTESIAN_POINT('Ctrl Pts',(3.55246772359,-23.1754360605,4.07295145689));
#87205=CARTESIAN_POINT('Ctrl Pts',(3.52205916937,-23.1639199413,4.06012436711));
#87206=CARTESIAN_POINT('Ctrl Pts',(3.49782440883,-23.1387632801,4.0495833606));
#87207=CARTESIAN_POINT('Ctrl Pts',(3.48593228125,-23.1063707663,4.04401105478));
#87208=CARTESIAN_POINT('Ctrl Pts',(3.48616082452,-23.0739782513,4.04345929461));
#87209=CARTESIAN_POINT('Ctrl Pts',(3.58428706187,-23.1740438603,4.0774752762));
#87210=CARTESIAN_POINT('Ctrl Pts',(3.55459496917,-23.1752205389,4.06519081505));
#87211=CARTESIAN_POINT('Ctrl Pts',(3.52453511246,-23.1634854888,4.05256335909));
#87212=CARTESIAN_POINT('Ctrl Pts',(3.50062992774,-23.1384044972,4.0422889011));
#87213=CARTESIAN_POINT('Ctrl Pts',(3.48886203891,-23.1062561396,4.03693799135));
#87214=CARTESIAN_POINT('Ctrl Pts',(3.48903050209,-23.0741077812,4.0365312801));
#87215=CARTESIAN_POINT('Ctrl Pts',(3.58619975923,-23.1741721033,4.06964640553));
#87216=CARTESIAN_POINT('Ctrl Pts',(3.55672714472,-23.1749477659,4.05744313429));
#87217=CARTESIAN_POINT('Ctrl Pts',(3.52701418337,-23.1630030668,4.04501650225));
#87218=CARTESIAN_POINT('Ctrl Pts',(3.50343441064,-23.1380016463,4.03500390673));
#87219=CARTESIAN_POINT('Ctrl Pts',(3.49179032375,-23.1060974606,4.02986848333));
#87220=CARTESIAN_POINT('Ctrl Pts',(3.49190073237,-23.0741932746,4.02960193123));
#87221=CARTESIAN_POINT('Ctrl Pts',(3.58811409552,-23.1742356128,4.0618243387));
#87222=CARTESIAN_POINT('Ctrl Pts',(3.5588640379,-23.1746190563,4.04970856814));
#87223=CARTESIAN_POINT('Ctrl Pts',(3.52949618126,-23.162473773,4.03748370929));
#87224=CARTESIAN_POINT('Ctrl Pts',(3.50623776954,-23.1375556813,4.02772840414));
#87225=CARTESIAN_POINT('Ctrl Pts',(3.49471701837,-23.1058956471,4.02280281538));
#87226=CARTESIAN_POINT('Ctrl Pts',(3.49477130203,-23.0742356128,4.02267176303));
#87227=CARTESIAN_POINT('Ctrl Pts',(3.59003001961,-23.1742356128,4.0540094681));
#87228=CARTESIAN_POINT('Ctrl Pts',(3.56100548808,-23.1742356128,4.0419871135));
#87229=CARTESIAN_POINT('Ctrl Pts',(3.53198095656,-23.1618986073,4.02996475891));
#87230=CARTESIAN_POINT('Ctrl Pts',(3.50903997323,-23.1370674659,4.02046229248));
#87231=CARTESIAN_POINT('Ctrl Pts',(3.49764206635,-23.1056515394,4.01574112487));
#87232=CARTESIAN_POINT('Ctrl Pts',(3.49764206635,-23.0742356128,4.01574112487));
#87233=CARTESIAN_POINT('',(3.59003001961,-23.1742356128,4.0540094681));
#87234=CARTESIAN_POINT('Origin',(3.58937674712371,-23.0749427098877,4.05373887377641));
#87235=CARTESIAN_POINT('Origin',(3.67125418556151,-22.686923854516,3.82239309382983));
#87236=CARTESIAN_POINT('Origin',(-8.51439015726E-16,-22.8742356128,0.729452270839));
#87237=CARTESIAN_POINT('',(3.96612236541,-23.1742356128,3.59491374888));
#87238=CARTESIAN_POINT('Origin',(3.42702565972E-16,-23.1742356128,0.729452270839));
#87239=CARTESIAN_POINT('',(4.2092958712,-22.8742356128,3.77060280966));
#87240=CARTESIAN_POINT('Origin',(3.96612236541,-22.8742356128,3.59491374888));
#87241=CARTESIAN_POINT('',(3.13117783752,-22.8742356128,4.87221628548));
#87242=CARTESIAN_POINT('Origin',(3.67394039744E-17,-22.8742356128,0.729452270839));
#87243=CARTESIAN_POINT('',(2.95028784657,-23.1742356128,4.63288636429));
#87244=CARTESIAN_POINT('Origin',(2.95028784657,-22.8742356128,4.63288636429));
#87245=CARTESIAN_POINT('Origin',(3.42702565972E-16,-23.1742356128,0.729452270839));
#87246=CARTESIAN_POINT('Origin',(3.31206782846,-22.8742356128,5.11154620667));
#87247=CARTESIAN_POINT('',(2.90473307408,-23.1742356128,5.55208950519));
#87248=CARTESIAN_POINT('Origin',(3.31206782846,-23.1742356128,5.11154620667));
#87249=CARTESIAN_POINT('',(3.10840045127,-22.8742356128,5.33181785593));
#87250=CARTESIAN_POINT('Origin',(3.31206782846,-22.8742356128,5.11154620667));
#87251=CARTESIAN_POINT('Origin',(2.90473307408,-22.8742356128,5.55208950519));
#87252=CARTESIAN_POINT('Origin',(6.6707290414,-22.8742356128,9.03420135995));
#87253=CARTESIAN_POINT('',(4.51260368036,-23.1742356128,7.03875740065));
#87254=CARTESIAN_POINT('',(3.70866837722,-23.1742356128,6.29542345292));
#87255=CARTESIAN_POINT('',(4.71627105755,-22.8742356128,6.81848575139));
#87256=CARTESIAN_POINT('',(3.91233575441,-22.8742356128,6.07515180366));
#87257=CARTESIAN_POINT('Origin',(4.51260368036,-22.8742356128,7.03875740065));
#87258=CARTESIAN_POINT('Origin',(4.91993843473,-22.8742356128,6.59821410213));
#87259=CARTESIAN_POINT('',(5.40800342362,-23.1742356128,6.94720201972));
#87260=CARTESIAN_POINT('Origin',(4.91993843473,-23.1742356128,6.59821410213));
#87261=CARTESIAN_POINT('',(5.16397092918,-22.8742356128,6.77270806092));
#87262=CARTESIAN_POINT('Origin',(4.91993843473,-22.8742356128,6.59821410213));
#87263=CARTESIAN_POINT('Origin',(5.40800342362,-22.8742356128,6.94720201972));
#87264=CARTESIAN_POINT('Origin',(0.00234331738835,-22.8742356128,3.08191746407));
#87265=CARTESIAN_POINT('',(6.57948381998,-23.1742356128,4.03207991826));
#87266=CARTESIAN_POINT('Origin',(0.00234331738835,-23.1742356128,3.08191746407));
#87267=CARTESIAN_POINT('',(6.28256615006,-22.8742356128,3.98918589435));
#87268=CARTESIAN_POINT('Origin',(0.00234331738835,-22.8742356128,3.08191746407));
#87269=CARTESIAN_POINT('Origin',(6.57948381998,-22.8742356128,4.03207991826));
#87270=CARTESIAN_POINT('Origin',(4.452469377,-22.8742356128,3.94629187045));
#87271=CARTESIAN_POINT('',(4.452469377,-23.1742356128,3.34629187045));
#87272=CARTESIAN_POINT('Origin',(4.452469377,-23.1742356128,3.94629187045));
#87273=CARTESIAN_POINT('',(4.452469377,-22.8742356128,3.64629187045));
#87274=CARTESIAN_POINT('Origin',(4.452469377,-22.8742356128,3.34629187045));
#87275=CARTESIAN_POINT('Origin',(4.452469377,-22.8742356128,3.94629187045));
#87276=CARTESIAN_POINT('Origin',(5.98564848014,-22.8742356128,3.94629187045));
#87277=CARTESIAN_POINT('',(5.98564848014,-23.1742356128,3.34629187045));
#87278=CARTESIAN_POINT('Origin',(5.98564848014,-23.1742356128,3.94629187045));
#87279=CARTESIAN_POINT('',(5.98564848014,-22.8742356128,3.64629187045));
#87280=CARTESIAN_POINT('Origin',(5.98564848014,-22.8742356128,3.94629187045));
#87281=CARTESIAN_POINT('Origin',(5.98564848014,-22.8742356128,3.34629187045));
#87282=CARTESIAN_POINT('Origin',(-6.6707290414,-22.8742356128,3.34629187045));
#87283=CARTESIAN_POINT('',(5.21905892857,-23.1742356128,3.34629187045));
#87284=CARTESIAN_POINT('',(5.21905892857,-22.8742356128,3.64629187045));
#87285=CARTESIAN_POINT('Origin',(4.1372329486,-21.0742356128,5.87450964899));
#87286=CARTESIAN_POINT('',(3.31206782846,-20.7742356128,5.11154620667));
#87287=CARTESIAN_POINT('',(4.91993843473,-20.7742356128,6.59821410213));
#87288=CARTESIAN_POINT('',(4.1160031316,-20.7742356128,5.8548801544));
#87289=CARTESIAN_POINT('',(4.71627105755,-21.0742356128,6.81848575139));
#87290=CARTESIAN_POINT('Origin',(4.91993843473344,-21.0742356128,6.59821410212948));
#87291=CARTESIAN_POINT('',(3.10840045127,-21.0742356128,5.33181785593));
#87292=CARTESIAN_POINT('',(3.91233575441,-21.0742356128,6.07515180366));
#87293=CARTESIAN_POINT('Ctrl Pts',(3.31206782846,-20.7742356128,5.11154620667));
#87294=CARTESIAN_POINT('Ctrl Pts',(3.30444954029279,-20.7742356127999,5.1197855865974));
#87295=CARTESIAN_POINT('Ctrl Pts',(3.2973316880372,-20.7748629748481,5.12745413063611));
#87296=CARTESIAN_POINT('Ctrl Pts',(3.29076617355475,-20.7758767399775,5.13452932895326));
#87297=CARTESIAN_POINT('Ctrl Pts',(3.28578446329595,-20.7766459537473,5.13989777161435));
#87298=CARTESIAN_POINT('Ctrl Pts',(3.28111988686524,-20.7776380915859,5.14492554135016));
#87299=CARTESIAN_POINT('Ctrl Pts',(3.27678437271589,-20.7787599076263,5.14961442549687));
#87300=CARTESIAN_POINT('Ctrl Pts',(3.27175967701396,-20.7800600496722,5.15504866356119));
#87301=CARTESIAN_POINT('Ctrl Pts',(3.26717209828427,-20.781533969113,5.16002543626601));
#87302=CARTESIAN_POINT('Ctrl Pts',(3.26300921844094,-20.7830586640124,5.16454845869607));
#87303=CARTESIAN_POINT('Ctrl Pts',(3.26120731138153,-20.7837186298548,5.16650625386511));
#87304=CARTESIAN_POINT('Ctrl Pts',(3.25974366013668,-20.784288939405,5.16809834768708));
#87305=CARTESIAN_POINT('Ctrl Pts',(3.25827854408097,-20.7848814548452,5.16969158096989));
#87306=CARTESIAN_POINT('Ctrl Pts',(3.25686452541498,-20.7854533057161,5.17122924864638));
#87307=CARTESIAN_POINT('Ctrl Pts',(3.25544907274139,-20.7860461299659,5.17276805295182));
#87308=CARTESIAN_POINT('Ctrl Pts',(3.25373460238829,-20.7868025675846,5.17462932065643));
#87309=CARTESIAN_POINT('Ctrl Pts',(3.25312148822844,-20.7870730783078,5.17529493122409));
#87310=CARTESIAN_POINT('Ctrl Pts',(3.25247021809243,-20.7873649214208,5.17600168928286));
#87311=CARTESIAN_POINT('Ctrl Pts',(3.25176754480936,-20.7876862654106,5.17676389831576));
#87312=CARTESIAN_POINT('Ctrl Pts',(3.24593338674452,-20.7903543213548,5.18309237000166));
#87313=CARTESIAN_POINT('Ctrl Pts',(3.24018276622,-20.793407990483,5.18930426249853));
#87314=CARTESIAN_POINT('Ctrl Pts',(3.23463241100123,-20.7967643371934,5.19529253398549));
#87315=CARTESIAN_POINT('Ctrl Pts',(3.22898905056823,-20.800176924943,5.20138114868485));
#87316=CARTESIAN_POINT('Ctrl Pts',(3.22355313365751,-20.8039018958713,5.20723814141231));
#87317=CARTESIAN_POINT('Ctrl Pts',(3.21842848080822,-20.8078052624877,5.21277141141798));
#87318=CARTESIAN_POINT('Ctrl Pts',(3.21304718125325,-20.8119041128203,5.21858179200272));
#87319=CARTESIAN_POINT('Ctrl Pts',(3.20800942685562,-20.8161989110882,5.22403486325186));
#87320=CARTESIAN_POINT('Ctrl Pts',(3.20340861986728,-20.8204929579054,5.22905297895093));
#87321=CARTESIAN_POINT('Ctrl Pts',(3.20280377184362,-20.8210574775076,5.22971268873028));
#87322=CARTESIAN_POINT('Ctrl Pts',(3.20220643643071,-20.8216219388458,5.23036492352408));
#87323=CARTESIAN_POINT('Ctrl Pts',(3.20161679072966,-20.822185857569,5.23100954489473));
#87324=CARTESIAN_POINT('Ctrl Pts',(3.19343867455265,-20.83000715233,5.23995014846391));
#87325=CARTESIAN_POINT('Ctrl Pts',(3.18586912350675,-20.8384449654876,5.24814241044823));
#87326=CARTESIAN_POINT('Ctrl Pts',(3.1789329133062,-20.8472632641887,5.25562483465526));
#87327=CARTESIAN_POINT('Ctrl Pts',(3.1743793788751,-20.8530523659601,5.260536951686));
#87328=CARTESIAN_POINT('Ctrl Pts',(3.17009808891465,-20.8590060228511,5.26514391381523));
#87329=CARTESIAN_POINT('Ctrl Pts',(3.16608953990945,-20.8650648258508,5.26946365924601));
#87330=CARTESIAN_POINT('Ctrl Pts',(3.16283874769359,-20.8699783019249,5.27296682081462));
#87331=CARTESIAN_POINT('Ctrl Pts',(3.15985829370293,-20.8748159171735,5.2761818264669));
#87332=CARTESIAN_POINT('Ctrl Pts',(3.15704171944077,-20.8796807375898,5.27922240091002));
#87333=CARTESIAN_POINT('Ctrl Pts',(3.15406822274213,-20.8848165962964,5.28243237772125));
#87334=CARTESIAN_POINT('Ctrl Pts',(3.15127701135179,-20.8899831652855,5.285448338928));
#87335=CARTESIAN_POINT('Ctrl Pts',(3.14857270050314,-20.8953444206099,5.28837178313741));
#87336=CARTESIAN_POINT('Ctrl Pts',(3.14600766127337,-20.9004295720579,5.29114467039145));
#87337=CARTESIAN_POINT('Ctrl Pts',(3.1435207243353,-20.9056904954052,5.29383440885434));
#87338=CARTESIAN_POINT('Ctrl Pts',(3.14105900613626,-20.9112961454075,5.29649677480764));
#87339=CARTESIAN_POINT('Ctrl Pts',(3.14092534444609,-20.9116005103238,5.29664133088773));
#87340=CARTESIAN_POINT('Ctrl Pts',(3.14079176474627,-20.9119058977849,5.29678579800486));
#87341=CARTESIAN_POINT('Ctrl Pts',(3.14065826128172,-20.9122123369602,5.29693018215617));
#87342=CARTESIAN_POINT('Ctrl Pts',(3.13742614659444,-20.9196312197803,5.30042571792873));
#87343=CARTESIAN_POINT('Ctrl Pts',(3.13478487531432,-20.9266420183846,5.30348849201042));
#87344=CARTESIAN_POINT('Ctrl Pts',(3.13253832728671,-20.9331835477761,5.30615752340709));
#87345=CARTESIAN_POINT('Ctrl Pts',(3.13015585898119,-20.9401208516989,5.30898803610073));
#87346=CARTESIAN_POINT('Ctrl Pts',(3.12821700234919,-20.9465310459643,5.31137606597068));
#87347=CARTESIAN_POINT('Ctrl Pts',(3.12651001133026,-20.952389618554,5.31334417593453));
#87348=CARTESIAN_POINT('Ctrl Pts',(3.12602179849174,-20.9540652163293,5.31390707084219));
#87349=CARTESIAN_POINT('Ctrl Pts',(3.12555269902518,-20.9556959443761,5.31443545748816));
#87350=CARTESIAN_POINT('Ctrl Pts',(3.12509810909517,-20.9572817858397,5.31492948511653));
#87351=CARTESIAN_POINT('Ctrl Pts',(3.12366652371443,-20.9622758855889,5.31648526689644));
#87352=CARTESIAN_POINT('Ctrl Pts',(3.12229520001995,-20.9671617422919,5.31782333881145));
#87353=CARTESIAN_POINT('Ctrl Pts',(3.12097486219589,-20.9721576961734,5.31906465725106));
#87354=CARTESIAN_POINT('Ctrl Pts',(3.11969224644078,-20.9770109155871,5.32027051120657));
#87355=CARTESIAN_POINT('Ctrl Pts',(3.11845767571797,-20.9819684491287,5.32138513596453));
#87356=CARTESIAN_POINT('Ctrl Pts',(3.11729333615592,-20.9872457021546,5.32248622269787));
#87357=CARTESIAN_POINT('Ctrl Pts',(3.11669009887985,-20.9899798149892,5.32305668906645));
#87358=CARTESIAN_POINT('Ctrl Pts',(3.11610622112494,-20.992799963711,5.32362297214742));
#87359=CARTESIAN_POINT('Ctrl Pts',(3.11554850316912,-20.99573729042,5.32419185848304));
#87360=CARTESIAN_POINT('Ctrl Pts',(3.11424881632856,-21.0025823360749,5.32551757173375));
#87361=CARTESIAN_POINT('Ctrl Pts',(3.11320374618487,-21.0090749065193,5.32659990756699));
#87362=CARTESIAN_POINT('Ctrl Pts',(3.11233787825752,-21.015348475393,5.32750975261846));
#87363=CARTESIAN_POINT('Ctrl Pts',(3.11142278559847,-21.0219786976718,5.32847132250826));
#87364=CARTESIAN_POINT('Ctrl Pts',(3.11070786593494,-21.0283649245797,5.3292402142949));
#87365=CARTESIAN_POINT('Ctrl Pts',(3.11014076856595,-21.0346836372789,5.32986044423484));
#87366=CARTESIAN_POINT('Ctrl Pts',(3.10956040449569,-21.0411501702262,5.33049518386179));
#87367=CARTESIAN_POINT('Ctrl Pts',(3.10913483212844,-21.0475465887847,5.3309742547607));
#87368=CARTESIAN_POINT('Ctrl Pts',(3.10884490269887,-21.0540718430784,5.33130485910088));
#87369=CARTESIAN_POINT('Ctrl Pts',(3.1085549732693,-21.0605970973721,5.33163546344106));
#87370=CARTESIAN_POINT('Ctrl Pts',(3.10840045126752,-21.0672518011227,5.33181785593268));
#87371=CARTESIAN_POINT('Ctrl Pts',(3.10840045126752,-21.0742356128,5.33181785593268));
#87372=CARTESIAN_POINT('Origin',(2.31985562646,-21.0742356128,7.05423263334));
#87373=CARTESIAN_POINT('',(1.2614400074,-20.7742356128,6.07560132137));
#87374=CARTESIAN_POINT('',(2.33982641743,-20.7742356128,7.0726980084));
#87375=CARTESIAN_POINT('',(1.46510738459,-21.0742356128,5.8553296721));
#87376=CARTESIAN_POINT('Ctrl Pts',(1.46510738458927,-21.0742356128,5.85532967210079));
#87377=CARTESIAN_POINT('Ctrl Pts',(1.46510738458927,-21.0568525598039,5.85532967210079));
#87378=CARTESIAN_POINT('Ctrl Pts',(1.46407993726464,-21.0394747640594,5.85643142737418));
#87379=CARTESIAN_POINT('Ctrl Pts',(1.46201327225789,-21.0222270827341,5.85865552532541));
#87380=CARTESIAN_POINT('Ctrl Pts',(1.46007045121047,-21.0060129608573,5.86074634521981));
#87381=CARTESIAN_POINT('Ctrl Pts',(1.45720859993379,-20.9899122151244,5.86382970774848));
#87382=CARTESIAN_POINT('Ctrl Pts',(1.45339155089049,-20.9740554909872,5.86795125690417));
#87383=CARTESIAN_POINT('Ctrl Pts',(1.45314823539463,-20.9730447136427,5.86821398257658));
#87384=CARTESIAN_POINT('Ctrl Pts',(1.45290103120873,-20.9720349420427,5.86848093475406));
#87385=CARTESIAN_POINT('Ctrl Pts',(1.45264992608831,-20.9710262162607,5.86875212837015));
#87386=CARTESIAN_POINT('Ctrl Pts',(1.44881627744658,-20.9556258922154,5.87289247021678));
#87387=CARTESIAN_POINT('Ctrl Pts',(1.44407550231965,-20.9404672608799,5.87802193854843));
#87388=CARTESIAN_POINT('Ctrl Pts',(1.43838489826456,-20.9257392878566,5.88418724678318));
#87389=CARTESIAN_POINT('Ctrl Pts',(1.43785540916636,-20.9243689058939,5.88476090530268));
#87390=CARTESIAN_POINT('Ctrl Pts',(1.43731769652213,-20.9230022902451,5.88534353204184));
#87391=CARTESIAN_POINT('Ctrl Pts',(1.43677172643757,-20.9216396173414,5.88593516408484));
#87392=CARTESIAN_POINT('Ctrl Pts',(1.43434334506759,-20.9155786817951,5.88856664202062));
#87393=CARTESIAN_POINT('Ctrl Pts',(1.43169370618827,-20.9094594010707,5.89143919340066));
#87394=CARTESIAN_POINT('Ctrl Pts',(1.42887798388927,-20.9034620318311,5.89449111102838));
#87395=CARTESIAN_POINT('Ctrl Pts',(1.42605752021122,-20.897454563655,5.89754816776313));
#87396=CARTESIAN_POINT('Ctrl Pts',(1.42307059144137,-20.89157000063,5.90078500266657));
#87397=CARTESIAN_POINT('Ctrl Pts',(1.42000271460379,-20.8859602994751,5.90410708155958));
#87398=CARTESIAN_POINT('Ctrl Pts',(1.41804423247998,-20.8823791585058,5.90622784209538));
#87399=CARTESIAN_POINT('Ctrl Pts',(1.41605337921587,-20.8789093883557,5.90838267412748));
#87400=CARTESIAN_POINT('Ctrl Pts',(1.41405795094043,-20.8755830313655,5.91054098330808));
#87401=CARTESIAN_POINT('Ctrl Pts',(1.4084018122684,-20.8661543104036,5.91665881584196));
#87402=CARTESIAN_POINT('Ctrl Pts',(1.40212266410665,-20.8568965367214,5.92343229913557));
#87403=CARTESIAN_POINT('Ctrl Pts',(1.39518571116258,-20.848004932525,5.93092317372076));
#87404=CARTESIAN_POINT('Ctrl Pts',(1.39201468675336,-20.8439403966731,5.93434740714826));
#87405=CARTESIAN_POINT('Ctrl Pts',(1.38870645133448,-20.8399529582422,5.93792128289567));
#87406=CARTESIAN_POINT('Ctrl Pts',(1.38525918280401,-20.8360642290584,5.94164907444906));
#87407=CARTESIAN_POINT('Ctrl Pts',(1.37976491537811,-20.8298663602549,5.94759044035116));
#87408=CARTESIAN_POINT('Ctrl Pts',(1.37391644984959,-20.8239192141413,5.95392220208472));
#87409=CARTESIAN_POINT('Ctrl Pts',(1.36770932510617,-20.8183217629177,5.96064509578293));
#87410=CARTESIAN_POINT('Ctrl Pts',(1.36460576273446,-20.8155230373059,5.96400654263203));
#87411=CARTESIAN_POINT('Ctrl Pts',(1.36141262995974,-20.8128119253493,5.96746550388978));
#87412=CARTESIAN_POINT('Ctrl Pts',(1.35813001664382,-20.8102018162985,5.97102026930888));
#87413=CARTESIAN_POINT('Ctrl Pts',(1.35668689185399,-20.8090543424072,5.97258303945712));
#87414=CARTESIAN_POINT('Ctrl Pts',(1.35499698359374,-20.8077487870536,5.97441253609893));
#87415=CARTESIAN_POINT('Ctrl Pts',(1.3533601637152,-20.806528824505,5.97618421836793));
#87416=CARTESIAN_POINT('Ctrl Pts',(1.35154453585483,-20.8051755919222,5.97814944113282));
#87417=CARTESIAN_POINT('Ctrl Pts',(1.34979443131247,-20.8039277560863,5.98004330913371));
#87418=CARTESIAN_POINT('Ctrl Pts',(1.34854061399836,-20.8030538894474,5.98139963746283));
#87419=CARTESIAN_POINT('Ctrl Pts',(1.34835363857244,-20.8029235741413,5.98160189983724));
#87420=CARTESIAN_POINT('Ctrl Pts',(1.34817772561819,-20.8028014882097,5.98179218024529));
#87421=CARTESIAN_POINT('Ctrl Pts',(1.34801432321358,-20.8026884535921,5.98196891154972));
#87422=CARTESIAN_POINT('Ctrl Pts',(1.34352037500665,-20.7995797373015,5.9868294356682));
#87423=CARTESIAN_POINT('Ctrl Pts',(1.338386211841,-20.7963192960567,5.99238226897694));
#87424=CARTESIAN_POINT('Ctrl Pts',(1.33256949718929,-20.7931259090584,5.99867323712446));
#87425=CARTESIAN_POINT('Ctrl Pts',(1.32726165318095,-20.7902118929754,6.00441384493968));
#87426=CARTESIAN_POINT('Ctrl Pts',(1.32138489117724,-20.7873543342918,6.01076970044963));
#87427=CARTESIAN_POINT('Ctrl Pts',(1.31492003594937,-20.7847629028735,6.0177615707223));
#87428=CARTESIAN_POINT('Ctrl Pts',(1.30867724066184,-20.7822604839831,6.02451327872669));
#87429=CARTESIAN_POINT('Ctrl Pts',(1.3018854602463,-20.780006593215,6.03185870664777));
#87430=CARTESIAN_POINT('Ctrl Pts',(1.29454848205839,-20.7782260704221,6.03979378406956));
#87431=CARTESIAN_POINT('Ctrl Pts',(1.28757944370676,-20.7765348385128,6.04733092776269));
#87432=CARTESIAN_POINT('Ctrl Pts',(1.28011810284529,-20.7752712828586,6.05540051297026));
#87433=CARTESIAN_POINT('Ctrl Pts',(1.27219412867516,-20.7746541176134,6.06397047369944));
#87434=CARTESIAN_POINT('Ctrl Pts',(1.26869756731923,-20.7743817850565,6.06775208540894));
#87435=CARTESIAN_POINT('Ctrl Pts',(1.26511131777583,-20.7742356127999,6.0716307022037));
#87436=CARTESIAN_POINT('Ctrl Pts',(1.2614400074,-20.7742356128,6.07560132137));
#87437=CARTESIAN_POINT('',(2.54349379462,-21.0742356128,6.85242635913));
#87438=CARTESIAN_POINT('Origin',(0.00234331738835,-21.0742356128,3.08191746407));
#87439=CARTESIAN_POINT('',(5.48986775992,-20.7742356128,0.545353000555));
#87440=CARTESIAN_POINT('',(5.92013962829,-20.7742356128,1.84629187045));
#87441=CARTESIAN_POINT('Origin',(0.00234331738835,-20.7742356128,3.08191746407));
#87442=CARTESIAN_POINT('',(5.76218263052,-21.0742356128,0.419477620705));
#87443=CARTESIAN_POINT('Ctrl Pts',(5.76218263051847,-21.0742356128,0.419477620705708));
#87444=CARTESIAN_POINT('Ctrl Pts',(5.76218263051847,-21.0711343099908,0.419477620705708));
#87445=CARTESIAN_POINT('Ctrl Pts',(5.76212789615905,-21.0683778932532,0.419463148787726));
#87446=CARTESIAN_POINT('Ctrl Pts',(5.76202961598976,-21.0655246169381,0.419448073937373));
#87447=CARTESIAN_POINT('Ctrl Pts',(5.7619393761782,-21.0629047688154,0.419434232369283));
#87448=CARTESIAN_POINT('Ctrl Pts',(5.76181222718317,-21.0602030737192,0.419419973460183));
#87449=CARTESIAN_POINT('Ctrl Pts',(5.76162093210155,-21.0570790738875,0.419432631131333));
#87450=CARTESIAN_POINT('Ctrl Pts',(5.76147715112112,-21.0547310168705,0.419442144874982));
#87451=CARTESIAN_POINT('Ctrl Pts',(5.76129676935522,-21.052144336212,0.419467032354691));
#87452=CARTESIAN_POINT('Ctrl Pts',(5.76105046867993,-21.0491764894497,0.419527108581872));
#87453=CARTESIAN_POINT('Ctrl Pts',(5.76058502600462,-21.0435680495402,0.419640636650235));
#87454=CARTESIAN_POINT('Ctrl Pts',(5.76005667105559,-21.0380145982917,0.419983502847117));
#87455=CARTESIAN_POINT('Ctrl Pts',(5.75940097602592,-21.0324707850792,0.420422476369964));
#87456=CARTESIAN_POINT('Ctrl Pts',(5.75907312851108,-21.0296988784729,0.420641963131388));
#87457=CARTESIAN_POINT('Ctrl Pts',(5.7587133084088,-21.0269297742481,0.420885538444297));
#87458=CARTESIAN_POINT('Ctrl Pts',(5.75831217072801,-21.0241602367083,0.421135173302448));
#87459=CARTESIAN_POINT('Ctrl Pts',(5.75810699640252,-21.0227436707164,0.421262856803883));
#87460=CARTESIAN_POINT('Ctrl Pts',(5.75796930454998,-21.0218220855038,0.421353628373918));
#87461=CARTESIAN_POINT('Ctrl Pts',(5.75778181250985,-21.0206347166969,0.421461893833452));
#87462=CARTESIAN_POINT('Ctrl Pts',(5.75761225171338,-21.0195609047075,0.421559805070305));
#87463=CARTESIAN_POINT('Ctrl Pts',(5.75740301623091,-21.0182694210857,0.421671535862888));
#87464=CARTESIAN_POINT('Ctrl Pts',(5.75703739192913,-21.0162038360199,0.421851176134806));
#87465=CARTESIAN_POINT('Ctrl Pts',(5.75701687667445,-21.0160879356175,0.421861255787364));
#87466=CARTESIAN_POINT('Ctrl Pts',(5.75699585603951,-21.0159696010428,0.421871555257977));
#87467=CARTESIAN_POINT('Ctrl Pts',(5.75697430408466,-21.0158487352453,0.421882086561721));
#87468=CARTESIAN_POINT('Ctrl Pts',(5.75585610863276,-21.0095777688301,0.422428489708489));
#87469=CARTESIAN_POINT('Ctrl Pts',(5.75441381085562,-21.0027231086594,0.423037486106193));
#87470=CARTESIAN_POINT('Ctrl Pts',(5.75254933409048,-20.9952668038011,0.423852701949254));
#87471=CARTESIAN_POINT('Ctrl Pts',(5.75164469012145,-20.9916490053134,0.424248244607481));
#87472=CARTESIAN_POINT('Ctrl Pts',(5.75064012302674,-20.9878899914571,0.424692579687064));
#87473=CARTESIAN_POINT('Ctrl Pts',(5.74952131287696,-20.9839906759573,0.425203525154008));
#87474=CARTESIAN_POINT('Ctrl Pts',(5.74780897051388,-20.9780227616345,0.42598552875707));
#87475=CARTESIAN_POINT('Ctrl Pts',(5.74582812460024,-20.9717317114928,0.42691700148707));
#87476=CARTESIAN_POINT('Ctrl Pts',(5.74350992019445,-20.9651556634559,0.428019179652195));
#87477=CARTESIAN_POINT('Ctrl Pts',(5.74235081799156,-20.9618676394374,0.428570268734759));
#87478=CARTESIAN_POINT('Ctrl Pts',(5.7411071187696,-20.9585087257985,0.429163558530631));
#87479=CARTESIAN_POINT('Ctrl Pts',(5.73976875796006,-20.9550856710468,0.429798754464527));
#87480=CARTESIAN_POINT('Ctrl Pts',(5.73909957755529,-20.9533741436709,0.430116352431476));
#87481=CARTESIAN_POINT('Ctrl Pts',(5.7384067253257,-20.9516465841452,0.430444429904209));
#87482=CARTESIAN_POINT('Ctrl Pts',(5.73768884898717,-20.9499039715201,0.430782712005881));
#87483=CARTESIAN_POINT('Ctrl Pts',(5.73723620114925,-20.9488051891885,0.430996011502904));
#87484=CARTESIAN_POINT('Ctrl Pts',(5.7369582236608,-20.9481396816218,0.431127352220856));
#87485=CARTESIAN_POINT('Ctrl Pts',(5.73650730043681,-20.9470757776858,0.431338468887568));
#87486=CARTESIAN_POINT('Ctrl Pts',(5.73624308247185,-20.9464523843498,0.43146217246521));
#87487=CARTESIAN_POINT('Ctrl Pts',(5.73591920109332,-20.9456923382671,0.431613397647289));
#87488=CARTESIAN_POINT('Ctrl Pts',(5.73545877283664,-20.9446319683954,0.431827894353049));
#87489=CARTESIAN_POINT('Ctrl Pts',(5.73241146794468,-20.9376140014255,0.433247522386909));
#87490=CARTESIAN_POINT('Ctrl Pts',(5.72880348035714,-20.9300323022399,0.434890170001915));
#87491=CARTESIAN_POINT('Ctrl Pts',(5.72450075487575,-20.9219992593249,0.43685668003197));
#87492=CARTESIAN_POINT('Ctrl Pts',(5.72176499618178,-20.9168916903924,0.438107026338003));
#87493=CARTESIAN_POINT('Ctrl Pts',(5.71874800465858,-20.9116025113626,0.439488469477967));
#87494=CARTESIAN_POINT('Ctrl Pts',(5.71541312463863,-20.9061714559532,0.441027877214491));
#87495=CARTESIAN_POINT('Ctrl Pts',(5.71112318117637,-20.8991850215064,0.443008150002585));
#87496=CARTESIAN_POINT('Ctrl Pts',(5.70630577576505,-20.8919640396089,0.445245856444974));
#87497=CARTESIAN_POINT('Ctrl Pts',(5.70087617302816,-20.8846214612248,0.44777265102263));
#87498=CARTESIAN_POINT('Ctrl Pts',(5.69816137165972,-20.8809501720327,0.449036048311459));
#87499=CARTESIAN_POINT('Ctrl Pts',(5.6952934808518,-20.8772489447893,0.450371431448299));
#87500=CARTESIAN_POINT('Ctrl Pts',(5.69226197710357,-20.8735347161601,0.451780936519775));
#87501=CARTESIAN_POINT('Ctrl Pts',(5.69074622522945,-20.8716776018455,0.452485689055514));
#87502=CARTESIAN_POINT('Ctrl Pts',(5.68940323754624,-20.8700725536964,0.453110116987698));
#87503=CARTESIAN_POINT('Ctrl Pts',(5.68791548452027,-20.8683345079178,0.453800644920927));
#87504=CARTESIAN_POINT('Ctrl Pts',(5.686539273402,-20.8667267693463,0.45443940162489));
#87505=CARTESIAN_POINT('Ctrl Pts',(5.68503937868389,-20.8650047885142,0.455134631163884));
#87506=CARTESIAN_POINT('Ctrl Pts',(5.68313710135166,-20.8628930892138,0.456014882216015));
#87507=CARTESIAN_POINT('Ctrl Pts',(5.68298292177862,-20.8627219359908,0.456086226561599));
#87508=CARTESIAN_POINT('Ctrl Pts',(5.68282608050964,-20.8625482437002,0.456158794840108));
#87509=CARTESIAN_POINT('Ctrl Pts',(5.68266641862616,-20.8623718778984,0.45623266036311));
#87510=CARTESIAN_POINT('Ctrl Pts',(5.67682336636476,-20.8559175221388,0.458935873564779));
#87511=CARTESIAN_POINT('Ctrl Pts',(5.67024533328323,-20.8492424579849,0.46196525160643));
#87512=CARTESIAN_POINT('Ctrl Pts',(5.66283907998627,-20.8425348446108,0.465380025587699));
#87513=CARTESIAN_POINT('Ctrl Pts',(5.65944809206181,-20.8394637322627,0.466943495924311));
#87514=CARTESIAN_POINT('Ctrl Pts',(5.65588362700338,-20.836386463225,0.468587688276975));
#87515=CARTESIAN_POINT('Ctrl Pts',(5.65213788215834,-20.8333245964127,0.47031774081465));
#87516=CARTESIAN_POINT('Ctrl Pts',(5.64617447097158,-20.8284499529021,0.47307207008257));
#87517=CARTESIAN_POINT('Ctrl Pts',(5.63975073557742,-20.8236137372718,0.476043246403684));
#87518=CARTESIAN_POINT('Ctrl Pts',(5.63283950439035,-20.818915369188,0.479242079185539));
#87519=CARTESIAN_POINT('Ctrl Pts',(5.62938388879682,-20.8165661851461,0.480841495576468));
#87520=CARTESIAN_POINT('Ctrl Pts',(5.62580651502869,-20.8142516964488,0.482497682560015));
#87521=CARTESIAN_POINT('Ctrl Pts',(5.622104846316,-20.8119857073957,0.484211032033263));
#87522=CARTESIAN_POINT('Ctrl Pts',(5.62014404904501,-20.8107853986982,0.485118604058787));
#87523=CARTESIAN_POINT('Ctrl Pts',(5.61787341347036,-20.8094357628297,0.486169352333183));
#87524=CARTESIAN_POINT('Ctrl Pts',(5.61572711915748,-20.8082031531422,0.48716234631413));
#87525=CARTESIAN_POINT('Ctrl Pts',(5.6138215562877,-20.8071087947219,0.488043964668452));
#87526=CARTESIAN_POINT('Ctrl Pts',(5.61201474620417,-20.8061054212397,0.48887971586325));
#87527=CARTESIAN_POINT('Ctrl Pts',(5.61062513049926,-20.805347934196,0.489522239721216));
#87528=CARTESIAN_POINT('Ctrl Pts',(5.60528025572931,-20.8024344140232,0.491993577333035));
#87529=CARTESIAN_POINT('Ctrl Pts',(5.59914555171968,-20.7993271570843,0.494830284396293));
#87530=CARTESIAN_POINT('Ctrl Pts',(5.5921663409056,-20.7962101943979,0.49805747101858));
#87531=CARTESIAN_POINT('Ctrl Pts',(5.58552594074091,-20.7932445468357,0.501127991618825));
#87532=CARTESIAN_POINT('Ctrl Pts',(5.57812019278002,-20.7902703605307,0.504552390383305));
#87533=CARTESIAN_POINT('Ctrl Pts',(5.56991509591193,-20.7874902135388,0.508346244034247));
#87534=CARTESIAN_POINT('Ctrl Pts',(5.56198690494279,-20.7848038910458,0.512012062578159));
#87535=CARTESIAN_POINT('Ctrl Pts',(5.55331157924344,-20.7822990373231,0.516023202866985));
#87536=CARTESIAN_POINT('Ctrl Pts',(5.54388302057105,-20.7801968080192,0.520382359688187));
#87537=CARTESIAN_POINT('Ctrl Pts',(5.53496122955905,-20.7782075696679,0.524507219860206));
#87538=CARTESIAN_POINT('Ctrl Pts',(5.52536442562282,-20.7765793991742,0.528943956612456));
#87539=CARTESIAN_POINT('Ctrl Pts',(5.51511959478089,-20.7755282547698,0.533679993439904));
#87540=CARTESIAN_POINT('Ctrl Pts',(5.50708945068104,-20.7747043425776,0.537392212682312));
#87541=CARTESIAN_POINT('Ctrl Pts',(5.49866164782896,-20.7742356127999,0.541288095915715));
#87542=CARTESIAN_POINT('Ctrl Pts',(5.48986775992,-20.7742356128,0.545353000555));
#87543=CARTESIAN_POINT('',(6.21380646358,-21.0742356128,1.78497474518));
#87544=CARTESIAN_POINT('Origin',(0.00234331738835,-21.0742356128,3.08191746407));
#87545=CARTESIAN_POINT('Origin',(5.92013962829301,-21.0742356128,1.84629187044622));
#87546=CARTESIAN_POINT('Origin',(5.48986775992,-21.0742356128,0.545353000555));
#87547=CARTESIAN_POINT('',(5.1900363009,-21.0742356128,0.55540766038));
#87548=CARTESIAN_POINT('Origin',(5.48986775992,-21.0742356128,0.545353000555));
#87549=CARTESIAN_POINT('Origin',(5.48986775992,-21.0742356128,0.545353000555));
#87550=CARTESIAN_POINT('Origin',(-9.64069499267E-16,-21.0742356128,0.729452270839));
#87551=CARTESIAN_POINT('',(5.08448267152,-21.0742356128,1.78529520144));
#87552=CARTESIAN_POINT('Origin',(2.57175827821E-16,-21.0742356128,0.729452270839));
#87553=CARTESIAN_POINT('',(5.3782162351,-20.7742356128,1.84629187045));
#87554=CARTESIAN_POINT('Origin',(4.75197961991E-16,-20.7742356128,0.729452270839));
#87555=CARTESIAN_POINT('Ctrl Pts',(5.08448267152151,-21.0742356128,1.78529520144031));
#87556=CARTESIAN_POINT('Ctrl Pts',(5.08448267152151,-21.0645012808632,1.78529520144031));
#87557=CARTESIAN_POINT('Ctrl Pts',(5.08493635413104,-21.0548222582473,1.78541942341338));
#87558=CARTESIAN_POINT('Ctrl Pts',(5.08585408050998,-21.0451000686285,1.78566598382418));
#87559=CARTESIAN_POINT('Ctrl Pts',(5.0861237656047,-21.0422430845769,1.78573843860947));
#87560=CARTESIAN_POINT('Ctrl Pts',(5.08643385657685,-21.0393824001939,1.78582152773478));
#87561=CARTESIAN_POINT('Ctrl Pts',(5.08678544912873,-21.0365156373058,1.7859153777379));
#87562=CARTESIAN_POINT('Ctrl Pts',(5.087358954137,-21.0318394777425,1.78606846245636));
#87563=CARTESIAN_POINT('Ctrl Pts',(5.08800922997164,-21.0273865922814,1.78624165419594));
#87564=CARTESIAN_POINT('Ctrl Pts',(5.0887681237863,-21.0228804144151,1.78643788818155));
#87565=CARTESIAN_POINT('Ctrl Pts',(5.08949382756653,-21.01857131313,1.78662553992205));
#87566=CARTESIAN_POINT('Ctrl Pts',(5.09031904028443,-21.0142131582222,1.78683430063852));
#87567=CARTESIAN_POINT('Ctrl Pts',(5.09131507023229,-21.0095725885318,1.78707576275223));
#87568=CARTESIAN_POINT('Ctrl Pts',(5.09208897432893,-21.0059669179375,1.78726337610601));
#87569=CARTESIAN_POINT('Ctrl Pts',(5.09296663835046,-21.0021907778178,1.78747086375398));
#87570=CARTESIAN_POINT('Ctrl Pts',(5.09400200555433,-20.9981410352675,1.7877079192303));
#87571=CARTESIAN_POINT('Ctrl Pts',(5.09735848797456,-20.9850124663638,1.78847641231749));
#87572=CARTESIAN_POINT('Ctrl Pts',(5.10160218254057,-20.9721584640941,1.78927961768519));
#87573=CARTESIAN_POINT('Ctrl Pts',(5.106717486722,-20.9595797111132,1.79023334935614));
#87574=CARTESIAN_POINT('Ctrl Pts',(5.10733456447915,-20.9580622903691,1.79034840147808));
#87575=CARTESIAN_POINT('Ctrl Pts',(5.10796438229745,-20.9565488997241,1.79046565666436));
#87576=CARTESIAN_POINT('Ctrl Pts',(5.10860695783828,-20.9550395633781,1.79058532849954));
#87577=CARTESIAN_POINT('Ctrl Pts',(5.1115915804258,-20.9480290267735,1.79114117795172));
#87578=CARTESIAN_POINT('Ctrl Pts',(5.11485094784533,-20.9411066703631,1.79174864351049));
#87579=CARTESIAN_POINT('Ctrl Pts',(5.11838596254678,-20.9342820340361,1.79242876609553));
#87580=CARTESIAN_POINT('Ctrl Pts',(5.11997031565205,-20.9312233101919,1.79273358924921));
#87581=CARTESIAN_POINT('Ctrl Pts',(5.12147401393412,-20.9284382834278,1.79302477068904));
#87582=CARTESIAN_POINT('Ctrl Pts',(5.12307240443405,-20.9255823146597,1.7933407263901));
#87583=CARTESIAN_POINT('Ctrl Pts',(5.12458936757298,-20.922871838498,1.79364058625043));
#87584=CARTESIAN_POINT('Ctrl Pts',(5.12619170434029,-20.9200972224439,1.79396277721054));
#87585=CARTESIAN_POINT('Ctrl Pts',(5.12806711119576,-20.9169866084276,1.79434799265438));
#87586=CARTESIAN_POINT('Ctrl Pts',(5.128624655078,-20.9160618470566,1.7944625142119));
#87587=CARTESIAN_POINT('Ctrl Pts',(5.12920660615708,-20.9151075694506,1.79458266270214));
#87588=CARTESIAN_POINT('Ctrl Pts',(5.12981865714652,-20.9141171584819,1.79470966561171));
#87589=CARTESIAN_POINT('Ctrl Pts',(5.13571048973975,-20.9045830906885,1.79593224329713));
#87590=CARTESIAN_POINT('Ctrl Pts',(5.14237609352167,-20.8949759521074,1.79734044684605));
#87591=CARTESIAN_POINT('Ctrl Pts',(5.14994010475542,-20.8854315566452,1.79893114249031));
#87592=CARTESIAN_POINT('Ctrl Pts',(5.15480356908058,-20.8792947562887,1.79995391880291));
#87593=CARTESIAN_POINT('Ctrl Pts',(5.16003847376736,-20.8731848198683,1.80105213969165));
#87594=CARTESIAN_POINT('Ctrl Pts',(5.16567611424345,-20.8671492374168,1.80222448041741));
#87595=CARTESIAN_POINT('Ctrl Pts',(5.1728789674508,-20.8594379591608,1.80372230529511));
#87596=CARTESIAN_POINT('Ctrl Pts',(5.18073771166217,-20.8518495686742,1.80534366782332));
#87597=CARTESIAN_POINT('Ctrl Pts',(5.18929178411293,-20.8445144710433,1.80710321495179));
#87598=CARTESIAN_POINT('Ctrl Pts',(5.19356882033831,-20.8408469222279,1.80798298851602));
#87599=CARTESIAN_POINT('Ctrl Pts',(5.19801929010056,-20.8372431454817,1.80889750837796));
#87600=CARTESIAN_POINT('Ctrl Pts',(5.2026453324478,-20.8337219160368,1.80984986035332));
#87601=CARTESIAN_POINT('Ctrl Pts',(5.20482458890421,-20.8320631197211,1.81029849852723));
#87602=CARTESIAN_POINT('Ctrl Pts',(5.20729377052198,-20.8302368573979,1.81080756543739));
#87603=CARTESIAN_POINT('Ctrl Pts',(5.20970255987384,-20.8285141256464,1.81130484348002));
#87604=CARTESIAN_POINT('Ctrl Pts',(5.21226982625804,-20.8266780533841,1.81183483801917));
#87605=CARTESIAN_POINT('Ctrl Pts',(5.21476811176166,-20.8249595464615,1.81235136263844));
#87606=CARTESIAN_POINT('Ctrl Pts',(5.21673873283519,-20.8236350991637,1.81275981371049));
#87607=CARTESIAN_POINT('Ctrl Pts',(5.21684407011857,-20.8235643023564,1.81278164699285));
#87608=CARTESIAN_POINT('Ctrl Pts',(5.2169478937756,-20.8234946216469,1.81280317024565));
#87609=CARTESIAN_POINT('Ctrl Pts',(5.21705013203445,-20.823426096337,1.81282436866361));
#87610=CARTESIAN_POINT('Ctrl Pts',(5.22311200407881,-20.8193631196666,1.81408125721617));
#87611=CARTESIAN_POINT('Ctrl Pts',(5.2299956639905,-20.815073378029,1.81550954592068));
#87612=CARTESIAN_POINT('Ctrl Pts',(5.23778079317007,-20.8107451705707,1.81712556253911));
#87613=CARTESIAN_POINT('Ctrl Pts',(5.2456193267744,-20.8063872724772,1.81875266470743));
#87614=CARTESIAN_POINT('Ctrl Pts',(5.25437302208229,-20.8019900893308,1.82057034556678));
#87615=CARTESIAN_POINT('Ctrl Pts',(5.26410524797891,-20.7977994050181,1.82259154001717));
#87616=CARTESIAN_POINT('Ctrl Pts',(5.27286540995792,-20.7940272902139,1.82441085565623));
#87617=CARTESIAN_POINT('Ctrl Pts',(5.28241898978949,-20.7904232329663,1.82639518524843));
#87618=CARTESIAN_POINT('Ctrl Pts',(5.29278538050293,-20.7872047120146,1.82854839034495));
#87619=CARTESIAN_POINT('Ctrl Pts',(5.30279387491744,-20.7840973094615,1.83062725672936));
#87620=CARTESIAN_POINT('Ctrl Pts',(5.31356076205147,-20.7813497253196,1.83286369230111));
#87621=CARTESIAN_POINT('Ctrl Pts',(5.32506738039261,-20.7791875533763,1.83525366970004));
#87622=CARTESIAN_POINT('Ctrl Pts',(5.33601843901391,-20.7771297748877,1.83752825479734));
#87623=CARTESIAN_POINT('Ctrl Pts',(5.34763998791755,-20.7756028672462,1.83994200986043));
#87624=CARTESIAN_POINT('Ctrl Pts',(5.35987426374726,-20.7748210789055,1.84248280497264));
#87625=CARTESIAN_POINT('Ctrl Pts',(5.36584662389524,-20.7744394362488,1.84372313531042));
#87626=CARTESIAN_POINT('Ctrl Pts',(5.37196431144922,-20.7742356127999,1.84499359689556));
#87627=CARTESIAN_POINT('Ctrl Pts',(5.3782162351,-20.7742356128,1.84629187045));
#87628=CARTESIAN_POINT('Origin',(5.92013962829,-21.0742356128,1.84629187045));
#87629=CARTESIAN_POINT('',(5.92013962829,-21.0742356128,2.14629187045));
#87630=CARTESIAN_POINT('Origin',(5.92013962829,-21.0742356128,1.84629187045));
#87631=CARTESIAN_POINT('Origin',(5.92013962829,-21.0742356128,1.84629187045));
#87632=CARTESIAN_POINT('Origin',(5.3782162351,-21.0742356128,1.84629187045));
#87633=CARTESIAN_POINT('',(5.3782162351,-21.0742356128,2.14629187045));
#87634=CARTESIAN_POINT('Origin',(5.3782162351,-21.0742356128,1.84629187045));
#87635=CARTESIAN_POINT('Origin',(5.3782162351,-21.0742356128,1.84629187045));
#87636=CARTESIAN_POINT('Origin',(3.31206782846,-21.0742356128,5.11154620667));
#87637=CARTESIAN_POINT('',(3.13117783752,-21.0742356128,4.87221628548));
#87638=CARTESIAN_POINT('Origin',(3.31206782846,-21.0742356128,5.11154620667));
#87639=CARTESIAN_POINT('Origin',(3.31206782846,-21.0742356128,5.11154620667));
#87640=CARTESIAN_POINT('Origin',(-5.60029074364,-21.0742356128,1.84629187045));
#87641=CARTESIAN_POINT('',(5.6491779317,-21.0742356128,2.14629187045));
#87642=CARTESIAN_POINT('',(5.6491779317,-20.7742356128,1.84629187045));
#87643=CARTESIAN_POINT('Origin',(-9.64069499267E-16,-21.0742356128,0.729452270839));
#87644=CARTESIAN_POINT('',(4.452469377,-20.7742356128,3.94629187045));
#87645=CARTESIAN_POINT('Origin',(4.75197961991E-16,-20.7742356128,0.729452270839));
#87646=CARTESIAN_POINT('',(4.2092958712,-21.0742356128,3.77060280966));
#87647=CARTESIAN_POINT('Origin',(2.57175827821E-16,-21.0742356128,0.729452270839));
#87648=CARTESIAN_POINT('Origin',(4.45246937699693,-21.0742356128,3.94629187044695));
#87649=CARTESIAN_POINT('Origin',(1.05,-22.8742356128,-4.99584562937));
#87650=CARTESIAN_POINT('',(1.01141425905,-22.8742356128,-4.69833741));
#87651=CARTESIAN_POINT('Origin',(1.05,-22.8742356128,-4.99584562937));
#87652=CARTESIAN_POINT('',(0.972828518105,-23.1742356128,-4.40082919062));
#87653=CARTESIAN_POINT('Origin',(0.972828518105,-22.8742356128,-4.40082919062));
#87654=CARTESIAN_POINT('Origin',(1.05,-23.1742356128,-4.99584562937));
#87655=CARTESIAN_POINT('Origin',(0.00234331738835,-22.8742356128,3.08191746407));
#87656=CARTESIAN_POINT('',(4.40684492179,-22.8742356128,-3.41045927235));
#87657=CARTESIAN_POINT('Origin',(0.00234331738835,-22.8742356128,3.08191746407));
#87658=CARTESIAN_POINT('',(4.23842172091,-23.1742356128,-3.16219806837));
#87659=CARTESIAN_POINT('Origin',(4.23842172091,-22.8742356128,-3.16219806837));
#87660=CARTESIAN_POINT('Origin',(0.00234331738835,-23.1742356128,3.08191746407));
#87661=CARTESIAN_POINT('Origin',(6.34552156645,-22.8742356128,-5.5301356238));
#87662=CARTESIAN_POINT('',(6.56346233154,-22.8742356128,-5.32397592135));
#87663=CARTESIAN_POINT('Origin',(6.34552156645,-22.8742356128,-5.5301356238));
#87664=CARTESIAN_POINT('',(6.78140309663,-23.1742356128,-5.11781621891));
#87665=CARTESIAN_POINT('Origin',(6.34552156645,-23.1742356128,-5.5301356238));
#87666=CARTESIAN_POINT('Origin',(6.78140309663,-22.8742356128,-5.11781621891));
#87667=CARTESIAN_POINT('Origin',(4.57526812267,-22.8742356128,-3.65872047634));
#87668=CARTESIAN_POINT('',(4.79320888776,-22.8742356128,-3.4525607739));
#87669=CARTESIAN_POINT('Origin',(4.57526812267,-22.8742356128,-3.65872047634));
#87670=CARTESIAN_POINT('',(5.01114965285,-23.1742356128,-3.24640107146));
#87671=CARTESIAN_POINT('Origin',(5.01114965285,-22.8742356128,-3.24640107146));
#87672=CARTESIAN_POINT('Origin',(4.57526812267,-23.1742356128,-3.65872047634));
#87673=CARTESIAN_POINT('Origin',(1.2614400074,-21.0742356128,6.07560132137));
#87674=CARTESIAN_POINT('',(1.19254592572,-21.0742356128,5.78361912069));
#87675=CARTESIAN_POINT('Origin',(1.2614400074,-21.0742356128,6.07560132137));
#87676=CARTESIAN_POINT('Origin',(1.2614400074,-21.0742356128,6.07560132137));
#87677=CARTESIAN_POINT('Origin',(-2.84607155346,-21.3642356128,5.53854202767));
#87678=CARTESIAN_POINT('',(0.24693418390444,-21.0742356128,-6.59919549800697));
#87679=CARTESIAN_POINT('',(0.530881034116209,-21.0742356128,-6.5232798892238));
#87680=CARTESIAN_POINT('Origin',(-2.84607155346,-21.0742356128,5.53854202767));
#87681=CARTESIAN_POINT('',(0.530881036642,-22.1242356128,-6.52327988851));
#87682=CARTESIAN_POINT('',(0.246934184763,-21.9742356128,-6.59919549778));
#87683=CARTESIAN_POINT('Origin',(0.45,-22.8742356128,-6.23438845923));
#87684=CARTESIAN_POINT('Origin',(0.45,-22.8742356128,-6.23438845923));
#87685=CARTESIAN_POINT('Origin',(-2.84607155346,-21.0742356128,5.53854202767));
#87686=CARTESIAN_POINT('',(-2.57204347673E-14,-20.7742356128,-6.9673210071));
#87687=CARTESIAN_POINT('',(1.05,-20.7742356128,-6.68100624476));
#87688=CARTESIAN_POINT('Origin',(-2.84607155346,-20.7742356128,5.53854202767));
#87689=CARTESIAN_POINT('Ctrl Pts',(1.05,-20.7742356128,-6.68100624476));
#87690=CARTESIAN_POINT('Ctrl Pts',(1.006378088465,-20.774235612803,-6.66794906990942));
#87691=CARTESIAN_POINT('Ctrl Pts',(0.971270142094555,-20.7774178420795,
-6.65723073068667));
#87692=CARTESIAN_POINT('Ctrl Pts',(0.931206866676575,-20.7823657860325,
-6.64516796906486));
#87693=CARTESIAN_POINT('Ctrl Pts',(0.919947591790132,-20.7840670881655,
-6.6417964225193));
#87694=CARTESIAN_POINT('Ctrl Pts',(0.906163283936589,-20.7863320840288,
-6.63767504469205));
#87695=CARTESIAN_POINT('Ctrl Pts',(0.900047303757202,-20.7873950394116,
-6.6358478896007));
#87696=CARTESIAN_POINT('Ctrl Pts',(0.894263030875596,-20.7884563412427,
-6.63411460040872));
#87697=CARTESIAN_POINT('Ctrl Pts',(0.892072910743004,-20.7888681600112,
-6.63345609672299));
#87698=CARTESIAN_POINT('Ctrl Pts',(0.890676953005833,-20.7891326580897,
-6.63303572875016));
#87699=CARTESIAN_POINT('Ctrl Pts',(0.891342463725141,-20.7890036879005,
-6.63323730344035));
#87700=CARTESIAN_POINT('Ctrl Pts',(0.857932066361018,-20.795432472259,-6.62313857302724));
#87701=CARTESIAN_POINT('Ctrl Pts',(0.829362919845069,-20.802875391614,-6.61444203033488));
#87702=CARTESIAN_POINT('Ctrl Pts',(0.790768248157906,-20.8150830094904,
-6.60272732837196));
#87703=CARTESIAN_POINT('Ctrl Pts',(0.772534435649399,-20.8214503084994,
-6.59719758887313));
#87704=CARTESIAN_POINT('Ctrl Pts',(0.753100910252478,-20.8291425208755,
-6.59130218188709));
#87705=CARTESIAN_POINT('Ctrl Pts',(0.745163626503657,-20.8324766906795,
-6.58889074338885));
#87706=CARTESIAN_POINT('Ctrl Pts',(0.739958766209563,-20.8347057549421,
-6.58730823813184));
#87707=CARTESIAN_POINT('Ctrl Pts',(0.738546223118208,-20.8353131034927,
-6.58687880685544));
#87708=CARTESIAN_POINT('Ctrl Pts',(0.70558389892941,-20.8499843029599,-6.57683802928427));
#87709=CARTESIAN_POINT('Ctrl Pts',(0.679666465671247,-20.8643807451744,
-6.56888477745874));
#87710=CARTESIAN_POINT('Ctrl Pts',(0.645800235846747,-20.8870802526004,
-6.55852605327747));
#87711=CARTESIAN_POINT('Ctrl Pts',(0.630118691860855,-20.8987080773537,
-6.5537351047842));
#87712=CARTESIAN_POINT('Ctrl Pts',(0.613992298402707,-20.9125803270019,
-6.54880951587271));
#87713=CARTESIAN_POINT('Ctrl Pts',(0.607543073274637,-20.9185736067731,
-6.5468369254342));
#87714=CARTESIAN_POINT('Ctrl Pts',(0.603345978244923,-20.9225778908473,
-6.5455521436202));
#87715=CARTESIAN_POINT('Ctrl Pts',(0.602161475406804,-20.9237156571488,
-6.54518957594162));
#87716=CARTESIAN_POINT('Ctrl Pts',(0.553555750815527,-20.9726539431238,
-6.53027978485194));
#87717=CARTESIAN_POINT('Ctrl Pts',(0.530881010941542,-21.02423748137,-6.52327989573953));
#87718=CARTESIAN_POINT('Ctrl Pts',(0.530881033271,-21.0742356128,-6.52327988945));
#87719=CARTESIAN_POINT('Ctrl Pts',(-2.57204347673E-14,-20.7742356128,-6.9673210071));
#87720=CARTESIAN_POINT('Ctrl Pts',(0.0620789114664,-20.7727817153,-6.86712083978));
#87721=CARTESIAN_POINT('Ctrl Pts',(0.126706651057,-20.809097628,-6.7683471563));
#87722=CARTESIAN_POINT('Ctrl Pts',(0.185538258403,-20.8478771982,-6.68330934255));
#87723=CARTESIAN_POINT('Ctrl Pts',(0.248193078621,-20.9544277624,-6.59756027965));
#87724=CARTESIAN_POINT('Ctrl Pts',(0.246934184763,-21.0742356128,-6.59919549778));
#87725=CARTESIAN_POINT('Origin',(2.45,-20.1742356128,10.7304528845));
#87726=CARTESIAN_POINT('',(2.45,-20.6742356128,10.4304528845));
#87727=CARTESIAN_POINT('',(2.45,-19.6742356128,10.4304528845));
#87728=CARTESIAN_POINT('',(2.45,-20.1742356128,10.4304528845));
#87729=CARTESIAN_POINT('',(2.75,-20.6742356128,10.7304528845));
#87730=CARTESIAN_POINT('Origin',(2.45,-20.6742356128,10.7304528845));
#87731=CARTESIAN_POINT('',(2.75,-19.6742356128,10.7304528845));
#87732=CARTESIAN_POINT('',(2.75,-20.1742356128,10.7304528845));
#87733=CARTESIAN_POINT('Origin',(2.45,-19.6742356128,10.7304528845));
#87734=CARTESIAN_POINT('Origin',(-9.64069499267E-16,-21.0742356128,0.729452270839));
#87735=CARTESIAN_POINT('',(1.05,-20.7742356128,6.12111625914));
#87736=CARTESIAN_POINT('Origin',(4.75197961991E-16,-20.7742356128,0.729452270839));
#87737=CARTESIAN_POINT('',(0.992653804111,-21.0742356128,5.82664824081));
#87738=CARTESIAN_POINT('Ctrl Pts',(0.992653804110976,-21.0742356128,5.82664824080987));
#87739=CARTESIAN_POINT('Ctrl Pts',(0.992653804110976,-21.0613737826999,
5.82664824080987));
#87740=CARTESIAN_POINT('Ctrl Pts',(0.992825465996969,-21.0486394859167,
5.82745302551633));
#87741=CARTESIAN_POINT('Ctrl Pts',(0.993151712284542,-21.0360081665505,
5.82904274860581));
#87742=CARTESIAN_POINT('Ctrl Pts',(0.993476339962666,-21.023439515094,5.8306245845839));
#87743=CARTESIAN_POINT('Ctrl Pts',(0.993954068039893,-21.0109715861115,
5.83298378539892));
#87744=CARTESIAN_POINT('Ctrl Pts',(0.994577669380009,-20.9985866770784,
5.83615027998842));
#87745=CARTESIAN_POINT('Ctrl Pts',(0.994884640200276,-20.9924901448225,
5.83770900249105));
#87746=CARTESIAN_POINT('Ctrl Pts',(0.995227101477724,-20.9864139435517,
5.8394640863575));
#87747=CARTESIAN_POINT('Ctrl Pts',(0.995604989294859,-20.9803579410823,
5.84142326476368));
#87748=CARTESIAN_POINT('Ctrl Pts',(0.996177838868538,-20.9711774957876,
5.84439323220866));
#87749=CARTESIAN_POINT('Ctrl Pts',(0.996830573889298,-20.962155591815,5.84779097546331));
#87750=CARTESIAN_POINT('Ctrl Pts',(0.997575235448733,-20.9532078147706,
5.85166511578626));
#87751=CARTESIAN_POINT('Ctrl Pts',(0.998306361330434,-20.9444226810437,
5.85546883604489));
#87752=CARTESIAN_POINT('Ctrl Pts',(0.999126166345993,-20.9357082365423,
5.85973212489889));
#87753=CARTESIAN_POINT('Ctrl Pts',(1.00005409684399,-20.9270106806024,5.86454224149691));
#87754=CARTESIAN_POINT('Ctrl Pts',(1.00094215928179,-20.918686810714,5.86914569389055));
#87755=CARTESIAN_POINT('Ctrl Pts',(1.00192934138979,-20.9103777939368,5.87425043911198));
#87756=CARTESIAN_POINT('Ctrl Pts',(1.00303902096319,-20.9020702878808,5.87996533679234));
#87757=CARTESIAN_POINT('Ctrl Pts',(1.00354099141114,-20.8983123359133,5.88255050625687));
#87758=CARTESIAN_POINT('Ctrl Pts',(1.00406810880741,-20.8945552183043,5.88526094126346));
#87759=CARTESIAN_POINT('Ctrl Pts',(1.00462291545805,-20.8908006844483,5.88810864711666));
#87760=CARTESIAN_POINT('Ctrl Pts',(1.00604541019738,-20.8811742593637,5.89541001344061));
#87761=CARTESIAN_POINT('Ctrl Pts',(1.00761700622559,-20.8716304920317,5.90356829143893));
#87762=CARTESIAN_POINT('Ctrl Pts',(1.00937693368903,-20.8623392678651,5.91267032767187));
#87763=CARTESIAN_POINT('Ctrl Pts',(1.01031913859313,-20.8573650645773,5.91754324621774));
#87764=CARTESIAN_POINT('Ctrl Pts',(1.01131528205079,-20.8524640313087,5.92268642406207));
#87765=CARTESIAN_POINT('Ctrl Pts',(1.01237095229975,-20.8476679491939,5.92811068835221));
#87766=CARTESIAN_POINT('Ctrl Pts',(1.01388472108653,-20.8407906507086,5.93588876297518));
#87767=CARTESIAN_POINT('Ctrl Pts',(1.01551908576205,-20.8341296333023,5.94424489985484));
#87768=CARTESIAN_POINT('Ctrl Pts',(1.0172728984018,-20.8277975927477,5.95319592166203));
#87769=CARTESIAN_POINT('Ctrl Pts',(1.01814980472168,-20.8246315724705,5.95767143256562));
#87770=CARTESIAN_POINT('Ctrl Pts',(1.01905633611331,-20.8215480876829,5.96229539287826));
#87771=CARTESIAN_POINT('Ctrl Pts',(1.01999076354253,-20.8185628017482,5.96706802156685));
#87772=CARTESIAN_POINT('Ctrl Pts',(1.02040789087176,-20.8172301735418,5.96919851752195));
#87773=CARTESIAN_POINT('Ctrl Pts',(1.0208895573644,-20.8157326799941,5.97166143704105));
#87774=CARTESIAN_POINT('Ctrl Pts',(1.0213573719682,-20.8143264991543,5.97405554883608));
#87775=CARTESIAN_POINT('Ctrl Pts',(1.02186869752868,-20.8127895308763,5.97667233451461));
#87776=CARTESIAN_POINT('Ctrl Pts',(1.02236341457022,-20.8113617135062,5.97920661000325));
#87777=CARTESIAN_POINT('Ctrl Pts',(1.02273276025893,-20.8103182140549,5.98110160177315));
#87778=CARTESIAN_POINT('Ctrl Pts',(1.02278248133912,-20.8101777388267,5.98135670435221));
#87779=CARTESIAN_POINT('Ctrl Pts',(1.02282992379982,-20.8100441598503,5.98160018774461));
#87780=CARTESIAN_POINT('Ctrl Pts',(1.0228748175706,-20.8099180973871,5.98183066934277));
#87781=CARTESIAN_POINT('Ctrl Pts',(1.02409474741574,-20.8064925138705,5.98809370707443));
#87782=CARTESIAN_POINT('Ctrl Pts',(1.02547918299804,-20.8028985711144,5.99520200039718));
#87783=CARTESIAN_POINT('Ctrl Pts',(1.02704067673227,-20.7993296264459,6.00321982941105));
#87784=CARTESIAN_POINT('Ctrl Pts',(1.02851792533699,-20.7959532321535,6.01080508349438));
#87785=CARTESIAN_POINT('Ctrl Pts',(1.03015381253913,-20.7925995024583,6.01920525300589));
#87786=CARTESIAN_POINT('Ctrl Pts',(1.03195568051599,-20.7894746092439,6.02845788990672));
#87787=CARTESIAN_POINT('Ctrl Pts',(1.0336950692818,-20.7864580707288,6.03738969450398));
#87788=CARTESIAN_POINT('Ctrl Pts',(1.03558929375091,-20.7836550977369,6.04711672596956));
#87789=CARTESIAN_POINT('Ctrl Pts',(1.03763939303912,-20.7812876463859,6.05764418362696));
#87790=CARTESIAN_POINT('Ctrl Pts',(1.03957796100886,-20.7790489912215,6.06759891720247));
#87791=CARTESIAN_POINT('Ctrl Pts',(1.04165601533973,-20.7772003243519,6.07826992132226));
#87792=CARTESIAN_POINT('Ctrl Pts',(1.04386745197186,-20.7759559810919,6.08962573416775));
#87793=CARTESIAN_POINT('Ctrl Pts',(1.04581189579586,-20.7748618708056,6.0996105285919));
#87794=CARTESIAN_POINT('Ctrl Pts',(1.04785943431315,-20.7742356127999,6.11012462968347));
#87795=CARTESIAN_POINT('Ctrl Pts',(1.05,-20.7742356128,6.12111625914));
#87796=CARTESIAN_POINT('Origin',(2.57175827821E-16,-21.0742356128,0.729452270839));
#87797=CARTESIAN_POINT('Origin',(9.79717439318E-17,-22.3742356128,0.729452270839));
#87798=CARTESIAN_POINT('',(10.7000575594,-22.3742356128,-2.76302312605));
#87799=CARTESIAN_POINT('',(10.9449284019,-22.3742356128,-2.34954507713));
#87800=CARTESIAN_POINT('Origin',(-2.84607155346,-22.3742356128,5.53854202767));
#87801=CARTESIAN_POINT('Origin',(11.0821857629,-22.3742356128,-2.71007990903));
#87802=CARTESIAN_POINT('Origin',(-2.84607155346,-19.6742356128,5.53854202767));
#87803=CARTESIAN_POINT('',(11.2744572343,-19.3742356128,-1.7432341771));
#87804=CARTESIAN_POINT('',(12.6801076867,-19.3742356128,8.90771939699));
#87805=CARTESIAN_POINT('Origin',(-2.84607155346,-19.3742356128,5.53854202767));
#87806=CARTESIAN_POINT('Origin',(12.6801076867,-19.6742356128,8.90771939699));
#87807=CARTESIAN_POINT('Origin',(11.2744572343,-19.6742356128,-1.7432341771));
#87808=CARTESIAN_POINT('Origin',(1.77004158042E-15,-19.6742356128,0.580061096523));
#87809=CARTESIAN_POINT('',(12.1784262599,-19.3742356128,9.98548517727));
#87810=CARTESIAN_POINT('',(3.05,-19.3742356128,15.662287998));
#87811=CARTESIAN_POINT('Origin',(-2.6471818243E-16,-19.3742356128,0.580061096523));
#87812=CARTESIAN_POINT('',(3.109463736,-19.6742356128,15.9563357222));
#87813=CARTESIAN_POINT('Origin',(3.05,-19.6742356128,15.662287998));
#87814=CARTESIAN_POINT('',(12.4158607189067,-19.6742356128,10.1688560519572));
#87815=CARTESIAN_POINT('Origin',(4.37773950874E-16,-19.6742356128,0.580061096523));
#87816=CARTESIAN_POINT('Origin',(12.1784262599,-19.6742356128,9.98548517727));
#87817=CARTESIAN_POINT('Origin',(-2.84607155346,-19.6742356128,5.53854202767));
#87818=CARTESIAN_POINT('',(-1.59504721506E-14,-19.3742356128,-10.0919881826));
#87819=CARTESIAN_POINT('Ctrl Pts',(0.647446102181,-19.6742356128,-10.2675153591));
#87820=CARTESIAN_POINT('Ctrl Pts',(0.647446102180998,-19.6661145052506,
-10.2675153591));
#87821=CARTESIAN_POINT('Ctrl Pts',(0.646514029910601,-19.6579171021141,
-10.2673712859773));
#87822=CARTESIAN_POINT('Ctrl Pts',(0.64468675786068,-19.649672691115,-10.2670767778534));
#87823=CARTESIAN_POINT('Ctrl Pts',(0.642484067022575,-19.6397344399529,
-10.2667217621094));
#87824=CARTESIAN_POINT('Ctrl Pts',(0.638978968301581,-19.629725348657,-10.266147977288));
#87825=CARTESIAN_POINT('Ctrl Pts',(0.634153962808074,-19.6196963097844,
-10.2653265413293));
#87826=CARTESIAN_POINT('Ctrl Pts',(0.63040461389043,-19.611903082172,-10.2646882311704));
#87827=CARTESIAN_POINT('Ctrl Pts',(0.62585543611501,-19.6040982920229,-10.263899832074));
#87828=CARTESIAN_POINT('Ctrl Pts',(0.620491482566137,-19.5963142733431,
-10.2629448315708));
#87829=CARTESIAN_POINT('Ctrl Pts',(0.614628484782217,-19.5878060556909,
-10.2619009810261));
#87830=CARTESIAN_POINT('Ctrl Pts',(0.6078099922246,-19.5793188188891,-10.260651735256));
#87831=CARTESIAN_POINT('Ctrl Pts',(0.600023817872344,-19.5709021743201,
-10.2591844483976));
#87832=CARTESIAN_POINT('Ctrl Pts',(0.595862391014903,-19.5664037840742,
-10.2584002369654));
#87833=CARTESIAN_POINT('Ctrl Pts',(0.591425464005122,-19.5619252987295,
-10.25755382013));
#87834=CARTESIAN_POINT('Ctrl Pts',(0.586716534392515,-19.5574710301045,
-10.2566435084696));
#87835=CARTESIAN_POINT('Ctrl Pts',(0.579956784063687,-19.5510768500509,
-10.2553367402543));
#87836=CARTESIAN_POINT('Ctrl Pts',(0.572632437983098,-19.5447350403784,
-10.2539002805891));
#87837=CARTESIAN_POINT('Ctrl Pts',(0.56474609288734,-19.5384613170291,-10.2523376323413));
#87838=CARTESIAN_POINT('Ctrl Pts',(0.560802920339461,-19.5353244553545,
-10.2515563082174));
#87839=CARTESIAN_POINT('Ctrl Pts',(0.556719258945826,-19.5322045354405,
-10.2507434914554));
#87840=CARTESIAN_POINT('Ctrl Pts',(0.552495335544852,-19.5291037878776,
-10.2498990306019));
#87841=CARTESIAN_POINT('Ctrl Pts',(0.550383373844366,-19.5275534140961,
-10.2494768001751));
#87842=CARTESIAN_POINT('Ctrl Pts',(0.548235277312453,-19.5260077421965,
-10.2490468190963));
#87843=CARTESIAN_POINT('Ctrl Pts',(0.546049957467887,-19.5244670276599,
-10.2486090864764));
#87844=CARTESIAN_POINT('Ctrl Pts',(0.544524237517349,-19.5233913503798,
-10.2483034756556));
#87845=CARTESIAN_POINT('Ctrl Pts',(0.542513261054432,-19.521993581982,-10.247899197113));
#87846=CARTESIAN_POINT('Ctrl Pts',(0.540999194023679,-19.5209556339349,
-10.2475938147385));
#87847=CARTESIAN_POINT('Ctrl Pts',(0.540344631924859,-19.5205069077963,
-10.2474617917013));
#87848=CARTESIAN_POINT('Ctrl Pts',(0.53978335417908,-19.5201246497013,-10.2473484155898));
#87849=CARTESIAN_POINT('Ctrl Pts',(0.539396023575437,-19.5198615198152,
-10.2472701690991));
#87850=CARTESIAN_POINT('Ctrl Pts',(0.5365359708291,-19.5179185663116,-10.2466923962906));
#87851=CARTESIAN_POINT('Ctrl Pts',(0.533598144968601,-19.5159691901031,
-10.2460961657641));
#87852=CARTESIAN_POINT('Ctrl Pts',(0.530579239314274,-19.514015815137,-10.2454801288448));
#87853=CARTESIAN_POINT('Ctrl Pts',(0.520942696132119,-19.5077805152082,
-10.2435136989345));
#87854=CARTESIAN_POINT('Ctrl Pts',(0.510477444889386,-19.5015000483366,
-10.241345014764));
#87855=CARTESIAN_POINT('Ctrl Pts',(0.499188517402588,-19.4951987036651,
-10.238944290718));
#87856=CARTESIAN_POINT('Ctrl Pts',(0.488625147959329,-19.4893023568392,
-10.2366978651776));
#87857=CARTESIAN_POINT('Ctrl Pts',(0.477341422036914,-19.4833898482769,
-10.2342485041625));
#87858=CARTESIAN_POINT('Ctrl Pts',(0.465340425103763,-19.4775255046665,
-10.2315715082685));
#87859=CARTESIAN_POINT('Ctrl Pts',(0.45701593025548,-19.473457701096,-10.2297146093248));
#87860=CARTESIAN_POINT('Ctrl Pts',(0.448344875980685,-19.4694104929294,
-10.2277440364128));
#87861=CARTESIAN_POINT('Ctrl Pts',(0.439325215689106,-19.4654018145338,
-10.225653455845));
#87862=CARTESIAN_POINT('Ctrl Pts',(0.432718427317387,-19.462465507738,-10.224122131722));
#87863=CARTESIAN_POINT('Ctrl Pts',(0.425924517260663,-19.4595485265549,
-10.2225263148284));
#87864=CARTESIAN_POINT('Ctrl Pts',(0.418945134426883,-19.4566588813194,
-10.220863546663));
#87865=CARTESIAN_POINT('Ctrl Pts',(0.410691277831415,-19.453241570942,-10.2188971478689));
#87866=CARTESIAN_POINT('Ctrl Pts',(0.402176808635664,-19.4498619528698,
-10.2168368040588));
#87867=CARTESIAN_POINT('Ctrl Pts',(0.393402134457967,-19.4465329233363,
-10.2146787128479));
#87868=CARTESIAN_POINT('Ctrl Pts',(0.389014797369119,-19.4448684085696,
-10.2135996672424));
#87869=CARTESIAN_POINT('Ctrl Pts',(0.384562409197909,-19.4432165396316,
-10.2124961856045));
#87870=CARTESIAN_POINT('Ctrl Pts',(0.380045035728103,-19.4415789656171,
-10.2113678424595));
#87871=CARTESIAN_POINT('Ctrl Pts',(0.3777863489932,-19.4407601786098,-10.210803670887));
#87872=CARTESIAN_POINT('Ctrl Pts',(0.375511415934218,-19.4399449653191,
-10.2102332839411));
#87873=CARTESIAN_POINT('Ctrl Pts',(0.373220246465779,-19.4391335362231,
-10.2096566337111));
#87874=CARTESIAN_POINT('Ctrl Pts',(0.37126483257825,-19.4384410166409,-10.2091644877204));
#87875=CARTESIAN_POINT('Ctrl Pts',(0.368456147018735,-19.4374586741451,
-10.2084548315196));
#87876=CARTESIAN_POINT('Ctrl Pts',(0.366948540082698,-19.4369360561463,
-10.2080727559659));
#87877=CARTESIAN_POINT('Ctrl Pts',(0.366689675478217,-19.4368463196916,
-10.2080071514408));
#87878=CARTESIAN_POINT('Ctrl Pts',(0.366469198567963,-19.4367700102461,
-10.2079512492117));
#87879=CARTESIAN_POINT('Ctrl Pts',(0.366298039268187,-19.4367108132956,
-10.2079078469347));
#87880=CARTESIAN_POINT('Ctrl Pts',(0.356260121683919,-19.4332391111383,
-10.2053624492886));
#87881=CARTESIAN_POINT('Ctrl Pts',(0.344523522384,-19.4293734552193,-10.2023698293493));
#87882=CARTESIAN_POINT('Ctrl Pts',(0.331093866419504,-19.4252612897843,
-10.1988398420676));
#87883=CARTESIAN_POINT('Ctrl Pts',(0.319521466675984,-19.421717816865,-10.1957980348895));
#87884=CARTESIAN_POINT('Ctrl Pts',(0.306692181674625,-19.4179917981974,
-10.1923571037522));
#87885=CARTESIAN_POINT('Ctrl Pts',(0.292589265961312,-19.4141990783959,
-10.1884495017355));
#87886=CARTESIAN_POINT('Ctrl Pts',(0.27735466068823,-19.4101020115012,-10.1842283338935));
#87887=CARTESIAN_POINT('Ctrl Pts',(0.260641154924078,-19.4059290029001,
-10.1794643813728));
#87888=CARTESIAN_POINT('Ctrl Pts',(0.24244820239673,-19.4018711064667,-10.1740860690497));
#87889=CARTESIAN_POINT('Ctrl Pts',(0.233353953358138,-19.3998426550274,
-10.1713975713141));
#87890=CARTESIAN_POINT('Ctrl Pts',(0.223581355390598,-19.3977783193054,
-10.1684623406569));
#87891=CARTESIAN_POINT('Ctrl Pts',(0.213592020167185,-19.3958100852677,
-10.1654109992299));
#87892=CARTESIAN_POINT('Ctrl Pts',(0.212217188156573,-19.3955391972557,
-10.1649910431692));
#87893=CARTESIAN_POINT('Ctrl Pts',(0.210838283811837,-19.3952700611272,
-10.1645689166307));
#87894=CARTESIAN_POINT('Ctrl Pts',(0.209456541976758,-19.3950029537208,
-10.1641449888382));
#87895=CARTESIAN_POINT('Ctrl Pts',(0.20079382531649,-19.3933283458306,-10.1614872084504));
#87896=CARTESIAN_POINT('Ctrl Pts',(0.192018974991822,-19.3917356758629,
-10.1587578386406));
#87897=CARTESIAN_POINT('Ctrl Pts',(0.183437645601415,-19.3902770692547,
-10.1560558665988));
#87898=CARTESIAN_POINT('Ctrl Pts',(0.162049521978107,-19.3866416350422,
-10.1493214657353));
#87899=CARTESIAN_POINT('Ctrl Pts',(0.141963744437887,-19.3838261803671,
-10.1427586050297));
#87900=CARTESIAN_POINT('Ctrl Pts',(0.123218156746419,-19.3816330503464,
-10.1364476902696));
#87901=CARTESIAN_POINT('Ctrl Pts',(0.10191282119446,-19.3791404439919,-10.1292750073525));
#87902=CARTESIAN_POINT('Ctrl Pts',(0.0823386209659976,-19.377452038616,
-10.1224257079578));
#87903=CARTESIAN_POINT('Ctrl Pts',(0.0645043297250956,-19.3763190342603,
-10.116009220907));
#87904=CARTESIAN_POINT('Ctrl Pts',(0.0455284429160304,-19.3751135048609,
-10.1091820063939));
#87905=CARTESIAN_POINT('Ctrl Pts',(0.0285209561981343,-19.3745367951057,
-10.1028465719473));
#87906=CARTESIAN_POINT('Ctrl Pts',(0.0134553406264266,-19.3743288400826,
-10.0971275629238));
#87907=CARTESIAN_POINT('Ctrl Pts',(0.00878408254826948,-19.3742643613644,
-10.0953543219319));
#87908=CARTESIAN_POINT('Ctrl Pts',(0.00429934326341183,-19.3742356128,-10.0936401659177));
#87909=CARTESIAN_POINT('Ctrl Pts',(1.13381424745833E-15,-19.3742356128,
-10.0919881826));
#87910=CARTESIAN_POINT('',(10.3267865236,-19.3742356128,-3.3434289261));
#87911=CARTESIAN_POINT('Origin',(-2.84607155346,-19.3742356128,5.53854202767));
#87912=CARTESIAN_POINT('Origin',(10.3267865236652,-19.6742356128,-3.34342892613464));
#87913=CARTESIAN_POINT('Origin',(11.0821857629,-19.6742356128,-2.71007990903));
#87914=CARTESIAN_POINT('',(11.2159436339,-19.6742356128,-2.03747244546));
#87915=CARTESIAN_POINT('Ctrl Pts',(11.2159436339004,-19.6742356128,-2.03747244545784));
#87916=CARTESIAN_POINT('Ctrl Pts',(11.2159436338995,-19.6693613928602,-2.03747244545767));
#87917=CARTESIAN_POINT('Ctrl Pts',(11.2159655230008,-19.6640117573582,-2.03735938679454));
#87918=CARTESIAN_POINT('Ctrl Pts',(11.2160281016569,-19.6580667153257,-2.0370446657002));
#87919=CARTESIAN_POINT('Ctrl Pts',(11.2160872352179,-19.6524489611568,-2.03674727070616));
#87920=CARTESIAN_POINT('Ctrl Pts',(11.2161826332475,-19.6462990285337,-2.03627014239475));
#87921=CARTESIAN_POINT('Ctrl Pts',(11.2163384018002,-19.6395287243193,-2.03549712925787));
#87922=CARTESIAN_POINT('Ctrl Pts',(11.2164821525656,-19.6332807596527,-2.03478375529222));
#87923=CARTESIAN_POINT('Ctrl Pts',(11.2166773185298,-19.6265039597716,-2.03381837797931));
#87924=CARTESIAN_POINT('Ctrl Pts',(11.2169504658595,-19.619147424528,-2.03247155937132));
#87925=CARTESIAN_POINT('Ctrl Pts',(11.2171665294076,-19.6133282971438,-2.03140620607881));
#87926=CARTESIAN_POINT('Ctrl Pts',(11.2174315183419,-19.6071465569882,-2.03010151757666));
#87927=CARTESIAN_POINT('Ctrl Pts',(11.2177623828648,-19.6005900787551,-2.02847447984685));
#87928=CARTESIAN_POINT('Ctrl Pts',(11.218258591935,-19.5907570995657,-2.02603435458925));
#87929=CARTESIAN_POINT('Ctrl Pts',(11.2188255021808,-19.5818481179776,-2.02330895032003));
#87930=CARTESIAN_POINT('Ctrl Pts',(11.2194011752077,-19.5738403257838,-2.0205239658219));
#87931=CARTESIAN_POINT('Ctrl Pts',(11.2198012071017,-19.5682757567871,-2.01858869602226));
#87932=CARTESIAN_POINT('Ctrl Pts',(11.2202056395416,-19.5631455115216,-2.01662372036666));
#87933=CARTESIAN_POINT('Ctrl Pts',(11.2205960026702,-19.5584353020539,-2.01469186385905));
#87934=CARTESIAN_POINT('Ctrl Pts',(11.2210720637434,-19.5526910418769,-2.01233589933555));
#87935=CARTESIAN_POINT('Ctrl Pts',(11.2215309766499,-19.5475701479139,-2.01003015077224));
#87936=CARTESIAN_POINT('Ctrl Pts',(11.2219592146484,-19.5430379937272,-2.00786819701386));
#87937=CARTESIAN_POINT('Ctrl Pts',(11.2221733336476,-19.5407719166338,-2.00678722013467));
#87938=CARTESIAN_POINT('Ctrl Pts',(11.2223799594567,-19.5386529605451,-2.00574183086384));
#87939=CARTESIAN_POINT('Ctrl Pts',(11.222578261594,-19.5366766942524,-2.0047416089727));
#87940=CARTESIAN_POINT('Ctrl Pts',(11.2226959635169,-19.5355036844903,-2.00414792883612));
#87941=CARTESIAN_POINT('Ctrl Pts',(11.2227632467704,-19.5348401327041,-2.00380636847078));
#87942=CARTESIAN_POINT('Ctrl Pts',(11.2228640658506,-19.5338660918148,-2.00330063603375));
#87943=CARTESIAN_POINT('Ctrl Pts',(11.22293310499,-19.5331990856817,-2.00295431932273));
#87944=CARTESIAN_POINT('Ctrl Pts',(11.2230179020481,-19.5323865415852,-2.0025308549887));
#87945=CARTESIAN_POINT('Ctrl Pts',(11.2231477904519,-19.5311716776,-2.00188466056667));
#87946=CARTESIAN_POINT('Ctrl Pts',(11.2243488190571,-19.5199382929807,-1.99590954683396));
#87947=CARTESIAN_POINT('Ctrl Pts',(11.2256255742843,-19.5095883708649,-1.98949289875886));
#87948=CARTESIAN_POINT('Ctrl Pts',(11.2269421893286,-19.5000727519268,-1.9828372680661));
#87949=CARTESIAN_POINT('Ctrl Pts',(11.2283389310385,-19.4899780306761,-1.97577658845831));
#87950=CARTESIAN_POINT('Ctrl Pts',(11.2297804517346,-19.4808214431763,-1.96844723872592));
#87951=CARTESIAN_POINT('Ctrl Pts',(11.2312343309138,-19.4725140943552,-1.96104193633524));
#87952=CARTESIAN_POINT('Ctrl Pts',(11.2327789135453,-19.4636884732944,-1.95317463785666));
#87953=CARTESIAN_POINT('Ctrl Pts',(11.2343374115243,-19.4558204434581,-1.94522171060417));
#87954=CARTESIAN_POINT('Ctrl Pts',(11.2358832957294,-19.448784286417,-1.93735720972956));
#87955=CARTESIAN_POINT('Ctrl Pts',(11.237350034937,-19.4421083611644,-1.92989534955764));
#87956=CARTESIAN_POINT('Ctrl Pts',(11.238805608868,-19.4361805746817,-1.92251221094851));
#87957=CARTESIAN_POINT('Ctrl Pts',(11.2402365654223,-19.4308894383749,-1.91531434798852));
#87958=CARTESIAN_POINT('Ctrl Pts',(11.2424783121132,-19.4226003066944,-1.90403812480444));
#87959=CARTESIAN_POINT('Ctrl Pts',(11.2447614681787,-19.4153947337217,-1.8925549054251));
#87960=CARTESIAN_POINT('Ctrl Pts',(11.2470547932876,-19.4091625001044,-1.88102151742434));
#87961=CARTESIAN_POINT('Ctrl Pts',(11.2495134495914,-19.4024809701238,-1.86865666038664));
#87962=CARTESIAN_POINT('Ctrl Pts',(11.2519838185799,-19.3969172471324,-1.85623401887946));
#87963=CARTESIAN_POINT('Ctrl Pts',(11.2544393837905,-19.392334226818,-1.84388652056322));
#87964=CARTESIAN_POINT('Ctrl Pts',(11.2569925855012,-19.3875689795923,-1.83104806948533));
#87965=CARTESIAN_POINT('Ctrl Pts',(11.2595299095001,-19.3838631500315,-1.81829021968229));
#87966=CARTESIAN_POINT('Ctrl Pts',(11.2620327668194,-19.3810753841191,-1.80570587411781));
#87967=CARTESIAN_POINT('Ctrl Pts',(11.2646923382581,-19.3781130647965,-1.79233357127776));
#87968=CARTESIAN_POINT('Ctrl Pts',(11.2673131246881,-19.3761865920875,-1.77915651243343));
#87969=CARTESIAN_POINT('Ctrl Pts',(11.2698832252856,-19.3751535179302,-1.76623371991554));
#87970=CARTESIAN_POINT('Ctrl Pts',(11.2714264017639,-19.3745332248019,-1.75847443241259));
#87971=CARTESIAN_POINT('Ctrl Pts',(11.2729514923844,-19.3742356128001,-1.75080586802915));
#87972=CARTESIAN_POINT('Ctrl Pts',(11.2744572343,-19.3742356128,-1.7432341771));
#87973=CARTESIAN_POINT('',(10.5566756949,-19.6742356128,-3.15068305993));
#87974=CARTESIAN_POINT('Origin',(11.0821857629,-19.6742356128,-2.71007990903));
#87975=CARTESIAN_POINT('Origin',(10.3267865236,-19.6742356128,-3.3434289261));
#87976=CARTESIAN_POINT('Origin',(11.0821857629,-19.3742356128,-2.71007990903));
#87977=CARTESIAN_POINT('Origin',(12.5441720511,-22.5760378048,9.34841724773));
#87978=CARTESIAN_POINT('',(12.8222448231109,-23.4742356815,9.46100293550673));
#87979=CARTESIAN_POINT('Origin',(12.5441720511,-23.4742356478461,9.34841724773));
#87980=CARTESIAN_POINT('',(12.8222448081,-25.4742356128,9.46100295649));
#87981=CARTESIAN_POINT('',(12.8222448081,-21.2742356128,9.46100295649));
#87982=CARTESIAN_POINT('Origin',(12.5441720511,-25.4742356128,9.34841724773));
#87983=CARTESIAN_POINT('Origin',(12.5441720511,-25.4742356128,9.34841724773));
#87984=CARTESIAN_POINT('Origin',(12.5441720511,-25.4742356128,9.34841724773));
#87985=CARTESIAN_POINT('Origin',(10.0415172382,-25.4742356128,8.33514586886));
#87986=CARTESIAN_POINT('Origin',(10.0415172382,-25.4742356128,8.33514586886));
#87987=CARTESIAN_POINT('Origin',(10.0415172382,-19.6742356128,8.33514586886));
#87988=CARTESIAN_POINT('Origin',(10.0415172382,-19.3742356128,8.33514586886));
#87989=CARTESIAN_POINT('Origin',(10.0415172382,-19.6742356128,8.33514586886));
#87990=CARTESIAN_POINT('Origin',(10.0415172382,-21.2742356128,8.33514586886));
#87991=CARTESIAN_POINT('',(12.4158608431,-21.2742356128,10.1688558911));
#87992=CARTESIAN_POINT('Ctrl Pts',(12.822244843051,-23.4742356815,9.46100291845212));
#87993=CARTESIAN_POINT('Ctrl Pts',(12.8222448374688,-23.4526557884998,9.46100292804296));
#87994=CARTESIAN_POINT('Ctrl Pts',(12.8227658011016,-23.4310761714824,9.459718249267));
#87995=CARTESIAN_POINT('Ctrl Pts',(12.8237956782946,-23.4096767931088,9.45716500907838));
#87996=CARTESIAN_POINT('Ctrl Pts',(12.8249218353694,-23.3862768561876,9.45437307473734));
#87997=CARTESIAN_POINT('Ctrl Pts',(12.8266564446377,-23.3630965146334,9.45006425351064));
#87998=CARTESIAN_POINT('Ctrl Pts',(12.8289489787169,-23.3403539792507,9.4443040829754));
#87999=CARTESIAN_POINT('Ctrl Pts',(12.8312709606729,-23.3173193132581,9.43846992235491));
#88000=CARTESIAN_POINT('Ctrl Pts',(12.8341646949754,-23.2947342337854,9.43114748157285));
#88001=CARTESIAN_POINT('Ctrl Pts',(12.8375494613154,-23.2727938554516,9.42244323588751));
#88002=CARTESIAN_POINT('Ctrl Pts',(12.8410023873676,-23.250411659361,9.41356371107774));
#88003=CARTESIAN_POINT('Ctrl Pts',(12.8449656668396,-23.2287009550523,9.40324680779877));
#88004=CARTESIAN_POINT('Ctrl Pts',(12.8493339497345,-23.2078282931751,9.39163588847771));
#88005=CARTESIAN_POINT('Ctrl Pts',(12.8533668576591,-23.1885581301571,9.38091639762304));
#88006=CARTESIAN_POINT('Ctrl Pts',(12.8577443119826,-23.1700021065795,9.36909474059184));
#88007=CARTESIAN_POINT('Ctrl Pts',(12.8623765483007,-23.1522553698924,9.35629852758267));
#88008=CARTESIAN_POINT('Ctrl Pts',(12.8676258737502,-23.1321444795705,9.34179765111725));
#88009=CARTESIAN_POINT('Ctrl Pts',(12.8732011777363,-23.1130741318264,9.3260463447321));
#88010=CARTESIAN_POINT('Ctrl Pts',(12.8789692176796,-23.0951288263937,9.30924271806145));
#88011=CARTESIAN_POINT('Ctrl Pts',(12.8847323055415,-23.0771989276877,9.29245351794285));
#88012=CARTESIAN_POINT('Ctrl Pts',(12.8906877245128,-23.0603914552665,9.27461404125843));
#88013=CARTESIAN_POINT('Ctrl Pts',(12.8967175034202,-23.0447417766193,9.25591265355548));
#88014=CARTESIAN_POINT('Ctrl Pts',(12.9032960762988,-23.0276677589662,9.23550917876373));
#88015=CARTESIAN_POINT('Ctrl Pts',(12.909961941791,-23.0119710592708,9.21408281923307));
#88016=CARTESIAN_POINT('Ctrl Pts',(12.9165837263722,-22.997646095339,9.1918614547601));
#88017=CARTESIAN_POINT('Ctrl Pts',(12.9229613039847,-22.9838494264575,9.17045959928658));
#88018=CARTESIAN_POINT('Ctrl Pts',(12.9292980187867,-22.9713240464602,9.14832050002835));
#88019=CARTESIAN_POINT('Ctrl Pts',(12.9354980002173,-22.9600302011921,9.12562740036042));
#88020=CARTESIAN_POINT('Ctrl Pts',(12.9422358704374,-22.9477565412539,9.10096552642308));
#88021=CARTESIAN_POINT('Ctrl Pts',(12.9488130289529,-22.9369364542937,9.07564536621217));
#88022=CARTESIAN_POINT('Ctrl Pts',(12.9551362385969,-22.9274915788356,9.04986970620133));
#88023=CARTESIAN_POINT('Ctrl Pts',(12.9614594482409,-22.9180467033774,9.02409404619048));
#88024=CARTESIAN_POINT('Ctrl Pts',(12.9675285501681,-22.9099757205391,8.99786337398523));
#88025=CARTESIAN_POINT('Ctrl Pts',(12.9732844031999,-22.9031898545,8.97133867789998));
#88026=CARTESIAN_POINT('Ctrl Pts',(10.5755264816041,-22.073347939028,-3.51114426672837));
#88027=CARTESIAN_POINT('Ctrl Pts',(10.6189732998864,-22.0734675796473,-3.44670824878185));
#88028=CARTESIAN_POINT('Ctrl Pts',(10.6415548738579,-22.073587220165,-3.36820356962979));
#88029=CARTESIAN_POINT('Ctrl Pts',(10.6370073188241,-22.0736899806765,-3.28463114868135));
#88030=CARTESIAN_POINT('Ctrl Pts',(10.6060354193007,-22.0737598091151,-3.20904188084407));
#88031=CARTESIAN_POINT('Ctrl Pts',(10.5558506553124,-22.0737923598628,-3.14970279055262));
#88032=CARTESIAN_POINT('Ctrl Pts',(10.5754458724638,-22.1652998410927,-3.51126386273525));
#88033=CARTESIAN_POINT('Ctrl Pts',(10.618903371002,-22.1530274460811,-3.44681323084733));
#88034=CARTESIAN_POINT('Ctrl Pts',(10.641496283718,-22.1407550510704,-3.36829411184493));
#88035=CARTESIAN_POINT('Ctrl Pts',(10.6369593909186,-22.1302141599519,-3.28470925230792));
#88036=CARTESIAN_POINT('Ctrl Pts',(10.6059957968922,-22.1230513527872,-3.20911112586287));
#88037=CARTESIAN_POINT('Ctrl Pts',(10.5558161001343,-22.1197123858053,-3.14976720010066));
#88038=CARTESIAN_POINT('Ctrl Pts',(10.5857997847365,-22.2572834900482,-3.49590425496629));
#88039=CARTESIAN_POINT('Ctrl Pts',(10.6278856426866,-22.2326147094154,-3.4333298375838));
#88040=CARTESIAN_POINT('Ctrl Pts',(10.6490223141032,-22.2079459286819,-3.35666455173243));
#88041=CARTESIAN_POINT('Ctrl Pts',(10.6431159920152,-22.1867575798953,-3.2746766456359));
#88042=CARTESIAN_POINT('Ctrl Pts',(10.6110854924619,-22.1723594349106,-3.20021597700034));
#88043=CARTESIAN_POINT('Ctrl Pts',(10.5602546815746,-22.1656479230153,-3.14149308533282));
#88044=CARTESIAN_POINT('Ctrl Pts',(10.6065715306299,-22.3443167259089,-3.46513076367994));
#88045=CARTESIAN_POINT('Ctrl Pts',(10.6459119686815,-22.3078279887505,-3.40630062234996));
#88046=CARTESIAN_POINT('Ctrl Pts',(10.6641106942264,-22.2713392514914,-3.3333218087324));
#88047=CARTESIAN_POINT('Ctrl Pts',(10.6554225922274,-22.2400430269978,-3.2544822528469));
#88048=CARTESIAN_POINT('Ctrl Pts',(10.6212346959669,-22.2188693850443,-3.18223722148648));
#88049=CARTESIAN_POINT('Ctrl Pts',(10.5691144274879,-22.209114211317,-3.12470547607949));
#88050=CARTESIAN_POINT('Ctrl Pts',(10.6748166371955,-22.5209266907492,-3.36289055825833));
#88051=CARTESIAN_POINT('Ctrl Pts',(10.7052316290396,-22.4602477908528,-3.31650182759889));
#88052=CARTESIAN_POINT('Ctrl Pts',(10.7138733888551,-22.3995688908556,-3.25576778202096));
#88053=CARTESIAN_POINT('Ctrl Pts',(10.6960859309467,-22.3476657503612,-3.18746418308737));
#88054=CARTESIAN_POINT('Ctrl Pts',(10.6546593558206,-22.3128693591781,-3.12274837994517));
#88055=CARTESIAN_POINT('Ctrl Pts',(10.5979621503895,-22.2973226488988,-3.06936176748442));
#88056=CARTESIAN_POINT('Ctrl Pts',(10.7770676343791,-22.6313508349927,-3.20587132888339));
#88057=CARTESIAN_POINT('Ctrl Pts',(10.7947683037157,-22.5535956183832,-3.17804091297403));
#88058=CARTESIAN_POINT('Ctrl Pts',(10.7887694347283,-22.4758404017738,-3.13498582812424));
#88059=CARTESIAN_POINT('Ctrl Pts',(10.7560189786525,-22.4102922092715,-3.08108257829107));
#88060=CARTESIAN_POINT('Ctrl Pts',(10.7022156734909,-22.3684261450212,-3.02593957847265));
#88061=CARTESIAN_POINT('Ctrl Pts',(10.6376381360204,-22.3525284903903,-2.97725090948219));
#88062=CARTESIAN_POINT('Ctrl Pts',(10.8411323863464,-22.6664009565298,-3.10546741472568));
#88063=CARTESIAN_POINT('Ctrl Pts',(10.8511507365709,-22.582155535137,-3.08929951273552));
#88064=CARTESIAN_POINT('Ctrl Pts',(10.8360597596591,-22.4979101137442,-3.05723132474782));
#88065=CARTESIAN_POINT('Ctrl Pts',(10.7937463726032,-22.4275879287889,-3.01219357566858));
#88066=CARTESIAN_POINT('Ctrl Pts',(10.7317180936056,-22.3842297203853,-2.96288258512268));
#88067=CARTESIAN_POINT('Ctrl Pts',(10.6616004183053,-22.3700818046728,-2.91694755475329));
#88068=CARTESIAN_POINT('Ctrl Pts',(10.9026335403798,-22.6742830962032,-3.00661736786854));
#88069=CARTESIAN_POINT('Ctrl Pts',(10.9059308011903,-22.5846434461728,-3.00123595319039));
#88070=CARTESIAN_POINT('Ctrl Pts',(10.8808935813686,-22.4950037961424,-2.97821475154161));
#88071=CARTESIAN_POINT('Ctrl Pts',(10.8265348140848,-22.4221227996667,-2.93850991788712));
#88072=CARTESIAN_POINT('Ctrl Pts',(10.754120168993,-22.3814334073002,-2.89056167992165));
#88073=CARTESIAN_POINT('Ctrl Pts',(10.6779444379831,-22.3741354186777,-2.84322868920662));
#88074=CARTESIAN_POINT('Ctrl Pts',(10.9562463120162,-22.6742354344034,-2.91912533867425));
#88075=CARTESIAN_POINT('Ctrl Pts',(10.9562214113882,-22.5796388423537,-2.91916597451867));
#88076=CARTESIAN_POINT('Ctrl Pts',(10.9244049920089,-22.4850422503039,-2.89972567303062));
#88077=CARTESIAN_POINT('Ctrl Pts',(10.8603955187549,-22.4104207249433,-2.86054658143736));
#88078=CARTESIAN_POINT('Ctrl Pts',(10.7795412374011,-22.3736906146549,-2.81102307954316));
#88079=CARTESIAN_POINT('Ctrl Pts',(10.6988848574274,-22.3742405364324,-2.76159881818277));
#88080=CARTESIAN_POINT('',(10.5566756928877,-22.0742356130312,-3.15068306070111));
#88081=CARTESIAN_POINT('Ctrl Pts',(10.5566756909963,-22.0742356130312,-3.15068305522312));
#88082=CARTESIAN_POINT('Ctrl Pts',(10.5566756934735,-22.0899525193036,-3.15068305815888));
#88083=CARTESIAN_POINT('Ctrl Pts',(10.5573623074021,-22.1056755510411,-3.14957422284101));
#88084=CARTESIAN_POINT('Ctrl Pts',(10.5586671517577,-22.1211849491845,-3.14730288034606));
#88085=CARTESIAN_POINT('Ctrl Pts',(10.559949323621,-22.136424861771,-3.14507100385689));
#88086=CARTESIAN_POINT('Ctrl Pts',(10.5618278097496,-22.1514578348887,-3.14171667117984));
#88087=CARTESIAN_POINT('Ctrl Pts',(10.5642316242454,-22.1660850328081,-3.13723770193223));
#88088=CARTESIAN_POINT('Ctrl Pts',(10.5666187611341,-22.1806107475803,-3.13278980766549));
#88089=CARTESIAN_POINT('Ctrl Pts',(10.5695234657495,-22.1947357268319,-3.12723298635599));
#88090=CARTESIAN_POINT('Ctrl Pts',(10.5728784346858,-22.208284065637,-3.12061247077665));
#88091=CARTESIAN_POINT('Ctrl Pts',(10.5762351667071,-22.2218395242907,-3.11398847602029));
#88092=CARTESIAN_POINT('Ctrl Pts',(10.5800422752663,-22.234817250828,-3.10629997477472));
#88093=CARTESIAN_POINT('Ctrl Pts',(10.5842410421963,-22.2470679396434,-3.09763643012156));
#88094=CARTESIAN_POINT('Ctrl Pts',(10.5882460917805,-22.2587534218252,-3.08937259302623));
#88095=CARTESIAN_POINT('Ctrl Pts',(10.5926074196856,-22.2697773332744,-3.08022227091879));
#88096=CARTESIAN_POINT('Ctrl Pts',(10.5972849163347,-22.2800381439071,-3.0702956139941));
#88097=CARTESIAN_POINT('Ctrl Pts',(10.6012330710361,-22.2886990304408,-3.06191677801711));
#88098=CARTESIAN_POINT('Ctrl Pts',(10.6054661382905,-22.296879480602,-3.05296180738476));
#88099=CARTESIAN_POINT('Ctrl Pts',(10.6098478833313,-22.3044716723759,-3.04340827272847));
#88100=CARTESIAN_POINT('Ctrl Pts',(10.6140927795382,-22.3118267479824,-3.03415311008243));
#88101=CARTESIAN_POINT('Ctrl Pts',(10.6184766453214,-22.3186295557672,-3.02433701732395));
#88102=CARTESIAN_POINT('Ctrl Pts',(10.6228936503569,-22.3248195086567,-3.0139710852086));
#88103=CARTESIAN_POINT('Ctrl Pts',(10.6272969718839,-22.3309902855951,-3.0036372658752));
#88104=CARTESIAN_POINT('Ctrl Pts',(10.6317327207341,-22.3365518968271,-2.99275788444388));
#88105=CARTESIAN_POINT('Ctrl Pts',(10.6361223115085,-22.3414844523268,-2.98136320543062));
#88106=CARTESIAN_POINT('Ctrl Pts',(10.6404844891338,-22.3463862038436,-2.97003968658923));
#88107=CARTESIAN_POINT('Ctrl Pts',(10.6448007098638,-22.3506668911406,-2.95820823841755));
#88108=CARTESIAN_POINT('Ctrl Pts',(10.6490263221702,-22.3543462073631,-2.9459038456027));
#88109=CARTESIAN_POINT('Ctrl Pts',(10.6531973013616,-22.3579779535552,-2.93375853678779));
#88110=CARTESIAN_POINT('Ctrl Pts',(10.6572797194545,-22.3610241695016,-2.92115327288598));
#88111=CARTESIAN_POINT('Ctrl Pts',(10.6612670512316,-22.3635379124603,-2.90811347414347));
#88112=CARTESIAN_POINT('Ctrl Pts',(10.6651259957032,-22.3659707159077,-2.89549354129583));
#88113=CARTESIAN_POINT('Ctrl Pts',(10.6688956905757,-22.3679053423702,-2.88246710423552));
#88114=CARTESIAN_POINT('Ctrl Pts',(10.6726076695519,-22.3694148940626,-2.86903976949775));
#88115=CARTESIAN_POINT('Ctrl Pts',(10.6762290310023,-22.3708875942965,-2.85594022536955));
#88116=CARTESIAN_POINT('Ctrl Pts',(10.6797951054022,-22.3719562403948,-2.84245930266272));
#88117=CARTESIAN_POINT('Ctrl Pts',(10.6833753682069,-22.3727050906066,-2.82858037372522));
#88118=CARTESIAN_POINT('Ctrl Pts',(10.6867948611643,-22.3734203140874,-2.81532467090519));
#88119=CARTESIAN_POINT('Ctrl Pts',(10.6902269714035,-22.3738442904274,-2.80170567475361));
#88120=CARTESIAN_POINT('Ctrl Pts',(10.6937740147699,-22.3740583609835,-2.78768927445374));
#88121=CARTESIAN_POINT('Ctrl Pts',(10.6958203922006,-22.3741818636051,-2.77960286493741));
#88122=CARTESIAN_POINT('Ctrl Pts',(10.6979058195049,-22.3742356128001,-2.77138381588323));
#88123=CARTESIAN_POINT('Ctrl Pts',(10.7000575594,-22.3742356128,-2.76302312605));
#88124=CARTESIAN_POINT('Origin',(10.7018662383156,-22.6721143297048,-2.76413150880985));
#88125=CARTESIAN_POINT('Origin',(10.3289417811658,-22.0742353985912,-3.34331623669745));
#88126=CARTESIAN_POINT('Origin',(-2.84607155346,-22.6742356128,5.53854202767));
#88127=CARTESIAN_POINT('Origin',(10.9449284019752,-22.6742356128,-2.34954507716718));
#88128=CARTESIAN_POINT('Ctrl Pts',(11.2053401891,-22.6742356128,-2.49849372966));
#88129=CARTESIAN_POINT('Ctrl Pts',(11.2053401891,-22.5799878332,-2.49849372966));
#88130=CARTESIAN_POINT('Ctrl Pts',(11.1732131726,-22.4857400536,-2.48011792621));
#88131=CARTESIAN_POINT('Ctrl Pts',(11.1085499535,-22.4112466293,-2.44313227564));
#88132=CARTESIAN_POINT('Ctrl Pts',(11.0267391777,-22.3742356128,-2.39633867638));
#88133=CARTESIAN_POINT('Ctrl Pts',(10.9449284019,-22.3742356128,-2.34954507713));
#88134=CARTESIAN_POINT('Ctrl Pts',(11.2476948874,-22.6742356128,-2.42444362923));
#88135=CARTESIAN_POINT('Ctrl Pts',(11.2450653313,-22.5840941242,-2.429040968));
#88136=CARTESIAN_POINT('Ctrl Pts',(11.2130113811,-22.4939526355,-2.41703302845));
#88137=CARTESIAN_POINT('Ctrl Pts',(11.1517699452,-22.4209218727,-2.38727936284));
#88138=CARTESIAN_POINT('Ctrl Pts',(11.0744430753,-22.3806857596,-2.34601859644));
#88139=CARTESIAN_POINT('Ctrl Pts',(10.9959501219,-22.3742356128,-2.30169489009));
#88140=CARTESIAN_POINT('Ctrl Pts',(11.2941946283,-22.6686213022,-2.34203463014));
#88141=CARTESIAN_POINT('Ctrl Pts',(11.2868586676,-22.5829413188,-2.35499473105));
#88142=CARTESIAN_POINT('Ctrl Pts',(11.2526857413,-22.4972613355,-2.35302785728));
#88143=CARTESIAN_POINT('Ctrl Pts',(11.1928402247,-22.426280398,-2.33351209766));
#88144=CARTESIAN_POINT('Ctrl Pts',(11.1189291588,-22.3836825181,-2.2998966476));
#88145=CARTESIAN_POINT('Ctrl Pts',(11.043868081,-22.3714284849,-2.25918468729));
#88146=CARTESIAN_POINT('Ctrl Pts',(11.3417981924,-22.6467118109,-2.25595171063));
#88147=CARTESIAN_POINT('Ctrl Pts',(11.3291442479,-22.5660000486,-2.27877967267));
#88148=CARTESIAN_POINT('Ctrl Pts',(11.2910933501,-22.4852882864,-2.28766776945));
#88149=CARTESIAN_POINT('Ctrl Pts',(11.229550879,-22.4176465288,-2.27867532762));
#88150=CARTESIAN_POINT('Ctrl Pts',(11.1557537306,-22.375311083,-2.25331234023));
#88151=CARTESIAN_POINT('Ctrl Pts',(11.0817600114,-22.3604736068,-2.21745676256));
#88152=CARTESIAN_POINT('Ctrl Pts',(11.4353537652,-22.5603047021,-2.08352845036));
#88153=CARTESIAN_POINT('Ctrl Pts',(11.4121163918,-22.4942390833,-2.12677174602));
#88154=CARTESIAN_POINT('Ctrl Pts',(11.3657157526,-22.4281734646,-2.15766880717));
#88155=CARTESIAN_POINT('Ctrl Pts',(11.2994862528,-22.3717132431,-2.16962607727));
#88156=CARTESIAN_POINT('Ctrl Pts',(11.2242843437,-22.3339703351,-2.16051799049));
#88157=CARTESIAN_POINT('Ctrl Pts',(11.1508960681,-22.3172702763,-2.13427099913));
#88158=CARTESIAN_POINT('Ctrl Pts',(11.5032693058,-22.4004263802,-1.95414386857));
#88159=CARTESIAN_POINT('Ctrl Pts',(11.4721201637,-22.3564749274,-2.01366537708));
#88160=CARTESIAN_POINT('Ctrl Pts',(11.418463566,-22.3125234745,-2.06143417372));
#88161=CARTESIAN_POINT('Ctrl Pts',(11.3465841747,-22.2747985542,-2.0888955933));
#88162=CARTESIAN_POINT('Ctrl Pts',(11.2678343078,-22.2492105131,-2.09172776553));
#88163=CARTESIAN_POINT('Ctrl Pts',(11.1928782665,-22.237330862,-2.07277075552));
#88164=CARTESIAN_POINT('Ctrl Pts',(11.5284593408,-22.2976444921,-1.90521795022));
#88165=CARTESIAN_POINT('Ctrl Pts',(11.4944206426,-22.2676340437,-1.97094002685));
#88166=CARTESIAN_POINT('Ctrl Pts',(11.4380739731,-22.2376235953,-2.02511044406));
#88167=CARTESIAN_POINT('Ctrl Pts',(11.3640715597,-22.2118199507,-2.05839415541));
#88168=CARTESIAN_POINT('Ctrl Pts',(11.283947635,-22.1942244807,-2.0655995494));
#88169=CARTESIAN_POINT('Ctrl Pts',(11.208324537,-22.1859402315,-2.04918926595));
#88170=CARTESIAN_POINT('Ctrl Pts',(11.5410916547,-22.1859264501,-1.88073379583));
#88171=CARTESIAN_POINT('Ctrl Pts',(11.5055896574,-22.1709238273,-1.9495777849));
#88172=CARTESIAN_POINT('Ctrl Pts',(11.4478685938,-22.1559212045,-2.00696368603));
#88173=CARTESIAN_POINT('Ctrl Pts',(11.3727622471,-22.1430213573,-2.04316893107));
#88174=CARTESIAN_POINT('Ctrl Pts',(11.2919149591,-22.1342242685,-2.05258032919));
#88175=CARTESIAN_POINT('Ctrl Pts',(11.2159437174,-22.1300808784,-2.0374723572));
#88176=CARTESIAN_POINT('Ctrl Pts',(11.5410916367,-22.0742358827,-1.88073379256));
#88177=CARTESIAN_POINT('Ctrl Pts',(11.5055896399,-22.0742358104,-1.94957779219));
#88178=CARTESIAN_POINT('Ctrl Pts',(11.4478685736,-22.0742357381,-2.00696370221));
#88179=CARTESIAN_POINT('Ctrl Pts',(11.3727622216,-22.074235676,-2.04316895153));
#88180=CARTESIAN_POINT('Ctrl Pts',(11.2919149284,-22.0742356336,-2.05258034776));
#88181=CARTESIAN_POINT('Ctrl Pts',(11.2159436836,-22.0742356136,-2.03747236903));
#88182=CARTESIAN_POINT('',(11.2159436600663,-22.0742356133472,-2.03747240750538));
#88183=CARTESIAN_POINT('Ctrl Pts',(10.9449284019,-22.3742356128,-2.34954507713));
#88184=CARTESIAN_POINT('Ctrl Pts',(10.9555579269,-22.3742356128,-2.33957628816333));
#88185=CARTESIAN_POINT('Ctrl Pts',(10.9660214617852,-22.3740877440668,-2.32988311338671));
#88186=CARTESIAN_POINT('Ctrl Pts',(10.9762103266067,-22.3736977371534,-2.3203917889783));
#88187=CARTESIAN_POINT('Ctrl Pts',(10.9866077289775,-22.3732997478899,-2.31070620372078));
#88188=CARTESIAN_POINT('Ctrl Pts',(10.99671966122,-22.3726496161805,-2.30123099399582));
#88189=CARTESIAN_POINT('Ctrl Pts',(11.006479915341,-22.3716678922283,-2.29191758434368));
#88190=CARTESIAN_POINT('Ctrl Pts',(11.0167560942109,-22.3706342745777,-2.28211187003672));
#88191=CARTESIAN_POINT('Ctrl Pts',(11.0266429407752,-22.3692329814202,-2.27248559795379));
#88192=CARTESIAN_POINT('Ctrl Pts',(11.0361092934492,-22.3673949047112,-2.26301295646525));
#88193=CARTESIAN_POINT('Ctrl Pts',(11.0462075675716,-22.3654341281477,-2.2529079737218));
#88194=CARTESIAN_POINT('Ctrl Pts',(11.0558281166974,-22.3629761417554,-2.24297794072533));
#88195=CARTESIAN_POINT('Ctrl Pts',(11.0649742091976,-22.3599654715829,-2.23322425948526));
#88196=CARTESIAN_POINT('Ctrl Pts',(11.0752293070643,-22.3565897439415,-2.22228789997717));
#88197=CARTESIAN_POINT('Ctrl Pts',(11.0848893155074,-22.3525186606634,-2.21157331885061));
#88198=CARTESIAN_POINT('Ctrl Pts',(11.0939918679988,-22.3477145948015,-2.20112134524111));
#88199=CARTESIAN_POINT('Ctrl Pts',(11.1031456188729,-22.3428835079033,-2.19061058327036));
#88200=CARTESIAN_POINT('Ctrl Pts',(11.1117380324015,-22.3373113929668,-2.18036628908064));
#88201=CARTESIAN_POINT('Ctrl Pts',(11.1198079816964,-22.3309999394505,-2.17045843415635));
#88202=CARTESIAN_POINT('Ctrl Pts',(11.1271861983587,-22.3252294854122,-2.16139985180119));
#88203=CARTESIAN_POINT('Ctrl Pts',(11.1341290619681,-22.3188416151799,-2.1526233573693));
#88204=CARTESIAN_POINT('Ctrl Pts',(11.1406408102254,-22.3118641259116,-2.14419334888398));
#88205=CARTESIAN_POINT('Ctrl Pts',(11.1491541793956,-22.3027418534165,-2.13317207295198));
#88206=CARTESIAN_POINT('Ctrl Pts',(11.1569273589696,-22.2926111216346,-2.12274422351284));
#88207=CARTESIAN_POINT('Ctrl Pts',(11.1639866875261,-22.2815665889067,-2.11305404282817));
#88208=CARTESIAN_POINT('Ctrl Pts',(11.1713496846492,-22.2700469575351,-2.10294702316865));
#88209=CARTESIAN_POINT('Ctrl Pts',(11.177935601256,-22.2575335578597,-2.09364320727755));
#88210=CARTESIAN_POINT('Ctrl Pts',(11.1837492551854,-22.2441835831467,-2.08529357693297));
#88211=CARTESIAN_POINT('Ctrl Pts',(11.1898122988749,-22.2302609312447,-2.0765857704167));
#88212=CARTESIAN_POINT('Ctrl Pts',(11.1950346999939,-22.2154289170774,-2.06891671406967));
#88213=CARTESIAN_POINT('Ctrl Pts',(11.1994045937774,-22.1999120981238,-2.06243120336764));
#88214=CARTESIAN_POINT('Ctrl Pts',(11.203749759914,-22.1844830832312,-2.05598239182281));
#88215=CARTESIAN_POINT('Ctrl Pts',(11.2072511776712,-22.1683779027648,-2.05070452963748));
#88216=CARTESIAN_POINT('Ctrl Pts',(11.2098925170254,-22.151850614658,-2.04670170035793));
#88217=CARTESIAN_POINT('Ctrl Pts',(11.2124164316883,-22.1360580718618,-2.04287682284054));
#88218=CARTESIAN_POINT('Ctrl Pts',(11.2141543672614,-22.1198809963637,-2.04021647547921));
#88219=CARTESIAN_POINT('Ctrl Pts',(11.215098859081,-22.1035583375612,-2.03876892570883));
#88220=CARTESIAN_POINT('Ctrl Pts',(11.2156624545062,-22.0938183105583,-2.03790514646659));
#88221=CARTESIAN_POINT('Ctrl Pts',(11.2159437036462,-22.0840267162861,-2.0374723697639));
#88222=CARTESIAN_POINT('Ctrl Pts',(11.2159436836,-22.0742356136,-2.03747236903));
#88223=CARTESIAN_POINT('Origin',(11.275394600458,-22.0742358814361,-1.74517805615967));
#88224=CARTESIAN_POINT('Origin',(11.2744572343,-19.6742356128,-1.7432341771));
#88225=CARTESIAN_POINT('Origin',(11.2744572343,-19.6742356128,-1.7432341771));
#88226=CARTESIAN_POINT('Origin',(11.2744572343,-21.2742356128,-1.7432341771));
#88227=CARTESIAN_POINT('',(11.2159436339,-20.8742356128,-2.03747244546));
#88228=CARTESIAN_POINT('Origin',(10.3267865236,-21.2742356128,-3.3434289261));
#88229=CARTESIAN_POINT('',(10.5566756949,-20.8742356128,-3.15068305993));
#88230=CARTESIAN_POINT('Origin',(10.3267865236,-19.6742356128,-3.3434289261));
#88231=CARTESIAN_POINT('Origin',(3.05,-19.6742356128,15.662287998));
#88232=CARTESIAN_POINT('',(2.75,-19.6742356128,15.662287998));
#88233=CARTESIAN_POINT('Origin',(3.05,-19.6742356128,15.662287998));
#88234=CARTESIAN_POINT('Origin',(3.05,-19.6742356128,15.662287998));
#88235=CARTESIAN_POINT('',(2.97246042119851,-19.3848539651149,15.6779684221767));
#88236=CARTESIAN_POINT('Origin',(3.05,-19.6742356128,15.662287998));
#88237=CARTESIAN_POINT('Origin',(3.05,-19.6742356128,2.96634320571));
#88238=CARTESIAN_POINT('',(3.05,-19.3742356128,10.7304528845));
#88239=CARTESIAN_POINT('',(3.05,-19.3742356128,13.1963704412));
#88240=CARTESIAN_POINT('Origin',(3.05,-19.6742356128,10.7304528845));
#88241=CARTESIAN_POINT('',(2.75,-19.6742356128,13.1963704412));
#88242=CARTESIAN_POINT('Origin',(3.05,-22.4223864096,15.662287998));
#88243=CARTESIAN_POINT('',(2.75,-20.6742356128027,15.662287996875));
#88244=CARTESIAN_POINT('',(2.75,-20.1742356128,15.662287998));
#88245=CARTESIAN_POINT('',(3.10946375819699,-20.6742355012686,15.9563357201073));
#88246=CARTESIAN_POINT('Origin',(3.05000000000001,-20.6742355569137,15.662287998));
#88247=CARTESIAN_POINT('',(3.109463736,-21.2742356128,15.9563357222));
#88248=CARTESIAN_POINT('Origin',(2.75,-19.3742356128,10.4304528845));
#88249=CARTESIAN_POINT('',(2.75,-20.6742356128,13.3490218086));
#88250=CARTESIAN_POINT('Ctrl Pts',(3.1094637805,-20.6742355012,15.9563357204));
#88251=CARTESIAN_POINT('Ctrl Pts',(3.00535146138,-20.6742355416,15.9773898081));
#88252=CARTESIAN_POINT('Ctrl Pts',(2.89192096986,-20.6742355819,15.9523656045));
#88253=CARTESIAN_POINT('Ctrl Pts',(2.7970110589,-20.6742356114,15.8747276156));
#88254=CARTESIAN_POINT('Ctrl Pts',(2.75000002192,-20.6742356209,15.7685078059));
#88255=CARTESIAN_POINT('Ctrl Pts',(2.75000002182,-20.6742356129,15.6622879962));
#88256=CARTESIAN_POINT('Ctrl Pts',(3.10946380353,-20.7613039297,15.9563357159));
#88257=CARTESIAN_POINT('Ctrl Pts',(3.00535147528,-20.7455779654,15.9773898056));
#88258=CARTESIAN_POINT('Ctrl Pts',(2.89192097435,-20.7298520012,15.9523656029));
#88259=CARTESIAN_POINT('Ctrl Pts',(2.79701105681,-20.7183575883,15.8747276131));
#88260=CARTESIAN_POINT('Ctrl Pts',(2.75000001886,-20.7146527462,15.7685078017));
#88261=CARTESIAN_POINT('Ctrl Pts',(2.75000002231,-20.7177698279,15.6622879905));
#88262=CARTESIAN_POINT('Ctrl Pts',(3.09336559174,-20.8484128662,15.9595900965));
#88263=CARTESIAN_POINT('Ctrl Pts',(2.99245619263,-20.8169453132,15.9798833716));
#88264=CARTESIAN_POINT('Ctrl Pts',(2.88234381849,-20.7854777603,15.9544199132));
#88265=CARTESIAN_POINT('Ctrl Pts',(2.78979771265,-20.7624813454,15.8769278231));
#88266=CARTESIAN_POINT('Ctrl Pts',(2.74323291398,-20.755077053,15.7712039881));
#88267=CARTESIAN_POINT('Ctrl Pts',(2.74210499444,-20.7613240613,15.6654801511));
#88268=CARTESIAN_POINT('Ctrl Pts',(3.0611129676,-20.9309303248,15.9661188953));
#88269=CARTESIAN_POINT('Ctrl Pts',(2.96663575098,-20.8849847431,15.9848817048));
#88270=CARTESIAN_POINT('Ctrl Pts',(2.86318716199,-20.8390391614,15.9585340485));
#88271=CARTESIAN_POINT('Ctrl Pts',(2.77538294467,-20.80528071,15.8813354034));
#88272=CARTESIAN_POINT('Ctrl Pts',(2.72969914456,-20.7940068531,15.7766097304));
#88273=CARTESIAN_POINT('Ctrl Pts',(2.72628672053,-20.8025832991,15.6718840609));
#88274=CARTESIAN_POINT('Ctrl Pts',(2.95857415151,-21.0968055424,15.9864129862));
#88275=CARTESIAN_POINT('Ctrl Pts',(2.883615269,-21.0232686806,16.0006863819));
#88276=CARTESIAN_POINT('Ctrl Pts',(2.80037813885,-20.9497318188,15.9717891925));
#88277=CARTESIAN_POINT('Ctrl Pts',(2.72731697454,-20.8948262684,15.8954574233));
#88278=CARTESIAN_POINT('Ctrl Pts',(2.68525006547,-20.8745215131,15.7936237677));
#88279=CARTESIAN_POINT('Ctrl Pts',(2.67599823713,-20.8855201685,15.6917901077));
#88280=CARTESIAN_POINT('Ctrl Pts',(2.802073414,-21.210145586,16.0157241263));
#88281=CARTESIAN_POINT('Ctrl Pts',(2.75443180074,-21.1206683319,16.0242286253));
#88282=CARTESIAN_POINT('Ctrl Pts',(2.69943877243,-21.0311910779,15.9921593039));
#88283=CARTESIAN_POINT('Ctrl Pts',(2.64793358485,-20.9628100879,15.9169517332));
#88284=CARTESIAN_POINT('Ctrl Pts',(2.61350648776,-20.9339674316,15.8187461919));
#88285=CARTESIAN_POINT('Ctrl Pts',(2.59924369788,-20.942191106,15.7205406559));
#88286=CARTESIAN_POINT('Ctrl Pts',(2.70443397686,-21.2527626391,16.0332525536));
#88287=CARTESIAN_POINT('Ctrl Pts',(2.67281955818,-21.1584143796,16.038616685));
#88288=CARTESIAN_POINT('Ctrl Pts',(2.63437509944,-21.0640661201,16.0048673446));
#88289=CARTESIAN_POINT('Ctrl Pts',(2.59591773658,-20.9910117695,15.9302754357));
#88290=CARTESIAN_POINT('Ctrl Pts',(2.56711899741,-20.9580670061,15.8340046748));
#88291=CARTESIAN_POINT('Ctrl Pts',(2.55135784288,-20.9634991119,15.7377339138));
#88292=CARTESIAN_POINT('Ctrl Pts',(2.60121936463,-21.2742356128,16.0507826341));
#88293=CARTESIAN_POINT('Ctrl Pts',(2.58568379068,-21.1783721495,16.0532881684));
#88294=CARTESIAN_POINT('Ctrl Pts',(2.56380921231,-21.0825086862,16.0180414277));
#88295=CARTESIAN_POINT('Ctrl Pts',(2.53876678585,-21.0074397583,15.9440093758));
#88296=CARTESIAN_POINT('Ctrl Pts',(2.51662240651,-20.9716977028,15.8494690665));
#88297=CARTESIAN_POINT('Ctrl Pts',(2.50073751227,-20.9742356128,15.7549287572));
#88298=CARTESIAN_POINT('Ctrl Pts',(2.49776595187,-21.2742356128,16.0674673138));
#88299=CARTESIAN_POINT('Ctrl Pts',(2.49776595187,-21.1799878332,16.0674673138));
#88300=CARTESIAN_POINT('Ctrl Pts',(2.49187306376,-21.0857400536,16.0309284411));
#88301=CARTESIAN_POINT('Ctrl Pts',(2.4800122327,-21.0112466293,15.9573853181));
#88302=CARTESIAN_POINT('Ctrl Pts',(2.46500611635,-20.9742356128,15.864339843));
#88303=CARTESIAN_POINT('Ctrl Pts',(2.45,-20.9742356128,15.7712943679));
#88304=CARTESIAN_POINT('',(2.45,-20.9742356128,15.7712943679));
#88305=CARTESIAN_POINT('Ctrl Pts',(2.75,-20.6742356128,15.6622879962));
#88306=CARTESIAN_POINT('Ctrl Pts',(2.75000002231,-20.7177698279,15.6622879905));
#88307=CARTESIAN_POINT('Ctrl Pts',(2.74210499444,-20.7613240613,15.6654801511));
#88308=CARTESIAN_POINT('Ctrl Pts',(2.72628672053,-20.8025832991,15.6718840609));
#88309=CARTESIAN_POINT('Ctrl Pts',(2.67599823713,-20.8855201685,15.6917901077));
#88310=CARTESIAN_POINT('Ctrl Pts',(2.59924369788,-20.942191106,15.7205406559));
#88311=CARTESIAN_POINT('Ctrl Pts',(2.55135784288,-20.9634991119,15.7377339138));
#88312=CARTESIAN_POINT('Ctrl Pts',(2.50073751227,-20.9742356128,15.7549287572));
#88313=CARTESIAN_POINT('Ctrl Pts',(2.45,-20.9742356128,15.7712943679));
#88314=CARTESIAN_POINT('',(2.49776595187,-21.2742356128,16.0674673138));
#88315=CARTESIAN_POINT('Origin',(2.45033775172211,-21.2721143211372,15.7733885986677));
#88316=CARTESIAN_POINT('Ctrl Pts',(3.10946378033133,-20.6742355013784,15.9563357204341));
#88317=CARTESIAN_POINT('Ctrl Pts',(3.10932768110122,-20.7015979331535,15.9563632431162));
#88318=CARTESIAN_POINT('Ctrl Pts',(3.10730450936222,-20.7288604793434,15.956772561971));
#88319=CARTESIAN_POINT('Ctrl Pts',(3.10345054269395,-20.7557624287955,15.9575502978747));
#88320=CARTESIAN_POINT('Ctrl Pts',(3.09926382748793,-20.7849870720104,15.958395182902));
#88321=CARTESIAN_POINT('Ctrl Pts',(3.09291696055621,-20.8137858925351,15.9596747192825));
#88322=CARTESIAN_POINT('Ctrl Pts',(3.08453096290127,-20.8418628784539,15.9613564337185));
#88323=CARTESIAN_POINT('Ctrl Pts',(3.07580203981782,-20.8710880059325,15.9631069178664));
#88324=CARTESIAN_POINT('Ctrl Pts',(3.06486464518896,-20.8995309366648,15.9652928813008));
#88325=CARTESIAN_POINT('Ctrl Pts',(3.05189543077425,-20.9269002090981,15.9678650667302));
#88326=CARTESIAN_POINT('Ctrl Pts',(3.03848325063018,-20.9552042836972,15.9705251055915));
#88327=CARTESIAN_POINT('Ctrl Pts',(3.02289902586137,-20.9823598229141,15.9735978967696));
#88328=CARTESIAN_POINT('Ctrl Pts',(3.00536632094155,-21.0080918248321,15.9770201456985));
#88329=CARTESIAN_POINT('Ctrl Pts',(2.99098985450783,-21.0291915503758,15.9798263211904));
#88330=CARTESIAN_POINT('Ctrl Pts',(2.97530407509012,-21.0493349218278,15.982867211148));
#88331=CARTESIAN_POINT('Ctrl Pts',(2.95843887653005,-21.0683954688054,15.9861059378342));
#88332=CARTESIAN_POINT('Ctrl Pts',(2.947268491013,-21.081019907062,15.988251054925));
#88333=CARTESIAN_POINT('Ctrl Pts',(2.93558083779082,-21.0931699793608,15.9904829195074));
#88334=CARTESIAN_POINT('Ctrl Pts',(2.92341504117381,-21.1048131353117,15.9927905019296));
#88335=CARTESIAN_POINT('Ctrl Pts',(2.90102154963683,-21.1262446060538,15.9970380517671));
#88336=CARTESIAN_POINT('Ctrl Pts',(2.87712998286052,-21.1457721989991,16.00151876457));
#88337=CARTESIAN_POINT('Ctrl Pts',(2.85200450801134,-21.1633257927321,16.0061638407846));
#88338=CARTESIAN_POINT('Ctrl Pts',(2.82373910759164,-21.1830730555658,16.0113894112455));
#88339=CARTESIAN_POINT('Ctrl Pts',(2.7939115527548,-21.2003241299158,16.0168230390457));
#88340=CARTESIAN_POINT('Ctrl Pts',(2.76283377953572,-21.2149836940284,16.0223832732222));
#88341=CARTESIAN_POINT('Ctrl Pts',(2.75087357606706,-21.2206253906942,16.0245231154694));
#88342=CARTESIAN_POINT('Ctrl Pts',(2.73872764677138,-21.2258831354447,16.0266818619891));
#88343=CARTESIAN_POINT('Ctrl Pts',(2.72641206839653,-21.2307506374264,16.0288553736645));
#88344=CARTESIAN_POINT('Ctrl Pts',(2.70470559779606,-21.2393297138976,16.032686234534));
#88345=CARTESIAN_POINT('Ctrl Pts',(2.68268567272168,-21.2466165494237,16.0365252973163));
#88346=CARTESIAN_POINT('Ctrl Pts',(2.66036444590225,-21.2526520015251,16.0403664154533));
#88347=CARTESIAN_POINT('Ctrl Pts',(2.63807259783438,-21.2586795098854,16.0442024779876));
#88348=CARTESIAN_POINT('Ctrl Pts',(2.61547922403521,-21.263459231883,16.0480407832021));
#88349=CARTESIAN_POINT('Ctrl Pts',(2.59257948477896,-21.2669830827316,16.0518780878269));
#88350=CARTESIAN_POINT('Ctrl Pts',(2.57021450818643,-21.2704246433914,16.0556257823816));
#88351=CARTESIAN_POINT('Ctrl Pts',(2.54755637811659,-21.2726683931181,16.0593726685482));
#88352=CARTESIAN_POINT('Ctrl Pts',(2.52459873201666,-21.2736576793356,16.0631159841377));
#88353=CARTESIAN_POINT('Ctrl Pts',(2.51569942332494,-21.2740411665362,16.0645670440946));
#88354=CARTESIAN_POINT('Ctrl Pts',(2.50675516073449,-21.2742356128,16.066017559107));
#88355=CARTESIAN_POINT('Ctrl Pts',(2.49776595187,-21.2742356128,16.0674673138));
#88356=CARTESIAN_POINT('Origin',(2.45,-20.6742356128,13.3490218086));
#88357=CARTESIAN_POINT('',(2.73249401778459,-20.7752152053705,10.7304528485382));
#88358=CARTESIAN_POINT('Origin',(2.45,-20.6742356128,10.7304528845));
#88359=CARTESIAN_POINT('',(2.73284184833111,-20.7742356128,10.7560440517756));
#88360=CARTESIAN_POINT('Origin',(2.6183724284568,-21.0942392385765,10.8006651610913));
#88361=CARTESIAN_POINT('',(2.7328425359048,-20.7742356128,14.7056612864094));
#88362=CARTESIAN_POINT('',(2.73284210357,-20.7742356128,12.7308526862));
#88363=CARTESIAN_POINT('',(2.45000000025794,-20.9742356128,15.0444077730863));
#88364=CARTESIAN_POINT('Ctrl Pts',(2.45000000065989,-20.9742356128,15.0444077754594));
#88365=CARTESIAN_POINT('Ctrl Pts',(2.45060618541105,-20.9742356127987,15.044305098672));
#88366=CARTESIAN_POINT('Ctrl Pts',(2.45121325755483,-20.9742337755027,15.0442015735626));
#88367=CARTESIAN_POINT('Ctrl Pts',(2.45286377483275,-20.9742237555269,15.0439181984608));
#88368=CARTESIAN_POINT('Ctrl Pts',(2.45390823845169,-20.9742119797694,15.0437368106927));
#88369=CARTESIAN_POINT('Ctrl Pts',(2.45715653062603,-20.9741583263579,15.0431662137099));
#88370=CARTESIAN_POINT('Ctrl Pts',(2.45936133985891,-20.9740976540959,15.0427696908689));
#88371=CARTESIAN_POINT('Ctrl Pts',(2.47380236930478,-20.97354037289,15.0401113790515));
#88372=CARTESIAN_POINT('Ctrl Pts',(2.4859522398806,-20.9723204874474,15.037590560837));
#88373=CARTESIAN_POINT('Ctrl Pts',(2.49792722488249,-20.9703825039116,15.0347954601431));
#88374=CARTESIAN_POINT('Ctrl Pts',(2.51978994719543,-20.9668443286334,15.0296924466282));
#88375=CARTESIAN_POINT('Ctrl Pts',(2.54102226288492,-20.9609132340753,15.0237041443004));
#88376=CARTESIAN_POINT('Ctrl Pts',(2.58663934051023,-20.9427190138178,15.0074386652922));
#88377=CARTESIAN_POINT('Ctrl Pts',(2.60989476914103,-20.9293629068578,14.9966041376225));
#88378=CARTESIAN_POINT('Ctrl Pts',(2.65288015563397,-20.8970213813152,14.9679758450514));
#88379=CARTESIAN_POINT('Ctrl Pts',(2.67115973053595,-20.8782900142092,14.9501370800874));
#88380=CARTESIAN_POINT('Ctrl Pts',(2.70119454675138,-20.8401597687455,14.9048926284374));
#88381=CARTESIAN_POINT('Ctrl Pts',(2.71168115894417,-20.8218448720293,14.8780286003523));
#88382=CARTESIAN_POINT('Ctrl Pts',(2.7267534339897,-20.791371833055,14.814608554777));
#88383=CARTESIAN_POINT('Ctrl Pts',(2.73059155074725,-20.7804840144795,14.7785359194907));
#88384=CARTESIAN_POINT('Ctrl Pts',(2.73261231507094,-20.7748951009433,14.7291853931118));
#88385=CARTESIAN_POINT('Ctrl Pts',(2.73284271201381,-20.7742356141034,14.7173522523963));
#88386=CARTESIAN_POINT('Ctrl Pts',(2.73284271247462,-20.7742356128,14.7056612864095));
#88387=CARTESIAN_POINT('',(2.45,-20.9742356128,15.4078510693));
#88388=CARTESIAN_POINT('Origin',(6.51383560964,-21.0742356128,10.9320666897));
#88389=CARTESIAN_POINT('',(4.98919124473,-20.7742356128,9.52235136777));
#88390=CARTESIAN_POINT('Origin',(4.98919124473,-21.0742356128,9.52235136777));
#88391=CARTESIAN_POINT('',(8.14487887576,-20.7742356128,12.4401604693));
#88392=CARTESIAN_POINT('Origin',(8.14487887576,-21.0742356128,12.4401604693));
#88393=CARTESIAN_POINT('',(6.56703506025,-20.7742356128,10.9812559186));
#88394=CARTESIAN_POINT('Origin',(4.98919124473,-21.0742356128,9.52235136777));
#88395=CARTESIAN_POINT('Origin',(4.98919124473,-21.0742356128,9.52235136777));
#88396=CARTESIAN_POINT('Origin',(0.00234331738803,-21.0742356128,3.08191746407));
#88397=CARTESIAN_POINT('',(1.01362103240136,-20.9742355987892,10.879187255885));
#88398=CARTESIAN_POINT('Origin',(1.05,-21.0742356128,11.1596805575));
#88399=CARTESIAN_POINT('Origin',(0.00234331738835,-20.7742356128,3.08191746407));
#88400=CARTESIAN_POINT('',(2.45,-20.9304376384,10.5743743079));
#88401=CARTESIAN_POINT('Ctrl Pts',(2.73249449536286,-20.7752151161147,10.7304528285094));
#88402=CARTESIAN_POINT('Ctrl Pts',(2.73245710700268,-20.7753197109045,10.7290952012981));
#88403=CARTESIAN_POINT('Ctrl Pts',(2.73240712664869,-20.7754319433538,10.727752397751));
#88404=CARTESIAN_POINT('Ctrl Pts',(2.73152298709635,-20.7771409318656,10.7087546905869));
#88405=CARTESIAN_POINT('Ctrl Pts',(2.72772545244807,-20.7809744979902,10.6881339522637));
#88406=CARTESIAN_POINT('Ctrl Pts',(2.71679996433014,-20.790736326335,10.6559122059645));
#88407=CARTESIAN_POINT('Ctrl Pts',(2.70771619875055,-20.7984214920223,10.6384138803735));
#88408=CARTESIAN_POINT('Ctrl Pts',(2.68765731828286,-20.8146185581327,10.6112737349406));
#88409=CARTESIAN_POINT('Ctrl Pts',(2.67249689114105,-20.8263682945712,10.5972506978324));
#88410=CARTESIAN_POINT('Ctrl Pts',(2.6394257692643,-20.8502432000307,10.5761069546454));
#88411=CARTESIAN_POINT('Ctrl Pts',(2.61427989630388,-20.866832947014,10.5673521750875));
#88412=CARTESIAN_POINT('Ctrl Pts',(2.57563645957671,-20.8884881384831,10.5611700175102));
#88413=CARTESIAN_POINT('Ctrl Pts',(2.55565602930822,-20.8983536598197,10.5602963146483));
#88414=CARTESIAN_POINT('Ctrl Pts',(2.51151087548647,-20.9166072793448,10.562148593287));
#88415=CARTESIAN_POINT('Ctrl Pts',(2.48028974593005,-20.925972433295,10.5670447011082));
#88416=CARTESIAN_POINT('Ctrl Pts',(2.45000000001651,-20.9304376384374,10.5743743079454));
#88417=CARTESIAN_POINT('',(1.82443157197449,-20.9742356128,10.7304528194434));
#88418=CARTESIAN_POINT('Ctrl Pts',(2.4500000000165,-20.9304376384374,10.5743743079454));
#88419=CARTESIAN_POINT('Ctrl Pts',(2.35301070638687,-20.9447354504351,10.5978440786011));
#88420=CARTESIAN_POINT('Ctrl Pts',(2.24920782247063,-20.9566073584057,10.6246065671936));
#88421=CARTESIAN_POINT('Ctrl Pts',(2.07922400989342,-20.9679537533597,10.6677900651879));
#88422=CARTESIAN_POINT('Ctrl Pts',(2.0255308573803,-20.9704953103501,10.6813308519351));
#88423=CARTESIAN_POINT('Ctrl Pts',(1.94060113457634,-20.9730149159474,10.7023545221609));
#88424=CARTESIAN_POINT('Ctrl Pts',(1.90970835320785,-20.9736270659681,10.7099231588312));
#88425=CARTESIAN_POINT('Ctrl Pts',(1.86062551950229,-20.9741422809688,10.7217960060706));
#88426=CARTESIAN_POINT('Ctrl Pts',(1.84256776105564,-20.9742356100387,10.7261321551956));
#88427=CARTESIAN_POINT('Ctrl Pts',(1.8244315417982,-20.9742356127999,10.7304526927731));
#88428=CARTESIAN_POINT('Origin',(0.00234331738803,-20.9742356128,3.08191746407));
#88429=CARTESIAN_POINT('Origin',(1.05,-21.0742356128,11.1596805575));
#88430=CARTESIAN_POINT('',(0.767157426230295,-20.9742355987887,11.1596805575));
#88431=CARTESIAN_POINT('Origin',(1.05,-20.9742356128,11.1596805575));
#88432=CARTESIAN_POINT('Origin',(1.05,-21.0742356128,11.1596805575));
#88433=CARTESIAN_POINT('Origin',(1.05,-21.0742356128,12.1167294155));
#88434=CARTESIAN_POINT('',(0.767157287525,-20.9742356128,14.92922515));
#88435=CARTESIAN_POINT('',(0.767157387839,-20.9742356128,13.0444528538));
#88436=CARTESIAN_POINT('Origin',(1.05,-21.0742356128,14.92922515));
#88437=CARTESIAN_POINT('Origin',(8.14487887576,-21.0742356128,12.4401604693));
#88438=CARTESIAN_POINT('Origin',(8.14487887576,-21.0742356128,12.4401604693));
#88439=CARTESIAN_POINT('Origin',(1.05,-21.0742356128,14.92922515));
#88440=CARTESIAN_POINT('',(1.07064182343228,-20.9742356126354,15.2113136364792));
#88441=CARTESIAN_POINT('Origin',(1.05,-20.9742356128,14.92922515));
#88442=CARTESIAN_POINT('Origin',(1.05,-21.0742356128,14.92922515));
#88443=CARTESIAN_POINT('Origin',(2.04268023839E-15,-21.0742356128,0.580061096523));
#88444=CARTESIAN_POINT('Origin',(1.14862552646E-15,-20.7742356128,0.580061096523));
#88445=CARTESIAN_POINT('Origin',(2.05492670639E-15,-20.9742356128,0.580061096523));
#88446=CARTESIAN_POINT('Origin',(2.93915231795E-16,-20.7742356128,0.729452270839));
#88447=CARTESIAN_POINT('Origin',(2.45,-20.6742356128,10.7304528845));
#88448=CARTESIAN_POINT('Origin',(2.45,-20.6742356128,10.7304528845));
#88449=CARTESIAN_POINT('Origin',(0.75,-23.1742356128,-8.70195642562));
#88450=CARTESIAN_POINT('',(0.74999999938425,-21.0742356128,-6.2343884565225));
#88451=CARTESIAN_POINT('',(0.75,-22.1242356128,-6.23438845923));
#88452=CARTESIAN_POINT('',(0.75,-21.0742356128,-4.99584562937));
#88453=CARTESIAN_POINT('',(0.75,-21.0742356128,-6.03615517446));
#88454=CARTESIAN_POINT('',(0.75,-22.1242356128,-4.99584562937));
#88455=CARTESIAN_POINT('Origin',(2.32682891838E-16,-21.2742356128,0.729452270839));
#88456=CARTESIAN_POINT('',(1.19254592572,-22.1242356128,5.7836191207));
#88457=CARTESIAN_POINT('',(0.992653804111,-22.1242356128,5.82664824081));
#88458=CARTESIAN_POINT('Origin',(1.05,-22.1242356128,6.12111625914));
#88459=CARTESIAN_POINT('',(0.75,-21.0742356128,6.12111625914));
#88460=CARTESIAN_POINT('Origin',(1.05,-21.0742356128,6.12111625914));
#88461=CARTESIAN_POINT('',(0.75,-21.9742356128,6.12111625914));
#88462=CARTESIAN_POINT('Origin',(0.75,-23.1742356128,-8.70195642562));
#88463=CARTESIAN_POINT('',(0.75,-21.0742356128,9.0358656718));
#88464=CARTESIAN_POINT('',(0.75,-21.0742356128,7.56406439184));
#88465=CARTESIAN_POINT('',(0.75,-22.1242356128,9.0358656718));
#88466=CARTESIAN_POINT('Origin',(1.05,-22.1242356128,9.0358656718));
#88467=CARTESIAN_POINT('',(1.10198928897,-21.0742356128,9.33132652171));
#88468=CARTESIAN_POINT('Origin',(1.05,-21.0742356128,9.0358656718));
#88469=CARTESIAN_POINT('',(1.10198928897,-21.2742356128,9.33132652171));
#88470=CARTESIAN_POINT('Origin',(0.00234331738835,-21.2742356128,3.08191746407));
#88471=CARTESIAN_POINT('Origin',(0.00234331738835,-21.0742356128,3.08191746407));
#88472=CARTESIAN_POINT('',(3.58772315463,-22.1242356128,8.31731489457));
#88473=CARTESIAN_POINT('Origin',(1.2614400074,-22.1242356128,6.07560132137));
#88474=CARTESIAN_POINT('',(1.46510738459,-21.9742356128,5.8553296721));
#88475=CARTESIAN_POINT('Origin',(3.41821282746,-22.1242356128,8.06979469543));
#88476=CARTESIAN_POINT('',(3.62188020465,-21.9742356128,7.84952304616));
#88477=CARTESIAN_POINT('Origin',(3.88971125292,-23.1742356128,8.09716475273));
#88478=CARTESIAN_POINT('Origin',(0.00234331738835,-21.2742356128,3.08191746407));
#88479=CARTESIAN_POINT('',(6.21380646358,-22.1242356128,1.78497474518));
#88480=CARTESIAN_POINT('',(5.76218263052,-22.1242356128,0.419477620705));
#88481=CARTESIAN_POINT('Origin',(5.48986775992,-22.1242356128,0.545353000555));
#88482=CARTESIAN_POINT('',(5.1900363009,-21.9742356128,0.55540766038));
#88483=CARTESIAN_POINT('Origin',(2.32682891838E-16,-21.2742356128,0.729452270839));
#88484=CARTESIAN_POINT('',(5.08448267152,-22.1242356128,1.78529520144));
#88485=CARTESIAN_POINT('Origin',(5.92013962829,-22.1242356128,1.84629187045));
#88486=CARTESIAN_POINT('',(5.92013962829,-21.9742356128,2.14629187045));
#88487=CARTESIAN_POINT('Origin',(5.3782162351,-22.1242356128,1.84629187045));
#88488=CARTESIAN_POINT('',(5.3782162351,-21.9742356128,2.14629187045));
#88489=CARTESIAN_POINT('Origin',(-11.4443506127,-23.1742356128,2.14629187045));
#88490=CARTESIAN_POINT('Origin',(2.32682891838E-16,-21.2742356128,0.729452270839));
#88491=CARTESIAN_POINT('',(4.2092958712,-22.1242356128,3.77060280966));
#88492=CARTESIAN_POINT('',(3.13117783752,-22.1242356128,4.87221628548));
#88493=CARTESIAN_POINT('Origin',(3.31206782846,-22.1242356128,5.11154620667));
#88494=CARTESIAN_POINT('',(3.10840045127,-21.9742356128,5.33181785593));
#88495=CARTESIAN_POINT('Origin',(9.80058174751,-23.1742356128,11.519536597));
#88496=CARTESIAN_POINT('',(4.71627105755,-22.1242356128,6.81848575139));
#88497=CARTESIAN_POINT('Origin',(4.91993843473,-22.1242356128,6.59821410213));
#88498=CARTESIAN_POINT('',(5.16397092918,-21.0742356128,6.77270806092));
#88499=CARTESIAN_POINT('Origin',(4.91993843473,-21.0742356128,6.59821410213));
#88500=CARTESIAN_POINT('',(5.16397092918,-21.2742356128,6.77270806092));
#88501=CARTESIAN_POINT('Origin',(0.00234331738835,-21.2742356128,3.08191746407));
#88502=CARTESIAN_POINT('',(6.28256615006,-21.0742356128,3.98918589435));
#88503=CARTESIAN_POINT('Origin',(0.00234331738835,-21.0742356128,3.08191746407));
#88504=CARTESIAN_POINT('',(6.28256615006,-22.1242356128,3.98918589435));
#88505=CARTESIAN_POINT('Origin',(4.452469377,-22.1242356128,3.94629187045));
#88506=CARTESIAN_POINT('',(4.452469377,-21.0742356128,3.64629187045));
#88507=CARTESIAN_POINT('',(4.452469377,-21.9742356128,3.64629187045));
#88508=CARTESIAN_POINT('Origin',(4.452469377,-21.0742356128,3.94629187045));
#88509=CARTESIAN_POINT('Origin',(5.98564848014,-22.1242356128,3.94629187045));
#88510=CARTESIAN_POINT('',(5.98564848014,-21.0742356128,3.64629187045));
#88511=CARTESIAN_POINT('Origin',(5.98564848014,-21.0742356128,3.94629187045));
#88512=CARTESIAN_POINT('',(5.98564848014,-21.9742356128,3.64629187045));
#88513=CARTESIAN_POINT('Origin',(-11.7190551593,-23.1742356128,3.64629187045));
#88514=CARTESIAN_POINT('',(-4.57919858809,-21.0742356128,3.64629187045));
#88515=CARTESIAN_POINT('Origin',(4.91993843473,-21.0742356128,6.59821410213));
#88516=CARTESIAN_POINT('Origin',(4.91993843473,-21.0742356128,6.59821410213));
#88517=CARTESIAN_POINT('Origin',(0.00234331738835,-21.0742356128,3.08191746407));
#88518=CARTESIAN_POINT('',(5.98564848014,-20.7742356128,3.94629187045));
#88519=CARTESIAN_POINT('Origin',(0.00234331738835,-20.7742356128,3.08191746407));
#88520=CARTESIAN_POINT('Ctrl Pts',(5.98564848014,-20.7742356128,3.94629187045));
#88521=CARTESIAN_POINT('Ctrl Pts',(6.00325376366273,-20.7742356128,3.94883520662962));
#88522=CARTESIAN_POINT('Ctrl Pts',(6.02086151892848,-20.7758219937196,3.95137159218802));
#88523=CARTESIAN_POINT('Ctrl Pts',(6.03819046933219,-20.7789698139932,3.95387127852019));
#88524=CARTESIAN_POINT('Ctrl Pts',(6.05551616145726,-20.7821170423974,3.95637049484844));
#88525=CARTESIAN_POINT('Ctrl Pts',(6.07256227259131,-20.7868248395128,3.95883357428083));
#88526=CARTESIAN_POINT('Ctrl Pts',(6.0890604606157,-20.7930184980419,3.96122159453396));
#88527=CARTESIAN_POINT('Ctrl Pts',(6.10203541218976,-20.7978894826229,3.96309964605673));
#88528=CARTESIAN_POINT('Ctrl Pts',(6.11467162344997,-20.8036783444377,3.96493111746659));
#88529=CARTESIAN_POINT('Ctrl Pts',(6.12684913512964,-20.8103298005963,3.96669033401031));
#88530=CARTESIAN_POINT('Ctrl Pts',(6.14176502552207,-20.8184769815329,3.96884514870751));
#88531=CARTESIAN_POINT('Ctrl Pts',(6.15599039473335,-20.8279195594011,3.97089881512368));
#88532=CARTESIAN_POINT('Ctrl Pts',(6.16931229547304,-20.8385161827716,3.97282398767375));
#88533=CARTESIAN_POINT('Ctrl Pts',(6.17525926176098,-20.8432465709633,3.9736833947867));
#88534=CARTESIAN_POINT('Ctrl Pts',(6.18102680506576,-20.8482065514678,3.97451707692433));
#88535=CARTESIAN_POINT('Ctrl Pts',(6.18659908662289,-20.8533824917211,3.97532207306466));
#88536=CARTESIAN_POINT('Ctrl Pts',(6.19562650893926,-20.8617678179239,3.97662621393537));
#88537=CARTESIAN_POINT('Ctrl Pts',(6.2041391134579,-20.87071888487,3.97785598197763));
#88538=CARTESIAN_POINT('Ctrl Pts',(6.21207169969898,-20.880167130521,3.97900195804526));
#88539=CARTESIAN_POINT('Ctrl Pts',(6.21603799281952,-20.8848912533465,3.97957494607907));
#88540=CARTESIAN_POINT('Ctrl Pts',(6.21985942235242,-20.8897395549112,3.98012700648607));
#88541=CARTESIAN_POINT('Ctrl Pts',(6.22352864890558,-20.8947027251433,3.98065707898559));
#88542=CARTESIAN_POINT('Ctrl Pts',(6.22536326218216,-20.8971843102593,3.98092211523535));
#88543=CARTESIAN_POINT('Ctrl Pts',(6.22715983319936,-20.8996946046435,3.98118165573411));
#88544=CARTESIAN_POINT('Ctrl Pts',(6.22891750090729,-20.9022324050138,3.98143557609082));
#88545=CARTESIAN_POINT('Ctrl Pts',(6.22992901378548,-20.9036928731929,3.98158170366073));
#88546=CARTESIAN_POINT('Ctrl Pts',(6.23113763302248,-20.905473872797,3.98176162924324));
#88547=CARTESIAN_POINT('Ctrl Pts',(6.23217750243642,-20.9070389005777,3.98191069395136));
#88548=CARTESIAN_POINT('Ctrl Pts',(6.2329445748111,-20.9081933624361,3.98202065335406));
#88549=CARTESIAN_POINT('Ctrl Pts',(6.23362112590207,-20.909229675745,3.98211508230871));
#88550=CARTESIAN_POINT('Ctrl Pts',(6.23407297039883,-20.9099270947014,3.98218035773892));
#88551=CARTESIAN_POINT('Ctrl Pts',(6.24140060621849,-20.9212372515438,3.98323894002544));
#88552=CARTESIAN_POINT('Ctrl Pts',(6.24797445346109,-20.9330497413319,3.98416457610613));
#88553=CARTESIAN_POINT('Ctrl Pts',(6.25373323382676,-20.9452535591513,3.9849466848626));
#88554=CARTESIAN_POINT('Ctrl Pts',(6.2546664150874,-20.9472311261662,3.98507342163479));
#88555=CARTESIAN_POINT('Ctrl Pts',(6.25557826501334,-20.9492190377732,3.98519644133876));
#88556=CARTESIAN_POINT('Ctrl Pts',(6.25646859717888,-20.9512169122126,3.98531575432681));
#88557=CARTESIAN_POINT('Ctrl Pts',(6.25966093983393,-20.9583804181927,3.98574355864053));
#88558=CARTESIAN_POINT('Ctrl Pts',(6.26257588740962,-20.965670468392,3.98612291044023));
#88559=CARTESIAN_POINT('Ctrl Pts',(6.26520446752445,-20.9730645987735,3.98645249592255));
#88560=CARTESIAN_POINT('Ctrl Pts',(6.26632784754956,-20.9762246387991,3.98659335133924));
#88561=CARTESIAN_POINT('Ctrl Pts',(6.26746961610877,-20.9796167701875,3.98674544026523));
#88562=CARTESIAN_POINT('Ctrl Pts',(6.26853189014378,-20.9829670042927,3.98687533316301));
#88563=CARTESIAN_POINT('Ctrl Pts',(6.26964178137131,-20.9864674150351,3.98701104860272));
#88564=CARTESIAN_POINT('Ctrl Pts',(6.2706648700053,-20.9899217568917,3.98712247524996));
#88565=CARTESIAN_POINT('Ctrl Pts',(6.27152961786085,-20.9930121729073,3.98721531003455));
#88566=CARTESIAN_POINT('Ctrl Pts',(6.27177382310526,-20.9938849079983,3.98724152662603));
#88567=CARTESIAN_POINT('Ctrl Pts',(6.27200562645505,-20.9947286067318,3.98726650908391));
#88568=CARTESIAN_POINT('Ctrl Pts',(6.27222388875607,-20.9955360948653,3.98729090767503));
#88569=CARTESIAN_POINT('Ctrl Pts',(6.2754008551609,-21.0072896714587,3.98764604689953));
#88570=CARTESIAN_POINT('Ctrl Pts',(6.27785776815197,-21.0192458614175,3.98798398659007));
#88571=CARTESIAN_POINT('Ctrl Pts',(6.27957628318323,-21.0313012257436,3.98828097625466));
#88572=CARTESIAN_POINT('Ctrl Pts',(6.28145475340164,-21.0444786739747,3.98860560899279));
#88573=CARTESIAN_POINT('Ctrl Pts',(6.28245216396942,-21.0577747139993,3.98888156993282));
#88574=CARTESIAN_POINT('Ctrl Pts',(6.28255779916532,-21.0710863072773,3.98912804850833));
#88575=CARTESIAN_POINT('Ctrl Pts',(6.28256612893013,-21.0721359805447,3.98914748434642));
#88576=CARTESIAN_POINT('Ctrl Pts',(6.28256891438073,-21.0731857638459,3.98916675941873));
#88577=CARTESIAN_POINT('Ctrl Pts',(6.28256615006486,-21.0742356128,3.9891858943507));
#88578=CARTESIAN_POINT('Origin',(4.452469377,-21.0742356128,3.94629187045));
#88579=CARTESIAN_POINT('Origin',(4.452469377,-21.0742356128,3.94629187045));
#88580=CARTESIAN_POINT('Origin',(5.98564848014,-21.0742356128,3.94629187045));
#88581=CARTESIAN_POINT('Origin',(5.98564848014,-21.0742356128,3.94629187045));
#88582=CARTESIAN_POINT('Origin',(-4.57919858809,-21.0742356128,3.94629187045));
#88583=CARTESIAN_POINT('',(5.21905892857,-20.7742356128,3.94629187045));
#88584=CARTESIAN_POINT('Origin',(2.93915231795E-16,-20.7742356128,0.729452270839));
#88585=CARTESIAN_POINT('',(1.05,-20.7742356128,9.0358656718));
#88586=CARTESIAN_POINT('',(1.05,-20.7742356128,7.56406439184));
#88587=CARTESIAN_POINT('Origin',(0.00234331738835,-20.7742356128,3.08191746407));
#88588=CARTESIAN_POINT('Origin',(10.3267865236,-19.6742356128,-3.3434289261));
#88589=CARTESIAN_POINT('Origin',(1.05,-21.0742356128,-4.99584562937));
#88590=CARTESIAN_POINT('',(1.01141425905,-21.0742356128,-4.69833741));
#88591=CARTESIAN_POINT('Origin',(1.05,-21.0742356128,-4.99584562937));
#88592=CARTESIAN_POINT('',(1.05,-20.7742356128,-4.99584562937));
#88593=CARTESIAN_POINT('Origin',(1.05,-21.0742356128,-4.99584562937));
#88594=CARTESIAN_POINT('Origin',(1.05,-21.0742356128,-4.99584562937));
#88595=CARTESIAN_POINT('Origin',(2.93915231795E-16,-20.7742356128,0.729452270839));
#88596=CARTESIAN_POINT('Origin',(2.93915231795E-16,-20.7742356128,0.729452270839));
#88597=CARTESIAN_POINT('Origin',(1.05,-22.1242356128,-4.99584562937));
#88598=CARTESIAN_POINT('',(1.01141425905,-21.2742356128,-4.69833741));
#88599=CARTESIAN_POINT('Origin',(11.0821857629,-20.8742356128,-2.71007990903));
#88600=CARTESIAN_POINT('Origin',(11.0821857629,-22.0742356128,-2.71007990903));
#88601=CARTESIAN_POINT('Origin',(1.05,-21.0742356128,6.12111625914));
#88602=CARTESIAN_POINT('Origin',(1.05,-21.0742356128,6.12111625914));
#88603=CARTESIAN_POINT('Origin',(0.00234331738835,-21.0742356128,3.08191746407));
#88604=CARTESIAN_POINT('Ctrl Pts',(1.05,-20.7742356128,9.0358656718));
#88605=CARTESIAN_POINT('Ctrl Pts',(1.05194346679646,-20.7742356127999,9.04691060744439));
#88606=CARTESIAN_POINT('Ctrl Pts',(1.05373571268161,-20.7748621802049,9.05721123155974));
#88607=CARTESIAN_POINT('Ctrl Pts',(1.05539004573013,-20.7758744125586,9.0667127620523));
#88608=CARTESIAN_POINT('Ctrl Pts',(1.05664195232833,-20.7766404133126,9.07390298818438));
#88609=CARTESIAN_POINT('Ctrl Pts',(1.05781511495567,-20.7776277333487,9.08063685240658));
#88610=CARTESIAN_POINT('Ctrl Pts',(1.05891817857726,-20.7787438986221,9.08690601609574));
#88611=CARTESIAN_POINT('Ctrl Pts',(1.06019853257273,-20.780039460038,9.09418279380878));
#88612=CARTESIAN_POINT('Ctrl Pts',(1.06137963728991,-20.7815082048312,9.10083598740895));
#88613=CARTESIAN_POINT('Ctrl Pts',(1.0624569555597,-20.783027573221,9.1068776662104));
#88614=CARTESIAN_POINT('Ctrl Pts',(1.06292348574346,-20.7836855321863,9.10949400123461));
#88615=CARTESIAN_POINT('Ctrl Pts',(1.0633037229392,-20.7842538831696,9.1116194090953));
#88616=CARTESIAN_POINT('Ctrl Pts',(1.06368406010907,-20.7848444845195,9.11374713142444));
#88617=CARTESIAN_POINT('Ctrl Pts',(1.0640510629429,-20.7854143798288,9.11580025740389));
#88618=CARTESIAN_POINT('Ctrl Pts',(1.06441817676359,-20.7860052807807,9.1178556394656));
#88619=CARTESIAN_POINT('Ctrl Pts',(1.06486103473096,-20.7867597488703,9.12034512089835));
#88620=CARTESIAN_POINT('Ctrl Pts',(1.06501903860616,-20.7870289297153,9.12123332375928));
#88621=CARTESIAN_POINT('Ctrl Pts',(1.06518666287036,-20.7873193387291,9.12217666319411));
#88622=CARTESIAN_POINT('Ctrl Pts',(1.06536725084921,-20.7876390838914,9.12319423081729));
#88623=CARTESIAN_POINT('Ctrl Pts',(1.06687631132471,-20.7903109936706,9.13169740523177));
#88624=CARTESIAN_POINT('Ctrl Pts',(1.06834277231229,-20.7933703249366,9.14006063447592));
#88625=CARTESIAN_POINT('Ctrl Pts',(1.06975205420403,-20.7967336412273,9.14812658276299));
#88626=CARTESIAN_POINT('Ctrl Pts',(1.07118502872607,-20.800153501074,9.15632813453146));
#88627=CARTESIAN_POINT('Ctrl Pts',(1.07255878230226,-20.8038871259129,9.16422173025703));
#88628=CARTESIAN_POINT('Ctrl Pts',(1.07386305000202,-20.8078000652983,9.17166940850749));
#88629=CARTESIAN_POINT('Ctrl Pts',(1.075232223093,-20.8119077276394,9.17948771195293));
#88630=CARTESIAN_POINT('Ctrl Pts',(1.07652474432684,-20.8162122271943,9.18681414579865));
#88631=CARTESIAN_POINT('Ctrl Pts',(1.07773580012668,-20.8205166591577,9.19352802619739));
#88632=CARTESIAN_POINT('Ctrl Pts',(1.07787931959557,-20.8210267676014,9.19432367289601));
#88633=CARTESIAN_POINT('Ctrl Pts',(1.07802170331068,-20.8215368384517,9.19511076325773));
#88634=CARTESIAN_POINT('Ctrl Pts',(1.0781629498924,-20.8220465170099,9.19588913334329));
#88635=CARTESIAN_POINT('Ctrl Pts',(1.08032804869949,-20.8298591268785,9.20782038239202));
#88636=CARTESIAN_POINT('Ctrl Pts',(1.08226652975325,-20.8382896507038,9.21881468989689));
#88637=CARTESIAN_POINT('Ctrl Pts',(1.08402351013971,-20.8471020783112,9.22887541721332));
#88638=CARTESIAN_POINT('Ctrl Pts',(1.08517584511253,-20.852881806193,9.23547385623297));
#88639=CARTESIAN_POINT('Ctrl Pts',(1.08625031498372,-20.8588263848537,9.24167173694038));
#88640=CARTESIAN_POINT('Ctrl Pts',(1.08726153943815,-20.86487656414,9.24747939313306));
#88641=CARTESIAN_POINT('Ctrl Pts',(1.08808125864387,-20.8697809630964,9.25218719791422));
#88642=CARTESIAN_POINT('Ctrl Pts',(1.08883536059498,-20.8746095350316,9.25650566075248));
#88643=CARTESIAN_POINT('Ctrl Pts',(1.08954994669871,-20.879465449889,9.26058857987151));
#88644=CARTESIAN_POINT('Ctrl Pts',(1.0903054586788,-20.8845994733886,9.26490533651148));
#88645=CARTESIAN_POINT('Ctrl Pts',(1.0910168938194,-20.8897644415258,9.26895933782676));
#88646=CARTESIAN_POINT('Ctrl Pts',(1.09170742387484,-20.8951252431836,9.27288880630623));
#88647=CARTESIAN_POINT('Ctrl Pts',(1.09236126852373,-20.9002012445105,9.27660951609725));
#88648=CARTESIAN_POINT('Ctrl Pts',(1.09299638824525,-20.9054534538637,9.28021867678994));
#88649=CARTESIAN_POINT('Ctrl Pts',(1.09362516937514,-20.9110509216446,9.2837922762023));
#88650=CARTESIAN_POINT('Ctrl Pts',(1.09366044853728,-20.9113649800093,9.28399278093614));
#88651=CARTESIAN_POINT('Ctrl Pts',(1.09369570566157,-20.9116801319542,9.28419316189014));
#88652=CARTESIAN_POINT('Ctrl Pts',(1.0937309421707,-20.9119964096905,9.28439342814165));
#88653=CARTESIAN_POINT('Ctrl Pts',(1.09455787442067,-20.9194188322443,9.28909328706713));
#88654=CARTESIAN_POINT('Ctrl Pts',(1.09539733055772,-20.9264344691809,9.29306015364301));
#88655=CARTESIAN_POINT('Ctrl Pts',(1.09616241712905,-20.9329817607834,9.29647355247341));
#88656=CARTESIAN_POINT('Ctrl Pts',(1.09697381650712,-20.9399253780594,9.30009357377806));
#88657=CARTESIAN_POINT('Ctrl Pts',(1.0977016092117,-20.9463428927236,9.30309156448054));
#88658=CARTESIAN_POINT('Ctrl Pts',(1.09823552189471,-20.9522094034754,9.30564980905609));
#88659=CARTESIAN_POINT('Ctrl Pts',(1.09838767546572,-20.9538812322006,9.30637885344867));
#88660=CARTESIAN_POINT('Ctrl Pts',(1.09852404269639,-20.9555085643539,9.30707197485802));
#88661=CARTESIAN_POINT('Ctrl Pts',(1.09864197616628,-20.9570913748885,9.30773289237069));
#88662=CARTESIAN_POINT('Ctrl Pts',(1.09901475411098,-20.9620945080828,9.30982199796739));
#88663=CARTESIAN_POINT('Ctrl Pts',(1.0992510098558,-20.9669907190302,9.3117310437097));
#88664=CARTESIAN_POINT('Ctrl Pts',(1.09944107532713,-20.9719977802765,9.31354051571788));
#88665=CARTESIAN_POINT('Ctrl Pts',(1.09962572085938,-20.9768620593187,9.3152983885167));
#88666=CARTESIAN_POINT('Ctrl Pts',(1.09976679713354,-20.981831375378,9.31696238538762));
#88667=CARTESIAN_POINT('Ctrl Pts',(1.09993952702919,-20.9871206659853,9.31856173716953));
#88668=CARTESIAN_POINT('Ctrl Pts',(1.10002874388929,-20.9898526418156,9.31938781967031));
#88669=CARTESIAN_POINT('Ctrl Pts',(1.10012627944569,-20.9926701971939,9.32019592075339));
#88670=CARTESIAN_POINT('Ctrl Pts',(1.10024158038163,-20.9956041247815,9.32098473025938));
#88671=CARTESIAN_POINT('Ctrl Pts',(1.1005109347092,-21.002458068213,9.32282746685415));
#88672=CARTESIAN_POINT('Ctrl Pts',(1.10074051696748,-21.0089603913746,9.32431951715542));
#88673=CARTESIAN_POINT('Ctrl Pts',(1.10094115953662,-21.015244260674,9.32556382456884));
#88674=CARTESIAN_POINT('Ctrl Pts',(1.10115318185268,-21.0218845291291,9.32687870476));
#88675=CARTESIAN_POINT('Ctrl Pts',(1.10133288275599,-21.0282814763706,9.32791692087774));
#88676=CARTESIAN_POINT('Ctrl Pts',(1.10148363819399,-21.0346111901984,9.32874677840441));
#88677=CARTESIAN_POINT('Ctrl Pts',(1.10163793722913,-21.041089687753,9.32959614223087));
#88678=CARTESIAN_POINT('Ctrl Pts',(1.10176192015105,-21.0474983506607,9.33022727982751));
#88679=CARTESIAN_POINT('Ctrl Pts',(1.10184974337085,-21.0540357911593,9.33065978940719));
#88680=CARTESIAN_POINT('Ctrl Pts',(1.10193756659064,-21.060573231658,9.33109229898687));
#88681=CARTESIAN_POINT('Ctrl Pts',(1.10198928897115,-21.0672400649741,9.33132652171654));
#88682=CARTESIAN_POINT('Ctrl Pts',(1.10198928897115,-21.0742356128,9.33132652171654));
#88683=CARTESIAN_POINT('Origin',(0.45,-22.1242356128,-6.23438845923));
#88684=CARTESIAN_POINT('Origin',(0.451735403140307,-21.0742356268872,-6.23570473075995));
#88685=CARTESIAN_POINT('Ctrl Pts',(0.530469794195843,-21.0743245297157,
-6.52339509610176));
#88686=CARTESIAN_POINT('Ctrl Pts',(0.605567644237528,-21.0743045727586,
-6.50248549027524));
#88687=CARTESIAN_POINT('Ctrl Pts',(0.673874294281432,-21.0742929409078,
-6.45718387642163));
#88688=CARTESIAN_POINT('Ctrl Pts',(0.724680377815537,-21.0742929154351,
-6.3902979847186));
#88689=CARTESIAN_POINT('Ctrl Pts',(0.750000527627887,-21.0743044999368,
-6.31234350391071));
#88690=CARTESIAN_POINT('Ctrl Pts',(0.750000364792457,-21.0743244203334,
-6.23438902308944));
#88691=CARTESIAN_POINT('Ctrl Pts',(0.529382289785393,-20.9333453475782,
-6.52305698967578));
#88692=CARTESIAN_POINT('Ctrl Pts',(0.604379979183787,-20.964969743794,-6.50191658027744));
#88693=CARTESIAN_POINT('Ctrl Pts',(0.672544464007601,-20.9834025266085,
-6.45625456200327));
#88694=CARTESIAN_POINT('Ctrl Pts',(0.723444072664958,-20.9834428927103,
-6.38924960266457));
#88695=CARTESIAN_POINT('Ctrl Pts',(0.749147469416239,-20.9650851420997,
-6.3113527732948));
#88696=CARTESIAN_POINT('Ctrl Pts',(0.749396133634582,-20.9335186780883,
-6.23345594923032));
#88697=CARTESIAN_POINT('Ctrl Pts',(0.682790624388214,-20.8340546276202,
-6.57041298136646));
#88698=CARTESIAN_POINT('Ctrl Pts',(0.708912783176195,-20.8612993243623,
-6.52470345794668));
#88699=CARTESIAN_POINT('Ctrl Pts',(0.735010274608166,-20.8749839393705,
-6.48004084831971));
#88700=CARTESIAN_POINT('Ctrl Pts',(0.764785838670641,-20.8750139028965,
-6.43996377974995));
#88701=CARTESIAN_POINT('Ctrl Pts',(0.79985759450253,-20.8613891112934,-6.4024626941325));
#88702=CARTESIAN_POINT('Ctrl Pts',(0.83594438370652,-20.8342039270154,-6.36496160653959));
#88703=CARTESIAN_POINT('Ctrl Pts',(0.784751637977717,-20.8055921195135,
-6.60126308111576));
#88704=CARTESIAN_POINT('Ctrl Pts',(0.81115374258346,-20.8073594222485,-6.57634919799807));
#88705=CARTESIAN_POINT('Ctrl Pts',(0.836973064211128,-20.8079610962015,
-6.54907865572581));
#88706=CARTESIAN_POINT('Ctrl Pts',(0.859860043401567,-20.8079624129721,
-6.51825025363853));
#88707=CARTESIAN_POINT('Ctrl Pts',(0.87856407045771,-20.8073639920301,-6.48547428652468));
#88708=CARTESIAN_POINT('Ctrl Pts',(0.894834790258138,-20.8056018007968,
-6.45269832121122));
#88709=CARTESIAN_POINT('Ctrl Pts',(0.922269592128314,-20.7721965716525,
-6.64281131501362));
#88710=CARTESIAN_POINT('Ctrl Pts',(0.931687523370322,-20.7721714559979,
-6.62728238450244));
#88711=CARTESIAN_POINT('Ctrl Pts',(0.941236644076639,-20.7721534139295,
-6.61231329467342));
#88712=CARTESIAN_POINT('Ctrl Pts',(0.951507076621634,-20.77215320473,-6.59822048475924));
#88713=CARTESIAN_POINT('Ctrl Pts',(0.962806769208053,-20.7721710748754,
-6.58460782258426));
#88714=CARTESIAN_POINT('Ctrl Pts',(0.9746824612806,-20.7721964339549,-6.57098901863393));
#88715=CARTESIAN_POINT('Ctrl Pts',(1.05,-20.7742356128,-6.68100624476));
#88716=CARTESIAN_POINT('Ctrl Pts',(1.05,-20.7742356128,-6.68100624476));
#88717=CARTESIAN_POINT('Ctrl Pts',(1.05,-20.7742356128,-6.68100624476));
#88718=CARTESIAN_POINT('Ctrl Pts',(1.05,-20.7742356128,-6.68100624476));
#88719=CARTESIAN_POINT('Ctrl Pts',(1.05,-20.7742356128,-6.68100624476));
#88720=CARTESIAN_POINT('Ctrl Pts',(1.05,-20.7742356128,-6.68100624476));
#88721=CARTESIAN_POINT('Ctrl Pts',(1.05,-20.7742356128,-6.68100624476));
#88722=CARTESIAN_POINT('Ctrl Pts',(1.04185133965169,-20.7740151821963,-6.66912323008901));
#88723=CARTESIAN_POINT('Ctrl Pts',(1.03364154604321,-20.7742886139255,-6.65712795842614));
#88724=CARTESIAN_POINT('Ctrl Pts',(1.0254283835494,-20.7749660951999,-6.64510629905131));
#88725=CARTESIAN_POINT('Ctrl Pts',(1.01686694079147,-20.7756723051592,-6.63257485958806));
#88726=CARTESIAN_POINT('Ctrl Pts',(1.00830156833828,-20.7768176645118,-6.62001433313557));
#88727=CARTESIAN_POINT('Ctrl Pts',(0.999773202279283,-20.7783415832968,
-6.60748637620009));
#88728=CARTESIAN_POINT('Ctrl Pts',(0.990516308375853,-20.7799956814457,
-6.59388823003983));
#88729=CARTESIAN_POINT('Ctrl Pts',(0.981302730655643,-20.7820956741035,
-6.58032799535186));
#88730=CARTESIAN_POINT('Ctrl Pts',(0.972160688749562,-20.7846119703408,
-6.56685002089311));
#88731=CARTESIAN_POINT('Ctrl Pts',(0.966662483256319,-20.7861253208523,
-6.55874409948429));
#88732=CARTESIAN_POINT('Ctrl Pts',(0.961189710615404,-20.7877901735135,
-6.55066730455419));
#88733=CARTESIAN_POINT('Ctrl Pts',(0.955745648342861,-20.7896074561403,
-6.54262532894721));
#88734=CARTESIAN_POINT('Ctrl Pts',(0.945091671144306,-20.7931638606596,
-6.52688726048678));
#88735=CARTESIAN_POINT('Ctrl Pts',(0.934548826309054,-20.7973004363901,
-6.51128114796628));
#88736=CARTESIAN_POINT('Ctrl Pts',(0.924133552938165,-20.8020720545725,
-6.49583202115931));
#88737=CARTESIAN_POINT('Ctrl Pts',(0.913983176009837,-20.806722313993,-6.48077581910679));
#88738=CARTESIAN_POINT('Ctrl Pts',(0.903952604551205,-20.8119771913179,
-6.46586663394951));
#88739=CARTESIAN_POINT('Ctrl Pts',(0.894062671861464,-20.8179299419942,
-6.45113668546664));
#88740=CARTESIAN_POINT('Ctrl Pts',(0.884728957361107,-20.8235479049317,
-6.43723516175994));
#88741=CARTESIAN_POINT('Ctrl Pts',(0.875519620967452,-20.8297886520844,
-6.42349192647127));
#88742=CARTESIAN_POINT('Ctrl Pts',(0.866472894903575,-20.8367498259702,
-6.40996619617227));
#88743=CARTESIAN_POINT('Ctrl Pts',(0.858512683717075,-20.8428749605046,
-6.39806491068275));
#88744=CARTESIAN_POINT('Ctrl Pts',(0.850678234212531,-20.8495585348559,
-6.38633181316587));
#88745=CARTESIAN_POINT('Ctrl Pts',(0.843017929021964,-20.8568702967361,
-6.37484167223405));
#88746=CARTESIAN_POINT('Ctrl Pts',(0.835728552685902,-20.8638280069967,
-6.36390790924122));
#88747=CARTESIAN_POINT('Ctrl Pts',(0.828596625165056,-20.871354920686,-6.35319378039933));
#88748=CARTESIAN_POINT('Ctrl Pts',(0.821688263209047,-20.8795073540466,
-6.34280129650637));
#88749=CARTESIAN_POINT('Ctrl Pts',(0.815188118199059,-20.887178057951,-6.33302290725166));
#88750=CARTESIAN_POINT('Ctrl Pts',(0.808885816695372,-20.8954027709262,
-6.32352915177084));
#88751=CARTESIAN_POINT('Ctrl Pts',(0.802860701131854,-20.9042208042776,
-6.31444228904566));
#88752=CARTESIAN_POINT('Ctrl Pts',(0.797952094672979,-20.9114047752748,
-6.30703930522012));
#88753=CARTESIAN_POINT('Ctrl Pts',(0.793227830308663,-20.9189824725644,
-6.29990695086639));
#88754=CARTESIAN_POINT('Ctrl Pts',(0.788744524978859,-20.9269695397081,
-6.2931323825073));
#88755=CARTESIAN_POINT('Ctrl Pts',(0.783537340438766,-20.9362462071424,
-6.28526398519098));
#88756=CARTESIAN_POINT('Ctrl Pts',(0.778654465486172,-20.9460755460276,
-6.27787710052425));
#88757=CARTESIAN_POINT('Ctrl Pts',(0.774208582045746,-20.9564706602872,
-6.27114504890079));
#88758=CARTESIAN_POINT('Ctrl Pts',(0.769935816653026,-20.9664609996781,
-6.26467513632118));
#88759=CARTESIAN_POINT('Ctrl Pts',(0.766066640928027,-20.9769740075416,
-6.25881000506791));
#88760=CARTESIAN_POINT('Ctrl Pts',(0.762726389024589,-20.9880079998434,
-6.25374228386215));
#88761=CARTESIAN_POINT('Ctrl Pts',(0.75945227095981,-20.9988235294999,-6.24877489875866));
#88762=CARTESIAN_POINT('Ctrl Pts',(0.756686247671062,-21.0101397324872,
-6.2445735214744));
#88763=CARTESIAN_POINT('Ctrl Pts',(0.754572184142313,-21.0219403794457,
-6.24135910637881));
#88764=CARTESIAN_POINT('Ctrl Pts',(0.752512978193132,-21.0334348128394,
-6.23822810175291));
#88765=CARTESIAN_POINT('Ctrl Pts',(0.751072291099966,-21.0453889517463,
-6.23603343627861));
#88766=CARTESIAN_POINT('Ctrl Pts',(0.75040877541252,-21.0577724001193,-6.2350186214298));
#88767=CARTESIAN_POINT('Ctrl Pts',(0.750119049159553,-21.0631796725678,
-6.23457549927133));
#88768=CARTESIAN_POINT('Ctrl Pts',(0.749977843125384,-21.0686685916167,
-6.234357854582));
#88769=CARTESIAN_POINT('Ctrl Pts',(0.749999997537,-21.0742356128,-6.23438845562));
#88770=CARTESIAN_POINT('Origin',(1.05,-21.0742356128,7.56406439184));
#88771=CARTESIAN_POINT('Ctrl Pts',(1.05,-20.7742356128,9.0358656718));
#88772=CARTESIAN_POINT('Ctrl Pts',(1.03202389557851,-20.7742356128,9.0358656718));
#88773=CARTESIAN_POINT('Ctrl Pts',(1.01404810351911,-20.7758556512248,9.03586567179998));
#88774=CARTESIAN_POINT('Ctrl Pts',(0.996361658047574,-20.7790696793446,
9.03586567179994));
#88775=CARTESIAN_POINT('Ctrl Pts',(0.978670794646673,-20.7822845103023,
9.0358656717999));
#88776=CARTESIAN_POINT('Ctrl Pts',(0.961270037985875,-20.7870940177168,
9.03586567179984));
#88777=CARTESIAN_POINT('Ctrl Pts',(0.94443931537033,-20.7934208306739,9.03586567179976));
#88778=CARTESIAN_POINT('Ctrl Pts',(0.931321632902273,-20.7983518799997,
9.03586567179969));
#88779=CARTESIAN_POINT('Ctrl Pts',(0.918550114703901,-20.8042035471181,
9.03586567179962));
#88780=CARTESIAN_POINT('Ctrl Pts',(0.906249801614279,-20.810918540691,9.03586567179953));
#88781=CARTESIAN_POINT('Ctrl Pts',(0.890471751000551,-20.8195321026135,
9.03586567179942));
#88782=CARTESIAN_POINT('Ctrl Pts',(0.875470244037574,-20.829567460778,9.03586567179929));
#88783=CARTESIAN_POINT('Ctrl Pts',(0.861486491178611,-20.8408632558426,
9.03586567179914));
#88784=CARTESIAN_POINT('Ctrl Pts',(0.856033990875819,-20.8452676762175,
9.03586567179908));
#88785=CARTESIAN_POINT('Ctrl Pts',(0.850735912921936,-20.8498632609397,
9.03586567179902));
#88786=CARTESIAN_POINT('Ctrl Pts',(0.845605262111768,-20.8546387295717,
9.03586567179895));
#88787=CARTESIAN_POINT('Ctrl Pts',(0.836460775867545,-20.8631501658067,
9.03586567179884));
#88788=CARTESIAN_POINT('Ctrl Pts',(0.827848666191205,-20.872233507004,9.03586567179871));
#88789=CARTESIAN_POINT('Ctrl Pts',(0.819835992199914,-20.8818180213137,
9.03586567179857));
#88790=CARTESIAN_POINT('Ctrl Pts',(0.815829655204269,-20.8866102784685,
9.03586567179851));
#88791=CARTESIAN_POINT('Ctrl Pts',(0.811973029026346,-20.8915277101616,
9.03586567179843));
#88792=CARTESIAN_POINT('Ctrl Pts',(0.808273644182413,-20.89656071614,9.03586567179836));
#88793=CARTESIAN_POINT('Ctrl Pts',(0.806423951760447,-20.8990772191291,
9.03586567179832));
#88794=CARTESIAN_POINT('Ctrl Pts',(0.804613560752439,-20.901622607585,9.03586567179828));
#88795=CARTESIAN_POINT('Ctrl Pts',(0.802843353271149,-20.9041956410941,
9.03586567179824));
#88796=CARTESIAN_POINT('Ctrl Pts',(0.801780698696832,-20.90574023169,9.03586567179822));
#88797=CARTESIAN_POINT('Ctrl Pts',(0.800495085070646,-20.90764888492,9.0358656717982));
#88798=CARTESIAN_POINT('Ctrl Pts',(0.799417570014984,-20.9092857847225,
9.03586567179817));
#88799=CARTESIAN_POINT('Ctrl Pts',(0.798700122475243,-20.9103756903622,
9.03586567179815));
#88800=CARTESIAN_POINT('Ctrl Pts',(0.798073491215928,-20.9113441289506,
9.03586567179814));
#88801=CARTESIAN_POINT('Ctrl Pts',(0.797654124306547,-20.9119964097062,
9.03586567179813));
#88802=CARTESIAN_POINT('Ctrl Pts',(0.78926050248039,-20.9250517983519,9.03586567179794));
#88803=CARTESIAN_POINT('Ctrl Pts',(0.78188214283678,-20.9387597450956,9.03589999168628));
#88804=CARTESIAN_POINT('Ctrl Pts',(0.775607596296699,-20.9529557348733,
9.03596863146315));
#88805=CARTESIAN_POINT('Ctrl Pts',(0.772470323026658,-20.9600537297621,
9.03600295135159));
#88806=CARTESIAN_POINT('Ctrl Pts',(0.76960860666254,-20.9672735141048,9.03604585121217));
#88807=CARTESIAN_POINT('Ctrl Pts',(0.767031056629434,-20.9745933673027,
9.03609733104487));
#88808=CARTESIAN_POINT('Ctrl Pts',(0.765851262758171,-20.9779438038919,
9.03612089434737));
#88809=CARTESIAN_POINT('Ctrl Pts',(0.764648990061719,-20.98156092275,9.03614854597792));
#88810=CARTESIAN_POINT('Ctrl Pts',(0.763545455771623,-20.9851076481037,
9.03617714035478));
#88811=CARTESIAN_POINT('Ctrl Pts',(0.762387498750328,-20.9888292864458,
9.03620714491354));
#88812=CARTESIAN_POINT('Ctrl Pts',(0.761338259871668,-20.99247304056,9.03623818749787));
#88813=CARTESIAN_POINT('Ctrl Pts',(0.76048046437477,-20.9956325690208,9.03626663380754));
#88814=CARTESIAN_POINT('Ctrl Pts',(0.760369753607963,-20.9960403513185,
9.0362703052103));
#88815=CARTESIAN_POINT('Ctrl Pts',(0.760262162949232,-20.9964400516044,
9.03627393336538));
#88816=CARTESIAN_POINT('Ctrl Pts',(0.760157814465616,-20.9968307842384,
9.0362775104594));
#88817=CARTESIAN_POINT('Ctrl Pts',(0.755519525522536,-21.0141988455,9.03643651224889));
#88818=CARTESIAN_POINT('Ctrl Pts',(0.752446613553971,-21.0319846306718,
9.03642084523756));
#88819=CARTESIAN_POINT('Ctrl Pts',(0.750988491653542,-21.0499021404548,
9.03623050942544));
#88820=CARTESIAN_POINT('Ctrl Pts',(0.750329859351278,-21.05799546291,9.03614453491666));
#88821=CARTESIAN_POINT('Ctrl Pts',(0.749999999999998,-21.0661155349141,
9.03602292237484));
#88822=CARTESIAN_POINT('Ctrl Pts',(0.749999999999998,-21.0742356128,9.0358656718));
#88823=CARTESIAN_POINT('Origin',(1.05,-21.0742356128,-6.03615517446));
#88824=CARTESIAN_POINT('',(1.05,-20.7742356128,-5.83842593707));
#88825=CARTESIAN_POINT('Origin',(1.05,-21.0742356128,9.0358656718));
#88826=CARTESIAN_POINT('Origin',(11.0821857629,-22.0742356128,-2.71007990903));
#88827=CARTESIAN_POINT('Origin',(2.45,-19.6742356128,10.7304528845));
#88828=CARTESIAN_POINT('',(2.45,-19.3742356128,10.1304528845));
#88829=CARTESIAN_POINT('Origin',(2.45,-19.3742356128,10.7304528845));
#88830=CARTESIAN_POINT('Origin',(2.45,-19.6742356128,10.1304528845));
#88831=CARTESIAN_POINT('Origin',(4.57526812267,-21.0742356128,-3.65872047634));
#88832=CARTESIAN_POINT('',(4.79320888776,-21.0742356128,-3.4525607739));
#88833=CARTESIAN_POINT('',(4.40684492179,-21.0742356128,-3.41045927235));
#88834=CARTESIAN_POINT('Origin',(4.57526812267,-21.0742356128,-3.65872047634));
#88835=CARTESIAN_POINT('',(4.57526812267,-20.7742356128,-3.65872047634));
#88836=CARTESIAN_POINT('Origin',(4.57526812267,-21.0742356128,-3.65872047634));
#88837=CARTESIAN_POINT('Origin',(4.57526812267,-21.0742356128,-3.65872047634));
#88838=CARTESIAN_POINT('Origin',(4.57526812267,-22.1242356128,-3.65872047634));
#88839=CARTESIAN_POINT('',(4.40684492179,-21.2742356128,-3.41045927235));
#88840=CARTESIAN_POINT('',(4.79320888776,-21.9742356128,-3.4525607739));
#88841=CARTESIAN_POINT('Origin',(0.00234331738835,-21.2742356128,3.08191746407));
#88842=CARTESIAN_POINT('Origin',(0.00234331738835,-21.0742356128,3.08191746407));
#88843=CARTESIAN_POINT('Origin',(0.00234331738835,-21.0742356128,3.08191746407));
#88844=CARTESIAN_POINT('Origin',(0.00234331738835,-20.7742356128,3.08191746407));
#88845=CARTESIAN_POINT('Origin',(3.69394702409,-21.0742356128,-6.14889144395));
#88846=CARTESIAN_POINT('',(3.69394702409,-20.7742356128,-7.0794205347));
#88847=CARTESIAN_POINT('Origin',(3.69394702409,-21.0742356128,-7.0794205347));
#88848=CARTESIAN_POINT('',(3.69394702409,-20.7742356128,-7.27665075431));
#88849=CARTESIAN_POINT('Origin',(3.69394702409,-21.0742356128,-7.27665075431));
#88850=CARTESIAN_POINT('',(3.69394702409,-20.7742356128,-7.17803564451));
#88851=CARTESIAN_POINT('Origin',(3.09394702409,-21.0742356128,-7.0794205347));
#88852=CARTESIAN_POINT('',(2.83839294143,-20.7742356128,-6.53656501909));
#88853=CARTESIAN_POINT('Origin',(2.83839294143,-21.0742356128,-6.53656501909));
#88854=CARTESIAN_POINT('Origin',(3.09394702409,-20.7742356128,-7.0794205347));
#88855=CARTESIAN_POINT('Origin',(-2.84607155346,-21.0742356128,5.53854202767));
#88856=CARTESIAN_POINT('',(2.48410064475,-20.7742356128,-6.69708673107));
#88857=CARTESIAN_POINT('Origin',(2.48410064475,-21.0742356128,-6.69708673107));
#88858=CARTESIAN_POINT('Origin',(-2.84607155346,-20.7742356128,5.53854202767));
#88859=CARTESIAN_POINT('Origin',(2.72372695744,-21.0742356128,-7.24715875387));
#88860=CARTESIAN_POINT('',(2.12372695744,-20.7742356128,-7.24715875387));
#88861=CARTESIAN_POINT('Origin',(2.12372695744,-21.0742356128,-7.24715875387));
#88862=CARTESIAN_POINT('Origin',(2.72372695744,-20.7742356128,-7.24715875387));
#88863=CARTESIAN_POINT('Origin',(2.12372695744,-21.0742356128,-6.11170048962));
#88864=CARTESIAN_POINT('',(2.12372695744,-20.7742356128,-7.96338790087));
#88865=CARTESIAN_POINT('Origin',(2.12372695744,-21.0742356128,-7.96338790087));
#88866=CARTESIAN_POINT('',(2.12372695744,-20.7742356128,-7.60527332737));
#88867=CARTESIAN_POINT('Origin',(3.69394702409,-21.0742356128,-7.27665075431));
#88868=CARTESIAN_POINT('',(3.83031550589,-21.0742356128,-7.54386534443));
#88869=CARTESIAN_POINT('Origin',(3.69394702409,-21.0742356128,-7.27665075431));
#88870=CARTESIAN_POINT('Origin',(3.69394702409,-21.0742356128,-7.27665075431));
#88871=CARTESIAN_POINT('',(3.69394702409,-20.7869530199367,-7.36307246360657));
#88872=CARTESIAN_POINT('Origin',(3.69394702409,-21.0742356128,-7.27665075431));
#88873=CARTESIAN_POINT('Origin',(-2.84607155346,-21.0742356128,5.53854202767));
#88874=CARTESIAN_POINT('',(6.53717906469,-21.0742356128,-5.76093294477));
#88875=CARTESIAN_POINT('Origin',(-2.84607155346,-21.0742356128,5.53854202767));
#88876=CARTESIAN_POINT('',(6.34552156645,-20.7742356128,-5.5301356238));
#88877=CARTESIAN_POINT('Ctrl Pts',(6.34552156645,-20.7742356128,-5.5301356238));
#88878=CARTESIAN_POINT('Ctrl Pts',(6.35174034324132,-20.7742356127986,-5.53762438388832));
#88879=CARTESIAN_POINT('Ctrl Pts',(6.35742859914234,-20.7747062490391,-5.54448824766959));
#88880=CARTESIAN_POINT('Ctrl Pts',(6.36256699872495,-20.7754276309491,-5.55070852110689));
#88881=CARTESIAN_POINT('Ctrl Pts',(6.3678994278893,-20.7761762527474,-5.55716367644349));
#88882=CARTESIAN_POINT('Ctrl Pts',(6.37264035260703,-20.7771944005427,-5.56292651713689));
#88883=CARTESIAN_POINT('Ctrl Pts',(6.37678906820952,-20.7782819825865,-5.5680013143877));
#88884=CARTESIAN_POINT('Ctrl Pts',(6.37894431376028,-20.7788469782588,-5.57063765663039));
#88885=CARTESIAN_POINT('Ctrl Pts',(6.38094000743543,-20.7794315014735,-5.57308863873272));
#88886=CARTESIAN_POINT('Ctrl Pts',(6.38277728175031,-20.7800126526577,-5.57535633957807));
#88887=CARTESIAN_POINT('Ctrl Pts',(6.38638444340125,-20.7811536397426,-5.57980856723886));
#88888=CARTESIAN_POINT('Ctrl Pts',(6.38939025144264,-20.7822789779567,-5.5835505570955));
#88889=CARTESIAN_POINT('Ctrl Pts',(6.39182761328184,-20.7832571893903,-5.58659360401943));
#88890=CARTESIAN_POINT('Ctrl Pts',(6.39235720901811,-20.7834697374807,-5.58725480444124));
#88891=CARTESIAN_POINT('Ctrl Pts',(6.39285996977376,-20.7836755352566,-5.58788300900781));
#88892=CARTESIAN_POINT('Ctrl Pts',(6.39333622863194,-20.7838735566742,-5.5884783276713));
#88893=CARTESIAN_POINT('Ctrl Pts',(6.39467030265331,-20.7844282450004,-5.5901459064465));
#88894=CARTESIAN_POINT('Ctrl Pts',(6.39579652923337,-20.7849214295115,-5.59155550086856));
#88895=CARTESIAN_POINT('Ctrl Pts',(6.3967213044829,-20.7853351743983,-5.59270930512864));
#88896=CARTESIAN_POINT('Ctrl Pts',(6.39718369210766,-20.7855420468417,-5.59328620725868));
#88897=CARTESIAN_POINT('Ctrl Pts',(6.39732902439631,-20.785609782216,-5.59347304518995));
#88898=CARTESIAN_POINT('Ctrl Pts',(6.39755820869149,-20.7857142794367,-5.59375953787831));
#88899=CARTESIAN_POINT('Ctrl Pts',(6.39778739298666,-20.7858187766574,-5.59404603056667));
#88900=CARTESIAN_POINT('Ctrl Pts',(6.39810064993959,-20.7859589015239,-5.59443244375046));
#88901=CARTESIAN_POINT('Ctrl Pts',(6.39889593392354,-20.7863267818361,-5.59540494006124));
#88902=CARTESIAN_POINT('Ctrl Pts',(6.40404794656149,-20.7887099858944,-5.60170497047125));
#88903=CARTESIAN_POINT('Ctrl Pts',(6.40977643932818,-20.7916764543232,-5.60846234457286));
#88904=CARTESIAN_POINT('Ctrl Pts',(6.41591040714488,-20.7954242675397,-5.61563336197756));
#88905=CARTESIAN_POINT('Ctrl Pts',(6.41735133745903,-20.7963046663023,-5.61731790559932));
#88906=CARTESIAN_POINT('Ctrl Pts',(6.41881449983512,-20.7972282257994,-5.61902510707537));
#88907=CARTESIAN_POINT('Ctrl Pts',(6.42029740193474,-20.7981975666476,-5.6207540767046));
#88908=CARTESIAN_POINT('Ctrl Pts',(6.42419517278191,-20.8007454546706,-5.62529862986033));
#88909=CARTESIAN_POINT('Ctrl Pts',(6.42822810099414,-20.8036096225989,-5.6299947451574));
#88910=CARTESIAN_POINT('Ctrl Pts',(6.43233592097233,-20.8068348561763,-5.63482617722769));
#88911=CARTESIAN_POINT('Ctrl Pts',(6.43408287762893,-20.808206470146,-5.63688086863602));
#88912=CARTESIAN_POINT('Ctrl Pts',(6.4360229497544,-20.8097917703793,-5.63917812802395));
#88913=CARTESIAN_POINT('Ctrl Pts',(6.43791817945649,-20.8114135266398,-5.64143439912276));
#88914=CARTESIAN_POINT('Ctrl Pts',(6.43989708759085,-20.813106886897,-5.6437902894013));
#88915=CARTESIAN_POINT('Ctrl Pts',(6.44182686918908,-20.8148399819277,-5.64610120824757));
#88916=CARTESIAN_POINT('Ctrl Pts',(6.44345562697637,-20.8163576317262,-5.64806724246914));
#88917=CARTESIAN_POINT('Ctrl Pts',(6.4439349217766,-20.8168042307618,-5.64864578765667));
#88918=CARTESIAN_POINT('Ctrl Pts',(6.44438827496193,-20.8172318574099,-5.64919461873951));
#88919=CARTESIAN_POINT('Ctrl Pts',(6.4448095419601,-20.8176333489548,-5.64970642349391));
#88920=CARTESIAN_POINT('Ctrl Pts',(6.45271403902305,-20.8251667867785,-5.65930973729628));
#88921=CARTESIAN_POINT('Ctrl Pts',(6.46005563597925,-20.8333640871257,-5.66815201559128));
#88922=CARTESIAN_POINT('Ctrl Pts',(6.46680425788755,-20.8419892536935,-5.67625933714307));
#88923=CARTESIAN_POINT('Ctrl Pts',(6.47106538871199,-20.8474352489837,-5.68137836118048));
#88924=CARTESIAN_POINT('Ctrl Pts',(6.47509076231836,-20.8530523456082,-5.68620517151398));
#88925=CARTESIAN_POINT('Ctrl Pts',(6.47887829642981,-20.8587871989418,-5.69075306944489));
#88926=CARTESIAN_POINT('Ctrl Pts',(6.4837713419325,-20.8661959502525,-5.69662841495012));
#88927=CARTESIAN_POINT('Ctrl Pts',(6.48827128604217,-20.8738016698329,-5.70203664313868));
#88928=CARTESIAN_POINT('Ctrl Pts',(6.49240130722295,-20.8815114106274,-5.70700767832463));
#88929=CARTESIAN_POINT('Ctrl Pts',(6.4941955719898,-20.8848608647012,-5.70916731695564));
#88930=CARTESIAN_POINT('Ctrl Pts',(6.49601100333805,-20.8884066452834,-5.71135394124107));
#88931=CARTESIAN_POINT('Ctrl Pts',(6.49772743922749,-20.8919183912156,-5.71342174719814));
#88932=CARTESIAN_POINT('Ctrl Pts',(6.4995360642771,-20.8956187517709,-5.71560061427653));
#88933=CARTESIAN_POINT('Ctrl Pts',(6.50123465242143,-20.8992809205782,-5.71764741014477));
#88934=CARTESIAN_POINT('Ctrl Pts',(6.5027136656765,-20.9026002822876,-5.71942893398982));
#88935=CARTESIAN_POINT('Ctrl Pts',(6.5030618778577,-20.9033817777726,-5.71984836789402));
#88936=CARTESIAN_POINT('Ctrl Pts',(6.50339804632306,-20.9041441473342,-5.72025325107986));
#88937=CARTESIAN_POINT('Ctrl Pts',(6.50372095659477,-20.9048832171215,-5.72064210415656));
#88938=CARTESIAN_POINT('Ctrl Pts',(6.50817483638558,-20.9150771572898,-5.72600552864804));
#88939=CARTESIAN_POINT('Ctrl Pts',(6.51208297248286,-20.9253660622679,-5.73071176481533));
#88940=CARTESIAN_POINT('Ctrl Pts',(6.51551887458798,-20.9356960421862,-5.7348493327296));
#88941=CARTESIAN_POINT('Ctrl Pts',(6.51908984608229,-20.9464321058739,-5.73914955334871));
#88942=CARTESIAN_POINT('Ctrl Pts',(6.52215114646008,-20.9572133335537,-5.74283602360956));
#88943=CARTESIAN_POINT('Ctrl Pts',(6.5247662065358,-20.9680266144033,-5.74598512619714));
#88944=CARTESIAN_POINT('Ctrl Pts',(6.52749312419639,-20.9793024266844,-5.74926892970927));
#88945=CARTESIAN_POINT('Ctrl Pts',(6.52973519744188,-20.9906139949508,-5.75196887803585));
#88946=CARTESIAN_POINT('Ctrl Pts',(6.53153761692296,-21.0019836757955,-5.75413938848151));
#88947=CARTESIAN_POINT('Ctrl Pts',(6.53341564424095,-21.0138302916622,-5.75640094743252));
#88948=CARTESIAN_POINT('Ctrl Pts',(6.53481674186588,-21.0257411027344,-5.75808818025164));
#88949=CARTESIAN_POINT('Ctrl Pts',(6.53575756861761,-21.0377652510857,-5.75922114543387));
#88950=CARTESIAN_POINT('Ctrl Pts',(6.53669839536933,-21.049789399437,-5.76035411061609));
#88951=CARTESIAN_POINT('Ctrl Pts',(6.53717906472003,-21.0619281910693,-5.76093294480616));
#88952=CARTESIAN_POINT('Ctrl Pts',(6.53717906472003,-21.0742356128,-5.76093294480616));
#88953=CARTESIAN_POINT('Origin',(-2.84607155346,-20.7742356128,5.53854202767));
#88954=CARTESIAN_POINT('Origin',(2.12372695744,-21.0742356128,-7.96338790087));
#88955=CARTESIAN_POINT('Origin',(2.12372695744,-21.0742356128,-7.96338790086));
#88956=CARTESIAN_POINT('Origin',(-2.84607155346,-21.0742356128,5.53854202767));
#88957=CARTESIAN_POINT('',(0.207931718075,-21.0742356128,-8.82796731988));
#88958=CARTESIAN_POINT('Origin',(-2.84607155346,-21.0742356128,5.53854202767));
#88959=CARTESIAN_POINT('',(2.93466272541E-14,-20.7742356128,-8.56468050289));
#88960=CARTESIAN_POINT('Origin',(-2.84607155346,-20.7742356128,5.53854202767));
#88961=CARTESIAN_POINT('Ctrl Pts',(0.207931718075,-21.0742356128,-8.82796731988));
#88962=CARTESIAN_POINT('Ctrl Pts',(0.208944325295,-20.9488183216,-8.82888814763));
#88963=CARTESIAN_POINT('Ctrl Pts',(0.15281970676,-20.8273615349,-8.76362621195));
#88964=CARTESIAN_POINT('Ctrl Pts',(0.0739219411508,-20.7751437694,-8.66437291113));
#88965=CARTESIAN_POINT('Ctrl Pts',(2.93466272541E-14,-20.7742356128,-8.56468050289));
#88966=CARTESIAN_POINT('Origin',(3.69394702409,-23.1223803511,-7.27665075431));
#88967=CARTESIAN_POINT('',(3.83031550589,-22.5742356128,-7.54386534443));
#88968=CARTESIAN_POINT('Origin',(-2.84607155346,-21.2742356128,5.53854202767));
#88969=CARTESIAN_POINT('',(6.53717906469,-22.1242356128,-5.76093294477));
#88970=CARTESIAN_POINT('Origin',(-2.84607155346,-22.6642356128,5.53854202767));
#88971=CARTESIAN_POINT('',(0.207931718075,-23.2742356128,-8.82796731988));
#88972=CARTESIAN_POINT('Origin',(6.34552156645,-22.1242356128,-5.5301356238));
#88973=CARTESIAN_POINT('',(6.56346233154,-21.0742356128,-5.32397592135));
#88974=CARTESIAN_POINT('',(6.56346233154,-21.9742356128,-5.32397592135));
#88975=CARTESIAN_POINT('Origin',(6.34552156645,-21.0742356128,-5.5301356238));
#88976=CARTESIAN_POINT('Origin',(6.34552156645,-21.0742356128,-5.5301356238));
#88977=CARTESIAN_POINT('Origin',(6.34552156645,-21.0742356128,-5.5301356238));
#88978=CARTESIAN_POINT('Origin',(5.6152263525,-21.0742356128,-4.75810745444));
#88979=CARTESIAN_POINT('',(5.67833560965,-21.0742356128,-4.38826834763));
#88980=CARTESIAN_POINT('',(5.46039484456,-20.7742356128,-4.59442805007));
#88981=CARTESIAN_POINT('Origin',(6.78099426296,-23.1742356128,-5.55393878512));
#88982=CARTESIAN_POINT('',(6.4527882763,-22.8742356128,-5.20697736155));
#88983=CARTESIAN_POINT('Origin',(6.6707290414,-22.8742356128,-5.00081765911));
#88984=CARTESIAN_POINT('',(5.89627637474,-23.1742356128,-4.18210864518));
#88985=CARTESIAN_POINT('Ctrl Pts',(8.01224741424,-22.8742356128,11.9089404858));
#88986=CARTESIAN_POINT('Ctrl Pts',(8.01224741424,-22.8742356128,11.9089404858));
#88987=CARTESIAN_POINT('Ctrl Pts',(8.01224741424,-22.8742356128,11.9089404858));
#88988=CARTESIAN_POINT('Ctrl Pts',(8.01224741424,-22.8742356128,11.9089404858));
#88989=CARTESIAN_POINT('Ctrl Pts',(8.01224741424,-22.8742356128,11.9089404858));
#88990=CARTESIAN_POINT('Ctrl Pts',(8.01224741423999,-22.8742356128,11.9089404858));
#88991=CARTESIAN_POINT('Ctrl Pts',(7.9829584197,-22.9540055384,11.8818593216));
#88992=CARTESIAN_POINT('Ctrl Pts',(7.9770990599352,-22.9460253560251,11.8764416455582));
#88993=CARTESIAN_POINT('Ctrl Pts',(7.97123968718953,-22.9380451737504,11.8710239575141));
#88994=CARTESIAN_POINT('Ctrl Pts',(7.96538034046018,-22.9300650091037,11.8656062935251));
#88995=CARTESIAN_POINT('Ctrl Pts',(7.95952098070146,-22.9220848089627,11.860188617489));
#88996=CARTESIAN_POINT('Ctrl Pts',(7.95366162093663,-22.914104626726,11.8547709414472));
#88997=CARTESIAN_POINT('Ctrl Pts',(7.95813278234,-23.0338190575,11.8499462819));
#88998=CARTESIAN_POINT('Ctrl Pts',(7.94825905166378,-23.0178496871499,11.8371162897713));
#88999=CARTESIAN_POINT('Ctrl Pts',(7.93746144800327,-23.0018803166997,11.8252680214644));
#89000=CARTESIAN_POINT('Ctrl Pts',(7.92573318729569,-22.9859083057293,11.8144258374139));
#89001=CARTESIAN_POINT('Ctrl Pts',(7.91307644092752,-22.969936608137,11.8045917287975));
#89002=CARTESIAN_POINT('Ctrl Pts',(7.8995045515438,-22.9539767898742,11.7957473669925));
#89003=CARTESIAN_POINT('Ctrl Pts',(7.93828028322,-23.1128615217,11.8131880532));
#89004=CARTESIAN_POINT('Ctrl Pts',(7.92683935647196,-23.0883986064311,11.7920888374253));
#89005=CARTESIAN_POINT('Ctrl Pts',(7.91212856723288,-23.0639356911622,11.7732848241785));
#89006=CARTESIAN_POINT('Ctrl Pts',(7.89438791009002,-23.0397784455373,11.7568870252871));
#89007=CARTESIAN_POINT('Ctrl Pts',(7.87382726489228,-23.0162127276929,11.7430895590338));
#89008=CARTESIAN_POINT('Ctrl Pts',(7.85061574634478,-22.9934900789388,11.7321598018371));
#89009=CARTESIAN_POINT('Ctrl Pts',(7.91959338184,-23.2114810387,11.7607695014));
#89010=CARTESIAN_POINT('Ctrl Pts',(7.91104290590454,-23.1749426359854,11.7286346798805));
#89011=CARTESIAN_POINT('Ctrl Pts',(7.89351740441245,-23.1384042333708,11.699893196182));
#89012=CARTESIAN_POINT('Ctrl Pts',(7.86768957667201,-23.103241423932,11.6760256725457));
#89013=CARTESIAN_POINT('Ctrl Pts',(7.83459760655358,-23.0708679220605,11.6579915758093));
#89014=CARTESIAN_POINT('Ctrl Pts',(7.79567993551832,-23.0427829224516,11.6462613688059));
#89015=CARTESIAN_POINT('Ctrl Pts',(7.9155846643,-23.3039994083,11.6969647216));
#89016=CARTESIAN_POINT('Ctrl Pts',(7.91452273992938,-23.2518430212389,11.6602665109009));
#89017=CARTESIAN_POINT('Ctrl Pts',(7.89658289688478,-23.1996866341778,11.6241420094615));
#89018=CARTESIAN_POINT('Ctrl Pts',(7.86183588918055,-23.1523923703251,11.5920351112702));
#89019=CARTESIAN_POINT('Ctrl Pts',(7.81377648892191,-23.1147174093106,11.5671753477237));
#89020=CARTESIAN_POINT('Ctrl Pts',(7.75766059577219,-23.0890492050938,11.5510403468213));
#89021=CARTESIAN_POINT('Ctrl Pts',(7.91547477954,-23.3227166577,11.6832984902));
#89022=CARTESIAN_POINT('Ctrl Pts',(7.91611368027112,-23.2671793589699,11.6460281227172));
#89023=CARTESIAN_POINT('Ctrl Pts',(7.89817677511925,-23.2116420601397,11.6085483823846));
#89024=CARTESIAN_POINT('Ctrl Pts',(7.8615589396166,-23.1618034258408,11.5747131302309));
#89025=CARTESIAN_POINT('Ctrl Pts',(7.81033796782714,-23.1232141110753,11.5482906652978));
#89026=CARTESIAN_POINT('Ctrl Pts',(7.75066973611005,-23.098410069918,11.5310175530077));
#89027=CARTESIAN_POINT('Ctrl Pts',(7.91677660432,-23.3563766548,11.6571003353));
#89028=CARTESIAN_POINT('Ctrl Pts',(7.9207682851848,-23.2942792858749,11.619652082997));
#89029=CARTESIAN_POINT('Ctrl Pts',(7.90297924229356,-23.2321819169498,11.5801041049053));
#89030=CARTESIAN_POINT('Ctrl Pts',(7.8628578513892,-23.1775788143209,11.5430317511911));
#89031=CARTESIAN_POINT('Ctrl Pts',(7.80571697781476,-23.1377014621359,11.5133446867667));
#89032=CARTESIAN_POINT('Ctrl Pts',(7.7395970182243,-23.1152461674912,11.493386398801));
#89033=CARTESIAN_POINT('Ctrl Pts',(7.92150726931,-23.3879026248,11.6287650914));
#89034=CARTESIAN_POINT('Ctrl Pts',(7.92877476677365,-23.318688693446,11.5932981429158));
#89035=CARTESIAN_POINT('Ctrl Pts',(7.91116012626247,-23.249474761992,11.5528780102254));
#89036=CARTESIAN_POINT('Ctrl Pts',(7.86749085858668,-23.1900474596595,11.5125263244749));
#89037=CARTESIAN_POINT('Ctrl Pts',(7.8046060841006,-23.1497152870341,11.4785634108322));
#89038=CARTESIAN_POINT('Ctrl Pts',(7.73273866216467,-23.1310192862307,11.4543385166681));
#89039=CARTESIAN_POINT('Ctrl Pts',(7.92449811306,-23.4017307742,11.6153459759));
#89040=CARTESIAN_POINT('Ctrl Pts',(7.933160012689,-23.329167474491,11.5813212138622));
#89041=CARTESIAN_POINT('Ctrl Pts',(7.91558915602351,-23.2566041748821,11.5408186562867));
#89042=CARTESIAN_POINT('Ctrl Pts',(7.87030342328902,-23.194978958134,11.4989724871098));
#89043=CARTESIAN_POINT('Ctrl Pts',(7.80489676739664,-23.1546275335721,11.4628007513679));
#89044=CARTESIAN_POINT('Ctrl Pts',(7.73064661099946,-23.1379387567491,11.4362192511351));
#89045=CARTESIAN_POINT('Ctrl Pts',(7.93181038161,-23.4257772831,11.589727728));
#89046=CARTESIAN_POINT('Ctrl Pts',(7.94259898634281,-23.3469242604025,11.5595784538612));
#89047=CARTESIAN_POINT('Ctrl Pts',(7.9249159224873,-23.2680712378051,11.5196955912591));
#89048=CARTESIAN_POINT('Ctrl Pts',(7.87670243326465,-23.202465097965,11.4751415902794));
#89049=CARTESIAN_POINT('Ctrl Pts',(7.80703642869538,-23.1624609825163,11.4343063448108));
#89050=CARTESIAN_POINT('Ctrl Pts',(7.72912102101426,-23.149972994791,11.4024242587647));
#89051=CARTESIAN_POINT('Ctrl Pts',(7.9432480685,-23.4460266432,11.5624437668));
#89052=CARTESIAN_POINT('Ctrl Pts',(7.95449392576775,-23.3611564773106,11.5385890032017));
#89053=CARTESIAN_POINT('Ctrl Pts',(7.93588514160407,-23.2762863115213,11.5010092226736));
#89054=CARTESIAN_POINT('Ctrl Pts',(7.8850335890661,-23.2070923242712,11.4540126467371));
#89055=CARTESIAN_POINT('Ctrl Pts',(7.81252461794977,-23.1679811870594,11.4073832166432));
#89056=CARTESIAN_POINT('Ctrl Pts',(7.73312092819091,-23.1601101382277,11.3682475271265));
#89057=CARTESIAN_POINT('Ctrl Pts',(7.94999449773,-23.4537301075,11.5494738265));
#89058=CARTESIAN_POINT('Ctrl Pts',(7.96070890734367,-23.3664431521595,11.529053261775));
#89059=CARTESIAN_POINT('Ctrl Pts',(7.94044985180303,-23.2791561968191,11.4939666534735));
#89060=CARTESIAN_POINT('Ctrl Pts',(7.88853929471968,-23.2085200743833,11.4459866136166));
#89061=CARTESIAN_POINT('Ctrl Pts',(7.81626122848945,-23.1698936980673,11.3955452574941));
#89062=CARTESIAN_POINT('Ctrl Pts',(7.73703971994881,-23.1639670049992,11.3526526368584));
#89063=CARTESIAN_POINT('Ctrl Pts',(7.96050853719668,-23.4651190523151,11.5297147907699));
#89064=CARTESIAN_POINT('Ctrl Pts',(7.97009076391529,-23.3740252890692,11.515240726516));
#89065=CARTESIAN_POINT('Ctrl Pts',(7.94977536603235,-23.2829315258232,11.4813952869434));
#89066=CARTESIAN_POINT('Ctrl Pts',(7.89632703655667,-23.2102050064346,11.4319920118367));
#89067=CARTESIAN_POINT('Ctrl Pts',(7.82189905423964,-23.1723857998439,11.3782644258795));
#89068=CARTESIAN_POINT('Ctrl Pts',(7.74337446791057,-23.1696699763263,11.3290106935214));
#89069=CARTESIAN_POINT('Ctrl Pts',(7.97509183792815,-23.4709933117087,11.5096161616792));
#89070=CARTESIAN_POINT('Ctrl Pts',(7.98108947414199,-23.3778496890314,11.5016366199269));
#89071=CARTESIAN_POINT('Ctrl Pts',(7.95748972962179,-23.2847060664544,11.4721514013342));
#89072=CARTESIAN_POINT('Ctrl Pts',(7.9031883490932,-23.21081514454,11.4219514862163));
#89073=CARTESIAN_POINT('Ctrl Pts',(7.83094794647299,-23.1735479550381,11.3628364646954));
#89074=CARTESIAN_POINT('Ctrl Pts',(7.75581025806313,-23.1726118741218,11.3069002853781));
#89075=CARTESIAN_POINT('Ctrl Pts',(7.97861893248622,-23.473260396731,11.5041318446739));
#89076=CARTESIAN_POINT('Ctrl Pts',(7.9838658852677,-23.3793118654716,11.4980034647542));
#89077=CARTESIAN_POINT('Ctrl Pts',(7.96094626176686,-23.2853633341106,11.4680133231507));
#89078=CARTESIAN_POINT('Ctrl Pts',(7.90635986062969,-23.2110860736012,11.4175510811059));
#89079=CARTESIAN_POINT('Ctrl Pts',(7.83296289653072,-23.1739766319726,11.3585003064285));
#89080=CARTESIAN_POINT('Ctrl Pts',(7.75850686040753,-23.1737472812249,11.3006412853113));
#89081=CARTESIAN_POINT('Ctrl Pts',(7.98975597461567,-23.4742457267098,11.4913611376641));
#89082=CARTESIAN_POINT('Ctrl Pts',(7.99160755459269,-23.3799440577819,11.4893633092269));
#89083=CARTESIAN_POINT('Ctrl Pts',(7.96482946649136,-23.285642388855,11.4637948888249));
#89084=CARTESIAN_POINT('Ctrl Pts',(7.91005112742093,-23.2110984877512,11.4131466533274));
#89085=CARTESIAN_POINT('Ctrl Pts',(7.84038338301816,-23.1741586517633,11.349542256543));
#89086=CARTESIAN_POINT('Ctrl Pts',(7.76929114060095,-23.1742407835368,11.2875250338872));
#89087=CARTESIAN_POINT('Ctrl Pts',(7.99571961591542,-23.4742355477988,11.4849187987967));
#89088=CARTESIAN_POINT('Ctrl Pts',(7.99569557118151,-23.3799375266448,11.4849447735798));
#89089=CARTESIAN_POINT('Ctrl Pts',(7.96848591980764,-23.2856395054908,11.459797141352));
#89090=CARTESIAN_POINT('Ctrl Pts',(7.91373170704263,-23.2111278317668,11.4091703379498));
#89091=CARTESIAN_POINT('Ctrl Pts',(7.8444766974065,-23.1741567081313,11.3451248634117));
#89092=CARTESIAN_POINT('Ctrl Pts',(7.77526352266813,-23.1742356855177,11.2810807525728));
#89093=CARTESIAN_POINT('',(7.77537149291,-23.1742356128,11.2813340821));
#89094=CARTESIAN_POINT('Origin',(7.77692918256182,-23.4721143225786,11.2827740387544));
#89095=CARTESIAN_POINT('Ctrl Pts',(7.77537149291,-23.1742356128,11.2813340821));
#89096=CARTESIAN_POINT('Ctrl Pts',(7.76374104627574,-23.1742356128017,11.293912717408));
#89097=CARTESIAN_POINT('Ctrl Pts',(7.75422556697312,-23.1727644436418,11.3086587661566));
#89098=CARTESIAN_POINT('Ctrl Pts',(7.74700423060917,-23.1697651572032,11.325378445193));
#89099=CARTESIAN_POINT('Ctrl Pts',(7.7425104458973,-23.1678987232268,11.3357829789599));
#89100=CARTESIAN_POINT('Ctrl Pts',(7.73890541557416,-23.1654413846783,11.3469514170409));
#89101=CARTESIAN_POINT('Ctrl Pts',(7.73623506584673,-23.1623888293302,11.3588340890296));
#89102=CARTESIAN_POINT('Ctrl Pts',(7.73275431717079,-23.1584098830982,11.3743229197122));
#89103=CARTESIAN_POINT('Ctrl Pts',(7.73086161191565,-23.153418739856,11.3910253167369));
#89104=CARTESIAN_POINT('Ctrl Pts',(7.73066226175709,-23.147426234148,11.4088273827439));
#89105=CARTESIAN_POINT('Ctrl Pts',(7.73056258667781,-23.144429981294,11.4177284157475));
#89106=CARTESIAN_POINT('Ctrl Pts',(7.73088630262042,-23.1411837592989,11.4269043094893));
#89107=CARTESIAN_POINT('Ctrl Pts',(7.73164678524262,-23.1376912299659,11.4363405978422));
#89108=CARTESIAN_POINT('Ctrl Pts',(7.73202702655371,-23.1359449652994,11.4410587420186));
#89109=CARTESIAN_POINT('Ctrl Pts',(7.73251645269071,-23.1341371416057,11.4458419922498));
#89110=CARTESIAN_POINT('Ctrl Pts',(7.73311675196239,-23.1322683759517,11.4506885225852));
#89111=CARTESIAN_POINT('Ctrl Pts',(7.73344741043022,-23.1312390174017,11.4533581015279));
#89112=CARTESIAN_POINT('Ctrl Pts',(7.7339045178077,-23.1299666679476,11.4566347081119));
#89113=CARTESIAN_POINT('Ctrl Pts',(7.73433695096052,-23.1288177725429,11.4595445510173));
#89114=CARTESIAN_POINT('Ctrl Pts',(7.73468958557988,-23.1278808871744,11.4619174295504));
#89115=CARTESIAN_POINT('Ctrl Pts',(7.73502509891724,-23.127027931523,11.4640471871358));
#89116=CARTESIAN_POINT('Ctrl Pts',(7.73525192860467,-23.1264799476953,11.4654161591939));
#89117=CARTESIAN_POINT('Ctrl Pts',(7.73848253767501,-23.1186753188378,11.4849136667643));
#89118=CARTESIAN_POINT('Ctrl Pts',(7.74349539285463,-23.1097913251982,11.5057237030058));
#89119=CARTESIAN_POINT('Ctrl Pts',(7.75044578480054,-23.0997931642341,11.5276783169699));
#89120=CARTESIAN_POINT('Ctrl Pts',(7.75218693764301,-23.0972885103214,11.5331781993948));
#89121=CARTESIAN_POINT('Ctrl Pts',(7.75404978036979,-23.0947141448011,11.5387498051114));
#89122=CARTESIAN_POINT('Ctrl Pts',(7.75603694220467,-23.0920699629726,11.5443902905449));
#89123=CARTESIAN_POINT('Ctrl Pts',(7.76099673254253,-23.0854703054841,11.5584684721317));
#89124=CARTESIAN_POINT('Ctrl Pts',(7.76673081976914,-23.0784351413131,11.5729759213888));
#89125=CARTESIAN_POINT('Ctrl Pts',(7.7732818622679,-23.0709684340554,11.5878665021477));
#89126=CARTESIAN_POINT('Ctrl Pts',(7.77655738351728,-23.0672350804265,11.5953117925271));
#89127=CARTESIAN_POINT('Ctrl Pts',(7.7800371228966,-23.0633938664975,11.6028528881567));
#89128=CARTESIAN_POINT('Ctrl Pts',(7.78372668136522,-23.0594462135951,11.6104837314509));
#89129=CARTESIAN_POINT('Ctrl Pts',(7.78557146059952,-23.0574723871439,11.614299153098));
#89130=CARTESIAN_POINT('Ctrl Pts',(7.78746869256675,-23.0554719535869,11.6181370138669));
#89131=CARTESIAN_POINT('Ctrl Pts',(7.78941907716873,-23.053445127409,11.6219965567953));
#89132=CARTESIAN_POINT('Ctrl Pts',(7.79039426946972,-23.0524317143201,11.6239263282596));
#89133=CARTESIAN_POINT('Ctrl Pts',(7.79138274980825,-23.0514117032099,11.6258615203947));
#89134=CARTESIAN_POINT('Ctrl Pts',(7.79238460634559,-23.0503851245528,11.627802037852));
#89135=CARTESIAN_POINT('Ctrl Pts',(7.79327498135915,-23.0494727783717,11.6295266243501));
#89136=CARTESIAN_POINT('Ctrl Pts',(7.79457377940076,-23.0481531572387,11.6320118167801));
#89137=CARTESIAN_POINT('Ctrl Pts',(7.79522040103178,-23.0474982175083,11.6332407477843));
#89138=CARTESIAN_POINT('Ctrl Pts',(7.79530136283287,-23.0474162142198,11.6333946190171));
#89139=CARTESIAN_POINT('Ctrl Pts',(7.79537206171456,-23.0473446716066,11.6335288379675));
#89140=CARTESIAN_POINT('Ctrl Pts',(7.7954303926167,-23.0472857178485,11.6336394709482));
#89141=CARTESIAN_POINT('Ctrl Pts',(7.80208355969398,-23.0405615084088,11.6462581632275));
#89142=CARTESIAN_POINT('Ctrl Pts',(7.80998678809139,-23.0329991199816,11.6602784378245));
#89143=CARTESIAN_POINT('Ctrl Pts',(7.81927494322304,-23.02451481789,11.6755544342307));
#89144=CARTESIAN_POINT('Ctrl Pts',(7.82866197294038,-23.0159401984164,11.6909930471946));
#89145=CARTESIAN_POINT('Ctrl Pts',(7.83946339968006,-23.0064225736304,11.7077144456189));
#89146=CARTESIAN_POINT('Ctrl Pts',(7.85185402085194,-22.9958996979574,11.7255295814866));
#89147=CARTESIAN_POINT('Ctrl Pts',(7.86292576688609,-22.9864968919653,11.7414484492459));
#89148=CARTESIAN_POINT('Ctrl Pts',(7.87526695740995,-22.9762909665692,11.7582400059061));
#89149=CARTESIAN_POINT('Ctrl Pts',(7.88902654132087,-22.9652683672498,11.7757431592995));
#89150=CARTESIAN_POINT('Ctrl Pts',(7.90232388219312,-22.9546160639972,11.7926583072079));
#89151=CARTESIAN_POINT('Ctrl Pts',(7.91694624226786,-22.943200344013,11.8102376925225));
#89152=CARTESIAN_POINT('Ctrl Pts',(7.93304631206559,-22.9310481852965,11.8283161764112));
#89153=CARTESIAN_POINT('Ctrl Pts',(7.94839546150332,-22.9194628131537,11.8455514650963));
#89154=CARTESIAN_POINT('Ctrl Pts',(7.9650881246001,-22.9072076806557,11.8632399135403));
#89155=CARTESIAN_POINT('Ctrl Pts',(7.98326798754674,-22.8943501383266,11.8812261213315));
#89156=CARTESIAN_POINT('Ctrl Pts',(7.99253469834919,-22.8877963415932,11.8903941214712));
#89157=CARTESIAN_POINT('Ctrl Pts',(8.00218796093379,-22.8810867861946,11.8996393229713));
#89158=CARTESIAN_POINT('Ctrl Pts',(8.01224741425247,-22.8742356128,11.9089404857865));
#89159=CARTESIAN_POINT('Origin',(6.6707290414,-22.8742356128,10.2599605573));
#89160=CARTESIAN_POINT('',(5.39652599911,-23.1742356128,9.08180806924));
#89161=CARTESIAN_POINT('Origin',(5.39652599911,-22.8742356128,9.08180806924));
#89162=CARTESIAN_POINT('',(6.58594874601,-23.1742356128,10.1815710757));
#89163=CARTESIAN_POINT('Origin',(4.98919124473,-22.8742356128,9.52235136777));
#89164=CARTESIAN_POINT('',(4.62185483489,-23.1742356128,9.04794230167));
#89165=CARTESIAN_POINT('Origin',(4.62185483489,-22.8742356128,9.04794230167));
#89166=CARTESIAN_POINT('Origin',(4.98919124473,-23.1742356128,9.52235136777));
#89167=CARTESIAN_POINT('Origin',(0.00234331738803,-22.8742356128,3.08191746407));
#89168=CARTESIAN_POINT('',(0.972828518105,-23.1742356128,10.5646641188));
#89169=CARTESIAN_POINT('Origin',(0.972828518105,-22.8742356128,10.5646641188));
#89170=CARTESIAN_POINT('Origin',(0.00234331738835,-23.1742356128,3.08191746407));
#89171=CARTESIAN_POINT('Origin',(1.05,-22.8742356128,11.1596805575));
#89172=CARTESIAN_POINT('',(0.45,-23.1742356128,11.1596805575));
#89173=CARTESIAN_POINT('Origin',(0.45,-22.8742356128,11.1596805575));
#89174=CARTESIAN_POINT('Origin',(1.05,-23.1742356128,11.1596805575));
#89175=CARTESIAN_POINT('Origin',(0.45,-22.8742356128,2.93538176615));
#89176=CARTESIAN_POINT('',(0.45,-23.1742356128,14.92922515));
#89177=CARTESIAN_POINT('Origin',(0.45,-22.8742356128,14.92922515));
#89178=CARTESIAN_POINT('',(0.45,-23.1742356128,13.0444528538));
#89179=CARTESIAN_POINT('Ctrl Pts',(8.78908955148,-23.4742356128,12.6272235745));
#89180=CARTESIAN_POINT('Ctrl Pts',(8.78908955148,-23.3799878332,12.6272235745));
#89181=CARTESIAN_POINT('Ctrl Pts',(8.76403540825,-23.2856521198,12.6543202923));
#89182=CARTESIAN_POINT('Ctrl Pts',(8.71344985896,-23.2111401141,12.7090299003));
#89183=CARTESIAN_POINT('Ctrl Pts',(8.64940616788,-23.1742356128,12.7782948442));
#89184=CARTESIAN_POINT('Ctrl Pts',(8.58542217429,-23.1742356128,12.8474952237));
#89185=CARTESIAN_POINT('Ctrl Pts',(8.71988917196,-23.4742356128,12.5632395809));
#89186=CARTESIAN_POINT('Ctrl Pts',(8.72947215345,-23.3790967554,12.5721001887));
#89187=CARTESIAN_POINT('Ctrl Pts',(8.71152123069,-23.285897088,12.6066774531));
#89188=CARTESIAN_POINT('Ctrl Pts',(8.66821560358,-23.2117943285,12.6661101146));
#89189=CARTESIAN_POINT('Ctrl Pts',(8.60980196734,-23.1742356128,12.7407571089));
#89190=CARTESIAN_POINT('Ctrl Pts',(8.55126681507,-23.1742356128,12.8159145257));
#89191=CARTESIAN_POINT('Ctrl Pts',(8.65068769611,-23.4557342571,12.4992545736));
#89192=CARTESIAN_POINT('Ctrl Pts',(8.67114447119,-23.3616092561,12.5181692988));
#89193=CARTESIAN_POINT('Ctrl Pts',(8.6616791149,-23.2705882254,12.5620766304));
#89194=CARTESIAN_POINT('Ctrl Pts',(8.62409294795,-23.1983198307,12.6285650769));
#89195=CARTESIAN_POINT('Ctrl Pts',(8.568611422,-23.16211697,12.707808508));
#89196=CARTESIAN_POINT('Ctrl Pts',(8.51298776904,-23.1652660131,12.7860692819));
#89197=CARTESIAN_POINT('Ctrl Pts',(8.58504814405,-23.4187037356,12.4385629891));
#89198=CARTESIAN_POINT('Ctrl Pts',(8.61720687318,-23.3287980114,12.4682975647));
#89199=CARTESIAN_POINT('Ctrl Pts',(8.61787660959,-23.2418003868,12.5228744536));
#89200=CARTESIAN_POINT('Ctrl Pts',(8.58556282332,-23.1726965799,12.5981338043));
#89201=CARTESIAN_POINT('Ctrl Pts',(8.53069999004,-23.1387145708,12.6814672949));
#89202=CARTESIAN_POINT('Ctrl Pts',(8.47363957019,-23.1456118409,12.7605886079));
#89203=CARTESIAN_POINT('Ctrl Pts',(8.46797276655,-23.3115821157,12.3303128573));
#89204=CARTESIAN_POINT('Ctrl Pts',(8.52237213304,-23.2378310806,12.3806115513));
#89205=CARTESIAN_POINT('Ctrl Pts',(8.54446981637,-23.1647358306,12.4578324878));
#89206=CARTESIAN_POINT('Ctrl Pts',(8.52245288296,-23.1060736658,12.5529815994));
#89207=CARTESIAN_POINT('Ctrl Pts',(8.46636077569,-23.0779179681,12.6438102103));
#89208=CARTESIAN_POINT('Ctrl Pts',(8.40034769996,-23.089880852,12.7198837328));
#89209=CARTESIAN_POINT('Ctrl Pts',(8.38931991359,-23.1521307593,12.2575889261));
#89210=CARTESIAN_POINT('Ctrl Pts',(8.45970633708,-23.1061611813,12.3226695586));
#89211=CARTESIAN_POINT('Ctrl Pts',(8.4993062219,-23.0588540528,12.4194802488));
#89212=CARTESIAN_POINT('Ctrl Pts',(8.48540796624,-23.0202466991,12.5332516118));
#89213=CARTESIAN_POINT('Ctrl Pts',(8.42613724507,-23.0015045278,12.6297956016));
#89214=CARTESIAN_POINT('Ctrl Pts',(8.34720486119,-23.0113292253,12.6980018322));
#89215=CARTESIAN_POINT('Ctrl Pts',(8.36213066678,-23.0627326652,12.2324492288));
#89216=CARTESIAN_POINT('Ctrl Pts',(8.43792182062,-23.0327194928,12.3025271783));
#89217=CARTESIAN_POINT('Ctrl Pts',(8.48363550117,-23.0005841899,12.4073998633));
#89218=CARTESIAN_POINT('Ctrl Pts',(8.47259449573,-22.9739829087,12.5290848856));
#89219=CARTESIAN_POINT('Ctrl Pts',(8.41152527253,-22.9610560938,12.6277894396));
#89220=CARTESIAN_POINT('Ctrl Pts',(8.32640121972,-22.9690248134,12.6908033837));
#89221=CARTESIAN_POINT('Ctrl Pts',(8.34854625295,-22.9684833924,12.2198888201));
#89222=CARTESIAN_POINT('Ctrl Pts',(8.42693586094,-22.9542535279,12.29236935));
#89223=CARTESIAN_POINT('Ctrl Pts',(8.47477476029,-22.9392158893,12.4011922791));
#89224=CARTESIAN_POINT('Ctrl Pts',(8.46499990031,-22.9265127562,12.5267357874));
#89225=CARTESIAN_POINT('Ctrl Pts',(8.40290084109,-22.9193127846,12.6268959398));
#89226=CARTESIAN_POINT('Ctrl Pts',(8.31471092647,-22.9207536636,12.6874600337));
#89227=CARTESIAN_POINT('Ctrl Pts',(8.34854625295,-22.8742356128,12.2198888201));
#89228=CARTESIAN_POINT('Ctrl Pts',(8.4275605919,-22.8742356128,12.2929469882));
#89229=CARTESIAN_POINT('Ctrl Pts',(8.47411942559,-22.8742356128,12.4014233916));
#89230=CARTESIAN_POINT('Ctrl Pts',(8.4651120838,-22.8742356128,12.5258960706));
#89231=CARTESIAN_POINT('Ctrl Pts',(8.40342053421,-22.8742356128,12.6265390425));
#89232=CARTESIAN_POINT('Ctrl Pts',(8.31471092647,-22.8742356128,12.6874600337));
#89233=CARTESIAN_POINT('',(8.58542217429,-23.1742356128,12.8474952237));
#89234=CARTESIAN_POINT('Origin',(8.58542217429,-23.4742356128,12.8474952237));
#89235=CARTESIAN_POINT('Ctrl Pts',(8.31471092647,-22.8742356128,12.6874600337));
#89236=CARTESIAN_POINT('Ctrl Pts',(8.31471092647,-22.8777933584003,12.6874600337));
#89237=CARTESIAN_POINT('Ctrl Pts',(8.31479323139441,-22.8809325043544,12.6874789206066));
#89238=CARTESIAN_POINT('Ctrl Pts',(8.31492315770647,-22.8839115627938,12.6875091517772));
#89239=CARTESIAN_POINT('Ctrl Pts',(8.31506107853501,-22.8870739261499,12.6875412431067));
#89240=CARTESIAN_POINT('Ctrl Pts',(8.31525325722673,-22.8900565885356,12.6875861793263));
#89241=CARTESIAN_POINT('Ctrl Pts',(8.31551250222541,-22.8931767624084,12.6876505482859));
#89242=CARTESIAN_POINT('Ctrl Pts',(8.31567428634882,-22.8951239343789,12.6876907183018));
#89243=CARTESIAN_POINT('Ctrl Pts',(8.31586311600635,-22.89712476739,12.6877387266233));
#89244=CARTESIAN_POINT('Ctrl Pts',(8.31609186404498,-22.899256284786,12.6877992720059));
#89245=CARTESIAN_POINT('Ctrl Pts',(8.31703246295758,-22.9080209629744,12.6880482311724));
#89246=CARTESIAN_POINT('Ctrl Pts',(8.3184720943893,-22.9172029832652,12.6884570892979));
#89247=CARTESIAN_POINT('Ctrl Pts',(8.32049148999543,-22.9267496321353,12.6890982804029));
#89248=CARTESIAN_POINT('Ctrl Pts',(8.32297113453986,-22.9384720978654,12.6898856080671));
#89249=CARTESIAN_POINT('Ctrl Pts',(8.32631087462861,-22.9507561859589,12.6910381665959));
#89250=CARTESIAN_POINT('Ctrl Pts',(8.33074250887902,-22.963423387773,12.6926430971044));
#89251=CARTESIAN_POINT('Ctrl Pts',(8.33352902430523,-22.9713882493269,12.6936522425724));
#89252=CARTESIAN_POINT('Ctrl Pts',(8.3367465938535,-22.9795039863439,12.6948406517394));
#89253=CARTESIAN_POINT('Ctrl Pts',(8.34044372268016,-22.9877227211584,12.6962343599784));
#89254=CARTESIAN_POINT('Ctrl Pts',(8.34224120057069,-22.9917185229845,12.6969119559896));
#89255=CARTESIAN_POINT('Ctrl Pts',(8.34390869384712,-22.995219463642,12.6975515515556));
#89256=CARTESIAN_POINT('Ctrl Pts',(8.34552920341066,-22.9984967024445,12.6981802531784));
#89257=CARTESIAN_POINT('Ctrl Pts',(8.34726210727647,-23.0020012419535,12.6988525599004));
#89258=CARTESIAN_POINT('Ctrl Pts',(8.34894196075464,-23.0052499587694,12.6995125290509));
#89259=CARTESIAN_POINT('Ctrl Pts',(8.35071808844439,-23.0085506780283,12.7002171923411));
#89260=CARTESIAN_POINT('Ctrl Pts',(8.35170576082534,-23.0103861481176,12.7006090428109));
#89261=CARTESIAN_POINT('Ctrl Pts',(8.35272393885807,-23.0122373070308,12.7010150983056));
#89262=CARTESIAN_POINT('Ctrl Pts',(8.3538036353473,-23.0141539170075,12.701448202217));
#89263=CARTESIAN_POINT('Ctrl Pts',(8.35864062942183,-23.022740247697,12.7033884892088));
#89264=CARTESIAN_POINT('Ctrl Pts',(8.36383403677917,-23.031093409479,12.7055393286181));
#89265=CARTESIAN_POINT('Ctrl Pts',(8.36933050847485,-23.0391865217467,12.7079039186945));
#89266=CARTESIAN_POINT('Ctrl Pts',(8.37670817730011,-23.0500495454068,12.7110778024979));
#89267=CARTESIAN_POINT('Ctrl Pts',(8.38462952763295,-23.0604448682787,12.7146360574884));
#89268=CARTESIAN_POINT('Ctrl Pts',(8.39305270598872,-23.0703067991067,12.7185390012323));
#89269=CARTESIAN_POINT('Ctrl Pts',(8.39710320140982,-23.0750491545425,12.720415829087));
#89270=CARTESIAN_POINT('Ctrl Pts',(8.40127001039262,-23.0796676000566,12.7223723738313));
#89271=CARTESIAN_POINT('Ctrl Pts',(8.40555038878184,-23.0841506907025,12.724404563646));
#89272=CARTESIAN_POINT('Ctrl Pts',(8.405631874623,-23.0842360355901,12.7244432505754));
#89273=CARTESIAN_POINT('Ctrl Pts',(8.40571340166903,-23.0843213313238,12.7244819649315));
#89274=CARTESIAN_POINT('Ctrl Pts',(8.40579496984911,-23.084406577819,12.7245207066686));
#89275=CARTESIAN_POINT('Ctrl Pts',(8.40850861987399,-23.0872425998286,12.7258095856842));
#89276=CARTESIAN_POINT('Ctrl Pts',(8.41092778889889,-23.0896803647717,12.7269739252582));
#89277=CARTESIAN_POINT('Ctrl Pts',(8.41326672462745,-23.0919820120415,12.7281155702397));
#89278=CARTESIAN_POINT('Ctrl Pts',(8.41566938155185,-23.0943463646327,12.7292883178216));
#89279=CARTESIAN_POINT('Ctrl Pts',(8.41798793352237,-23.0965670756276,12.7304373235459));
#89280=CARTESIAN_POINT('Ctrl Pts',(8.42048300223408,-23.0988941811888,12.731700441442));
#89281=CARTESIAN_POINT('Ctrl Pts',(8.42150070885261,-23.0998433777862,12.7322156510781));
#89282=CARTESIAN_POINT('Ctrl Pts',(8.42254806424813,-23.1008098845419,12.7327501444207));
#89283=CARTESIAN_POINT('Ctrl Pts',(8.42364392096638,-23.101808858012,12.73331460736));
#89284=CARTESIAN_POINT('Ctrl Pts',(8.43004185632291,-23.1076411603363,12.7366101088038));
#89285=CARTESIAN_POINT('Ctrl Pts',(8.43685251341664,-23.1134783932573,12.7403437273528));
#89286=CARTESIAN_POINT('Ctrl Pts',(8.44411972875044,-23.1191908462093,12.7445439750782));
#89287=CARTESIAN_POINT('Ctrl Pts',(8.45142329300889,-23.1249318715254,12.748765231468));
#89288=CARTESIAN_POINT('Ctrl Pts',(8.45918899558952,-23.1305448328952,12.753452576356));
#89289=CARTESIAN_POINT('Ctrl Pts',(8.46745203663362,-23.1358786540093,12.7586265124918));
#89290=CARTESIAN_POINT('Ctrl Pts',(8.4756328294368,-23.141159383604,12.7637489485632));
#89291=CARTESIAN_POINT('Ctrl Pts',(8.4843014823735,-23.1461660797944,12.7693486066843));
#89292=CARTESIAN_POINT('Ctrl Pts',(8.49345089413583,-23.1507232195509,12.7754411948738));
#89293=CARTESIAN_POINT('Ctrl Pts',(8.49676613901879,-23.1523744769925,12.7776488145922));
#89294=CARTESIAN_POINT('Ctrl Pts',(8.49966497227245,-23.1537362767192,12.7796135340646));
#89295=CARTESIAN_POINT('Ctrl Pts',(8.50237503110583,-23.154959764541,12.7814721598892));
#89296=CARTESIAN_POINT('Ctrl Pts',(8.5052438883696,-23.1562549437753,12.7834396936312));
#89297=CARTESIAN_POINT('Ctrl Pts',(8.50790164006921,-23.1573947053208,12.7852887419358));
#89298=CARTESIAN_POINT('Ctrl Pts',(8.51062282062748,-23.1585068781719,12.7872069045525));
#89299=CARTESIAN_POINT('Ctrl Pts',(8.51207455775593,-23.1591002171975,12.7882302353568));
#89300=CARTESIAN_POINT('Ctrl Pts',(8.51354438219107,-23.1596849239924,12.7892736043561));
#89301=CARTESIAN_POINT('Ctrl Pts',(8.51507388564811,-23.1602748447744,12.79036794282));
#89302=CARTESIAN_POINT('Ctrl Pts',(8.51588296434197,-23.1605869018238,12.7909468273795));
#89303=CARTESIAN_POINT('Ctrl Pts',(8.51671436748897,-23.1609023851636,12.7915440936407));
#89304=CARTESIAN_POINT('Ctrl Pts',(8.51754234275166,-23.1612111635393,12.7921414367448));
#89305=CARTESIAN_POINT('Ctrl Pts',(8.52886755029603,-23.1654346945393,12.8003120125255));
#89306=CARTESIAN_POINT('Ctrl Pts',(8.54029588627425,-23.1686990756866,12.8090252630494));
#89307=CARTESIAN_POINT('Ctrl Pts',(8.55166402911457,-23.1708993416419,12.8182595233406));
#89308=CARTESIAN_POINT('Ctrl Pts',(8.56115568234122,-23.1727364193202,12.8259695246768));
#89309=CARTESIAN_POINT('Ctrl Pts',(8.57060899114612,-23.1738324293023,12.8340455882575));
#89310=CARTESIAN_POINT('Ctrl Pts',(8.57991872237668,-23.1741433117178,12.8424633105735));
#89311=CARTESIAN_POINT('Ctrl Pts',(8.58175924620776,-23.1742047728364,12.8441274852035));
#89312=CARTESIAN_POINT('Ctrl Pts',(8.58359405486515,-23.1742356128,12.8458049095361));
#89313=CARTESIAN_POINT('Ctrl Pts',(8.58542217429,-23.1742356128,12.8474952237));
#89314=CARTESIAN_POINT('Origin',(8.14487887576,-22.8742356128,12.4401604693));
#89315=CARTESIAN_POINT('',(8.48454297717,-23.1742356128,12.9347595981));
#89316=CARTESIAN_POINT('Origin',(8.14487887576,-23.1742356128,12.4401604693));
#89317=CARTESIAN_POINT('Origin',(8.48454297717,-22.8742356128,12.9347595981));
#89318=CARTESIAN_POINT('Origin',(1.05,-22.8742356128,14.92922515));
#89319=CARTESIAN_POINT('',(1.09378792023,-23.1742356128,15.5276251985));
#89320=CARTESIAN_POINT('Origin',(1.09378792023,-22.8742356128,15.5276251985));
#89321=CARTESIAN_POINT('Origin',(1.05,-23.1742356128,14.92922515));
#89322=CARTESIAN_POINT('Origin',(-2.61864828395E-15,-22.8742356128,0.580061096523));
#89323=CARTESIAN_POINT('Origin',(3.98755858312E-16,-23.1742356128,0.580061096523));
#89324=CARTESIAN_POINT('Origin',(8.21591479143,-23.4742356128,11.6886688365));
#89325=CARTESIAN_POINT('',(7.85913400544,-23.1742356128,11.2062712093));
#89326=CARTESIAN_POINT('Origin',(7.85913400544,-23.4742356128,11.2062712093));
#89327=CARTESIAN_POINT('Origin',(8.21591479143,-23.1742356128,11.6886688365));
#89328=CARTESIAN_POINT('Origin',(2.30650470794E-14,-23.4742356128,0.580061096523));
#89329=CARTESIAN_POINT('',(8.48602987721,-23.1742356128,10.7126632105));
#89330=CARTESIAN_POINT('Origin',(8.48602987717703,-23.4742356128,10.7126632104571));
#89331=CARTESIAN_POINT('Origin',(-8.67605652836E-16,-23.1742356128,0.580061096523));
#89332=CARTESIAN_POINT('Ctrl Pts',(12.9732843937,-22.9031898545,8.97133867634));
#89333=CARTESIAN_POINT('Ctrl Pts',(12.9781011914,-22.9849535816,8.94914145692));
#89334=CARTESIAN_POINT('Ctrl Pts',(12.9535953066,-23.0667173088,8.92058122207));
#89335=CARTESIAN_POINT('Ctrl Pts',(12.8986935104,-23.1346740075,8.88934991896));
#89336=CARTESIAN_POINT('Ctrl Pts',(12.8237786321,-23.1759719524,8.86135389883));
#89337=CARTESIAN_POINT('Ctrl Pts',(12.7426122303,-23.1887127298,8.84011906693));
#89338=CARTESIAN_POINT('Ctrl Pts',(12.9823757633,-22.8915014019,8.92944287783));
#89339=CARTESIAN_POINT('Ctrl Pts',(12.9862583246,-22.9763016188,8.91126726307));
#89340=CARTESIAN_POINT('Ctrl Pts',(12.9595430587,-23.0611018356,8.88653324147));
#89341=CARTESIAN_POINT('Ctrl Pts',(12.9012478152,-23.1309752745,8.85841244838));
#89342=CARTESIAN_POINT('Ctrl Pts',(12.822883741,-23.172105454,8.83249977476));
#89343=CARTESIAN_POINT('Ctrl Pts',(12.7392305459,-23.1828685028,8.81230742555));
#89344=CARTESIAN_POINT('Ctrl Pts',(12.9914751666,-22.882822481,8.8868408148));
#89345=CARTESIAN_POINT('Ctrl Pts',(12.9944056315,-22.9704026765,8.87289342313));
#89346=CARTESIAN_POINT('Ctrl Pts',(12.9654027633,-23.0579828719,8.85218917069));
#89347=CARTESIAN_POINT('Ctrl Pts',(12.9035898329,-23.1294730391,8.82727742946));
#89348=CARTESIAN_POINT('Ctrl Pts',(12.8217308477,-23.1700741969,8.8033687928));
#89349=CARTESIAN_POINT('Ctrl Pts',(12.7356821525,-23.1785290452,8.78399143876));
#89350=CARTESIAN_POINT('Ctrl Pts',(13.000513389,-22.8770866751,8.84380834125));
#89351=CARTESIAN_POINT('Ctrl Pts',(13.0024779758,-22.9671810863,8.834295766));
#89352=CARTESIAN_POINT('Ctrl Pts',(12.9711165232,-23.0572754975,8.81782605389));
#89353=CARTESIAN_POINT('Ctrl Pts',(12.9056733165,-23.1300795876,8.79620887499));
#89354=CARTESIAN_POINT('Ctrl Pts',(12.820300204,-23.1698045819,8.77418794581));
#89355=CARTESIAN_POINT('Ctrl Pts',(12.731982211,-23.1756611501,8.75535198255));
#89356=CARTESIAN_POINT('Ctrl Pts',(13.0094376369,-22.8742356128,8.80057964365));
#89357=CARTESIAN_POINT('Ctrl Pts',(13.0104250706,-22.9665621944,8.79571296462));
#89358=CARTESIAN_POINT('Ctrl Pts',(12.97663939,-23.0588887759,8.78368803172));
#89359=CARTESIAN_POINT('Ctrl Pts',(12.9074626588,-23.1326978759,8.76544020738));
#89360=CARTESIAN_POINT('Ctrl Pts',(12.8185800084,-23.171217802,8.7451543519));
#89361=CARTESIAN_POINT('Ctrl Pts',(12.728148167,-23.1742356128,8.7265439874));
#89362=CARTESIAN_POINT('Ctrl Pts',(13.018207968,-22.8742356128,8.75735407375));
#89363=CARTESIAN_POINT('Ctrl Pts',(13.018207968,-22.9684833924,8.75735407375));
#89364=CARTESIAN_POINT('Ctrl Pts',(12.9819360276,-23.0627311721,8.74999461196));
#89365=CARTESIAN_POINT('Ctrl Pts',(12.9089301686,-23.1372245963,8.73518195451));
#89366=CARTESIAN_POINT('Ctrl Pts',(12.8165644307,-23.1742356128,8.71644123897));
#89367=CARTESIAN_POINT('Ctrl Pts',(12.7241986928,-23.1742356128,8.69770052342));
#89368=CARTESIAN_POINT('',(12.7426122114145,-23.1887126377471,8.8401190872892));
#89369=CARTESIAN_POINT('',(12.7241986928,-23.1742356128,8.69770052342));
#89370=CARTESIAN_POINT('Origin',(12.6973454005032,-23.4896761342038,8.67085289361702));
#89371=CARTESIAN_POINT('Origin',(12.7262776236387,-22.8763569039497,8.69812233191237));
#89372=CARTESIAN_POINT('Origin',(12.6820770505264,-22.9047706797711,8.90769738430112));
#89373=CARTESIAN_POINT('Ctrl Pts',(12.8222448424,-23.4742356815,9.46100292006));
#89374=CARTESIAN_POINT('Ctrl Pts',(12.8494736832,-23.4742356636,9.39375104048));
#89375=CARTESIAN_POINT('Ctrl Pts',(12.8563714436,-23.4742356458,9.31826754191));
#89376=CARTESIAN_POINT('Ctrl Pts',(12.8394938336,-23.4742356301,9.24276446755));
#89377=CARTESIAN_POINT('Ctrl Pts',(12.8011121316,-23.4742356188,9.17740252767));
#89378=CARTESIAN_POINT('Ctrl Pts',(12.7478394439,-23.4742356125,9.1281455822));
#89379=CARTESIAN_POINT('Ctrl Pts',(12.8222448265,-23.4046541603,9.4610029458));
#89380=CARTESIAN_POINT('Ctrl Pts',(12.8494736715,-23.4136498524,9.39375106135));
#89381=CARTESIAN_POINT('Ctrl Pts',(12.8563714358,-23.4226455445,9.31826755752));
#89382=CARTESIAN_POINT('Ctrl Pts',(12.8394938286,-23.4305372305,9.24276447831));
#89383=CARTESIAN_POINT('Ctrl Pts',(12.801112128,-23.4362628909,9.17740253498));
#89384=CARTESIAN_POINT('Ctrl Pts',(12.7478394405,-23.4394448584,9.12814558784));
#89385=CARTESIAN_POINT('Ctrl Pts',(12.8267376752,-23.3350444003,9.44989804488));
#89386=CARTESIAN_POINT('Ctrl Pts',(12.8532287465,-23.3530402345,9.38369795688));
#89387=CARTESIAN_POINT('Ctrl Pts',(12.8592761475,-23.3710360687,9.30931517965));
#89388=CARTESIAN_POINT('Ctrl Pts',(12.8415116196,-23.3868230014,9.23486539817));
#89389=CARTESIAN_POINT('Ctrl Pts',(12.8023354301,-23.3982761819,9.17041054742));
#89390=CARTESIAN_POINT('Ctrl Pts',(12.7484601992,-23.4046400789,9.12185309334));
#89391=CARTESIAN_POINT('Ctrl Pts',(12.8357660159,-23.2683909506,9.42765504858));
#89392=CARTESIAN_POINT('Ctrl Pts',(12.8607726482,-23.2950473443,9.36356310571));
#89393=CARTESIAN_POINT('Ctrl Pts',(12.8651123819,-23.3217037379,9.29138732719));
#89394=CARTESIAN_POINT('Ctrl Pts',(12.8455698325,-23.3450683354,9.21904951484));
#89395=CARTESIAN_POINT('Ctrl Pts',(12.8048034097,-23.3619761005,9.15641249749));
#89396=CARTESIAN_POINT('Ctrl Pts',(12.7497239393,-23.3713130963,9.10925542748));
#89397=CARTESIAN_POINT('Ctrl Pts',(12.8654176334,-23.1205674467,9.35093873948));
#89398=CARTESIAN_POINT('Ctrl Pts',(12.8856609251,-23.1667016048,9.29404448239));
#89399=CARTESIAN_POINT('Ctrl Pts',(12.88434645,-23.2128357629,9.22937157743));
#89400=CARTESIAN_POINT('Ctrl Pts',(12.8587400955,-23.2531200257,9.16420855068));
#89401=CARTESIAN_POINT('Ctrl Pts',(12.8124201304,-23.2819402616,9.10778516284));
#89402=CARTESIAN_POINT('Ctrl Pts',(12.7530521925,-23.2974017916,9.06547349059));
#89403=CARTESIAN_POINT('Ctrl Pts',(12.9068680488,-23.010101918,9.22909905079));
#89404=CARTESIAN_POINT('Ctrl Pts',(12.9207907755,-23.0719215919,9.18344085273));
#89405=CARTESIAN_POINT('Ctrl Pts',(12.9112658476,-23.1337412658,9.13042485238));
#89406=CARTESIAN_POINT('Ctrl Pts',(12.8761980932,-23.187134812,9.07635129743));
#89407=CARTESIAN_POINT('Ctrl Pts',(12.8208608743,-23.2240649689,9.02951363011));
#89408=CARTESIAN_POINT('Ctrl Pts',(12.7544308643,-23.2421683956,8.99467312589));
#89409=CARTESIAN_POINT('Ctrl Pts',(12.9314667335,-22.9612266295,9.14763068363));
#89410=CARTESIAN_POINT('Ctrl Pts',(12.9418297489,-23.0307478118,9.10939417332));
#89411=CARTESIAN_POINT('Ctrl Pts',(12.9272163182,-23.1002689941,9.06405821655));
#89412=CARTESIAN_POINT('Ctrl Pts',(12.8858996435,-23.1597742276,9.01725069446));
#89413=CARTESIAN_POINT('Ctrl Pts',(12.8244369644,-23.1997556874,8.97665312932));
#89414=CARTESIAN_POINT('Ctrl Pts',(12.7531935733,-23.2177311451,8.94663366293));
#89415=CARTESIAN_POINT('Ctrl Pts',(12.9538489501,-22.9261034781,9.0609030715));
#89416=CARTESIAN_POINT('Ctrl Pts',(12.9611499959,-23.0022194475,9.03052977793));
#89417=CARTESIAN_POINT('Ctrl Pts',(12.941507993,-23.078335417,8.99337186849));
#89418=CARTESIAN_POINT('Ctrl Pts',(12.8935474744,-23.1426522193,8.95421942683));
#89419=CARTESIAN_POINT('Ctrl Pts',(12.8254935651,-23.1840524297,8.91999612505));
#89420=CARTESIAN_POINT('Ctrl Pts',(12.7492414901,-23.2001695455,8.89463935599));
#89421=CARTESIAN_POINT('Ctrl Pts',(12.9732844032,-22.9031895891,8.9713386779));
#89422=CARTESIAN_POINT('Ctrl Pts',(12.9781011912,-22.9849533577,8.94914147504));
#89423=CARTESIAN_POINT('Ctrl Pts',(12.9535952945,-23.0667171263,8.92058125628));
#89424=CARTESIAN_POINT('Ctrl Pts',(12.8986934857,-23.1346738584,8.88934996626));
#89425=CARTESIAN_POINT('Ctrl Pts',(12.8237785974,-23.1759718213,8.86135395422));
#89426=CARTESIAN_POINT('Ctrl Pts',(12.7426121901,-23.188712601,8.84011912524));
#89427=CARTESIAN_POINT('Ctrl Pts',(12.7478394286,-23.4742356128,9.12814559875));
#89428=CARTESIAN_POINT('Ctrl Pts',(12.7478394405,-23.4394448584,9.12814558784));
#89429=CARTESIAN_POINT('Ctrl Pts',(12.7484601992,-23.4046400789,9.12185309334));
#89430=CARTESIAN_POINT('Ctrl Pts',(12.7497239393,-23.3713130963,9.10925542748));
#89431=CARTESIAN_POINT('Ctrl Pts',(12.7530521925,-23.2974017916,9.06547349059));
#89432=CARTESIAN_POINT('Ctrl Pts',(12.7544308643,-23.2421683956,8.99467312589));
#89433=CARTESIAN_POINT('Ctrl Pts',(12.7531935733,-23.2177311451,8.94663366293));
#89434=CARTESIAN_POINT('Ctrl Pts',(12.7492414901,-23.2001695455,8.89463935599));
#89435=CARTESIAN_POINT('Ctrl Pts',(12.7426122014,-23.188712592,8.84011909812));
#89436=CARTESIAN_POINT('Origin',(6.6707290414,-23.4742356128,3.1005467775));
#89437=CARTESIAN_POINT('',(11.9421544921,-23.1742356128,7.97460750747));
#89438=CARTESIAN_POINT('Origin',(11.9421544921158,-23.4742356128,7.97460750744535));
#89439=CARTESIAN_POINT('',(12.3331765925,-23.1742356128,8.33615401544));
#89440=CARTESIAN_POINT('Ctrl Pts',(3.81744045688,-22.8742356128,-9.21387212773));
#89441=CARTESIAN_POINT('Ctrl Pts',(3.81744045688,-22.9684833924,-9.21387212773));
#89442=CARTESIAN_POINT('Ctrl Pts',(3.80220506528,-23.0627311721,-9.18014234586));
#89443=CARTESIAN_POINT('Ctrl Pts',(3.77154023633,-23.1372245963,-9.11225318231));
#89444=CARTESIAN_POINT('Ctrl Pts',(3.73274363021,-23.1742356128,-9.02636099807));
#89445=CARTESIAN_POINT('Ctrl Pts',(3.69394702409,-23.1742356128,-8.94046881382));
#89446=CARTESIAN_POINT('Ctrl Pts',(3.71160470889,-22.8742356128,-9.26167703413));
#89447=CARTESIAN_POINT('Ctrl Pts',(3.72515638761,-22.9642074605,-9.25555588183));
#89448=CARTESIAN_POINT('Ctrl Pts',(3.7250970863,-23.0541793081,-9.21865622161));
#89449=CARTESIAN_POINT('Ctrl Pts',(3.70844285493,-23.1271496569,-9.15193510136));
#89450=CARTESIAN_POINT('Ctrl Pts',(3.67843010495,-23.1675189946,-9.06966143177));
#89451=CARTESIAN_POINT('Ctrl Pts',(3.64200986566,-23.1742356128,-8.98738776219));
#89452=CARTESIAN_POINT('Ctrl Pts',(3.60518947181,-22.8967702026,-9.30860522068));
#89453=CARTESIAN_POINT('Ctrl Pts',(3.63104913481,-22.9796757788,-9.29721692608));
#89454=CARTESIAN_POINT('Ctrl Pts',(3.64474315,-23.0625813551,-9.25775017492));
#89455=CARTESIAN_POINT('Ctrl Pts',(3.64141126432,-23.131420749,-9.19204052568));
#89456=CARTESIAN_POINT('Ctrl Pts',(3.62129881914,-23.1730680404,-9.11274337915));
#89457=CARTESIAN_POINT('Ctrl Pts',(3.58978817426,-23.1855028319,-9.03344623294));
#89458=CARTESIAN_POINT('Ctrl Pts',(3.50276689342,-22.9419634255,-9.35255588844));
#89459=CARTESIAN_POINT('Ctrl Pts',(3.53957219131,-23.0156863099,-9.33675316789));
#89460=CARTESIAN_POINT('Ctrl Pts',(3.56543990858,-23.0894091943,-9.29523917398));
#89461=CARTESIAN_POINT('Ctrl Pts',(3.57431565494,-23.1517903264,-9.2303724476));
#89462=CARTESIAN_POINT('Ctrl Pts',(3.56438630978,-23.1921341626,-9.15347743429));
#89463=CARTESIAN_POINT('Ctrl Pts',(3.53952573637,-23.2081001313,-9.07658241785));
#89464=CARTESIAN_POINT('Ctrl Pts',(3.34853990601,-23.0590627588,-9.41717252271));
#89465=CARTESIAN_POINT('Ctrl Pts',(3.40101481294,-23.1138397009,-9.39536923091));
#89466=CARTESIAN_POINT('Ctrl Pts',(3.44422712818,-23.1686166429,-9.35116723508));
#89467=CARTESIAN_POINT('Ctrl Pts',(3.47088045966,-23.2161685094,-9.28743732801));
#89468=CARTESIAN_POINT('Ctrl Pts',(3.47682492232,-23.2495777226,-9.21371939274));
#89469=CARTESIAN_POINT('Ctrl Pts',(3.4638420321,-23.2666487717,-9.14000145959));
#89470=CARTESIAN_POINT('Ctrl Pts',(3.24903060406,-23.2324009559,-9.45772855228));
#89471=CARTESIAN_POINT('Ctrl Pts',(3.31106586193,-23.2635682408,-9.43250094395));
#89472=CARTESIAN_POINT('Ctrl Pts',(3.36479660614,-23.2947355258,-9.38683384758));
#89473=CARTESIAN_POINT('Ctrl Pts',(3.40250113652,-23.322122922,-9.32374506153));
#89474=CARTESIAN_POINT('Ctrl Pts',(3.41904507547,-23.3420909713,-9.25177549042));
#89475=CARTESIAN_POINT('Ctrl Pts',(3.41500902577,-23.3533185645,-9.17980591789));
#89476=CARTESIAN_POINT('Ctrl Pts',(3.22037852073,-23.3101536719,-9.46927274181));
#89477=CARTESIAN_POINT('Ctrl Pts',(3.28511942878,-23.331162522,-9.44310189027));
#89478=CARTESIAN_POINT('Ctrl Pts',(3.34181908965,-23.3521713721,-9.39703707137));
#89479=CARTESIAN_POINT('Ctrl Pts',(3.38266593906,-23.3706950509,-9.33412380265));
#89480=CARTESIAN_POINT('Ctrl Pts',(3.40228901679,-23.384336583,-9.2626299648));
#89481=CARTESIAN_POINT('Ctrl Pts',(3.40094883361,-23.3921942807,-9.19113612813));
#89482=CARTESIAN_POINT('Ctrl Pts',(3.2061108834,-23.3922234913,-9.47502541989));
#89483=CARTESIAN_POINT('Ctrl Pts',(3.27219964976,-23.4027249383,-9.44838409371));
#89484=CARTESIAN_POINT('Ctrl Pts',(3.33037855145,-23.4132263854,-9.4021208728));
#89485=CARTESIAN_POINT('Ctrl Pts',(3.37279084839,-23.422485337,-9.33929519246));
#89486=CARTESIAN_POINT('Ctrl Pts',(3.393947035,-23.4293033961,-9.26803870195));
#89487=CARTESIAN_POINT('Ctrl Pts',(3.39394702816,-23.4332296702,-9.19678221123));
#89488=CARTESIAN_POINT('Ctrl Pts',(3.20611087388,-23.4742356128,-9.47502544833));
#89489=CARTESIAN_POINT('Ctrl Pts',(3.27219964627,-23.4742356465,-9.44838411889));
#89490=CARTESIAN_POINT('Ctrl Pts',(3.33037855462,-23.4742356801,-9.40212089616));
#89491=CARTESIAN_POINT('Ctrl Pts',(3.37279085872,-23.4742357098,-9.33929521563));
#89492=CARTESIAN_POINT('Ctrl Pts',(3.39394705252,-23.4742357316,-9.26803872592));
#89493=CARTESIAN_POINT('Ctrl Pts',(3.39394705213,-23.4742357442,-9.19678223621));
#89494=CARTESIAN_POINT('',(3.69394702409,-23.1742356128,-8.94046881382));
#89495=CARTESIAN_POINT('Ctrl Pts',(3.69394702409,-23.1742356128,-8.94046881382));
#89496=CARTESIAN_POINT('Ctrl Pts',(3.64200986566,-23.1742356128,-8.98738776219));
#89497=CARTESIAN_POINT('Ctrl Pts',(3.58978817426,-23.1855028319,-9.03344623294));
#89498=CARTESIAN_POINT('Ctrl Pts',(3.53952573637,-23.2081001313,-9.07658241785));
#89499=CARTESIAN_POINT('Ctrl Pts',(3.4638420321,-23.2666487717,-9.14000145959));
#89500=CARTESIAN_POINT('Ctrl Pts',(3.41500902577,-23.3533185645,-9.17980591789));
#89501=CARTESIAN_POINT('Ctrl Pts',(3.40094883361,-23.3921942807,-9.19113612813));
#89502=CARTESIAN_POINT('Ctrl Pts',(3.39394702816,-23.4332296702,-9.19678221123));
#89503=CARTESIAN_POINT('Ctrl Pts',(3.39394702409,-23.4742356128,-9.19678210318));
#89504=CARTESIAN_POINT('Origin',(3.69482032662239,-22.876356953309,-8.94240205678344));
#89505=CARTESIAN_POINT('Origin',(3.69394702409,-23.4742356128,3.39628270998));
#89506=CARTESIAN_POINT('',(3.69394702409,-23.1742356128,-8.44362980932));
#89507=CARTESIAN_POINT('Ctrl Pts',(9.06991786197,-22.8742351711,13.3798726472));
#89508=CARTESIAN_POINT('Ctrl Pts',(9.06991791346,-22.9684830268,13.3798726085));
#89509=CARTESIAN_POINT('Ctrl Pts',(9.04851963512,-23.0627308825,13.3496744364));
#89510=CARTESIAN_POINT('Ctrl Pts',(9.00545047601,-23.1372243637,13.2888935201));
#89511=CARTESIAN_POINT('Ctrl Pts',(8.95096009845,-23.1742354012,13.2119945921));
#89512=CARTESIAN_POINT('Ctrl Pts',(8.89646970336,-23.1742353894,13.1350956831));
#89513=CARTESIAN_POINT('Ctrl Pts',(9.22406041417,-22.8742363569,13.2706476151));
#89514=CARTESIAN_POINT('Ctrl Pts',(9.20132424908,-22.9647386701,13.2867584141));
#89515=CARTESIAN_POINT('Ctrl Pts',(9.15852680885,-23.0552409834,13.275328887));
#89516=CARTESIAN_POINT('Ctrl Pts',(9.10021479707,-23.128400233,13.232683254));
#89517=CARTESIAN_POINT('Ctrl Pts',(9.0393710411,-23.168352818,13.1677082076));
#89518=CARTESIAN_POINT('Ctrl Pts',(8.986120014,-23.1742360128,13.0945214235));
#89519=CARTESIAN_POINT('Ctrl Pts',(9.3768173424,-22.9427255764,13.1589191215));
#89520=CARTESIAN_POINT('Ctrl Pts',(9.33383370545,-23.019699187,13.1904054535));
#89521=CARTESIAN_POINT('Ctrl Pts',(9.27188264132,-23.0966727976,13.1965141601));
#89522=CARTESIAN_POINT('Ctrl Pts',(9.19881019143,-23.1602830893,13.1710975036));
#89523=CARTESIAN_POINT('Ctrl Pts',(9.1296041316,-23.1981089887,13.1188723071));
#89524=CARTESIAN_POINT('Ctrl Pts',(9.07411181992,-23.2084805514,13.051815332));
#89525=CARTESIAN_POINT('Ctrl Pts',(9.5056235281,-23.0835945845,13.0599834668));
#89526=CARTESIAN_POINT('Ctrl Pts',(9.44694848687,-23.1391655975,13.1046059873));
#89527=CARTESIAN_POINT('Ctrl Pts',(9.36995382261,-23.1947366105,13.1251829804));
#89528=CARTESIAN_POINT('Ctrl Pts',(9.2844923694,-23.2410848235,13.113878162));
#89529=CARTESIAN_POINT('Ctrl Pts',(9.20688851793,-23.2696054116,13.0728111063));
#89530=CARTESIAN_POINT('Ctrl Pts',(9.14715364651,-23.2789180606,13.0124182766));
#89531=CARTESIAN_POINT('Ctrl Pts',(9.57074430825,-23.2789184576,13.0098414435));
#89532=CARTESIAN_POINT('Ctrl Pts',(9.50407307406,-23.3067030636,13.0611772932));
#89533=CARTESIAN_POINT('Ctrl Pts',(9.41940322383,-23.3344876695,13.0891378612));
#89534=CARTESIAN_POINT('Ctrl Pts',(9.32764499777,-23.3576610293,13.0850021715));
#89535=CARTESIAN_POINT('Ctrl Pts',(9.2458338001,-23.3719208617,13.049538037));
#89536=CARTESIAN_POINT('Ctrl Pts',(9.18405109086,-23.3765770352,12.9924125631));
#89537=CARTESIAN_POINT('Ctrl Pts',(9.57074430825,-23.4742356128,13.0098414435));
#89538=CARTESIAN_POINT('Ctrl Pts',(9.50407307406,-23.4742356128,13.0611772932));
#89539=CARTESIAN_POINT('Ctrl Pts',(9.41940322382,-23.4742356128,13.0891378611));
#89540=CARTESIAN_POINT('Ctrl Pts',(9.32764499778,-23.4742356128,13.0850021715));
#89541=CARTESIAN_POINT('Ctrl Pts',(9.2458338001,-23.4742356128,13.049538037));
#89542=CARTESIAN_POINT('Ctrl Pts',(9.18405109086,-23.4742356128,12.9924125631));
#89543=CARTESIAN_POINT('',(8.89646971542626,-23.1742355011026,13.1350957106811));
#89544=CARTESIAN_POINT('Ctrl Pts',(8.89646970862946,-23.1742353894,13.1350956905365));
#89545=CARTESIAN_POINT('Ctrl Pts',(8.91341513014285,-23.1742355071256,13.1274264703531));
#89546=CARTESIAN_POINT('Ctrl Pts',(8.93029127126005,-23.1757068619148,13.1196632450321));
#89547=CARTESIAN_POINT('Ctrl Pts',(8.94689277562026,-23.1786594058135,13.11190151293));
#89548=CARTESIAN_POINT('Ctrl Pts',(8.96413730237382,-23.1817263099414,13.1038391473766));
#89549=CARTESIAN_POINT('Ctrl Pts',(8.98108480439148,-23.1863918522805,13.0957789597802));
#89550=CARTESIAN_POINT('Ctrl Pts',(8.99748754661613,-23.1926227295045,13.0878568815035));
#89551=CARTESIAN_POINT('Ctrl Pts',(9.01388437542077,-23.1988513604093,13.0799376592479));
#89552=CARTESIAN_POINT('Ctrl Pts',(9.02973598052021,-23.2066444162773,13.0721572366115));
#89553=CARTESIAN_POINT('Ctrl Pts',(9.04478970250645,-23.2159201010348,13.0646691125016));
#89554=CARTESIAN_POINT('Ctrl Pts',(9.05953393120249,-23.2250050846357,13.0573349386354));
#89555=CARTESIAN_POINT('Ctrl Pts',(9.07351197595636,-23.2355123975707,13.0502819205507));
#89556=CARTESIAN_POINT('Ctrl Pts',(9.08649348099754,-23.2473169973954,13.0436598229282));
#89557=CARTESIAN_POINT('Ctrl Pts',(9.09906099757469,-23.258745141013,13.0372489082166));
#89558=CARTESIAN_POINT('Ctrl Pts',(9.11069392323561,-23.2713890780425,13.0312424769986));
#89559=CARTESIAN_POINT('Ctrl Pts',(9.12119976253034,-23.28509010912,13.0257718268833));
#89560=CARTESIAN_POINT('Ctrl Pts',(9.13117359321529,-23.2980973292328,13.0205782067968));
#89561=CARTESIAN_POINT('Ctrl Pts',(9.14013124265935,-23.3120570858951,13.0158678825228));
#89562=CARTESIAN_POINT('Ctrl Pts',(9.14792971774513,-23.3267943578383,13.0117419122437));
#89563=CARTESIAN_POINT('Ctrl Pts',(9.1554919724439,-23.3410852291655,13.0077409200259));
#89564=CARTESIAN_POINT('Ctrl Pts',(9.16196389354133,-23.3561071559953,13.004289751406));
#89565=CARTESIAN_POINT('Ctrl Pts',(9.16724094845525,-23.3716644543252,13.0014643636574));
#89566=CARTESIAN_POINT('Ctrl Pts',(9.17238371002682,-23.3868258421284,12.9987108779015));
#89567=CARTESIAN_POINT('Ctrl Pts',(9.17639137749551,-23.4024956538032,12.9965520057846));
#89568=CARTESIAN_POINT('Ctrl Pts',(9.17919641784377,-23.4184587554085,12.9950379956692));
#89569=CARTESIAN_POINT('Ctrl Pts',(9.18191243967219,-23.4339152647724,12.9935720329694));
#89570=CARTESIAN_POINT('Ctrl Pts',(9.18350078228183,-23.449646661283,12.9927108436825));
#89571=CARTESIAN_POINT('Ctrl Pts',(9.1839310101514,-23.4654263360779,12.9924776563453));
#89572=CARTESIAN_POINT('Ctrl Pts',(9.18401104207622,-23.4683617055323,12.9924342783293));
#89573=CARTESIAN_POINT('Ctrl Pts',(9.18405109089593,-23.4712986577741,12.9924125631332));
#89574=CARTESIAN_POINT('Ctrl Pts',(9.18405109086,-23.4742356128,12.9924125631));
#89575=CARTESIAN_POINT('',(9.069917864047,-22.8742353916481,13.3798726501317));
#89576=CARTESIAN_POINT('Ctrl Pts',(9.06991786197,-22.8742351711,13.3798726472));
#89577=CARTESIAN_POINT('Ctrl Pts',(9.08998575407497,-22.8742353255134,13.3656525883774));
#89578=CARTESIAN_POINT('Ctrl Pts',(9.10955660519836,-22.8756242289139,13.3517136535672));
#89579=CARTESIAN_POINT('Ctrl Pts',(9.12864703192581,-22.8782518413693,13.3380519691444));
#89580=CARTESIAN_POINT('Ctrl Pts',(9.14793774246996,-22.8809070209535,13.3242469555893));
#89581=CARTESIAN_POINT('Ctrl Pts',(9.16673844715609,-22.88482699622,13.310724778741));
#89582=CARTESIAN_POINT('Ctrl Pts',(9.18507464936658,-22.889909819839,13.2974764327235));
#89583=CARTESIAN_POINT('Ctrl Pts',(9.20358499520628,-22.8950409163415,13.2841022637558));
#89584=CARTESIAN_POINT('Ctrl Pts',(9.22162263549148,-22.9013571522458,13.271006726178));
#89585=CARTESIAN_POINT('Ctrl Pts',(9.23921303209337,-22.9088067632157,13.2581807473248));
#89586=CARTESIAN_POINT('Ctrl Pts',(9.25678868288205,-22.9162501292683,13.245365520332));
#89587=CARTESIAN_POINT('Ctrl Pts',(9.27391854665928,-22.9248252575798,13.232818884081));
#89588=CARTESIAN_POINT('Ctrl Pts',(9.29061694379971,-22.934530243736,13.2205390954791));
#89589=CARTESIAN_POINT('Ctrl Pts',(9.30710079952112,-22.9441105399902,13.2084170779046));
#89590=CARTESIAN_POINT('Ctrl Pts',(9.32316487751703,-22.9547923032227,13.1965545677702));
#89591=CARTESIAN_POINT('Ctrl Pts',(9.33880195550392,-22.9666165308916,13.1849647453894));
#89592=CARTESIAN_POINT('Ctrl Pts',(9.35387417400676,-22.9780136309893,13.1737935831378));
#89593=CARTESIAN_POINT('Ctrl Pts',(9.36855017700297,-22.9904727776667,13.1628753549093));
#89594=CARTESIAN_POINT('Ctrl Pts',(9.382795583024,-23.004062622776,13.1522424354472));
#89595=CARTESIAN_POINT('Ctrl Pts',(9.39534907250807,-23.0160384118421,13.1428723801146));
#89596=CARTESIAN_POINT('Ctrl Pts',(9.4075680781392,-23.0288929873676,13.1337239314646));
#89597=CARTESIAN_POINT('Ctrl Pts',(9.41940527139236,-23.0426889421547,13.1248372557628));
#89598=CARTESIAN_POINT('Ctrl Pts',(9.43131771533443,-23.0565725997511,13.1158940862238));
#89599=CARTESIAN_POINT('Ctrl Pts',(9.44248897416376,-23.0710261714051,13.1074823780018));
#89600=CARTESIAN_POINT('Ctrl Pts',(9.4529877344115,-23.0860428865014,13.0995587831363));
#89601=CARTESIAN_POINT('Ctrl Pts',(9.46345139189945,-23.1010093929892,13.0916616809272));
#89602=CARTESIAN_POINT('Ctrl Pts',(9.47324759923271,-23.1165359483353,13.0842489546468));
#89603=CARTESIAN_POINT('Ctrl Pts',(9.48241933488591,-23.13265844651,13.0772947232701));
#89604=CARTESIAN_POINT('Ctrl Pts',(9.4916372236028,-23.1488620746599,13.0703054975265));
#89605=CARTESIAN_POINT('Ctrl Pts',(9.50022492714466,-23.165668329315,13.0637789008759));
#89606=CARTESIAN_POINT('Ctrl Pts',(9.50819213354862,-23.183146856145,13.0577131974299));
#89607=CARTESIAN_POINT('Ctrl Pts',(9.51615933995259,-23.200625382975,13.0516474939839));
#89608=CARTESIAN_POINT('Ctrl Pts',(9.52350662524997,-23.2187770242996,13.0460422080318));
#89609=CARTESIAN_POINT('Ctrl Pts',(9.53020114144296,-23.237693246794,13.0409273075514));
#89610=CARTESIAN_POINT('Ctrl Pts',(9.53760959696005,-23.2586267973092,13.0352669264887));
#89611=CARTESIAN_POINT('Ctrl Pts',(9.54395926915395,-23.2798231161351,13.0304053695222));
#89612=CARTESIAN_POINT('Ctrl Pts',(9.54930506873862,-23.3012669711949,13.0263077604947));
#89613=CARTESIAN_POINT('Ctrl Pts',(9.55465924086306,-23.3227444114139,13.0222037338315));
#89614=CARTESIAN_POINT('Ctrl Pts',(9.55900668819699,-23.344471439241,13.0188657804003));
#89615=CARTESIAN_POINT('Ctrl Pts',(9.56236311517375,-23.3664524350163,13.0162868858771));
#89616=CARTESIAN_POINT('Ctrl Pts',(9.5656336340413,-23.3878708248423,13.0137739984365));
#89617=CARTESIAN_POINT('Ctrl Pts',(9.56796318463351,-23.409531684921,13.0119818130114));
#89618=CARTESIAN_POINT('Ctrl Pts',(9.56932722686825,-23.4314384942518,13.0109321578799));
#89619=CARTESIAN_POINT('Ctrl Pts',(9.57020916152404,-23.4456025529991,13.0102534932363));
#89620=CARTESIAN_POINT('Ctrl Pts',(9.57068667570032,-23.4598693913192,13.0098858196983));
#89621=CARTESIAN_POINT('Ctrl Pts',(9.57074430825,-23.4742356128,13.0098414435));
#89622=CARTESIAN_POINT('Origin',(8.89769590716719,-22.8763565140159,13.1368267800033));
#89623=CARTESIAN_POINT('Origin',(6.6707290414,-23.4742356128,11.0771333555));
#89624=CARTESIAN_POINT('',(8.74094594938,-23.1742356128,12.9912954789));
#89625=CARTESIAN_POINT('Origin',(-2.84607155346,-22.8742356128,5.53854202767));
#89626=CARTESIAN_POINT('Origin',(-2.84607155346,-23.1742356128,5.53854202767));
#89627=CARTESIAN_POINT('Origin',(10.1862176145,-22.8742356128,9.72278707155));
#89628=CARTESIAN_POINT('',(11.1383462684,-22.8742356128,10.0284846777));
#89629=CARTESIAN_POINT('Ctrl Pts',(11.138346268408,-22.8742356128,10.0284846777026));
#89630=CARTESIAN_POINT('Ctrl Pts',(11.1304025349713,-22.8879754443996,10.0532263049571));
#89631=CARTESIAN_POINT('Ctrl Pts',(11.1227115500163,-22.9011602400043,10.0769601464436));
#89632=CARTESIAN_POINT('Ctrl Pts',(11.1149362788915,-22.9142785484054,10.1007522253721));
#89633=CARTESIAN_POINT('Ctrl Pts',(11.1089402979403,-22.9243948679554,10.1190997337428));
#89634=CARTESIAN_POINT('Ctrl Pts',(11.1028949842124,-22.9344737618983,10.1374798306995));
#89635=CARTESIAN_POINT('Ctrl Pts',(11.0966317645807,-22.9447233863069,10.1563922783035));
#89636=CARTESIAN_POINT('Ctrl Pts',(11.0947731720942,-22.9477649329931,10.1620044929607));
#89637=CARTESIAN_POINT('Ctrl Pts',(11.0928952369663,-22.9508212969781,10.1676637551768));
#89638=CARTESIAN_POINT('Ctrl Pts',(11.090993057621,-22.9538972342935,10.1733836478105));
#89639=CARTESIAN_POINT('',(10.9304145503,-22.8742356128,10.3907473403));
#89640=CARTESIAN_POINT('Ctrl Pts',(10.9304145503437,-22.8742356128,10.3907473403392));
#89641=CARTESIAN_POINT('Ctrl Pts',(10.9481405479233,-22.8882672659973,10.3709982119854));
#89642=CARTESIAN_POINT('Ctrl Pts',(10.9645717766644,-22.9013026990597,10.3525880372788));
#89643=CARTESIAN_POINT('Ctrl Pts',(10.9810103536057,-22.9142753573368,10.3340804995609));
#89644=CARTESIAN_POINT('Ctrl Pts',(10.992000443497,-22.9229482905903,10.3217071959644));
#89645=CARTESIAN_POINT('Ctrl Pts',(11.002992272732,-22.9315950772944,10.3092917362859));
#89646=CARTESIAN_POINT('Ctrl Pts',(11.0143770648586,-22.9404798718002,10.2963873039649));
#89647=CARTESIAN_POINT('Ctrl Pts',(11.0200212309283,-22.944884629931,10.2899897555297));
#89648=CARTESIAN_POINT('Ctrl Pts',(11.0257621179678,-22.9493475068719,10.2834716325873));
#89649=CARTESIAN_POINT('Ctrl Pts',(11.031648508022,-22.9538972342928,10.2767748704144));
#89650=CARTESIAN_POINT('Origin',(10.1862176145,-22.8742356128,9.72278707155));
#89651=CARTESIAN_POINT('Ctrl Pts',(11.9005548436,-23.1693861532,7.89557218486));
#89652=CARTESIAN_POINT('Ctrl Pts',(11.8339499555,-23.1595472711,7.96980237474));
#89653=CARTESIAN_POINT('Ctrl Pts',(11.7599452826,-23.1908783468,8.04284981847));
#89654=CARTESIAN_POINT('Ctrl Pts',(11.6942870876,-23.2663663442,8.09701806802));
#89655=CARTESIAN_POINT('Ctrl Pts',(11.6548578916,-23.3654515188,8.11755397837));
#89656=CARTESIAN_POINT('Ctrl Pts',(11.6438378503,-23.4645366935,8.10736463748));
#89657=CARTESIAN_POINT('Ctrl Pts',(11.8668157199,-23.1614761236,7.83132058431));
#89658=CARTESIAN_POINT('Ctrl Pts',(11.8129234492,-23.1460753827,7.92069454621));
#89659=CARTESIAN_POINT('Ctrl Pts',(11.7451516804,-23.1734640687,8.00787961054));
#89660=CARTESIAN_POINT('Ctrl Pts',(11.6772007057,-23.2482114783,8.07033400293));
#89661=CARTESIAN_POINT('Ctrl Pts',(11.6288782137,-23.3484640563,8.08997448939));
#89662=CARTESIAN_POINT('Ctrl Pts',(11.6054955414,-23.4487166343,8.07191260584));
#89663=CARTESIAN_POINT('Ctrl Pts',(11.8201190291,-23.1436931675,7.77911937176));
#89664=CARTESIAN_POINT('Ctrl Pts',(11.7896480761,-23.1271929291,7.88233980762));
#89665=CARTESIAN_POINT('Ctrl Pts',(11.7361184989,-23.1516755686,7.98200912796));
#89666=CARTESIAN_POINT('Ctrl Pts',(11.6667987778,-23.2222222498,8.05091722103));
#89667=CARTESIAN_POINT('Ctrl Pts',(11.6024958012,-23.3176864267,8.06826984747));
#89668=CARTESIAN_POINT('Ctrl Pts',(11.5554237252,-23.4131506081,8.04186749464));
#89669=CARTESIAN_POINT('Ctrl Pts',(11.7752729456,-23.1083028984,7.76843597189));
#89670=CARTESIAN_POINT('Ctrl Pts',(11.7595402729,-23.1052304081,7.86585583205));
#89671=CARTESIAN_POINT('Ctrl Pts',(11.7167014673,-23.1327309513,7.95914759566));
#89672=CARTESIAN_POINT('Ctrl Pts',(11.6496136328,-23.1915820263,8.02617572742));
#89673=CARTESIAN_POINT('Ctrl Pts',(11.5756983226,-23.2669761984,8.04953640203));
#89674=CARTESIAN_POINT('Ctrl Pts',(11.5102889752,-23.3423703627,8.03319245204));
#89675=CARTESIAN_POINT('Ctrl Pts',(11.717675025,-23.0445100599,7.76252036052));
#89676=CARTESIAN_POINT('Ctrl Pts',(11.7084114695,-23.0501289834,7.8515782493));
#89677=CARTESIAN_POINT('Ctrl Pts',(11.6708968566,-23.0738598269,7.93631728547));
#89678=CARTESIAN_POINT('Ctrl Pts',(11.6066799831,-23.1148476696,8.0001560579));
#89679=CARTESIAN_POINT('Ctrl Pts',(11.5292674801,-23.1648160129,8.02969505599));
#89680=CARTESIAN_POINT('Ctrl Pts',(11.4529027709,-23.2147843626,8.02583184946));
#89681=CARTESIAN_POINT('Ctrl Pts',(11.6840057838,-22.9724912879,7.77196745159));
#89682=CARTESIAN_POINT('Ctrl Pts',(11.6739934323,-22.9791841994,7.85280062059));
#89683=CARTESIAN_POINT('Ctrl Pts',(11.6374046012,-22.9945001244,7.92955173236));
#89684=CARTESIAN_POINT('Ctrl Pts',(11.575491188,-23.017355905,7.98966707089));
#89685=CARTESIAN_POINT('Ctrl Pts',(11.4989860406,-23.044051495,8.02274251311));
#89686=CARTESIAN_POINT('Ctrl Pts',(11.4203500465,-23.0707470797,8.02802946276));
#89687=CARTESIAN_POINT('Ctrl Pts',(11.674734675,-22.9402340389,7.77528500471));
#89688=CARTESIAN_POINT('Ctrl Pts',(11.6632751245,-22.9448939304,7.85395206414));
#89689=CARTESIAN_POINT('Ctrl Pts',(11.6261291027,-22.9551888401,7.92866239052));
#89690=CARTESIAN_POINT('Ctrl Pts',(11.5648099781,-22.9704904338,7.98774399745));
#89691=CARTESIAN_POINT('Ctrl Pts',(11.4893943947,-22.9883613924,8.02148806052));
#89692=CARTESIAN_POINT('Ctrl Pts',(11.4114432261,-23.0062323557,8.02896986926));
#89693=CARTESIAN_POINT('Ctrl Pts',(11.6698654776,-22.907226316,7.77708988832));
#89694=CARTESIAN_POINT('Ctrl Pts',(11.6579204713,-22.9095613324,7.85454768026));
#89695=CARTESIAN_POINT('Ctrl Pts',(11.6206811584,-22.914710848,7.92810475864));
#89696=CARTESIAN_POINT('Ctrl Pts',(11.5596933648,-22.9223583919,7.98661599137));
#89697=CARTESIAN_POINT('Ctrl Pts',(11.4846565636,-22.931287768,8.02077577683));
#89698=CARTESIAN_POINT('Ctrl Pts',(11.4067703651,-22.9402171391,8.02950137053));
#89699=CARTESIAN_POINT('Ctrl Pts',(11.6698655273,-22.8742356121,7.77708987718));
#89700=CARTESIAN_POINT('Ctrl Pts',(11.6579205194,-22.8742356226,7.85454767439));
#89701=CARTESIAN_POINT('Ctrl Pts',(11.6206812044,-22.8742356357,7.92810475784));
#89702=CARTESIAN_POINT('Ctrl Pts',(11.5596934089,-22.87423565,7.98661599254));
#89703=CARTESIAN_POINT('Ctrl Pts',(11.4846566078,-22.8742356631,8.02077577467));
#89704=CARTESIAN_POINT('Ctrl Pts',(11.4067704135,-22.8742356736,8.02950136067));
#89705=CARTESIAN_POINT('',(11.669865562592,-22.8742356128,7.77708987370031));
#89706=CARTESIAN_POINT('Origin',(11.3748952831028,-22.8742356444552,7.73295572116956));
#89707=CARTESIAN_POINT('',(11.9005548348247,-23.1693861585283,7.89557218624769));
#89708=CARTESIAN_POINT('Ctrl Pts',(11.6698655614,-22.8742356128,7.77708988131));
#89709=CARTESIAN_POINT('Ctrl Pts',(11.6698654776,-22.907226316,7.77708988832));
#89710=CARTESIAN_POINT('Ctrl Pts',(11.674734675,-22.9402340389,7.77528500471));
#89711=CARTESIAN_POINT('Ctrl Pts',(11.6840057838,-22.9724912879,7.77196745159));
#89712=CARTESIAN_POINT('Ctrl Pts',(11.717675025,-23.0445100599,7.76252036052));
#89713=CARTESIAN_POINT('Ctrl Pts',(11.7752729456,-23.1083028984,7.76843597189));
#89714=CARTESIAN_POINT('Ctrl Pts',(11.8201190291,-23.1436931675,7.77911937176));
#89715=CARTESIAN_POINT('Ctrl Pts',(11.8668157199,-23.1614761236,7.83132058431));
#89716=CARTESIAN_POINT('Ctrl Pts',(11.900554836,-23.1693861518,7.89557218629));
#89717=CARTESIAN_POINT('Ctrl Pts',(11.6438378503,-23.4645366935,8.10736463748));
#89718=CARTESIAN_POINT('Ctrl Pts',(11.6457407548972,-23.4474269895683,8.10912409945425));
#89719=CARTESIAN_POINT('Ctrl Pts',(11.6486630325428,-23.4303180321677,8.10978091601121));
#89720=CARTESIAN_POINT('Ctrl Pts',(11.65256298317,-23.4134680180269,8.10932257821117));
#89721=CARTESIAN_POINT('Ctrl Pts',(11.6565377789634,-23.3962946300209,8.10885544430778));
#89722=CARTESIAN_POINT('Ctrl Pts',(11.6615279369715,-23.37939060852,8.10723006852047));
#89723=CARTESIAN_POINT('Ctrl Pts',(11.6674552116862,-23.3630165572466,8.10447292972245));
#89724=CARTESIAN_POINT('Ctrl Pts',(11.6735237627704,-23.3462522310777,8.10165007462501));
#89725=CARTESIAN_POINT('Ctrl Pts',(11.6805744213503,-23.3300439067293,8.09764098964142));
#89726=CARTESIAN_POINT('Ctrl Pts',(11.6884909237533,-23.3146514397464,8.09251343822578));
#89727=CARTESIAN_POINT('Ctrl Pts',(11.6964815336893,-23.2991148816364,8.0873378870539));
#89728=CARTESIAN_POINT('Ctrl Pts',(11.7053539547591,-23.2844099860543,8.08102307394607));
#89729=CARTESIAN_POINT('Ctrl Pts',(11.7149602963441,-23.2707770127254,8.073675339938));
#89730=CARTESIAN_POINT('Ctrl Pts',(11.7245993021421,-23.2570976835241,8.06630262160608));
#89731=CARTESIAN_POINT('Ctrl Pts',(11.7349768686908,-23.2444980259262,8.05789023480772));
#89732=CARTESIAN_POINT('Ctrl Pts',(11.745920364852,-23.2331869359498,8.04857827595082));
#89733=CARTESIAN_POINT('Ctrl Pts',(11.756829296706,-23.2219115713012,8.03929572829864));
#89734=CARTESIAN_POINT('Ctrl Pts',(11.7683002094792,-23.2119170519958,8.02911960219298));
#89735=CARTESIAN_POINT('Ctrl Pts',(11.7801446348235,-23.2033704216458,8.01821646048037));
#89736=CARTESIAN_POINT('Ctrl Pts',(11.7918096503827,-23.1949532487468,8.00747847074887));
#89737=CARTESIAN_POINT('Ctrl Pts',(11.8038365705567,-23.1879407235758,7.99603566767177));
#89738=CARTESIAN_POINT('Ctrl Pts',(11.8160340495087,-23.1824486649995,7.98406915540296));
#89739=CARTESIAN_POINT('Ctrl Pts',(11.8280723255704,-23.1770282893999,7.97225883142101));
#89740=CARTESIAN_POINT('Ctrl Pts',(11.840276398251,-23.1730892198954,7.95993868610934));
#89741=CARTESIAN_POINT('Ctrl Pts',(11.8524564888357,-23.1706957080467,7.94729963439744));
#89742=CARTESIAN_POINT('Ctrl Pts',(11.8643709607006,-23.1683543929817,7.93493621025267));
#89743=CARTESIAN_POINT('Ctrl Pts',(11.8762621855935,-23.1674921212114,7.92226792528629));
#89744=CARTESIAN_POINT('Ctrl Pts',(11.8879515998144,-23.1681206308898,7.90948528184542));
#89745=CARTESIAN_POINT('Ctrl Pts',(11.892181889249,-23.1683480826509,7.90485936300358));
#89746=CARTESIAN_POINT('Ctrl Pts',(11.8963857612096,-23.1687702957837,7.90021856034556));
#89747=CARTESIAN_POINT('Ctrl Pts',(11.9005548359276,-23.1693861518639,7.89557218635399));
#89748=CARTESIAN_POINT('Ctrl Pts',(11.9421544921,-23.1742356128,7.97460750747));
#89749=CARTESIAN_POINT('Ctrl Pts',(11.8781704985,-23.1742356128,8.04380788698));
#89750=CARTESIAN_POINT('Ctrl Pts',(11.8141865049,-23.2112466293,8.11300826649));
#89751=CARTESIAN_POINT('Ctrl Pts',(11.7636135705,-23.2857400536,8.16770423124));
#89752=CARTESIAN_POINT('Ctrl Pts',(11.7384871149,-23.3799878332,8.19487915673));
#89753=CARTESIAN_POINT('Ctrl Pts',(11.7384871149,-23.4742356128,8.19487915673));
#89754=CARTESIAN_POINT('Ctrl Pts',(11.9338050766,-23.1742356128,7.95878179633));
#89755=CARTESIAN_POINT('Ctrl Pts',(11.8690129979,-23.1723658919,8.02885614127));
#89756=CARTESIAN_POINT('Ctrl Pts',(11.8029049395,-23.2084420454,8.09871370492));
#89757=CARTESIAN_POINT('Ctrl Pts',(11.7493954495,-23.283359451,8.15328464759));
#89758=CARTESIAN_POINT('Ctrl Pts',(11.7215525483,-23.3787975319,8.17922113275));
#89759=CARTESIAN_POINT('Ctrl Pts',(11.7194707712,-23.4742356128,8.17729628178));
#89760=CARTESIAN_POINT('Ctrl Pts',(11.925456866,-23.1737486504,7.94293960289));
#89761=CARTESIAN_POINT('Ctrl Pts',(11.8599896787,-23.169946111,8.01395123592));
#89762=CARTESIAN_POINT('Ctrl Pts',(11.7918088017,-23.204981018,8.08451905773));
#89763=CARTESIAN_POINT('Ctrl Pts',(11.7353200262,-23.2802129884,8.13897414048));
#89764=CARTESIAN_POINT('Ctrl Pts',(11.704689803,-23.37673734,8.16362951651));
#89765=CARTESIAN_POINT('Ctrl Pts',(11.7004667677,-23.4732616915,8.15972481694));
#89766=CARTESIAN_POINT('Ctrl Pts',(11.9171250584,-23.1727778426,7.92710974195));
#89767=CARTESIAN_POINT('Ctrl Pts',(11.8511250917,-23.166992891,7.99912450114));
#89768=CARTESIAN_POINT('Ctrl Pts',(11.7809316294,-23.2008856654,8.07045852272));
#89769=CARTESIAN_POINT('Ctrl Pts',(11.721423774,-23.276320039,8.12480753543));
#89770=CARTESIAN_POINT('Ctrl Pts',(11.6879347422,-23.3738200593,8.14813746342));
#89771=CARTESIAN_POINT('Ctrl Pts',(11.6815098074,-23.471320079,8.14219684908));
#89772=CARTESIAN_POINT('Ctrl Pts',(11.9088198181,-23.171323915,7.91131175397));
#89773=CARTESIAN_POINT('Ctrl Pts',(11.8424378979,-23.1635210449,7.98439851249));
#89774=CARTESIAN_POINT('Ctrl Pts',(11.7703001202,-23.1961765665,8.0565580465));
#89775=CARTESIAN_POINT('Ctrl Pts',(11.7077347865,-23.2716977713,8.11081129139));
#89776=CARTESIAN_POINT('Ctrl Pts',(11.6713131361,-23.3700549965,8.13276881012));
#89777=CARTESIAN_POINT('Ctrl Pts',(11.6626231066,-23.4684122213,8.12473384452));
#89778=CARTESIAN_POINT('Ctrl Pts',(11.9005548343,-23.1693861722,7.89557218484));
#89779=CARTESIAN_POINT('Ctrl Pts',(11.8339499495,-23.1595472906,7.96980237485));
#89780=CARTESIAN_POINT('Ctrl Pts',(11.7599452801,-23.1908783692,8.04284981853));
#89781=CARTESIAN_POINT('Ctrl Pts',(11.6942870876,-23.2663663719,8.09701806797));
#89782=CARTESIAN_POINT('Ctrl Pts',(11.6548578924,-23.3654515527,8.11755397832));
#89783=CARTESIAN_POINT('Ctrl Pts',(11.6438378503,-23.4645367334,8.10736463748));
#89784=CARTESIAN_POINT('Origin',(11.9551818975745,-22.3491879643317,7.96775954099132));
#89785=CARTESIAN_POINT('Origin',(-2.84607155346,-22.8742356128,5.53854202767));
#89786=CARTESIAN_POINT('',(11.7512376696,-22.8742356128,3.91309124051));
#89787=CARTESIAN_POINT('Origin',(-2.84607155346,-22.8742356128,5.53854202767));
#89788=CARTESIAN_POINT('',(12.0493948734,-23.1742356128,3.87989061057));
#89789=CARTESIAN_POINT('Origin',(12.0493948734,-22.8742356128,3.87989061057));
#89790=CARTESIAN_POINT('Origin',(-2.84607155346,-23.1742356128,5.53854202767));
#89791=CARTESIAN_POINT('Origin',(11.4530804658,-22.8742356128,3.94629187045));
#89792=CARTESIAN_POINT('',(11.4530804658,-22.8742356128,3.64629187045));
#89793=CARTESIAN_POINT('Origin',(11.4530804658,-22.8742356128,3.94629187045));
#89794=CARTESIAN_POINT('',(11.4530804658,-23.1742356128,3.34629187045));
#89795=CARTESIAN_POINT('Origin',(11.4530804658,-22.8742356128,3.34629187045));
#89796=CARTESIAN_POINT('Origin',(11.4530804658,-23.1742356128,3.94629187045));
#89797=CARTESIAN_POINT('Origin',(-6.6707290414,-22.8742356128,3.34629187045));
#89798=CARTESIAN_POINT('',(8.10176909975,-22.8742356128,3.64629187045));
#89799=CARTESIAN_POINT('',(9.77742478279,-22.8742356128,3.64629187045));
#89800=CARTESIAN_POINT('',(8.10176909975,-23.1742356128,3.34629187045));
#89801=CARTESIAN_POINT('Origin',(8.10176909975,-22.8742356128,3.34629187045));
#89802=CARTESIAN_POINT('',(9.77742478279,-23.1742356128,3.34629187045));
#89803=CARTESIAN_POINT('Origin',(8.10176909975,-22.8742356128,3.94629187045));
#89804=CARTESIAN_POINT('',(7.80346303227,-22.8742356128,3.91445651114));
#89805=CARTESIAN_POINT('Origin',(8.10176909975,-22.8742356128,3.94629187045));
#89806=CARTESIAN_POINT('',(7.50515696478,-23.1742356128,3.88262115182));
#89807=CARTESIAN_POINT('Origin',(7.50515696478,-22.8742356128,3.88262115182));
#89808=CARTESIAN_POINT('Origin',(8.10176909975,-23.1742356128,3.94629187045));
#89809=CARTESIAN_POINT('Origin',(0.00234331738835,-22.8742356128,3.08191746407));
#89810=CARTESIAN_POINT('',(6.23264645859,-22.8742356128,7.84992678029));
#89811=CARTESIAN_POINT('Origin',(0.00234331738835,-22.8742356128,3.08191746407));
#89812=CARTESIAN_POINT('',(5.99440665492,-23.1742356128,7.66760345225));
#89813=CARTESIAN_POINT('Origin',(5.99440665492,-22.8742356128,7.66760345225));
#89814=CARTESIAN_POINT('Origin',(0.00234331738835,-23.1742356128,3.08191746407));
#89815=CARTESIAN_POINT('Origin',(6.47088626226,-22.8742356128,8.03225010833));
#89816=CARTESIAN_POINT('',(6.26721888507,-22.8742356128,8.25252175759));
#89817=CARTESIAN_POINT('Origin',(6.47088626226,-22.8742356128,8.03225010833));
#89818=CARTESIAN_POINT('',(6.06355150788,-23.1742356128,8.47279340685));
#89819=CARTESIAN_POINT('Origin',(6.06355150788,-22.8742356128,8.47279340685));
#89820=CARTESIAN_POINT('Origin',(6.47088626226,-23.1742356128,8.03225010833));
#89821=CARTESIAN_POINT('Ctrl Pts',(8.73611662316,-23.4697910609,10.8942571942));
#89822=CARTESIAN_POINT('Ctrl Pts',(8.72752432309,-23.3771104598,10.9015348722));
#89823=CARTESIAN_POINT('Ctrl Pts',(8.69545860941,-23.2844298587,10.881098933));
#89824=CARTESIAN_POINT('Ctrl Pts',(8.6413960311,-23.2107990757,10.8311116668));
#89825=CARTESIAN_POINT('Ctrl Pts',(8.57793853593,-23.1733813929,10.7632250691));
#89826=CARTESIAN_POINT('Ctrl Pts',(8.51747666777,-23.1720133445,10.6920986219));
#89827=CARTESIAN_POINT('Ctrl Pts',(8.72470175689,-23.4715681133,10.9039255852));
#89828=CARTESIAN_POINT('Ctrl Pts',(8.7177987489,-23.3784476295,10.9097561006));
#89829=CARTESIAN_POINT('Ctrl Pts',(8.68736831632,-23.2853271458,10.8877470417));
#89830=CARTESIAN_POINT('Ctrl Pts',(8.63454393537,-23.211417996,10.8363489167));
#89831=CARTESIAN_POINT('Ctrl Pts',(8.57168882428,-23.1740163051,10.7675887259));
#89832=CARTESIAN_POINT('Ctrl Pts',(8.51124350946,-23.1729018671,10.696222277));
#89833=CARTESIAN_POINT('Ctrl Pts',(8.71323427675,-23.4729019084,10.9136114204));
#89834=CARTESIAN_POINT('Ctrl Pts',(8.70803661002,-23.3794040149,10.9179891886));
#89835=CARTESIAN_POINT('Ctrl Pts',(8.67925545718,-23.2859061213,10.8943982297));
#89836=CARTESIAN_POINT('Ctrl Pts',(8.62767478659,-23.2117711836,10.8415808992));
#89837=CARTESIAN_POINT('Ctrl Pts',(8.5654164258,-23.1744185718,10.771945772));
#89838=CARTESIAN_POINT('Ctrl Pts',(8.50497501432,-23.1735687617,10.7003455662));
#89839=CARTESIAN_POINT('Ctrl Pts',(8.70172748022,-23.4737911951,10.9233030613));
#89840=CARTESIAN_POINT('Ctrl Pts',(8.69824977302,-23.3799791247,10.9262239001));
#89841=CARTESIAN_POINT('Ctrl Pts',(8.67113050266,-23.2861670544,10.9010437414));
#89842=CARTESIAN_POINT('Ctrl Pts',(8.62079773014,-23.2118592846,10.8468003207));
#89843=CARTESIAN_POINT('Ctrl Pts',(8.55912932234,-23.1745884938,10.7762902146));
#89844=CARTESIAN_POINT('Ctrl Pts',(8.49867834935,-23.1740134037,10.7044634205));
#89845=CARTESIAN_POINT('Ctrl Pts',(8.69019480669,-23.4742356128,10.9329890024));
#89846=CARTESIAN_POINT('Ctrl Pts',(8.68845018412,-23.3801733377,10.9344501196));
#89847=CARTESIAN_POINT('Ctrl Pts',(8.66300395829,-23.2861110626,10.9076749542));
#89848=CARTESIAN_POINT('Ctrl Pts',(8.61392194556,-23.2116837148,10.8520000359));
#89849=CARTESIAN_POINT('Ctrl Pts',(8.55283556198,-23.1745270026,10.7806162216));
#89850=CARTESIAN_POINT('Ctrl Pts',(8.49236081888,-23.1742356128,10.7085709021));
#89851=CARTESIAN_POINT('Ctrl Pts',(8.67864985337,-23.4742356128,10.942657873));
#89852=CARTESIAN_POINT('Ctrl Pts',(8.67864985337,-23.3799878332,10.942657873));
#89853=CARTESIAN_POINT('Ctrl Pts',(8.65488631632,-23.2857400536,10.9142834188));
#89854=CARTESIAN_POINT('Ctrl Pts',(8.60705657762,-23.2112466293,10.8571731189));
#89855=CARTESIAN_POINT('Ctrl Pts',(8.54654322741,-23.1742356128,10.7849181647));
#89856=CARTESIAN_POINT('Ctrl Pts',(8.48602987721,-23.1742356128,10.7126632105));
#89857=CARTESIAN_POINT('',(8.51747674095254,-23.1720132750395,10.6920985878956));
#89858=CARTESIAN_POINT('Origin',(8.54339070302529,-23.4677320541598,10.6671045573098));
#89859=CARTESIAN_POINT('Origin',(8.46564327939413,-22.8727019153709,10.6937226627841));
#89860=CARTESIAN_POINT('Ctrl Pts',(8.73611663424,-23.4697908757,10.8942572059));
#89861=CARTESIAN_POINT('Ctrl Pts',(8.72752435034,-23.3771103023,10.9015348641));
#89862=CARTESIAN_POINT('Ctrl Pts',(8.69545865342,-23.2844297289,10.881098906));
#89863=CARTESIAN_POINT('Ctrl Pts',(8.64139608915,-23.2107989673,10.8311116257));
#89864=CARTESIAN_POINT('Ctrl Pts',(8.57793860163,-23.1733812942,10.7632250217));
#89865=CARTESIAN_POINT('Ctrl Pts',(8.51747673428,-23.1720132443,10.6920985753));
#89866=CARTESIAN_POINT('Ctrl Pts',(8.85271909481,-23.4283765706,10.7986501186));
#89867=CARTESIAN_POINT('Ctrl Pts',(8.80174479507,-23.3522217493,10.8290472717));
#89868=CARTESIAN_POINT('Ctrl Pts',(8.74702097884,-23.2760669279,10.8249995844));
#89869=CARTESIAN_POINT('Ctrl Pts',(8.69926483364,-23.2110252232,10.7808433397));
#89870=CARTESIAN_POINT('Ctrl Pts',(8.66655321101,-23.1680969408,10.704046549));
#89871=CARTESIAN_POINT('Ctrl Pts',(8.64928312709,-23.1513060056,10.6105493344));
#89872=CARTESIAN_POINT('Ctrl Pts',(8.95374236957,-23.2551805764,10.8169485727));
#89873=CARTESIAN_POINT('Ctrl Pts',(8.90906105284,-23.2232432649,10.7961844516));
#89874=CARTESIAN_POINT('Ctrl Pts',(8.87369407635,-23.1913059533,10.770178964));
#89875=CARTESIAN_POINT('Ctrl Pts',(8.84720879161,-23.1552341963,10.7456901634));
#89876=CARTESIAN_POINT('Ctrl Pts',(8.82709666423,-23.1116114836,10.7203986113));
#89877=CARTESIAN_POINT('Ctrl Pts',(8.81389010608,-23.0647081339,10.6876384968));
#89878=CARTESIAN_POINT('Ctrl Pts',(9.01791018836,-23.1549008445,10.8214049608));
#89879=CARTESIAN_POINT('Ctrl Pts',(8.99622746462,-23.1216722312,10.8155316644));
#89880=CARTESIAN_POINT('Ctrl Pts',(8.97425273896,-23.0884436179,10.8039507789));
#89881=CARTESIAN_POINT('Ctrl Pts',(8.95224692858,-23.0584727018,10.783603786));
#89882=CARTESIAN_POINT('Ctrl Pts',(8.93220449355,-23.0344758471,10.7563348016));
#89883=CARTESIAN_POINT('Ctrl Pts',(8.91487253124,-23.0145682268,10.7261343735));
#89884=CARTESIAN_POINT('Ctrl Pts',(9.08532173979,-23.0061361581,10.858062108));
#89885=CARTESIAN_POINT('Ctrl Pts',(9.07401122054583,-22.994360504385,10.847601774363));
#89886=CARTESIAN_POINT('Ctrl Pts',(9.06350105813443,-22.9825848532249,10.8378821902984));
#89887=CARTESIAN_POINT('Ctrl Pts',(9.05419277619886,-22.9699073952249,10.8292755748936));
#89888=CARTESIAN_POINT('Ctrl Pts',(9.04554579428692,-22.955591884285,10.8212820971294));
#89889=CARTESIAN_POINT('Ctrl Pts',(9.03689844897,-22.9401858313,10.8132890077));
#89890=CARTESIAN_POINT('Ctrl Pts',(9.1336794452,-22.8742356128,10.9029059811));
#89891=CARTESIAN_POINT('Ctrl Pts',(9.1336794452,-22.8742356128,10.9029059811));
#89892=CARTESIAN_POINT('Ctrl Pts',(9.1336794452,-22.8742356128,10.9029059811));
#89893=CARTESIAN_POINT('Ctrl Pts',(9.1336794452,-22.8742356128,10.9029059811));
#89894=CARTESIAN_POINT('Ctrl Pts',(9.1336794452,-22.8742356128,10.9029059811));
#89895=CARTESIAN_POINT('Ctrl Pts',(9.1336794452,-22.8742356128,10.9029059811));
#89896=CARTESIAN_POINT('Ctrl Pts',(9.1336794452,-22.8742356128,10.9029059811));
#89897=CARTESIAN_POINT('Ctrl Pts',(9.12513493716062,-22.8800589421312,10.894993962939));
#89898=CARTESIAN_POINT('Ctrl Pts',(9.1165963718414,-22.8858083341009,10.8873291251196));
#89899=CARTESIAN_POINT('Ctrl Pts',(9.10813461288467,-22.891442518539,10.8799452426598));
#89900=CARTESIAN_POINT('Ctrl Pts',(9.0987334575265,-22.897702191438,10.8717416260707));
#89901=CARTESIAN_POINT('Ctrl Pts',(9.08942655406422,-22.9038201324466,10.8638840973876));
#89902=CARTESIAN_POINT('Ctrl Pts',(9.08026451623907,-22.9097707148096,10.8563787344658));
#89903=CARTESIAN_POINT('Ctrl Pts',(9.06975354042648,-22.9165974086611,10.8477683478202));
#89904=CARTESIAN_POINT('Ctrl Pts',(9.05943264238283,-22.9232043535186,10.8396206480343));
#89905=CARTESIAN_POINT('Ctrl Pts',(9.04932970007876,-22.9295830542483,10.8319075912454));
#89906=CARTESIAN_POINT('Ctrl Pts',(9.03694696588163,-22.9374011485502,10.8224540351238));
#89907=CARTESIAN_POINT('Ctrl Pts',(9.02489106059946,-22.9448769807609,10.813652296514));
#89908=CARTESIAN_POINT('Ctrl Pts',(9.01315523782939,-22.9520273019305,10.8054156098417));
#89909=CARTESIAN_POINT('Ctrl Pts',(9.00003909933142,-22.9600186123484,10.7962101604006));
#89910=CARTESIAN_POINT('Ctrl Pts',(8.98732119582686,-22.9676044421161,10.7877087692407));
#89911=CARTESIAN_POINT('Ctrl Pts',(8.97494743412375,-22.9748283264758,10.7797773122612));
#89912=CARTESIAN_POINT('Ctrl Pts',(8.95691518561776,-22.9853556730562,10.7682188220704));
#89913=CARTESIAN_POINT('Ctrl Pts',(8.93983387064254,-22.9950142631594,10.7580274751551));
#89914=CARTESIAN_POINT('Ctrl Pts',(8.92385304365272,-23.0038402727672,10.7490310140701));
#89915=CARTESIAN_POINT('Ctrl Pts',(8.91881256768606,-23.0066240642028,10.7461934609252));
#89916=CARTESIAN_POINT('Ctrl Pts',(8.91388163935561,-23.0093251472349,10.7434751434281));
#89917=CARTESIAN_POINT('Ctrl Pts',(8.90906530481319,-23.0119447843037,10.7408717490746));
#89918=CARTESIAN_POINT('Ctrl Pts',(8.89902204419398,-23.0174073819654,10.7354430215317));
#89919=CARTESIAN_POINT('Ctrl Pts',(8.88947488845928,-23.0225171138711,10.7305122434003));
#89920=CARTESIAN_POINT('Ctrl Pts',(8.88045886577374,-23.0272916226541,10.7260415210383));
#89921=CARTESIAN_POINT('Ctrl Pts',(8.87595085443097,-23.0296788770456,10.7238061598573));
#89922=CARTESIAN_POINT('Ctrl Pts',(8.87157553457791,-23.0319822448368,10.7216857056986));
#89923=CARTESIAN_POINT('Ctrl Pts',(8.86734037703127,-23.0342103559124,10.7196849617963));
#89924=CARTESIAN_POINT('Ctrl Pts',(8.86522279825795,-23.0353244114502,10.7186845898452));
#89925=CARTESIAN_POINT('Ctrl Pts',(8.86313980497631,-23.0364188696591,10.7177131043847));
#89926=CARTESIAN_POINT('Ctrl Pts',(8.86109074211417,-23.0374921538938,10.7167673462285));
#89927=CARTESIAN_POINT('Ctrl Pts',(8.8600662106831,-23.0380287960111,10.7162944671504));
#89928=CARTESIAN_POINT('Ctrl Pts',(8.85905016031001,-23.038560143269,10.7158280141272));
#89929=CARTESIAN_POINT('Ctrl Pts',(8.85804263220622,-23.0390862143151,10.7153678876521));
#89930=CARTESIAN_POINT('Ctrl Pts',(8.85753886815433,-23.0393492498382,10.7151378244146));
#89931=CARTESIAN_POINT('Ctrl Pts',(8.85737477662451,-23.0394348372563,10.7150631549235));
#89932=CARTESIAN_POINT('Ctrl Pts',(8.8570442017229,-23.039607264533,10.7149127131171));
#89933=CARTESIAN_POINT('Ctrl Pts',(8.8567136268213,-23.0397796918097,10.7147622713108));
#89934=CARTESIAN_POINT('Ctrl Pts',(8.85621672904443,-23.0400390597548,10.7145355866259));
#89935=CARTESIAN_POINT('Ctrl Pts',(8.85504565480858,-23.0406486176515,10.7140063890137));
#89936=CARTESIAN_POINT('Ctrl Pts',(8.8375081072783,-23.0497771171593,10.706081333545));
#89937=CARTESIAN_POINT('Ctrl Pts',(8.82035364600279,-23.0584559152379,10.6990667696001));
#89938=CARTESIAN_POINT('Ctrl Pts',(8.80361240503948,-23.0666866946299,10.6929251497074));
#89939=CARTESIAN_POINT('Ctrl Pts',(8.7814795534295,-23.0775682427372,10.6848055866458));
#89940=CARTESIAN_POINT('Ctrl Pts',(8.76006900585031,-23.0876660498215,10.6782137157404));
#89941=CARTESIAN_POINT('Ctrl Pts',(8.73951183134782,-23.0969407417162,10.6731237801854));
#89942=CARTESIAN_POINT('Ctrl Pts',(8.71985880705542,-23.1058075120541,10.6682577113053));
#89943=CARTESIAN_POINT('Ctrl Pts',(8.70098941074461,-23.113919168474,10.6647686786032));
#89944=CARTESIAN_POINT('Ctrl Pts',(8.68302914806466,-23.1212408406627,10.6626236735639));
#89945=CARTESIAN_POINT('Ctrl Pts',(8.66738338370802,-23.1276189855596,10.6607550904597));
#89946=CARTESIAN_POINT('Ctrl Pts',(8.6524284691694,-23.1333971706594,10.6599068060774));
#89947=CARTESIAN_POINT('Ctrl Pts',(8.63822807834273,-23.1385709426346,10.6600230757282));
#89948=CARTESIAN_POINT('Ctrl Pts',(8.62419824174967,-23.1436825748613,10.6601379489188));
#89949=CARTESIAN_POINT('Ctrl Pts',(8.6109053274306,-23.1482040959269,10.6611942792068));
#89950=CARTESIAN_POINT('Ctrl Pts',(8.59838126145788,-23.1521547389558,10.6631008777657));
#89951=CARTESIAN_POINT('Ctrl Pts',(8.58543739956392,-23.1562378041415,10.6650713838686));
#89952=CARTESIAN_POINT('Ctrl Pts',(8.57331497071912,-23.1597111696374,10.6679496544977));
#89953=CARTESIAN_POINT('Ctrl Pts',(8.56201267336647,-23.162621878775,10.6715985087102));
#89954=CARTESIAN_POINT('Ctrl Pts',(8.54945169004857,-23.1658567404831,10.6756537193866));
#89955=CARTESIAN_POINT('Ctrl Pts',(8.53790390195525,-23.1683968954813,10.6806597285344));
#89956=CARTESIAN_POINT('Ctrl Pts',(8.52731880357864,-23.1703362662535,10.6863944651257));
#89957=CARTESIAN_POINT('Ctrl Pts',(8.52394129456544,-23.1709550835786,10.6882243134499));
#89958=CARTESIAN_POINT('Ctrl Pts',(8.52066145345847,-23.1715129157972,10.6901281926098));
#89959=CARTESIAN_POINT('Ctrl Pts',(8.51747674491568,-23.1720132445407,10.6920985878117));
#89960=CARTESIAN_POINT('Origin',(6.6707290414,-22.8742356128,9.03420135995));
#89961=CARTESIAN_POINT('',(7.27479069254,-23.1742356128,9.59272830866));
#89962=CARTESIAN_POINT('',(7.70044916513,-22.8742356128,9.57771386935));
#89963=CARTESIAN_POINT('Origin',(7.16045579301E-17,-22.6642356128,0.580061096523));
#89964=CARTESIAN_POINT('',(10.0062431967,-21.0742356128,11.3317411468));
#89965=CARTESIAN_POINT('',(10.0062431967,-23.2742356128,11.3317411468));
#89966=CARTESIAN_POINT('',(10.9304145503,-21.0742356128,10.3907473403));
#89967=CARTESIAN_POINT('Origin',(-1.51003344041E-15,-21.0742356128,0.580061096523));
#89968=CARTESIAN_POINT('',(10.9304145503,-21.9742356128,10.3907473403));
#89969=CARTESIAN_POINT('Origin',(10.1862176145,-21.9742356128,9.72278707155));
#89970=CARTESIAN_POINT('',(11.1383462684,-21.0742356128,10.0284846777));
#89971=CARTESIAN_POINT('Origin',(10.1862176145,-21.0742356128,9.72278707155));
#89972=CARTESIAN_POINT('',(11.1383462684,-22.6642356128,10.0284846777));
#89973=CARTESIAN_POINT('Origin',(-2.84607155346,-22.6642356128,5.53854202767));
#89974=CARTESIAN_POINT('Origin',(-2.84607155346,-21.0742356128,5.53854202767));
#89975=CARTESIAN_POINT('Origin',(11.3733704264,-23.1237854196,7.73136642019));
#89976=CARTESIAN_POINT('',(11.669865565,-21.0742356128,7.77708985809));
#89977=CARTESIAN_POINT('Origin',(11.3733704264,-21.0742356128,7.73136642019));
#89978=CARTESIAN_POINT('',(11.669865565,-22.5742356128,7.77708985809));
#89979=CARTESIAN_POINT('Origin',(-2.84607155346,-21.2742356128,5.53854202767));
#89980=CARTESIAN_POINT('',(11.7512376696,-21.0742356128,3.91309124051));
#89981=CARTESIAN_POINT('Origin',(-2.84607155346,-21.0742356128,5.53854202767));
#89982=CARTESIAN_POINT('',(11.7512376696,-22.1242356128,3.91309124051));
#89983=CARTESIAN_POINT('Origin',(11.4530804658,-22.1242356128,3.94629187045));
#89984=CARTESIAN_POINT('',(11.4530804658,-21.0742356128,3.64629187045));
#89985=CARTESIAN_POINT('Origin',(11.4530804658,-21.0742356128,3.94629187045));
#89986=CARTESIAN_POINT('',(11.4530804658,-21.9742356128,3.64629187045));
#89987=CARTESIAN_POINT('Origin',(-11.7190551593,-23.1742356128,3.64629187045));
#89988=CARTESIAN_POINT('',(8.10176909975,-21.0742356128,3.64629187045));
#89989=CARTESIAN_POINT('',(-8.95225019493,-21.0742356128,3.64629187045));
#89990=CARTESIAN_POINT('',(8.10176909975,-22.1242356128,3.64629187045));
#89991=CARTESIAN_POINT('Origin',(8.10176909975,-22.1242356128,3.94629187045));
#89992=CARTESIAN_POINT('',(7.80346303227,-21.0742356128,3.91445651114));
#89993=CARTESIAN_POINT('Origin',(8.10176909975,-21.0742356128,3.94629187045));
#89994=CARTESIAN_POINT('',(7.80346303227,-21.2742356128,3.91445651114));
#89995=CARTESIAN_POINT('Origin',(0.00234331738835,-21.2742356128,3.08191746407));
#89996=CARTESIAN_POINT('',(6.23264645859,-21.0742356128,7.84992678029));
#89997=CARTESIAN_POINT('Origin',(0.00234331738835,-21.0742356128,3.08191746407));
#89998=CARTESIAN_POINT('',(6.23264645859,-22.1242356128,7.84992678029));
#89999=CARTESIAN_POINT('Origin',(6.47088626226,-22.1242356128,8.03225010833));
#90000=CARTESIAN_POINT('',(6.26721888507,-21.0742356128,8.25252175759));
#90001=CARTESIAN_POINT('Origin',(6.47088626226,-21.0742356128,8.03225010833));
#90002=CARTESIAN_POINT('',(6.26721888507,-21.9742356128,8.25252175759));
#90003=CARTESIAN_POINT('Origin',(9.80058174751,-23.1742356128,11.519536597));
#90004=CARTESIAN_POINT('',(9.59819339216,-21.0742356128,11.3324044552));
#90005=CARTESIAN_POINT('',(8.22276378328,-21.0742356128,10.0606559488));
#90006=CARTESIAN_POINT('',(9.59819339216,-23.2742356128,11.3324044552));
#90007=CARTESIAN_POINT('Origin',(9.80186076935,-23.2742356128,11.1121328059));
#90008=CARTESIAN_POINT('Origin',(9.80186076935,-21.0742356128,11.1121328059));
#90009=CARTESIAN_POINT('Origin',(9.80186076935,-21.0742356128,11.1121328059));
#90010=CARTESIAN_POINT('',(9.80186076935,-20.7742356128,11.1121328059));
#90011=CARTESIAN_POINT('Origin',(9.80186076935,-21.0742356128,11.1121328059));
#90012=CARTESIAN_POINT('Origin',(9.80186076935,-21.0742356128,11.1121328059));
#90013=CARTESIAN_POINT('Origin',(-1.51003344041E-15,-21.0742356128,0.580061096523));
#90014=CARTESIAN_POINT('',(10.7071554695,-20.7742356128,10.1903592597));
#90015=CARTESIAN_POINT('Origin',(1.14862552646E-15,-20.7742356128,0.580061096523));
#90016=CARTESIAN_POINT('Origin',(10.7071554695,-21.0742356128,10.1903592597));
#90017=CARTESIAN_POINT('Origin',(10.1862176145,-21.0742356128,9.72278707155));
#90018=CARTESIAN_POINT('',(10.8527076722,-20.7742356128,9.93677539585));
#90019=CARTESIAN_POINT('Origin',(10.1862176145,-20.7742356128,9.72278707155));
#90020=CARTESIAN_POINT('Origin',(10.8527076722,-21.0742356128,9.93677539585));
#90021=CARTESIAN_POINT('Origin',(10.8795671881,-21.0742356128,9.85222376962));
#90022=CARTESIAN_POINT('',(10.8795671881,-20.7742356128,9.85222376962));
#90023=CARTESIAN_POINT('Origin',(10.8795671881,-21.0742356128,9.85222376962));
#90024=CARTESIAN_POINT('Origin',(10.8795671881,-21.0742356128,9.85222376962));
#90025=CARTESIAN_POINT('Origin',(-2.84607155346,-21.0742356128,5.53854202767));
#90026=CARTESIAN_POINT('Origin',(-2.84607155346,-20.7742356128,5.53854202767));
#90027=CARTESIAN_POINT('Origin',(11.3733704264,-21.0742356128,7.73136642019));
#90028=CARTESIAN_POINT('',(11.3733704264,-20.7742356128,7.73136642019));
#90029=CARTESIAN_POINT('Origin',(11.3733704264,-21.0742356128,7.73136642019));
#90030=CARTESIAN_POINT('Origin',(11.3733704264,-21.0742356128,7.73136642019));
#90031=CARTESIAN_POINT('Origin',(-2.84607155346,-21.0742356128,5.53854202767));
#90032=CARTESIAN_POINT('',(11.4530804658,-20.7742356128,3.94629187045));
#90033=CARTESIAN_POINT('Origin',(-2.84607155346,-20.7742356128,5.53854202767));
#90034=CARTESIAN_POINT('Ctrl Pts',(11.7512376696703,-21.0742356128,3.91309124050216));
#90035=CARTESIAN_POINT('Ctrl Pts',(11.7512376696703,-21.061953784972,3.91309124050216));
#90036=CARTESIAN_POINT('Ctrl Pts',(11.7504944812795,-21.0498158353317,3.91319258196987));
#90037=CARTESIAN_POINT('Ctrl Pts',(11.7490326898121,-21.0377819506246,3.91337662775074));
#90038=CARTESIAN_POINT('Ctrl Pts',(11.7475741872629,-21.0257751412316,3.91356025944277));
#90039=CARTESIAN_POINT('Ctrl Pts',(11.7454001436074,-21.0138707693975,3.91382623933377));
#90040=CARTESIAN_POINT('Ctrl Pts',(11.7424843663441,-21.0020342015883,3.91416170558472));
#90041=CARTESIAN_POINT('Ctrl Pts',(11.7408977618661,-20.9955933970294,3.91434424773657));
#90042=CARTESIAN_POINT('Ctrl Pts',(11.7390906675882,-20.989172855015,3.91454746142827));
#90043=CARTESIAN_POINT('Ctrl Pts',(11.7370528663661,-20.9827694783049,3.91476994898516));
#90044=CARTESIAN_POINT('Ctrl Pts',(11.7331534939108,-20.9705164918538,3.91519568327249));
#90045=CARTESIAN_POINT('Ctrl Pts',(11.7284135628784,-20.9583285255006,3.9157030054636));
#90046=CARTESIAN_POINT('Ctrl Pts',(11.7227474029947,-20.9462470252009,3.91631409645459));
#90047=CARTESIAN_POINT('Ctrl Pts',(11.7214850798771,-20.9435554744087,3.91645023703317));
#90048=CARTESIAN_POINT('Ctrl Pts',(11.7201766628825,-20.9408693694333,3.91659154143874));
#90049=CARTESIAN_POINT('Ctrl Pts',(11.7188210035705,-20.9381894695388,3.91673827700573));
#90050=CARTESIAN_POINT('Ctrl Pts',(11.7151006159899,-20.930834917996,3.9171409690215));
#90051=CARTESIAN_POINT('Ctrl Pts',(11.711024953989,-20.9235274344412,3.91758468300204));
#90052=CARTESIAN_POINT('Ctrl Pts',(11.7065715477149,-20.9162925106405,3.91807400392752));
#90053=CARTESIAN_POINT('Ctrl Pts',(11.7046069350836,-20.9131008362658,3.91828986702461));
#90054=CARTESIAN_POINT('Ctrl Pts',(11.7024319865283,-20.9097091974042,3.91852987197131));
#90055=CARTESIAN_POINT('Ctrl Pts',(11.7002182775194,-20.9064091635286,3.91877487588534));
#90056=CARTESIAN_POINT('Ctrl Pts',(11.6979303480295,-20.9029984872422,3.91902809420708));
#90057=CARTESIAN_POINT('Ctrl Pts',(11.6956012072243,-20.8996859843533,3.91928663093016));
#90058=CARTESIAN_POINT('Ctrl Pts',(11.6934678401137,-20.8967605599251,3.91952405550537));
#90059=CARTESIAN_POINT('Ctrl Pts',(11.6929863050353,-20.8961002448419,3.91957764602941));
#90060=CARTESIAN_POINT('Ctrl Pts',(11.6925149133686,-20.8954595177209,3.91963014209845));
#90061=CARTESIAN_POINT('Ctrl Pts',(11.692056655695,-20.894841483953,3.91968121022605));
#90062=CARTESIAN_POINT('Ctrl Pts',(11.6868870171147,-20.8878693994812,3.92025731353614));
#90063=CARTESIAN_POINT('Ctrl Pts',(11.681028978478,-20.8806146987769,3.92079056445445));
#90064=CARTESIAN_POINT('Ctrl Pts',(11.6743536993568,-20.8731965252264,3.92136149180633));
#90065=CARTESIAN_POINT('Ctrl Pts',(11.6679298789804,-20.8660577953628,3.92191091224103));
#90066=CARTESIAN_POINT('Ctrl Pts',(11.6607485156396,-20.8587673526175,3.92249531322976));
#90067=CARTESIAN_POINT('Ctrl Pts',(11.6526950743861,-20.8514781481433,3.92318622219881));
#90068=CARTESIAN_POINT('Ctrl Pts',(11.6450908858519,-20.8445955642465,3.92383858954033));
#90069=CARTESIAN_POINT('Ctrl Pts',(11.6367084813275,-20.8377140858643,3.92458600237492));
#90070=CARTESIAN_POINT('Ctrl Pts',(11.6274618609907,-20.8310069727909,3.92548719456923));
#90071=CARTESIAN_POINT('Ctrl Pts',(11.6216163226962,-20.8267668629034,3.92605691121063));
#90072=CARTESIAN_POINT('Ctrl Pts',(11.6154256196503,-20.8225973359018,3.92668805493909));
#90073=CARTESIAN_POINT('Ctrl Pts',(11.6088725503865,-20.8185520694094,3.92739486347025));
#90074=CARTESIAN_POINT('Ctrl Pts',(11.5990462859797,-20.8124862311662,3.92845471607254));
#90075=CARTESIAN_POINT('Ctrl Pts',(11.5884024743053,-20.8066968351051,3.92972025328186));
#90076=CARTESIAN_POINT('Ctrl Pts',(11.5769335115456,-20.8014122888872,3.93113673006546));
#90077=CARTESIAN_POINT('Ctrl Pts',(11.5658173333816,-20.7962902949891,3.9325096361095));
#90078=CARTESIAN_POINT('Ctrl Pts',(11.5539255155658,-20.7916431888797,3.93402438121635));
#90079=CARTESIAN_POINT('Ctrl Pts',(11.5412952243341,-20.7876957303457,3.93562656642631));
#90080=CARTESIAN_POINT('Ctrl Pts',(11.5289826087367,-20.7838475578353,3.93718845365792));
#90081=CARTESIAN_POINT('Ctrl Pts',(11.515967870747,-20.7806649881655,3.93883346656174));
#90082=CARTESIAN_POINT('Ctrl Pts',(11.5023338717146,-20.7783628051133,3.94050629235595));
#90083=CARTESIAN_POINT('Ctrl Pts',(11.4891284616509,-20.7761329918961,3.9421265323549));
#90084=CARTESIAN_POINT('Ctrl Pts',(11.4753420359553,-20.7747298298989,3.94377286916209));
#90085=CARTESIAN_POINT('Ctrl Pts',(11.4610987246952,-20.7743441416219,3.94539013989711));
#90086=CARTESIAN_POINT('Ctrl Pts',(11.4584413983245,-20.7742721850655,3.94569186862397));
#90087=CARTESIAN_POINT('Ctrl Pts',(11.4557683109257,-20.7742356127993,3.94599257145532));
#90088=CARTESIAN_POINT('Ctrl Pts',(11.4530804658,-20.7742356128,3.94629187045));
#90089=CARTESIAN_POINT('Origin',(11.4530804658,-21.0742356128,3.94629187045));
#90090=CARTESIAN_POINT('Origin',(11.4530804658,-21.0742356128,3.94629187045));
#90091=CARTESIAN_POINT('Origin',(-8.95225019493,-21.0742356128,3.94629187045));
#90092=CARTESIAN_POINT('',(8.10176909975,-20.7742356128,3.94629187045));
#90093=CARTESIAN_POINT('',(9.77742478279,-20.7742356128,3.94629187045));
#90094=CARTESIAN_POINT('Ctrl Pts',(8.10176909975,-21.0742356128,3.64629187045));
#90095=CARTESIAN_POINT('Ctrl Pts',(8.10176909975,-21.0619847846212,3.64629187045));
#90096=CARTESIAN_POINT('Ctrl Pts',(8.10178777058952,-21.0498787025718,3.64703790633803));
#90097=CARTESIAN_POINT('Ctrl Pts',(8.10180917103989,-21.0378767553172,3.64850329867038));
#90098=CARTESIAN_POINT('Ctrl Pts',(8.1018305261806,-21.0259002189328,3.64996558843165));
#90099=CARTESIAN_POINT('Ctrl Pts',(8.10185459938597,-21.0140262212391,3.65214435902398));
#90100=CARTESIAN_POINT('Ctrl Pts',(8.1018655504668,-21.0022192441784,3.65506405129366));
#90101=CARTESIAN_POINT('Ctrl Pts',(8.10187153783563,-20.9957639245915,3.65666035715581));
#90102=CARTESIAN_POINT('Ctrl Pts',(8.10187360271116,-20.9893288232958,3.6584790192082));
#90103=CARTESIAN_POINT('Ctrl Pts',(8.10186915629961,-20.9829106437654,3.66053016897335));
#90104=CARTESIAN_POINT('Ctrl Pts',(8.10186068552984,-20.9706834982078,3.66443777339922));
#90105=CARTESIAN_POINT('Ctrl Pts',(8.101840116808,-20.9585199787489,3.6691862056774));
#90106=CARTESIAN_POINT('Ctrl Pts',(8.10182011974497,-20.9464605656251,3.6748631738841));
#90107=CARTESIAN_POINT('Ctrl Pts',(8.10181564929347,-20.9437646186569,3.67613229080285));
#90108=CARTESIAN_POINT('Ctrl Pts',(8.10181120741178,-20.9410740368944,3.67744793841355));
#90109=CARTESIAN_POINT('Ctrl Pts',(8.1018069356528,-20.9383895761731,3.67881130230953));
#90110=CARTESIAN_POINT('Ctrl Pts',(8.1017952456339,-20.9310433291839,3.68254225945719));
#90111=CARTESIAN_POINT('Ctrl Pts',(8.10178500679284,-20.9237432623569,3.68663004481532));
#90112=CARTESIAN_POINT('Ctrl Pts',(8.10177833444282,-20.9165146982158,3.69109760503107));
#90113=CARTESIAN_POINT('Ctrl Pts',(8.10177538111668,-20.9133151797057,3.69307504361027));
#90114=CARTESIAN_POINT('Ctrl Pts',(8.10177315721422,-20.9099165309174,3.69526371375841));
#90115=CARTESIAN_POINT('Ctrl Pts',(8.10177162915918,-20.9066099782108,3.69749145520004));
#90116=CARTESIAN_POINT('Ctrl Pts',(8.10177005043771,-20.9031937886207,3.69979306288564));
#90117=CARTESIAN_POINT('Ctrl Pts',(8.10176921447374,-20.8998762238456,3.70213617883799));
#90118=CARTESIAN_POINT('Ctrl Pts',(8.1017690842391,-20.8969455452457,3.70428312691668));
#90119=CARTESIAN_POINT('Ctrl Pts',(8.10176905573697,-20.8963041598008,3.70475299121658));
#90120=CARTESIAN_POINT('Ctrl Pts',(8.10176906103665,-20.8956811799168,3.70521329960476));
#90121=CARTESIAN_POINT('Ctrl Pts',(8.10176909975,-20.8950794308293,3.70566131864562));
#90122=CARTESIAN_POINT('Ctrl Pts',(8.10176954837301,-20.8881061653975,3.71085310996751));
#90123=CARTESIAN_POINT('Ctrl Pts',(8.10165103493539,-20.8808495135392,3.71672358548636));
#90124=CARTESIAN_POINT('Ctrl Pts',(8.10147915722924,-20.8734282573273,3.72340982543949));
#90125=CARTESIAN_POINT('Ctrl Pts',(8.10131375448263,-20.8662865739282,3.72984418203802));
#90126=CARTESIAN_POINT('Ctrl Pts',(8.10109893240106,-20.8589921286811,3.73703471542109));
#90127=CARTESIAN_POINT('Ctrl Pts',(8.10089315097308,-20.851697542693,3.74510338332156));
#90128=CARTESIAN_POINT('Ctrl Pts',(8.10069886081103,-20.8448103016647,3.75272147990688));
#90129=CARTESIAN_POINT('Ctrl Pts',(8.10051262979633,-20.8379229353717,3.76112310089669));
#90130=CARTESIAN_POINT('Ctrl Pts',(8.10038366104728,-20.8312084104219,3.77040048662393));
#90131=CARTESIAN_POINT('Ctrl Pts',(8.10030161028707,-20.8269365858078,3.77630281999828));
#90132=CARTESIAN_POINT('Ctrl Pts',(8.10024273692979,-20.822735620552,3.78255940771729));
#90133=CARTESIAN_POINT('Ctrl Pts',(8.10021971127824,-20.8186601819094,3.78918935893252));
#90134=CARTESIAN_POINT('Ctrl Pts',(8.10018536535161,-20.8125811045673,3.79907884316888));
#90135=CARTESIAN_POINT('Ctrl Pts',(8.10026502916778,-20.8067783917534,3.80980573572973));
#90136=CARTESIAN_POINT('Ctrl Pts',(8.10040384447576,-20.8014812562884,3.82137165189451));
#90137=CARTESIAN_POINT('Ctrl Pts',(8.10053823548761,-20.7963529501573,3.83256894129223));
#90138=CARTESIAN_POINT('Ctrl Pts',(8.10072806754702,-20.7916991304606,3.844553088688));
#90139=CARTESIAN_POINT('Ctrl Pts',(8.10092356229844,-20.7877445949121,3.85728121564088));
#90140=CARTESIAN_POINT('Ctrl Pts',(8.10111414163741,-20.7838894900292,3.86968931357396));
#90141=CARTESIAN_POINT('Ctrl Pts',(8.10131010248906,-20.7806996541778,3.88280478000332));
#90142=CARTESIAN_POINT('Ctrl Pts',(8.10146532767923,-20.7783899206235,3.89653921805234));
#90143=CARTESIAN_POINT('Ctrl Pts',(8.10161566583163,-20.7761529056471,3.90984124743561));
#90144=CARTESIAN_POINT('Ctrl Pts',(8.1017277929501,-20.7747421928388,3.9237239632078));
#90145=CARTESIAN_POINT('Ctrl Pts',(8.10175981195886,-20.7743486289048,3.93805798374527));
#90146=CARTESIAN_POINT('Ctrl Pts',(8.10176590746594,-20.7742737055441,3.94078677289168));
#90147=CARTESIAN_POINT('Ctrl Pts',(8.10176909975,-20.7742356128,3.94353176975334));
#90148=CARTESIAN_POINT('Ctrl Pts',(8.10176909975,-20.7742356128,3.94629187045));
#90149=CARTESIAN_POINT('Origin',(8.10176909975,-21.0742356128,3.94629187045));
#90150=CARTESIAN_POINT('Origin',(8.10176909975,-21.0742356128,3.94629187045));
#90151=CARTESIAN_POINT('Origin',(0.00234331738835,-21.0742356128,3.08191746407));
#90152=CARTESIAN_POINT('',(6.47088626226,-20.7742356128,8.03225010833));
#90153=CARTESIAN_POINT('Origin',(0.00234331738835,-20.7742356128,3.08191746407));
#90154=CARTESIAN_POINT('Ctrl Pts',(6.23264645858874,-21.0742356128,7.84992678028904));
#90155=CARTESIAN_POINT('Ctrl Pts',(6.23264645858874,-21.0620738653159,7.84992678028904));
#90156=CARTESIAN_POINT('Ctrl Pts',(6.23324197790072,-21.0500593540845,7.85035827840671));
#90157=CARTESIAN_POINT('Ctrl Pts',(6.23440148065616,-21.0381491830447,7.85121773708456));
#90158=CARTESIAN_POINT('Ctrl Pts',(6.23555896176804,-21.0262597779071,7.85207569725876));
#90159=CARTESIAN_POINT('Ctrl Pts',(6.23727859457928,-21.0144732053028,7.85336022155103));
#90160=CARTESIAN_POINT('Ctrl Pts',(6.23956950843529,-21.0027514162633,7.85509881860574));
#90161=CARTESIAN_POINT('Ctrl Pts',(6.24083883124489,-20.99625674421,7.85606212016877));
#90162=CARTESIAN_POINT('Ctrl Pts',(6.242284241646,-20.9897821389332,7.85716536211542));
#90163=CARTESIAN_POINT('Ctrl Pts',(6.24391239277648,-20.9833237084844,7.85841714394168));
#90164=CARTESIAN_POINT('Ctrl Pts',(6.24697603836402,-20.9711710639439,7.86077258613424));
#90165=CARTESIAN_POINT('Ctrl Pts',(6.25069157623758,-20.9590780258119,7.86364274042942));
#90166=CARTESIAN_POINT('Ctrl Pts',(6.25513679500523,-20.9470823057364,7.86707079100242));
#90167=CARTESIAN_POINT('Ctrl Pts',(6.25614018231608,-20.9443745979863,7.86784458024109));
#90168=CARTESIAN_POINT('Ctrl Pts',(6.25718085020712,-20.9416720126045,7.8686468730048));
#90169=CARTESIAN_POINT('Ctrl Pts',(6.25825986455158,-20.9389752940825,7.8694782961947));
#90170=CARTESIAN_POINT('Ctrl Pts',(6.26118950301342,-20.9316534170906,7.87173569839489));
#90171=CARTESIAN_POINT('Ctrl Pts',(6.26440152010394,-20.9243751453831,7.8742073792891));
#90172=CARTESIAN_POINT('Ctrl Pts',(6.26791574646482,-20.9171653086749,7.87690568653838));
#90173=CARTESIAN_POINT('Ctrl Pts',(6.26948675885108,-20.913942197353,7.87811194751171));
#90174=CARTESIAN_POINT('Ctrl Pts',(6.27122487389521,-20.9105224459337,7.87944512175967));
#90175=CARTESIAN_POINT('Ctrl Pts',(6.27299449129919,-20.9071962313223,7.88080146346944));
#90176=CARTESIAN_POINT('Ctrl Pts',(6.27482085484793,-20.9037633553189,7.88220129885351));
#90177=CARTESIAN_POINT('Ctrl Pts',(6.27668060789435,-20.9004304235927,7.88362568450306));
#90178=CARTESIAN_POINT('Ctrl Pts',(6.27838681422104,-20.8974837625284,7.88493158970018));
#90179=CARTESIAN_POINT('Ctrl Pts',(6.2787254732354,-20.8968988899277,7.88519079432273));
#90180=CARTESIAN_POINT('Ctrl Pts',(6.27905797805986,-20.8963291325229,7.88544525088481));
#90181=CARTESIAN_POINT('Ctrl Pts',(6.27938272573509,-20.8957765857997,7.88569373289182));
#90182=CARTESIAN_POINT('Ctrl Pts',(6.28348298362732,-20.8888001415159,7.888831061926));
#90183=CARTESIAN_POINT('Ctrl Pts',(6.28804763236961,-20.8815380508843,7.89247468318607));
#90184=CARTESIAN_POINT('Ctrl Pts',(6.29322559803938,-20.8741080370697,7.89665611919858));
#90185=CARTESIAN_POINT('Ctrl Pts',(6.29820836303392,-20.8669581223917,7.90067992204296));
#90186=CARTESIAN_POINT('Ctrl Pts',(6.30375962933618,-20.8596523763411,7.90520220172809));
#90187=CARTESIAN_POINT('Ctrl Pts',(6.31001241524958,-20.8523424382694,7.91025080344716));
#90188=CARTESIAN_POINT('Ctrl Pts',(6.31591479917088,-20.8454421442984,7.91501648486092));
#90189=CARTESIAN_POINT('Ctrl Pts',(6.32244284542141,-20.8385381115029,7.92025160452025));
#90190=CARTESIAN_POINT('Ctrl Pts',(6.32970078569121,-20.8318024119911,7.92597298656875));
#90191=CARTESIAN_POINT('Ctrl Pts',(6.33440503712393,-20.827436652161,7.92968131409671));
#90192=CARTESIAN_POINT('Ctrl Pts',(6.33941576294771,-20.8231425171236,7.933593787265));
#90193=CARTESIAN_POINT('Ctrl Pts',(6.34475758866928,-20.8189776690091,7.93771186558751));
#90194=CARTESIAN_POINT('Ctrl Pts',(6.35260440530219,-20.8128597607952,7.94376107182541));
#90195=CARTESIAN_POINT('Ctrl Pts',(6.36119100892562,-20.8070179672896,7.95023172960266));
#90196=CARTESIAN_POINT('Ctrl Pts',(6.37048584081494,-20.8016838718932,7.95716832362973));
#90197=CARTESIAN_POINT('Ctrl Pts',(6.37945335292896,-20.7965376179691,7.96386064380384));
#90198=CARTESIAN_POINT('Ctrl Pts',(6.38908045099127,-20.7918645698442,7.97098691526333));
#90199=CARTESIAN_POINT('Ctrl Pts',(6.39930314779427,-20.7878895669207,7.97856062207488));
#90200=CARTESIAN_POINT('Ctrl Pts',(6.4092689470059,-20.7840144562953,7.98594400072988));
#90201=CARTESIAN_POINT('Ctrl Pts',(6.41980105771033,-20.7808034552105,7.9937527988218));
#90202=CARTESIAN_POINT('Ctrl Pts',(6.43080104167877,-20.7784714692945,8.00197063081155));
#90203=CARTESIAN_POINT('Ctrl Pts',(6.44145351983779,-20.7762131542725,8.00992884929957));
#90204=CARTESIAN_POINT('Ctrl Pts',(6.45254484058177,-20.7747799372274,8.01827070709806));
#90205=CARTESIAN_POINT('Ctrl Pts',(6.46394607649882,-20.7743626945913,8.02695229170245));
#90206=CARTESIAN_POINT('Ctrl Pts',(6.46624740026132,-20.77427847474,8.02870465759433));
#90207=CARTESIAN_POINT('Ctrl Pts',(6.46856121725986,-20.7742356128,8.03047076694482));
#90208=CARTESIAN_POINT('Ctrl Pts',(6.47088626226,-20.7742356128,8.03225010833));
#90209=CARTESIAN_POINT('Origin',(6.47088626226,-21.0742356128,8.03225010833));
#90210=CARTESIAN_POINT('Origin',(6.47088626226,-21.0742356128,8.03225010833));
#90211=CARTESIAN_POINT('Origin',(8.42643116047,-21.0742356128,9.84038429957));
#90212=CARTESIAN_POINT('',(8.1363735158,-20.7742356128,9.57219145714));
#90213=CARTESIAN_POINT('Origin',(9.00617217252,-21.0742356128,8.1200469301));
#90214=CARTESIAN_POINT('',(10.5002881066,-20.7742356128,9.5015350813));
#90215=CARTESIAN_POINT('',(10.6899276473,-20.7742356128,9.67687942546));
#90216=CARTESIAN_POINT('Origin',(10.5002881066,-21.0742356128,9.5015350813));
#90217=CARTESIAN_POINT('Origin',(10.9076228609,-21.0742356128,9.06099178277));
#90218=CARTESIAN_POINT('',(10.4339531167,-20.7742356128,8.69270253038));
#90219=CARTESIAN_POINT('Origin',(10.9076228609,-20.7742356128,9.06099178277));
#90220=CARTESIAN_POINT('Origin',(10.4339531167,-21.0742356128,8.69270253038));
#90221=CARTESIAN_POINT('Origin',(-5.06274711921E-15,-21.0742356128,0.580061096523));
#90222=CARTESIAN_POINT('',(10.9433745451,-20.7742356128,7.99119341506));
#90223=CARTESIAN_POINT('Origin',(-1.97939039323E-16,-20.7742356128,0.580061096523));
#90224=CARTESIAN_POINT('Origin',(10.9433745451,-21.0742356128,7.99119341506));
#90225=CARTESIAN_POINT('Origin',(11.4401704731,-21.0742356128,8.32763628675));
#90226=CARTESIAN_POINT('Origin',(11.4401704731,-20.7742356128,8.32763628675));
#90227=CARTESIAN_POINT('Origin',(2.93915231795E-16,-20.7742356128,0.729452270839));
#90228=CARTESIAN_POINT('Origin',(-8.21591479143,-23.2742356128,11.6886688365));
#90229=CARTESIAN_POINT('',(-8.01224741424,-22.8742356128,11.9089404858));
#90230=CARTESIAN_POINT('',(-8.01224741424,-25.4742356128,11.9089404858));
#90231=CARTESIAN_POINT('',(-8.01224741424,-24.1742356128,11.9089404858));
#90232=CARTESIAN_POINT('',(-8.03752439844,-25.4742356128,11.4474700229));
#90233=CARTESIAN_POINT('Origin',(-8.21591479143,-25.4742356128,11.6886688365));
#90234=CARTESIAN_POINT('',(-8.03752439844,-23.4742356128,11.4474700229));
#90235=CARTESIAN_POINT('',(-8.03752439844,-22.6642356128,11.4474700229));
#90236=CARTESIAN_POINT('',(-7.99564314217,-23.4742356128,11.4850014593));
#90237=CARTESIAN_POINT('Origin',(-8.21591479143,-23.4742356128,11.6886688365));
#90238=CARTESIAN_POINT('Ctrl Pts',(-7.99564314217397,-23.4742356128,11.4850014593037));
#90239=CARTESIAN_POINT('Ctrl Pts',(-7.98401306350167,-23.4742356128,11.4975796966502));
#90240=CARTESIAN_POINT('Ctrl Pts',(-7.9733574518956,-23.4712114944548,11.5112709020565));
#90241=CARTESIAN_POINT('Ctrl Pts',(-7.9638973064836,-23.4651632577643,11.5259199892497));
#90242=CARTESIAN_POINT('Ctrl Pts',(-7.95801133283008,-23.4614001272563,
11.53503445182));
#90243=CARTESIAN_POINT('Ctrl Pts',(-7.95258786652577,-23.456466312469,11.544518764159));
#90244=CARTESIAN_POINT('Ctrl Pts',(-7.94767597957468,-23.4503618134027,
11.5543262155101));
#90245=CARTESIAN_POINT('Ctrl Pts',(-7.94127275672447,-23.4424038802702,
11.5671113828436));
#90246=CARTESIAN_POINT('Ctrl Pts',(-7.9357395366415,-23.4324564638547,11.5804463404673));
#90247=CARTESIAN_POINT('Ctrl Pts',(-7.93117367235329,-23.420519564156,11.5942098765918));
#90248=CARTESIAN_POINT('Ctrl Pts',(-7.92889074020919,-23.4145511143067,
11.601091644654));
#90249=CARTESIAN_POINT('Ctrl Pts',(-7.92684942663567,-23.4080852936365,
11.6080802486667));
#90250=CARTESIAN_POINT('Ctrl Pts',(-7.92506041898695,-23.4011221021457,
11.6151587417459));
#90251=CARTESIAN_POINT('Ctrl Pts',(-7.92416591516259,-23.3976405064002,
11.6186979882854));
#90252=CARTESIAN_POINT('Ctrl Pts',(-7.92333446790805,-23.3940345679496,
11.6222597024052));
#90253=CARTESIAN_POINT('Ctrl Pts',(-7.92256731255003,-23.3903042867937,
11.6258416398829));
#90254=CARTESIAN_POINT('Ctrl Pts',(-7.92214484180027,-23.3882500292561,
11.6278142048869));
#90255=CARTESIAN_POINT('Ctrl Pts',(-7.92165638884266,-23.385690596397,11.6302162286501));
#90256=CARTESIAN_POINT('Ctrl Pts',(-7.92124875102252,-23.3833982859291,
11.6323489942543));
#90257=CARTESIAN_POINT('Ctrl Pts',(-7.92091616827586,-23.3815280401522,
11.6340890708803));
#90258=CARTESIAN_POINT('Ctrl Pts',(-7.9206353184784,-23.3798356062595,11.635649439268));
#90259=CARTESIAN_POINT('Ctrl Pts',(-7.92045987171943,-23.3787404152106,
11.6366458567813));
#90260=CARTESIAN_POINT('Ctrl Pts',(-7.9179685496474,-23.3631888390565,11.6507948610625));
#90261=CARTESIAN_POINT('Ctrl Pts',(-7.91642902368058,-23.3454430882469,
11.665497956093));
#90262=CARTESIAN_POINT('Ctrl Pts',(-7.91602298477787,-23.325503162782,11.6806125158188));
#90263=CARTESIAN_POINT('Ctrl Pts',(-7.91591988682191,-23.3204401859498,
11.6844502766898));
#90264=CARTESIAN_POINT('Ctrl Pts',(-7.91588981140854,-23.3152357483491,
11.688314310615));
#90265=CARTESIAN_POINT('Ctrl Pts',(-7.91593559468154,-23.3098898499798,
11.6922017557107));
#90266=CARTESIAN_POINT('Ctrl Pts',(-7.91604864227584,-23.2966898118354,
11.7018005957939));
#90267=CARTESIAN_POINT('Ctrl Pts',(-7.91662445381236,-23.2826273017215,
11.7115427457266));
#90268=CARTESIAN_POINT('Ctrl Pts',(-7.91770341386166,-23.2677023196379,
11.7213792979579));
#90269=CARTESIAN_POINT('Ctrl Pts',(-7.91824289388631,-23.2602398285961,
11.7262975740736));
#90270=CARTESIAN_POINT('Ctrl Pts',(-7.91890812230629,-23.2525617195619,
11.731239455762));
#90271=CARTESIAN_POINT('Ctrl Pts',(-7.91970373737013,-23.2446679925353,
11.7361978955349));
#90272=CARTESIAN_POINT('Ctrl Pts',(-7.92010154490205,-23.240721129022,11.7386771154213));
#90273=CARTESIAN_POINT('Ctrl Pts',(-7.92053194513749,-23.2367203610106,
11.7411604752441));
#90274=CARTESIAN_POINT('Ctrl Pts',(-7.92099549064719,-23.2326656885011,
11.7436470687904));
#90275=CARTESIAN_POINT('Ctrl Pts',(-7.92122726340204,-23.2306383522464,
11.7448903655636));
#90276=CARTESIAN_POINT('Ctrl Pts',(-7.92146732225737,-23.2285975398671,
11.7461344708073));
#90277=CARTESIAN_POINT('Ctrl Pts',(-7.92171573426593,-23.2265432513633,
11.7473792679732));
#90278=CARTESIAN_POINT('Ctrl Pts',(-7.92193628450917,-23.2247193708197,
11.7484844493182));
#90279=CARTESIAN_POINT('Ctrl Pts',(-7.92226510694275,-23.2220783175044,
11.7500732961721));
#90280=CARTESIAN_POINT('Ctrl Pts',(-7.9224315764798,-23.2207683548869,11.7508588882968));
#90281=CARTESIAN_POINT('Ctrl Pts',(-7.92245260631457,-23.22060286937,11.7509581309143));
#90282=CARTESIAN_POINT('Ctrl Pts',(-7.92247097527054,-23.2204586265584,
11.7510445692356));
#90283=CARTESIAN_POINT('Ctrl Pts',(-7.92248609565397,-23.2203399574783,
11.7511156178036));
#90284=CARTESIAN_POINT('Ctrl Pts',(-7.92419557411386,-23.2069234831436,
11.7591482181149));
#90285=CARTESIAN_POINT('Ctrl Pts',(-7.92639661216216,-23.1916362840756,
11.7678836193289));
#90286=CARTESIAN_POINT('Ctrl Pts',(-7.92928545952422,-23.1744783602743,
11.7772330848807));
#90287=CARTESIAN_POINT('Ctrl Pts',(-7.93206140751313,-23.1579909872495,
11.7862171629034));
#90288=CARTESIAN_POINT('Ctrl Pts',(-7.93547326947577,-23.139776252284,11.7957687872142));
#90289=CARTESIAN_POINT('Ctrl Pts',(-7.93971042418088,-23.119834155378,11.8057634457376));
#90290=CARTESIAN_POINT('Ctrl Pts',(-7.94370007518413,-23.1010569304558,
11.8151742891409));
#90291=CARTESIAN_POINT('Ctrl Pts',(-7.94842224736297,-23.080748249551,11.8249780647689));
#90292=CARTESIAN_POINT('Ctrl Pts',(-7.95403716199756,-23.0589081126635,
11.835024933752));
#90293=CARTESIAN_POINT('Ctrl Pts',(-7.95946291660408,-23.0378037449151,
11.844733335253));
#90294=CARTESIAN_POINT('Ctrl Pts',(-7.96572310798611,-23.0152693690631,
11.8546688582846));
#90295=CARTESIAN_POINT('Ctrl Pts',(-7.9729525225692,-22.9913049851077,11.8646499034078));
#90296=CARTESIAN_POINT('Ctrl Pts',(-7.97983963799616,-22.9684752695698,
11.8741583648545));
#90297=CARTESIAN_POINT('Ctrl Pts',(-7.98760710476378,-22.9443477564508,
11.883707961496));
#90298=CARTESIAN_POINT('Ctrl Pts',(-7.99635127818823,-22.9189224457506,
11.893099420447));
#90299=CARTESIAN_POINT('Ctrl Pts',(-8.00132945383483,-22.9044474740876,
11.8984461044578));
#90300=CARTESIAN_POINT('Ctrl Pts',(-8.00662377160518,-22.8895518631041,
11.9037407582921));
#90301=CARTESIAN_POINT('Ctrl Pts',(-8.01224741425901,-22.8742356128,11.9089404857794));
#90302=CARTESIAN_POINT('Origin',(7.16045579301E-17,-22.6642356128,0.580061096523));
#90303=CARTESIAN_POINT('',(-8.73611663980898,-23.4697909663899,10.8942572011661));
#90304=CARTESIAN_POINT('',(-8.67864985337,-23.4742356128,10.942657873));
#90305=CARTESIAN_POINT('Origin',(-8.65818093366798,-22.8777633816448,10.9233631052074));
#90306=CARTESIAN_POINT('Origin',(-2.3120230745E-14,-23.4742356128,0.580061096523));
#90307=CARTESIAN_POINT('',(-8.73611663424,-25.4742356128,10.8942572059));
#90308=CARTESIAN_POINT('Origin',(1.5714690362E-14,-25.4742356128,0.580061096523));
#90309=CARTESIAN_POINT('',(-8.73611663424,-23.2742356128,10.8942572059));
#90310=CARTESIAN_POINT('Origin',(-8.93001206801,-23.2742356128,11.1231776304));
#90311=CARTESIAN_POINT('',(-9.1336794452,-25.4742356128,10.9029059811));
#90312=CARTESIAN_POINT('Origin',(-8.93001206801,-25.4742356128,11.1231776304));
#90313=CARTESIAN_POINT('',(-9.1336794452,-22.8742356128,10.9029059811));
#90314=CARTESIAN_POINT('',(-9.1336794452,-24.1742356128,10.9029059811));
#90315=CARTESIAN_POINT('Ctrl Pts',(-9.1336794452,-22.8742356128,10.9029059811));
#90316=CARTESIAN_POINT('Ctrl Pts',(-9.12940941048534,-22.8858810056524,
10.8989462223991));
#90317=CARTESIAN_POINT('Ctrl Pts',(-9.1250732717887,-22.8973540636349,10.8951670399834));
#90318=CARTESIAN_POINT('Ctrl Pts',(-9.12071717713756,-22.9085797926161,
10.8915793258319));
#90319=CARTESIAN_POINT('Ctrl Pts',(-9.11587741156969,-22.9210519496623,
10.8875932564721));
#90320=CARTESIAN_POINT('Ctrl Pts',(-9.11101276238942,-22.9332196957832,
10.8838431045504));
#90321=CARTESIAN_POINT('Ctrl Pts',(-9.10616236875762,-22.945041707572,10.8803242976032));
#90322=CARTESIAN_POINT('Ctrl Pts',(-9.10059797910354,-22.9586039635624,
10.8762875091572));
#90323=CARTESIAN_POINT('Ctrl Pts',(-9.09505210507099,-22.9717121890023,
10.8725546903098));
#90324=CARTESIAN_POINT('Ctrl Pts',(-9.08955784168385,-22.9843649123,10.8691025663662));
#90325=CARTESIAN_POINT('Ctrl Pts',(-9.08282324320706,-22.9998739996959,
10.8648711222191));
#90326=CARTESIAN_POINT('Ctrl Pts',(-9.07616602179342,-23.0146999042907,
10.8610606879207));
#90327=CARTESIAN_POINT('Ctrl Pts',(-9.06961407777495,-23.0289064212666,
10.8576164151034));
#90328=CARTESIAN_POINT('Ctrl Pts',(-9.06227588436141,-23.0448177552169,
10.8537588210777));
#90329=CARTESIAN_POINT('Ctrl Pts',(-9.05506908330778,-23.0599544556301,
10.850359635989));
#90330=CARTESIAN_POINT('Ctrl Pts',(-9.04800375660265,-23.0744480608874,
10.8473434006867));
#90331=CARTESIAN_POINT('Ctrl Pts',(-9.03773489471981,-23.0955133048292,
10.842959554756));
#90332=CARTESIAN_POINT('Ctrl Pts',(-9.0278615445671,-23.1149522563626,10.8394273586293));
#90333=CARTESIAN_POINT('Ctrl Pts',(-9.01851166005801,-23.1327720803782,
10.8365549291929));
#90334=CARTESIAN_POINT('Ctrl Pts',(-9.01554963574945,-23.1384173642164,
10.8356449494165));
#90335=CARTESIAN_POINT('Ctrl Pts',(-9.01263990783723,-23.1438998494754,
10.8348012685031));
#90336=CARTESIAN_POINT('Ctrl Pts',(-9.00978606355942,-23.1492187492881,
10.8340181186981));
#90337=CARTESIAN_POINT('Ctrl Pts',(-9.00385493895204,-23.1602729815769,
10.8323905039343));
#90338=CARTESIAN_POINT('Ctrl Pts',(-8.99816412150493,-23.1706234478825,
10.8310236012099));
#90339=CARTESIAN_POINT('Ctrl Pts',(-8.99273569023084,-23.1802701547496,
10.8298674484874));
#90340=CARTESIAN_POINT('Ctrl Pts',(-8.9900214745938,-23.1850935081831,10.8292893721262));
#90341=CARTESIAN_POINT('Ctrl Pts',(-8.98737294268441,-23.1897410872773,
10.8287640185669));
#90342=CARTESIAN_POINT('Ctrl Pts',(-8.98478347236165,-23.1942025419636,
10.8282841697181));
#90343=CARTESIAN_POINT('Ctrl Pts',(-8.98348873720026,-23.1964332693068,
10.8280442452937));
#90344=CARTESIAN_POINT('Ctrl Pts',(-8.98221073044467,-23.198619790564,10.8278160958339));
#90345=CARTESIAN_POINT('Ctrl Pts',(-8.98095114953504,-23.2007638642198,
10.8275992663868));
#90346=CARTESIAN_POINT('Ctrl Pts',(-8.98032135908022,-23.2018359010476,
10.8274908516632));
#90347=CARTESIAN_POINT('Ctrl Pts',(-8.97969617700721,-23.2028973291489,
10.8273852661301));
#90348=CARTESIAN_POINT('Ctrl Pts',(-8.97907565827039,-23.2039481859462,
10.8272824227911));
#90349=CARTESIAN_POINT('Ctrl Pts',(-8.97876539890198,-23.2044736143448,
10.8272310011215));
#90350=CARTESIAN_POINT('Ctrl Pts',(-8.97866475208692,-23.2046437660682,
10.8272145374228));
#90351=CARTESIAN_POINT('Ctrl Pts',(-8.9784612739697,-23.2049877805326,10.82718123946));
#90352=CARTESIAN_POINT('Ctrl Pts',(-8.9783587400747,-23.2051611315713,10.8271644604084));
#90353=CARTESIAN_POINT('Ctrl Pts',(-8.97823005958759,-23.2053786520945,
10.8271434289838));
#90354=CARTESIAN_POINT('Ctrl Pts',(-8.97803512506575,-23.20570783814,10.8271118119532));
#90355=CARTESIAN_POINT('Ctrl Pts',(-8.97793803853632,-23.2058717882213,
10.8270960651899));
#90356=CARTESIAN_POINT('Ctrl Pts',(-8.97782451443108,-23.206063436029,10.827077696863));
#90357=CARTESIAN_POINT('Ctrl Pts',(-8.97768956490296,-23.2062911099582,
10.8270559676401));
#90358=CARTESIAN_POINT('Ctrl Pts',(-8.97757894031321,-23.2064777451793,
10.8270381551556));
#90359=CARTESIAN_POINT('Ctrl Pts',(-8.97745391794019,-23.2066885894156,
10.8270180844363));
#90360=CARTESIAN_POINT('Ctrl Pts',(-8.97731173154554,-23.206928224683,10.8269953726106));
#90361=CARTESIAN_POINT('Ctrl Pts',(-8.97723087601023,-23.2070644953711,
10.8269824573325));
#90362=CARTESIAN_POINT('Ctrl Pts',(-8.97714435523225,-23.2072102659226,
10.8269686725624));
#90363=CARTESIAN_POINT('Ctrl Pts',(-8.97705970789074,-23.2073528287402,
10.8269552241012));
#90364=CARTESIAN_POINT('Ctrl Pts',(-8.96621708389224,-23.22561394598,10.8252325875136));
#90365=CARTESIAN_POINT('Ctrl Pts',(-8.95542760073463,-23.2429744055504,
10.8241158085228));
#90366=CARTESIAN_POINT('Ctrl Pts',(-8.94472278985177,-23.2594373001478,
10.8235685069978));
#90367=CARTESIAN_POINT('Ctrl Pts',(-8.93052828447575,-23.2812669848033,
10.8228427889515));
#90368=CARTESIAN_POINT('Ctrl Pts',(-8.91648221334131,-23.3015171376975,
10.8231198537275));
#90369=CARTESIAN_POINT('Ctrl Pts',(-8.9026880892877,-23.3201078063195,10.824346632956));
#90370=CARTESIAN_POINT('Ctrl Pts',(-8.8895824540684,-23.3377705821867,10.8255121814896));
#90371=CARTESIAN_POINT('Ctrl Pts',(-8.87670585544422,-23.3539298048985,
10.8275373802581));
#90372=CARTESIAN_POINT('Ctrl Pts',(-8.86415748997195,-23.3685165511626,
10.8303657063101));
#90373=CARTESIAN_POINT('Ctrl Pts',(-8.8532047363803,-23.3812484912618,10.8328343910478));
#90374=CARTESIAN_POINT('Ctrl Pts',(-8.84250263762646,-23.3927815156541,
10.8359149806679));
#90375=CARTESIAN_POINT('Ctrl Pts',(-8.8321114600471,-23.4031070884454,10.8395485817495));
#90376=CARTESIAN_POINT('Ctrl Pts',(-8.82183938576005,-23.413314309904,10.8431405346302));
#90377=CARTESIAN_POINT('Ctrl Pts',(-8.81187146444347,-23.4223413440303,
10.8472727389923));
#90378=CARTESIAN_POINT('Ctrl Pts',(-8.80225367273463,-23.430227052521,10.8518668482273));
#90379=CARTESIAN_POINT('Ctrl Pts',(-8.79231137006379,-23.4383788302848,
10.8566159658938));
#90380=CARTESIAN_POINT('Ctrl Pts',(-8.78274346738949,-23.4453111491342,
10.8618582840456));
#90381=CARTESIAN_POINT('Ctrl Pts',(-8.77358312485918,-23.4511185790067,
10.8674882887901));
#90382=CARTESIAN_POINT('Ctrl Pts',(-8.76340116713159,-23.4575736875654,
10.8737461847284));
#90383=CARTESIAN_POINT('Ctrl Pts',(-8.75372315170681,-23.4626395111084,
10.8804822534289));
#90384=CARTESIAN_POINT('Ctrl Pts',(-8.74456740587474,-23.4665045713782,
10.8875378283139));
#90385=CARTESIAN_POINT('Ctrl Pts',(-8.74169943618646,-23.4677152729311,
10.8897479349808));
#90386=CARTESIAN_POINT('Ctrl Pts',(-8.73888250639547,-23.4688085064365,
10.8919893551245));
#90387=CARTESIAN_POINT('Ctrl Pts',(-8.73611663424,-23.4697908757,10.8942572059));
#90388=CARTESIAN_POINT('Origin',(-10.806321674,-23.2742356128,10.0787147334));
#90389=CARTESIAN_POINT('',(-11.031648508,-22.9538972343,10.2767748704));
#90390=CARTESIAN_POINT('',(-11.0909930576,-22.9538972343,10.1733836478));
#90391=CARTESIAN_POINT('Ctrl Pts',(-11.0316485080236,-22.9538972342712,
10.2767748704012));
#90392=CARTESIAN_POINT('Ctrl Pts',(-11.0364414874478,-22.9576018392429,
10.2713220473568));
#90393=CARTESIAN_POINT('Ctrl Pts',(-11.0412887837959,-22.9605581903059,
10.2654028401508));
#90394=CARTESIAN_POINT('Ctrl Pts',(-11.050182860397,-22.9647393225438,10.2535848889028));
#90395=CARTESIAN_POINT('Ctrl Pts',(-11.0542446140175,-22.9661256456956,
10.247786383537));
#90396=CARTESIAN_POINT('Ctrl Pts',(-11.0610297049498,-22.9675767047451,
10.2373096114452));
#90397=CARTESIAN_POINT('Ctrl Pts',(-11.0638318077743,-22.9678862078995,
10.2327193905693));
#90398=CARTESIAN_POINT('Ctrl Pts',(-11.0665081104589,-22.9678862078995,
10.2280566842471));
#90399=CARTESIAN_POINT('Ctrl Pts',(-11.0692420535233,-22.9678862078995,
10.2232935557399));
#90400=CARTESIAN_POINT('Ctrl Pts',(-11.071844430281,-22.9675632436939,10.2184552280518));
#90401=CARTESIAN_POINT('Ctrl Pts',(-11.077589003477,-22.9660452016239,10.2070412179224));
#90402=CARTESIAN_POINT('Ctrl Pts',(-11.0806076488283,-22.9645897469489,
10.2004413153353));
#90403=CARTESIAN_POINT('Ctrl Pts',(-11.0862338558044,-22.9603378044189,
10.1869112738819));
#90404=CARTESIAN_POINT('Ctrl Pts',(-11.0887879815709,-22.9574629735521,
10.1800143570539));
#90405=CARTESIAN_POINT('Ctrl Pts',(-11.0909930576014,-22.9538972342539,
10.1733836478253));
#90406=CARTESIAN_POINT('',(-11.031648508,-25.4742356128,10.2767748704));
#90407=CARTESIAN_POINT('',(-11.031648508,-22.6642356128,10.2767748704));
#90408=CARTESIAN_POINT('',(-11.0909930576,-25.4742356128,10.1733836478));
#90409=CARTESIAN_POINT('Origin',(-10.806321674,-25.4742356128,10.0787147334));
#90410=CARTESIAN_POINT('',(-11.0909930576,-22.6642356128,10.1733836478));
#90411=CARTESIAN_POINT('Origin',(-10.8795671881,-23.2742356128,9.85222376962));
#90412=CARTESIAN_POINT('',(-11.1657658425,-21.0742356128,9.94217003248));
#90413=CARTESIAN_POINT('',(-11.0832345653,-21.0742356128,9.63195212036));
#90414=CARTESIAN_POINT('Ctrl Pts',(-11.1657658425273,-21.0742356128,9.94217003248857));
#90415=CARTESIAN_POINT('Ctrl Pts',(-11.1701441004766,-21.0742356127987,
9.92823891969006));
#90416=CARTESIAN_POINT('Ctrl Pts',(-11.1733712020923,-21.0741948386066,
9.91441315929395));
#90417=CARTESIAN_POINT('Ctrl Pts',(-11.1755965166384,-21.0741446195935,
9.90087185946038));
#90418=CARTESIAN_POINT('Ctrl Pts',(-11.1779157725236,-21.0740922805919,
9.88675891556742));
#90419=CARTESIAN_POINT('Ctrl Pts',(-11.1791476929329,-21.0740296825142,
9.87295501972334));
#90420=CARTESIAN_POINT('Ctrl Pts',(-11.1794763079321,-21.0739922922776,
9.85960752486672));
#90421=CARTESIAN_POINT('Ctrl Pts',(-11.179675594885,-21.0739696171522,9.85151300214193));
#90422=CARTESIAN_POINT('Ctrl Pts',(-11.1795428889997,-21.0739562128569,
9.84358524958266));
#90423=CARTESIAN_POINT('Ctrl Pts',(-11.1791199073328,-21.0739599897817,
9.83584792154246));
#90424=CARTESIAN_POINT('Ctrl Pts',(-11.1786092657732,-21.0739645494469,
9.82650708820039));
#90425=CARTESIAN_POINT('Ctrl Pts',(-11.1776611953628,-21.0739888517107,
9.81726250742656));
#90426=CARTESIAN_POINT('Ctrl Pts',(-11.1763323365263,-21.0740212860748,
9.80828692085334));
#90427=CARTESIAN_POINT('Ctrl Pts',(-11.1749746890983,-21.0740544231017,
9.7991168858652));
#90428=CARTESIAN_POINT('Ctrl Pts',(-11.1732200234797,-21.0740960483956,
9.79022835166622));
#90429=CARTESIAN_POINT('Ctrl Pts',(-11.1711809999612,-21.0741337803976,
9.78178667192448));
#90430=CARTESIAN_POINT('Ctrl Pts',(-11.1690077288837,-21.0741739966422,
9.77278919923085));
#90431=CARTESIAN_POINT('Ctrl Pts',(-11.1665121299432,-21.0742097900565,
9.76430006175474));
#90432=CARTESIAN_POINT('Ctrl Pts',(-11.1638809828609,-21.0742261689598,
9.75648628423073));
#90433=CARTESIAN_POINT('Ctrl Pts',(-11.1629285294711,-21.0742320979867,
9.75365776166727));
#90434=CARTESIAN_POINT('Ctrl Pts',(-11.1619587083146,-21.0742354829752,
9.75091738912241));
#90435=CARTESIAN_POINT('Ctrl Pts',(-11.1609814983982,-21.0742356128,9.74827192519493));
#90436=CARTESIAN_POINT('Ctrl Pts',(-11.1566371977885,-21.0742361899513,
9.73651120688754));
#90437=CARTESIAN_POINT('Ctrl Pts',(-11.1516844235512,-21.074236478527,9.72535793251623));
#90438=CARTESIAN_POINT('Ctrl Pts',(-11.146209343146,-21.074236586743,9.71473936631389));
#90439=CARTESIAN_POINT('Ctrl Pts',(-11.1406978489627,-21.0742366956787,
9.70405017793173));
#90440=CARTESIAN_POINT('Ctrl Pts',(-11.1346564614678,-21.0742366218476,
9.69390176377249));
#90441=CARTESIAN_POINT('Ctrl Pts',(-11.1281164027013,-21.074236475639,9.68422588891586));
#90442=CARTESIAN_POINT('Ctrl Pts',(-11.1214821824725,-21.0742363273254,
9.67441070422159));
#90443=CARTESIAN_POINT('Ctrl Pts',(-11.1143342358999,-21.0742361045353,
9.6650807888115));
#90444=CARTESIAN_POINT('Ctrl Pts',(-11.1066561229926,-21.0742359224949,
9.65618648834588));
#90445=CARTESIAN_POINT('Ctrl Pts',(-11.099345990661,-21.0742357491789,9.64771845535586));
#90446=CARTESIAN_POINT('Ctrl Pts',(-11.0915543979062,-21.0742356128004,
9.63964479662113));
#90447=CARTESIAN_POINT('Ctrl Pts',(-11.0832345652963,-21.0742356128,9.63195212036397));
#90448=CARTESIAN_POINT('',(-11.1657658425,-25.4742356128,9.94217003248));
#90449=CARTESIAN_POINT('',(-11.1657658425,-22.6642356128,9.94217003248));
#90450=CARTESIAN_POINT('',(-11.0832345653,-25.4742356128,9.63195212036));
#90451=CARTESIAN_POINT('Origin',(-10.8795671881,-25.4742356128,9.85222376962));
#90452=CARTESIAN_POINT('',(-11.0832345653,-23.2742356128,9.63195212036));
#90453=CARTESIAN_POINT('Origin',(-11.221722051,-23.1742356128,9.76000029674));
#90454=CARTESIAN_POINT('',(-10.7039554837,-21.0742356128,9.28126343203));
#90455=CARTESIAN_POINT('',(-9.20983954971,-21.0742356128,7.89977528084));
#90456=CARTESIAN_POINT('',(-10.7039554837,-25.4742356128,9.28126343203));
#90457=CARTESIAN_POINT('',(-11.080905232,-25.4742356128,9.62979837427));
#90458=CARTESIAN_POINT('',(-10.7039554837,-23.2742356128,9.28126343203));
#90459=CARTESIAN_POINT('Origin',(-10.9076228609,-23.2742356128,9.06099178277));
#90460=CARTESIAN_POINT('',(-10.6707879888,-25.4742356128,8.87684715658));
#90461=CARTESIAN_POINT('Origin',(-10.9076228609,-25.4742356128,9.06099178277));
#90462=CARTESIAN_POINT('',(-10.6707879888,-21.0742356128,8.87684715658));
#90463=CARTESIAN_POINT('',(-10.6707879888,-22.6642356128,8.87684715658));
#90464=CARTESIAN_POINT('Origin',(-10.9076228609,-21.0742356128,9.06099178277));
#90465=CARTESIAN_POINT('Origin',(7.16045579301E-17,-22.6642356128,0.580061096523));
#90466=CARTESIAN_POINT('',(-11.1917725091,-21.0742356128,8.1594148509));
#90467=CARTESIAN_POINT('Origin',(5.59539391719E-15,-21.0742356128,0.580061096523));
#90468=CARTESIAN_POINT('',(-11.1917725091,-25.4742356128,8.1594148509));
#90469=CARTESIAN_POINT('Origin',(-2.15888032654E-14,-25.4742356128,0.580061096523));
#90470=CARTESIAN_POINT('',(-11.1917725091,-23.2742356128,8.1594148509));
#90471=CARTESIAN_POINT('Origin',(-11.4401704731,-23.2742356128,8.32763628675));
#90472=CARTESIAN_POINT('',(-11.6438378503,-25.4742356128,8.10736463748));
#90473=CARTESIAN_POINT('Origin',(-11.4401704731,-25.4742356128,8.32763628675));
#90474=CARTESIAN_POINT('',(-11.6438378497605,-23.4645367153794,8.10736463698115));
#90475=CARTESIAN_POINT('',(-11.6438378503,-24.4693861731,8.10736463748));
#90476=CARTESIAN_POINT('',(-11.4067704324827,-22.8742356736,8.0295013564461));
#90477=CARTESIAN_POINT('Ctrl Pts',(-11.4067704237,-22.8742356736,8.02950135638));
#90478=CARTESIAN_POINT('Ctrl Pts',(-11.4067703651,-22.9402171391,8.02950137053));
#90479=CARTESIAN_POINT('Ctrl Pts',(-11.4114432261,-23.0062323557,8.02896986926));
#90480=CARTESIAN_POINT('Ctrl Pts',(-11.4203500465,-23.0707470797,8.02802946276));
#90481=CARTESIAN_POINT('Ctrl Pts',(-11.4529027709,-23.2147843626,8.02583184946));
#90482=CARTESIAN_POINT('Ctrl Pts',(-11.5102889752,-23.3423703627,8.03319245204));
#90483=CARTESIAN_POINT('Ctrl Pts',(-11.5554237252,-23.4131506081,8.04186749464));
#90484=CARTESIAN_POINT('Ctrl Pts',(-11.6054955414,-23.4487166343,8.07191260584));
#90485=CARTESIAN_POINT('Ctrl Pts',(-11.6438378503,-23.4645367334,8.10736463748));
#90486=CARTESIAN_POINT('',(-11.4067704497,-21.0742356128,8.02950135347));
#90487=CARTESIAN_POINT('',(-11.4067704497,-23.1237854196,8.02950135347));
#90488=CARTESIAN_POINT('Origin',(-11.4401704731,-21.0742356128,8.32763628675));
#90489=CARTESIAN_POINT('Origin',(-12.8942551175,-23.1742356128,9.2635243433));
#90490=CARTESIAN_POINT('',(-11.7384871149,-23.4742356128,8.19487915673));
#90491=CARTESIAN_POINT('',(-12.7478394324279,-23.4742356126688,9.12814559461005));
#90492=CARTESIAN_POINT('',(-6.46706166421,-23.4742356128,3.32081842676));
#90493=CARTESIAN_POINT('Origin',(-11.7384707086266,-22.6130235696614,8.19486399662491));
#90494=CARTESIAN_POINT('',(-12.7478394283,-25.4742356128,9.12814559847));
#90495=CARTESIAN_POINT('',(-12.1510854644,-25.4742356128,8.57637547707));
#90496=CARTESIAN_POINT('',(-12.7478394283,-22.5760378048,9.12814559847));
#90497=CARTESIAN_POINT('Origin',(-8.92072771219,-25.4742356128,12.3403523349));
#90498=CARTESIAN_POINT('',(-8.21591479143,-25.7742356128,11.6886688365));
#90499=CARTESIAN_POINT('',(-9.38771846805,-25.7742356128,12.7721409138));
#90500=CARTESIAN_POINT('',(-8.80181662974,-25.7742356128,12.2304048752));
#90501=CARTESIAN_POINT('Origin',(-8.21591479143,-25.4742356128,11.6886688365));
#90502=CARTESIAN_POINT('',(-9.18405109086,-25.4742356128,12.9924125631));
#90503=CARTESIAN_POINT('',(-8.59814925255,-25.4742356128,12.4506765244));
#90504=CARTESIAN_POINT('Origin',(-9.38771846803591,-25.4742356128,12.772140913833));
#90505=CARTESIAN_POINT('Origin',(-8.21591479143,-25.4742356128,11.6886688365));
#90506=CARTESIAN_POINT('Origin',(-8.21591479143,-25.4742356128,11.6886688365));
#90507=CARTESIAN_POINT('Origin',(1.5714690362E-14,-25.4742356128,0.580061096523));
#90508=CARTESIAN_POINT('',(-8.93001206801,-25.7742356128,11.1231776304));
#90509=CARTESIAN_POINT('Origin',(-8.93001206801,-25.4742356128,11.1231776304));
#90510=CARTESIAN_POINT('Origin',(-3.09260596606E-16,-25.7742356128,0.580061096523));
#90511=CARTESIAN_POINT('Origin',(-8.93001206801,-25.4742356128,11.1231776304));
#90512=CARTESIAN_POINT('Origin',(-8.93001206801,-25.4742356128,11.1231776304));
#90513=CARTESIAN_POINT('Origin',(-9.58357319026,-25.4742356128,11.7274727362));
#90514=CARTESIAN_POINT('',(-9.39452601497,-25.7742356128,11.5526761045));
#90515=CARTESIAN_POINT('',(-9.59819339216,-25.4742356128,11.3324044552));
#90516=CARTESIAN_POINT('Origin',(-9.39452601497,-25.4742356128,11.5526761045));
#90517=CARTESIAN_POINT('',(-9.36593641868,-25.4742356128,11.1176552182));
#90518=CARTESIAN_POINT('',(-9.16226904149,-25.7742356128,11.3379268674));
#90519=CARTESIAN_POINT('Origin',(-9.80186076935,-25.4742356128,11.1121328059));
#90520=CARTESIAN_POINT('',(-10.2106256241,-25.7742356128,11.5513494877));
#90521=CARTESIAN_POINT('',(-10.0062431967,-25.4742356128,11.3317411468));
#90522=CARTESIAN_POINT('Origin',(-10.2106256241,-25.4742356128,11.5513494877));
#90523=CARTESIAN_POINT('Origin',(-9.80186076935,-25.4742356128,11.1121328059));
#90524=CARTESIAN_POINT('Origin',(-9.80186076935,-25.7742356128,11.1121328059));
#90525=CARTESIAN_POINT('Origin',(-3.82523487143E-15,-25.4742356128,0.580061096523));
#90526=CARTESIAN_POINT('',(-11.256975342,-25.7742356128,10.4748350074));
#90527=CARTESIAN_POINT('Origin',(-11.256975342,-25.4742356128,10.4748350074));
#90528=CARTESIAN_POINT('Origin',(-2.72521192632E-16,-25.4742356128,0.580061096523));
#90529=CARTESIAN_POINT('Origin',(-1.47808545802E-15,-25.7742356128,0.580061096523));
#90530=CARTESIAN_POINT('Origin',(-10.806321674,-25.4742356128,10.0787147334));
#90531=CARTESIAN_POINT('',(-11.3756644412,-25.7742356128,10.2680525622));
#90532=CARTESIAN_POINT('Origin',(-11.3756644412,-25.4742356128,10.2680525622));
#90533=CARTESIAN_POINT('Origin',(-10.806321674,-25.7742356128,10.0787147334));
#90534=CARTESIAN_POINT('Origin',(2.84607155346,-25.4742356128,5.53854202767));
#90535=CARTESIAN_POINT('',(-11.4519644969,-25.7742356128,10.0321162953));
#90536=CARTESIAN_POINT('Origin',(-11.4519644969,-25.4742356128,10.0321162953));
#90537=CARTESIAN_POINT('Origin',(2.84607155346,-25.4742356128,5.53854202767));
#90538=CARTESIAN_POINT('Origin',(2.84607155346,-25.7742356128,5.53854202767));
#90539=CARTESIAN_POINT('Origin',(-10.8795671881,-25.4742356128,9.85222376962));
#90540=CARTESIAN_POINT('',(-11.2869019425,-25.7742356128,9.4116804711));
#90541=CARTESIAN_POINT('Origin',(-11.2869019425,-25.4742356128,9.4116804711));
#90542=CARTESIAN_POINT('Origin',(-10.8795671881,-25.7742356128,9.85222376962));
#90543=CARTESIAN_POINT('Origin',(-11.2845726092,-25.4742356128,9.409526725));
#90544=CARTESIAN_POINT('',(-10.9076228609,-25.7742356128,9.06099178277));
#90545=CARTESIAN_POINT('Origin',(-10.9076228609,-25.4742356128,9.06099178277));
#90546=CARTESIAN_POINT('',(-11.0972624017,-25.7742356128,9.23633612693));
#90547=CARTESIAN_POINT('Origin',(-10.9076228609,-25.4742356128,9.06099178277));
#90548=CARTESIAN_POINT('Origin',(-10.9076228609,-25.4742356128,9.06099178277));
#90549=CARTESIAN_POINT('Origin',(-2.15888032654E-14,-25.4742356128,0.580061096523));
#90550=CARTESIAN_POINT('',(-11.4401704731,-25.7742356128,8.32763628675));
#90551=CARTESIAN_POINT('Origin',(-11.4401704731,-25.4742356128,8.32763628675));
#90552=CARTESIAN_POINT('Origin',(-3.09260596606E-16,-25.7742356128,0.580061096523));
#90553=CARTESIAN_POINT('Origin',(-11.4401704731,-25.4742356128,8.32763628675));
#90554=CARTESIAN_POINT('Origin',(-11.4401704731,-25.4742356128,8.32763628675));
#90555=CARTESIAN_POINT('Origin',(-11.9474180872,-25.4742356128,8.79664712633));
#90556=CARTESIAN_POINT('',(-12.5441720511,-25.7742356128,9.34841724773));
#90557=CARTESIAN_POINT('',(-11.9921712621,-25.7742356128,8.83802676724));
#90558=CARTESIAN_POINT('Origin',(-12.5441720511046,-25.4742356128,9.34841724773267));
#90559=CARTESIAN_POINT('Origin',(-3.18408167778E-16,-25.7742356128,0.729452270839));
#90560=CARTESIAN_POINT('',(-12.1784264826,-25.7742356128,9.98548488886));
#90561=CARTESIAN_POINT('Origin',(-3.09260596606E-16,-25.7742356128,0.580061096523));
#90562=CARTESIAN_POINT('Origin',(-10.0415172382,-25.7742356128,8.33514586886));
#90563=CARTESIAN_POINT('Origin',(-3.39394702409,-23.1742356128,-9.39793292047));
#90564=CARTESIAN_POINT('',(-3.39394702409,-21.0742356128,-7.0794205347));
#90565=CARTESIAN_POINT('',(-3.39394702409,-21.0742356128,-7.27665075431));
#90566=CARTESIAN_POINT('',(-3.39394702409,-21.0742356128,-6.14889144395));
#90567=CARTESIAN_POINT('',(-3.39394702409,-22.8742356071,-7.27665075406));
#90568=CARTESIAN_POINT('',(-3.39394702409,-23.1223803511,-7.27665075431));
#90569=CARTESIAN_POINT('',(-3.39394702409,-23.4742356128,-7.94679080481));
#90570=CARTESIAN_POINT('Ctrl Pts',(-3.39394702409,-22.8742356071,-7.27665075406));
#90571=CARTESIAN_POINT('Ctrl Pts',(-3.39394702409,-22.8963796807801,-7.27665075202916));
#90572=CARTESIAN_POINT('Ctrl Pts',(-3.39394702409,-22.9185266226574,-7.27803164667852));
#90573=CARTESIAN_POINT('Ctrl Pts',(-3.39394702409019,-22.9404763729725,
-7.28076880448012));
#90574=CARTESIAN_POINT('Ctrl Pts',(-3.39394702409038,-22.9635612306701,
-7.28364751141022));
#90575=CARTESIAN_POINT('Ctrl Pts',(-3.39394702409077,-22.9864277437381,
-7.28802596271889));
#90576=CARTESIAN_POINT('Ctrl Pts',(-3.39394702409072,-23.0088766193784,
-7.29382800372885));
#90577=CARTESIAN_POINT('Ctrl Pts',(-3.3939470240907,-23.0181604618048,-7.29622746619418));
#90578=CARTESIAN_POINT('Ctrl Pts',(-3.39394702409061,-23.0273732778489,
-7.29886989897477));
#90579=CARTESIAN_POINT('Ctrl Pts',(-3.39394702409046,-23.0365026587174,
-7.30174800896343));
#90580=CARTESIAN_POINT('Ctrl Pts',(-3.39394702409007,-23.0599555275722,
-7.30914171255472));
#90581=CARTESIAN_POINT('Ctrl Pts',(-3.39394702409004,-23.0828466467018,
-7.31809082810804));
#90582=CARTESIAN_POINT('Ctrl Pts',(-3.39394702409001,-23.1049940708735,
-7.32844271008414));
#90583=CARTESIAN_POINT('Ctrl Pts',(-3.39394702408999,-23.1281264931002,
-7.33925498797506));
#90584=CARTESIAN_POINT('Ctrl Pts',(-3.39394702409,-23.1504472805791,-7.35159636510977));
#90585=CARTESIAN_POINT('Ctrl Pts',(-3.39394702409,-23.1717995438951,-7.36526779521605));
#90586=CARTESIAN_POINT('Ctrl Pts',(-3.39394702409,-23.1802621945299,-7.37068626233385));
#90587=CARTESIAN_POINT('Ctrl Pts',(-3.39394702409,-23.1885732730389,-7.37631349194848));
#90588=CARTESIAN_POINT('Ctrl Pts',(-3.39394702409,-23.1967252289902,-7.38213675751289));
#90589=CARTESIAN_POINT('Ctrl Pts',(-3.39394702409,-23.216964154042,-7.39659422465562));
#90590=CARTESIAN_POINT('Ctrl Pts',(-3.39394702409,-23.2362264780343,-7.41226456121671));
#90591=CARTESIAN_POINT('Ctrl Pts',(-3.39394702409,-23.2544248664386,-7.42895825046336));
#90592=CARTESIAN_POINT('Ctrl Pts',(-3.39394702409,-23.2663051018241,-7.43985619116538));
#90593=CARTESIAN_POINT('Ctrl Pts',(-3.39394702409,-23.2777329032204,-7.45119035077379));
#90594=CARTESIAN_POINT('Ctrl Pts',(-3.39394702409,-23.2886950564466,-7.46291290030111));
#90595=CARTESIAN_POINT('Ctrl Pts',(-3.39394702409,-23.3092436284265,-7.48488683624042));
#90596=CARTESIAN_POINT('Ctrl Pts',(-3.39394702407267,-23.3281539933134,
-7.5082252168758));
#90597=CARTESIAN_POINT('Ctrl Pts',(-3.39394702415533,-23.3453669419493,
-7.53263177580096));
#90598=CARTESIAN_POINT('Ctrl Pts',(-3.39394702418428,-23.351396654865,-7.54118141750917));
#90599=CARTESIAN_POINT('Ctrl Pts',(-3.39394702422707,-23.3572183823464,
-7.54986251226728));
#90600=CARTESIAN_POINT('Ctrl Pts',(-3.39394702429189,-23.3628304875723,
-7.55866347490331));
#90601=CARTESIAN_POINT('Ctrl Pts',(-3.39394702449706,-23.3805929863697,
-7.58651881295321));
#90602=CARTESIAN_POINT('Ctrl Pts',(-3.39394702467124,-23.3962633147006,
-7.61557726389403));
#90603=CARTESIAN_POINT('Ctrl Pts',(-3.39394702467555,-23.4098082144408,
-7.64551044052));
#90604=CARTESIAN_POINT('Ctrl Pts',(-3.39394702468063,-23.4257384366872,
-7.68071499465771));
#90605=CARTESIAN_POINT('Ctrl Pts',(-3.39394702450576,-23.4387297283905,
-7.71712955274666));
#90606=CARTESIAN_POINT('Ctrl Pts',(-3.3939470243646,-23.448763496914,-7.75428420736052));
#90607=CARTESIAN_POINT('Ctrl Pts',(-3.39394702420207,-23.4603148681498,
-7.79705848579653));
#90608=CARTESIAN_POINT('Ctrl Pts',(-3.39394702411207,-23.4679503272946,
-7.84081579026664));
#90609=CARTESIAN_POINT('Ctrl Pts',(-3.39394702409605,-23.4716451363039,
-7.88490127919122));
#90610=CARTESIAN_POINT('Ctrl Pts',(-3.39394702408857,-23.4733699118574,
-7.90548084727437));
#90611=CARTESIAN_POINT('Ctrl Pts',(-3.39394702409,-23.4742356128,-7.92613251437262));
#90612=CARTESIAN_POINT('Ctrl Pts',(-3.39394702409,-23.4742356128,-7.94679080481));
#90613=CARTESIAN_POINT('',(-3.39394703109999,-23.4742356128,-9.19678217153944));
#90614=CARTESIAN_POINT('',(-3.39394702409,-23.4742356128,3.39628270998));
#90615=CARTESIAN_POINT('',(-3.39394702409,-25.4742356128,-9.19678210318));
#90616=CARTESIAN_POINT('',(-3.39394702409,-23.2742356128,-9.19678210318));
#90617=CARTESIAN_POINT('',(-3.39394702409,-25.4742356128,-7.0794205347));
#90618=CARTESIAN_POINT('',(-3.39394702409,-25.4742356128,-8.58812386759));
#90619=CARTESIAN_POINT('',(-3.39394702409,-23.2742356128,-7.0794205347));
#90620=CARTESIAN_POINT('Origin',(-3.09394702409,-23.2742356128,-7.0794205347));
#90621=CARTESIAN_POINT('',(-2.96616998276,-25.4742356128,-6.8079927769));
#90622=CARTESIAN_POINT('Origin',(-3.09394702409,-25.4742356128,-7.0794205347));
#90623=CARTESIAN_POINT('',(-2.96616998276,-21.0742356128,-6.8079927769));
#90624=CARTESIAN_POINT('',(-2.96616998276,-22.6642356128,-6.8079927769));
#90625=CARTESIAN_POINT('Origin',(-3.09394702409,-21.0742356128,-7.0794205347));
#90626=CARTESIAN_POINT('Origin',(2.84607155346,-22.6642356128,5.53854202767));
#90627=CARTESIAN_POINT('',(-2.60391380109,-21.0742356128,-6.97212274247));
#90628=CARTESIAN_POINT('Origin',(2.84607155346,-21.0742356128,5.53854202767));
#90629=CARTESIAN_POINT('',(-2.60391380109,-25.4742356128,-6.97212274247));
#90630=CARTESIAN_POINT('Origin',(2.84607155346,-25.4742356128,5.53854202767));
#90631=CARTESIAN_POINT('',(-2.60391380109,-23.2742356128,-6.97212274247));
#90632=CARTESIAN_POINT('Origin',(-2.72372695744,-23.2742356128,-7.24715875387));
#90633=CARTESIAN_POINT('',(-2.42372695744,-25.4742356128,-7.24715875387));
#90634=CARTESIAN_POINT('Origin',(-2.72372695744,-25.4742356128,-7.24715875387));
#90635=CARTESIAN_POINT('',(-2.42372695744,-21.0742356128,-7.24715875387));
#90636=CARTESIAN_POINT('',(-2.42372695744,-23.2742356128,-7.24715875387));
#90637=CARTESIAN_POINT('Origin',(-2.72372695744,-21.0742356128,-7.24715875387));
#90638=CARTESIAN_POINT('Origin',(-2.42372695744,-23.1742356128,-8.1710440518));
#90639=CARTESIAN_POINT('',(-2.42372695744,-25.4742356128,-7.96338790087));
#90640=CARTESIAN_POINT('',(-2.42372695744,-25.4742356128,-8.58812386759));
#90641=CARTESIAN_POINT('',(-2.42372695744,-21.0742356128,-7.96338790087));
#90642=CARTESIAN_POINT('',(-2.42372695744,-23.2742356128,-7.96338790087));
#90643=CARTESIAN_POINT('',(-2.42372695744,-21.0742356128,-6.11170048962));
#90644=CARTESIAN_POINT('Origin',(-2.12372695744,-23.2742356128,-7.96338790087));
#90645=CARTESIAN_POINT('',(-2.22735416732,-21.0742356128,-8.24492191546));
#90646=CARTESIAN_POINT('Origin',(-2.12372695744,-21.0742356128,-7.96338790087));
#90647=CARTESIAN_POINT('',(-2.22735416732,-25.4742356128,-8.24492191546));
#90648=CARTESIAN_POINT('Origin',(-2.12372695744,-25.4742356128,-7.96338790087));
#90649=CARTESIAN_POINT('',(-2.22735416732,-22.6642356128,-8.24492191546));
#90650=CARTESIAN_POINT('Origin',(-3.09394702409,-23.2742356128,-9.19678210318));
#90651=CARTESIAN_POINT('',(-3.20611083607784,-23.4742356128,-9.47502535777846));
#90652=CARTESIAN_POINT('',(-3.20611081633,-25.4742356128,-9.47502531282));
#90653=CARTESIAN_POINT('',(-3.20611081633,-20.0742356128,-9.47502531282));
#90654=CARTESIAN_POINT('Origin',(-3.09394702409,-25.4742356128,-9.19678210318));
#90655=CARTESIAN_POINT('Origin',(-3.09394702409079,-23.474235151356,-9.19678210318053));
#90656=CARTESIAN_POINT('Origin',(-3.09394702409,-25.4742356128,-8.58812386759));
#90657=CARTESIAN_POINT('',(-3.09394702409,-25.7742356128,-7.0794205347));
#90658=CARTESIAN_POINT('Origin',(-3.09394702409,-25.4742356128,-7.0794205347));
#90659=CARTESIAN_POINT('',(-3.09394702409,-25.7742356128,-9.19678210318));
#90660=CARTESIAN_POINT('Origin',(-3.09394702409,-25.4742356128,-9.19678210318));
#90661=CARTESIAN_POINT('',(-3.09394702409,-25.7742356128,-8.13810131894));
#90662=CARTESIAN_POINT('Origin',(-3.09394702409,-25.4742356128,-7.0794205347));
#90663=CARTESIAN_POINT('Origin',(-3.09394702409,-25.4742356128,-7.0794205347));
#90664=CARTESIAN_POINT('Origin',(2.84607155346,-25.4742356128,5.53854202767));
#90665=CARTESIAN_POINT('',(-2.72372695744,-25.7742356128,-7.24715875387));
#90666=CARTESIAN_POINT('Origin',(-2.72372695744,-25.4742356128,-7.24715875387));
#90667=CARTESIAN_POINT('Origin',(2.84607155346,-25.7742356128,5.53854202767));
#90668=CARTESIAN_POINT('Origin',(-2.72372695744,-25.4742356128,-7.24715875387));
#90669=CARTESIAN_POINT('Origin',(-2.72372695744,-25.4742356128,-7.24715875387));
#90670=CARTESIAN_POINT('Origin',(-2.72372695744,-25.4742356128,-8.58812386759));
#90671=CARTESIAN_POINT('',(-2.72372695744,-25.7742356128,-7.96338790087));
#90672=CARTESIAN_POINT('Origin',(-2.72372695744,-25.4742356128,-7.96338790087));
#90673=CARTESIAN_POINT('',(-2.72372695744,-25.7742356128,-7.60527332737));
#90674=CARTESIAN_POINT('Origin',(-2.12372695744,-25.4742356128,-7.96338790087));
#90675=CARTESIAN_POINT('',(-2.3309813772,-25.7742356128,-8.52645593005));
#90676=CARTESIAN_POINT('Origin',(-2.3309813772,-25.4742356128,-8.52645593005));
#90677=CARTESIAN_POINT('Origin',(-2.12372695744,-25.7742356128,-7.96338790087));
#90678=CARTESIAN_POINT('Ctrl Pts',(2.72048009119833E-16,-25.7742356128,
-9.1762777575));
#90679=CARTESIAN_POINT('Ctrl Pts',(2.72048009119833E-16,-25.7742356128,
-9.1762777575));
#90680=CARTESIAN_POINT('Ctrl Pts',(2.72048009119833E-16,-25.7742356128,
-9.1762777575));
#90681=CARTESIAN_POINT('Ctrl Pts',(2.72048009119833E-16,-25.7742356128,
-9.1762777575));
#90682=CARTESIAN_POINT('Ctrl Pts',(2.72048009119833E-16,-25.7742356128,
-9.1762777575));
#90683=CARTESIAN_POINT('Ctrl Pts',(2.72048009119833E-16,-25.7742356128,
-9.1762777575));
#90684=CARTESIAN_POINT('Ctrl Pts',(-0.0543179010659,-25.7751862689,-9.07845703679));
#90685=CARTESIAN_POINT('Ctrl Pts',(-0.0326006378767,-25.7751848901861,-9.0785989038544));
#90686=CARTESIAN_POINT('Ctrl Pts',(-0.0108684102149,-25.7751842248025,-9.07866737056662));
#90687=CARTESIAN_POINT('Ctrl Pts',(0.0108684102491,-25.7751842248025,-9.07866737056662));
#90688=CARTESIAN_POINT('Ctrl Pts',(0.0326006378991,-25.775184890186,-9.0785989038644));
#90689=CARTESIAN_POINT('Ctrl Pts',(0.0543179010637,-25.7751862689,-9.07845703679));
#90690=CARTESIAN_POINT('Ctrl Pts',(-0.109343357829,-25.7400248661,-8.98386898437));
#90691=CARTESIAN_POINT('Ctrl Pts',(-0.0655774722522,-25.7385135131,-8.98345841906));
#90692=CARTESIAN_POINT('Ctrl Pts',(-0.0218550902065,-25.7377882247,-8.98326842912));
#90693=CARTESIAN_POINT('Ctrl Pts',(0.0218550900655,-25.7377882247,-8.98326842912));
#90694=CARTESIAN_POINT('Ctrl Pts',(0.0655774721579,-25.7385135131,-8.98345841906));
#90695=CARTESIAN_POINT('Ctrl Pts',(0.109343357832,-25.7400248661,-8.98386898437));
#90696=CARTESIAN_POINT('Ctrl Pts',(-0.163251797833,-25.6940006666,-8.89703057892));
#90697=CARTESIAN_POINT('Ctrl Pts',(-0.098232070722,-25.681892459,-8.90144092994));
#90698=CARTESIAN_POINT('Ctrl Pts',(-0.0327886103307,-25.6757886735,-8.90359473304));
#90699=CARTESIAN_POINT('Ctrl Pts',(0.0327886095603,-25.6757886735,-8.90359473304));
#90700=CARTESIAN_POINT('Ctrl Pts',(0.0982320702102,-25.681892459,-8.90144092994));
#90701=CARTESIAN_POINT('Ctrl Pts',(0.16325179783,-25.6940006666,-8.89703057892));
#90702=CARTESIAN_POINT('Ctrl Pts',(-0.208904902042,-25.586489454,-8.82655958228));
#90703=CARTESIAN_POINT('Ctrl Pts',(-0.126605010039,-25.5795174219,-8.84455225061));
#90704=CARTESIAN_POINT('Ctrl Pts',(-0.0424177258938,-25.5759707943,-8.85368477148));
#90705=CARTESIAN_POINT('Ctrl Pts',(0.0424177261375,-25.5759707943,-8.85368477148));
#90706=CARTESIAN_POINT('Ctrl Pts',(0.126605010201,-25.5795174219,-8.84455225061));
#90707=CARTESIAN_POINT('Ctrl Pts',(0.208904902043,-25.586489454,-8.82655958228));
#90708=CARTESIAN_POINT('Ctrl Pts',(-0.20793136194,-25.4742356094,-8.82796730262));
#90709=CARTESIAN_POINT('Ctrl Pts',(-0.125978740127,-25.4742355994,-8.84538857459));
#90710=CARTESIAN_POINT('Ctrl Pts',(-0.042201592792,-25.4742355944,-8.85422697274));
#90711=CARTESIAN_POINT('Ctrl Pts',(0.042201592792,-25.4742355944,-8.85422697274));
#90712=CARTESIAN_POINT('Ctrl Pts',(0.125978740127,-25.4742355994,-8.84538857459));
#90713=CARTESIAN_POINT('Ctrl Pts',(0.20793136194,-25.4742356094,-8.82796730262));
#90714=CARTESIAN_POINT('',(-0.207931539813729,-25.4742356124822,-8.8279673345371));
#90715=CARTESIAN_POINT('Origin',(1.53982046821E-14,-25.4742356128,-7.84982397628));
#90716=CARTESIAN_POINT('Ctrl Pts',(-4.87606379654255E-15,-25.7742356128,
-9.17627775749999));
#90717=CARTESIAN_POINT('Ctrl Pts',(-0.00568547427394062,-25.7743351183165,
-9.16603882742094));
#90718=CARTESIAN_POINT('Ctrl Pts',(-0.011368426530604,-25.7739612468302,
-9.15579871367803));
#90719=CARTESIAN_POINT('Ctrl Pts',(-0.0170703292688694,-25.7731573020962,
-9.14559137800037));
#90720=CARTESIAN_POINT('Ctrl Pts',(-0.0226364418683845,-25.7723725032108,
-9.13562712881359));
#90721=CARTESIAN_POINT('Ctrl Pts',(-0.0282205239040065,-25.7711779079194,
-9.12569413414896));
#90722=CARTESIAN_POINT('Ctrl Pts',(-0.0337959481892083,-25.7696026140516,
-9.11582586073));
#90723=CARTESIAN_POINT('Ctrl Pts',(-0.0394393811271053,-25.7680081048545,
-9.10583721477161));
#90724=CARTESIAN_POINT('Ctrl Pts',(-0.0450930084467941,-25.7660239966216,
-9.09591552325664));
#90725=CARTESIAN_POINT('Ctrl Pts',(-0.0507631920877221,-25.7636711985576,
-9.08609020857896));
#90726=CARTESIAN_POINT('Ctrl Pts',(-0.0534551785308526,-25.7625541799753,
-9.08142552475446));
#90727=CARTESIAN_POINT('Ctrl Pts',(-0.056005605584535,-25.7614179275892,
-9.07703139117622));
#90728=CARTESIAN_POINT('Ctrl Pts',(-0.0586150679449305,-25.7601797386401,
-9.0725547076834));
#90729=CARTESIAN_POINT('Ctrl Pts',(-0.0611360075911444,-25.7589835536869,
-9.06822989002293));
#90730=CARTESIAN_POINT('Ctrl Pts',(-0.0637121682055152,-25.7576922631742,
-9.06382781887072));
#90731=CARTESIAN_POINT('Ctrl Pts',(-0.0665212281533235,-25.7561855928279,
-9.05904218763215));
#90732=CARTESIAN_POINT('Ctrl Pts',(-0.0669290135226217,-25.7559668726386,
-9.05834746753425));
#90733=CARTESIAN_POINT('Ctrl Pts',(-0.0673416988396855,-25.7557435281346,
-9.05764469015058));
#90734=CARTESIAN_POINT('Ctrl Pts',(-0.0677598182107501,-25.7555150997744,
-9.05693294696415));
#90735=CARTESIAN_POINT('Ctrl Pts',(-0.075841245909943,-25.7511000274162,
-9.04317634657783));
#90736=CARTESIAN_POINT('Ctrl Pts',(-0.083598223070189,-25.7460632812599,
-9.03005200253529));
#90737=CARTESIAN_POINT('Ctrl Pts',(-0.0909902917209981,-25.7405256146399,
-9.01760109199645));
#90738=CARTESIAN_POINT('Ctrl Pts',(-0.0950863809707422,-25.7374570856824,
-9.01070179990153));
#90739=CARTESIAN_POINT('Ctrl Pts',(-0.0990713564419826,-25.7342344321942,
-9.00400917533817));
#90740=CARTESIAN_POINT('Ctrl Pts',(-0.102944990399136,-25.7308778204123,
-8.99752866965076));
#90741=CARTESIAN_POINT('Ctrl Pts',(-0.108377113069743,-25.7261707347252,
-8.98844084611067));
#90742=CARTESIAN_POINT('Ctrl Pts',(-0.113590978844581,-25.7211999701095,
-8.97976991046837));
#90743=CARTESIAN_POINT('Ctrl Pts',(-0.118573216099615,-25.7160195091,-8.97152442357315));
#90744=CARTESIAN_POINT('Ctrl Pts',(-0.121064334727132,-25.7134292785952,
-8.96740168012554));
#90745=CARTESIAN_POINT('Ctrl Pts',(-0.123497555221235,-25.7107867120833,
-8.96338529594356));
#90746=CARTESIAN_POINT('Ctrl Pts',(-0.125871825980486,-25.7080985186622,
-8.9594754157065));
#90747=CARTESIAN_POINT('Ctrl Pts',(-0.127058961360111,-25.7067544219517,
-8.95752047558797));
#90748=CARTESIAN_POINT('Ctrl Pts',(-0.128010959055845,-25.7056534598856,
-8.95595469215668));
#90749=CARTESIAN_POINT('Ctrl Pts',(-0.1290598601512,-25.7044204435857,-8.95423111088934));
#90750=CARTESIAN_POINT('Ctrl Pts',(-0.130001663376611,-25.7033133242079,
-8.95268351559744));
#90751=CARTESIAN_POINT('Ctrl Pts',(-0.131021744978592,-25.7020999937992,
-8.95100844782097));
#90752=CARTESIAN_POINT('Ctrl Pts',(-0.132351089285718,-25.700475004152,
-8.94882886846802));
#90753=CARTESIAN_POINT('Ctrl Pts',(-0.132502256684463,-25.7002902172186,
-8.94858101594451));
#90754=CARTESIAN_POINT('Ctrl Pts',(-0.132657409241681,-25.7001000597447,
-8.94832666705564));
#90755=CARTESIAN_POINT('Ctrl Pts',(-0.132816874301156,-25.6999040417534,
-8.94806529151949));
#90756=CARTESIAN_POINT('Ctrl Pts',(-0.142818422392116,-25.687609916797,
-8.93167198251981));
#90757=CARTESIAN_POINT('Ctrl Pts',(-0.151863061499928,-25.6742515575359,
-8.91697497315247));
#90758=CARTESIAN_POINT('Ctrl Pts',(-0.159899286686074,-25.6601365363902,
-8.90397985664614));
#90759=CARTESIAN_POINT('Ctrl Pts',(-0.168778192586148,-25.6445414103669,
-8.88962206876096));
#90760=CARTESIAN_POINT('Ctrl Pts',(-0.176426109948507,-25.6280246493504,
-8.87734215821455));
#90761=CARTESIAN_POINT('Ctrl Pts',(-0.182828262798463,-25.6110143627422,
-8.86711124483626));
#90762=CARTESIAN_POINT('Ctrl Pts',(-0.189130157638363,-25.5942704580099,
-8.85704054803518));
#90763=CARTESIAN_POINT('Ctrl Pts',(-0.194226910336029,-25.5770510543607,
-8.8489534320159));
#90764=CARTESIAN_POINT('Ctrl Pts',(-0.198138215714044,-25.5597363439882,
-8.84280068827599));
#90765=CARTESIAN_POINT('Ctrl Pts',(-0.201688146798981,-25.5440213786154,
-8.83721641035621));
#90766=CARTESIAN_POINT('Ctrl Pts',(-0.204263213458548,-25.5282278823503,
-8.83322384006026));
#90767=CARTESIAN_POINT('Ctrl Pts',(-0.205880845811087,-25.5126006491252,
-8.83079326747201));
#90768=CARTESIAN_POINT('Ctrl Pts',(-0.207220444982422,-25.4996593719272,
-8.82878045348497));
#90769=CARTESIAN_POINT('Ctrl Pts',(-0.207903911128972,-25.4868311126593,
-8.82783840536747));
#90770=CARTESIAN_POINT('Ctrl Pts',(-0.207931361961233,-25.4742356118482,
-8.8279673025893));
#90771=CARTESIAN_POINT('Origin',(2.84607155346,-25.4742356128,5.53854202767));
#90772=CARTESIAN_POINT('Origin',(2.84607155346,-25.4742356128,5.53854202767));
#90773=CARTESIAN_POINT('Origin',(2.84607155346,-25.7742356128,5.53854202767));
#90774=CARTESIAN_POINT('Origin',(-3.09394702409,-25.4742356128,-9.19678210318));
#90775=CARTESIAN_POINT('Origin',(-3.09394702409,-25.4742356128,-9.19678210318));
#90776=CARTESIAN_POINT('Ctrl Pts',(-0.647446102181,-25.4742356128,-10.2675153591));
#90777=CARTESIAN_POINT('Ctrl Pts',(-0.392565377877,-25.4742356128,-10.3238501103));
#90778=CARTESIAN_POINT('Ctrl Pts',(-0.131557494527,-25.4742356128,-10.3524631675));
#90779=CARTESIAN_POINT('Ctrl Pts',(0.131557494527,-25.4742356128,-10.3524631675));
#90780=CARTESIAN_POINT('Ctrl Pts',(0.392565377877,-25.4742356128,-10.3238501103));
#90781=CARTESIAN_POINT('Ctrl Pts',(0.647446102181,-25.4742356128,-10.2675153591));
#90782=CARTESIAN_POINT('Ctrl Pts',(-0.647446102181,-25.5155830458,-10.2675153591));
#90783=CARTESIAN_POINT('Ctrl Pts',(-0.392565377877,-25.5235347589,-10.3238501103));
#90784=CARTESIAN_POINT('Ctrl Pts',(-0.131557494811,-25.5275737357,-10.3524631688));
#90785=CARTESIAN_POINT('Ctrl Pts',(0.131557494823,-25.5275737357,-10.3524631688));
#90786=CARTESIAN_POINT('Ctrl Pts',(0.392565377877,-25.5235347589,-10.3238501103));
#90787=CARTESIAN_POINT('Ctrl Pts',(0.647446102181,-25.5155830458,-10.2675153591));
#90788=CARTESIAN_POINT('Ctrl Pts',(-0.627595169723,-25.5568342995,-10.2641149764));
#90789=CARTESIAN_POINT('Ctrl Pts',(-0.380265102139,-25.5727314135,-10.3153699887));
#90790=CARTESIAN_POINT('Ctrl Pts',(-0.127389297365,-25.5808054122,-10.3413729865));
#90791=CARTESIAN_POINT('Ctrl Pts',(0.127389292297,-25.5808054122,-10.3413729864));
#90792=CARTESIAN_POINT('Ctrl Pts',(0.380265098792,-25.5727314135,-10.3153699887));
#90793=CARTESIAN_POINT('Ctrl Pts',(0.627595169723,-25.5568342995,-10.2641149764));
#90794=CARTESIAN_POINT('Ctrl Pts',(-0.597178385154,-25.585971161,-10.2587039368));
#90795=CARTESIAN_POINT('Ctrl Pts',(-0.361468937707,-25.6047622193,-10.3027765927));
#90796=CARTESIAN_POINT('Ctrl Pts',(-0.121028943718,-25.614285036,-10.3250995669));
#90797=CARTESIAN_POINT('Ctrl Pts',(0.121028934599,-25.614285036,-10.3250995669));
#90798=CARTESIAN_POINT('Ctrl Pts',(0.361468931643,-25.6047622194,-10.3027765927));
#90799=CARTESIAN_POINT('Ctrl Pts',(0.597178385154,-25.585971161,-10.2587039368));
#90800=CARTESIAN_POINT('Ctrl Pts',(-0.530488628937,-25.640279625,-10.2458929885));
#90801=CARTESIAN_POINT('Ctrl Pts',(-0.320457713344,-25.662289159,-10.27663424));
#90802=CARTESIAN_POINT('Ctrl Pts',(-0.107186299105,-25.6734095169,-10.2921548338));
#90803=CARTESIAN_POINT('Ctrl Pts',(0.107186308951,-25.6734095169,-10.2921548338));
#90804=CARTESIAN_POINT('Ctrl Pts',(0.320457719891,-25.662289159,-10.27663424));
#90805=CARTESIAN_POINT('Ctrl Pts',(0.530488628937,-25.640279625,-10.2458929885));
#90806=CARTESIAN_POINT('Ctrl Pts',(-0.4531778394,-25.6783993125,-10.2291640789));
#90807=CARTESIAN_POINT('Ctrl Pts',(-0.273239866064,-25.6975272473,-10.2484964575));
#90808=CARTESIAN_POINT('Ctrl Pts',(-0.0913048492628,-25.70716081,-10.258228475));
#90809=CARTESIAN_POINT('Ctrl Pts',(0.091304838632,-25.70716081,-10.258228475));
#90810=CARTESIAN_POINT('Ctrl Pts',(0.273239858995,-25.6975272473,-10.2484964575));
#90811=CARTESIAN_POINT('Ctrl Pts',(0.4531778394,-25.6783993125,-10.2291640789));
#90812=CARTESIAN_POINT('Ctrl Pts',(-0.413292394149,-25.6957964187,-10.2198588554));
#90813=CARTESIAN_POINT('Ctrl Pts',(-0.248982805037,-25.7129087236,-10.2346106919));
#90814=CARTESIAN_POINT('Ctrl Pts',(-0.0831639035802,-25.7215163706,-10.2420292941));
#90815=CARTESIAN_POINT('Ctrl Pts',(0.0831639040251,-25.7215163706,-10.2420292941));
#90816=CARTESIAN_POINT('Ctrl Pts',(0.24898280533,-25.7129087236,-10.2346106919));
#90817=CARTESIAN_POINT('Ctrl Pts',(0.41329239415,-25.6957964187,-10.2198588554));
#90818=CARTESIAN_POINT('Ctrl Pts',(-0.307070337712,-25.7341644835,-10.1935337935));
#90819=CARTESIAN_POINT('Ctrl Pts',(-0.184562591785,-25.7449724555,-10.1984969504));
#90820=CARTESIAN_POINT('Ctrl Pts',(-0.0615742676879,-25.7503882214,-10.2009791749));
#90821=CARTESIAN_POINT('Ctrl Pts',(0.0615742669891,-25.7503882214,-10.2009791749));
#90822=CARTESIAN_POINT('Ctrl Pts',(0.184562591324,-25.7449724555,-10.1984969504));
#90823=CARTESIAN_POINT('Ctrl Pts',(0.30707033771,-25.7341644835,-10.1935337935));
#90824=CARTESIAN_POINT('Ctrl Pts',(-0.198295724974,-25.7583712199,-10.1618347919));
#90825=CARTESIAN_POINT('Ctrl Pts',(-0.119029769688,-25.7627099942,-10.1626983779));
#90826=CARTESIAN_POINT('Ctrl Pts',(-0.0396853151447,-25.7648787482,-10.1631301076));
#90827=CARTESIAN_POINT('Ctrl Pts',(0.0396853162421,-25.7648787482,-10.1631301076));
#90828=CARTESIAN_POINT('Ctrl Pts',(0.119029770412,-25.7627099942,-10.1626983779));
#90829=CARTESIAN_POINT('Ctrl Pts',(0.198295724976,-25.7583712199,-10.1618347919));
#90830=CARTESIAN_POINT('Ctrl Pts',(-0.131798268447,-25.7686774631,-10.1406643293));
#90831=CARTESIAN_POINT('Ctrl Pts',(-0.0790791152422,-25.7701121563,-10.1406657135));
#90832=CARTESIAN_POINT('Ctrl Pts',(-0.0263597373143,-25.770829644,-10.1406665006));
#90833=CARTESIAN_POINT('Ctrl Pts',(0.0263597378916,-25.770829644,-10.1406665006));
#90834=CARTESIAN_POINT('Ctrl Pts',(0.0790791156243,-25.7701121563,-10.1406657135));
#90835=CARTESIAN_POINT('Ctrl Pts',(0.131798268439,-25.7686774631,-10.1406643293));
#90836=CARTESIAN_POINT('Ctrl Pts',(-0.065481115176,-25.7742356128,-10.1171486981));
#90837=CARTESIAN_POINT('Ctrl Pts',(-0.0392886691043,-25.7742356128,-10.1171486981));
#90838=CARTESIAN_POINT('Ctrl Pts',(-0.0130962204949,-25.7742356128,-10.1171486842));
#90839=CARTESIAN_POINT('Ctrl Pts',(0.0130962205017,-25.7742356128,-10.1171486842));
#90840=CARTESIAN_POINT('Ctrl Pts',(0.039288669111,-25.7742356128,-10.1171486981));
#90841=CARTESIAN_POINT('Ctrl Pts',(0.0654811151827,-25.7742356128,-10.1171486981));
#90842=CARTESIAN_POINT('Ctrl Pts',(3.42781358853E-16,-25.7742356128,-10.0919881826));
#90843=CARTESIAN_POINT('Ctrl Pts',(3.42781358853E-16,-25.7742356128,-10.0919881826));
#90844=CARTESIAN_POINT('Ctrl Pts',(3.42781358853E-16,-25.7742356128,-10.0919881826));
#90845=CARTESIAN_POINT('Ctrl Pts',(3.42781358853E-16,-25.7742356128,-10.0919881826));
#90846=CARTESIAN_POINT('Ctrl Pts',(3.42781358853E-16,-25.7742356128,-10.0919881826));
#90847=CARTESIAN_POINT('Ctrl Pts',(3.42781358853E-16,-25.7742356128,-10.0919881826));
#90848=CARTESIAN_POINT('',(-0.647446102181,-25.4742356128,-10.2675153591));
#90849=CARTESIAN_POINT('Ctrl Pts',(-3.24740234702858E-14,-25.7742356128,
-10.0919881826));
#90850=CARTESIAN_POINT('Ctrl Pts',(-0.0235196339982131,-25.7742356128,-10.1010256276367));
#90851=CARTESIAN_POINT('Ctrl Pts',(-0.0471678069020204,-25.7733772305021,
-10.1098045487055));
#90852=CARTESIAN_POINT('Ctrl Pts',(-0.0708866431001756,-25.7717289970315,
-10.1182789368445));
#90853=CARTESIAN_POINT('Ctrl Pts',(-0.0966290502736267,-25.7699401446291,
-10.1274763168592));
#90854=CARTESIAN_POINT('Ctrl Pts',(-0.122455512086546,-25.767221846971,
-10.1363160322598));
#90855=CARTESIAN_POINT('Ctrl Pts',(-0.148303169698643,-25.7636236570487,
-10.1447855092778));
#90856=CARTESIAN_POINT('Ctrl Pts',(-0.174041159353539,-25.7600407337376,
-10.1532190515022));
#90857=CARTESIAN_POINT('Ctrl Pts',(-0.199801235626655,-25.7555858123977,
-10.1612873432931));
#90858=CARTESIAN_POINT('Ctrl Pts',(-0.225517053246078,-25.7502618225559,
-10.1689985160843));
#90859=CARTESIAN_POINT('Ctrl Pts',(-0.249359974970968,-25.7453255815644,
-10.1761480802937));
#90860=CARTESIAN_POINT('Ctrl Pts',(-0.273165470049946,-25.7396420837996,
-10.1829919915144));
#90861=CARTESIAN_POINT('Ctrl Pts',(-0.296865340757198,-25.7331730781103,
-10.1895318604185));
#90862=CARTESIAN_POINT('Ctrl Pts',(-0.308029880813459,-25.7301256575553,
-10.1926126632315));
#90863=CARTESIAN_POINT('Ctrl Pts',(-0.319170697082919,-25.7269033259966,
-10.195625803403));
#90864=CARTESIAN_POINT('Ctrl Pts',(-0.330278797444865,-25.7234987590446,
-10.1985698394716));
#90865=CARTESIAN_POINT('Ctrl Pts',(-0.34261025619996,-25.7197192399929,
-10.2018381084078));
#90866=CARTESIAN_POINT('Ctrl Pts',(-0.354897638044309,-25.7157145097747,
-10.2050204892709));
#90867=CARTESIAN_POINT('Ctrl Pts',(-0.367105872537722,-25.7114687570995,
-10.2081139321681));
#90868=CARTESIAN_POINT('Ctrl Pts',(-0.385126196057862,-25.7052016890124,
-10.2126800995225));
#90869=CARTESIAN_POINT('Ctrl Pts',(-0.40297610449847,-25.6984122503821,
-10.2170528265071));
#90870=CARTESIAN_POINT('Ctrl Pts',(-0.420636994599819,-25.6910428686672,
-10.2212375928647));
#90871=CARTESIAN_POINT('Ctrl Pts',(-0.433545439506098,-25.6856565457064,
-10.2242962623691));
#90872=CARTESIAN_POINT('Ctrl Pts',(-0.446356355529867,-25.6799606038231,
-10.2272550722783));
#90873=CARTESIAN_POINT('Ctrl Pts',(-0.459049014260705,-25.6739129474909,
-10.2301142135947));
#90874=CARTESIAN_POINT('Ctrl Pts',(-0.470368158089606,-25.6685197282054,
-10.2326639577005));
#90875=CARTESIAN_POINT('Ctrl Pts',(-0.481594267898779,-25.662846955066,
-10.235134598567));
#90876=CARTESIAN_POINT('Ctrl Pts',(-0.492677079222134,-25.6568444879693,
-10.2375207710333));
#90877=CARTESIAN_POINT('Ctrl Pts',(-0.502760483560487,-25.6513833011821,
-10.2396917672812));
#90878=CARTESIAN_POINT('Ctrl Pts',(-0.512725655776792,-25.6456492313659,
-10.2417929043888));
#90879=CARTESIAN_POINT('Ctrl Pts',(-0.52249481072194,-25.6395855696877,
-10.2438139229356));
#90880=CARTESIAN_POINT('Ctrl Pts',(-0.525208289062237,-25.6379013283465,
-10.2443752806049));
#90881=CARTESIAN_POINT('Ctrl Pts',(-0.527906371542221,-25.6361915361913,
-10.2449304144876));
#90882=CARTESIAN_POINT('Ctrl Pts',(-0.530586719226974,-25.6344546812032,
-10.2454789998168));
#90883=CARTESIAN_POINT('Ctrl Pts',(-0.537810197396088,-25.6297738951391,
-10.246957425236));
#90884=CARTESIAN_POINT('Ctrl Pts',(-0.544908504816467,-25.6248998886178,
-10.2483888192076));
#90885=CARTESIAN_POINT('Ctrl Pts',(-0.551874314062618,-25.6198254103934,
-10.2497728843233));
#90886=CARTESIAN_POINT('Ctrl Pts',(-0.559323254554293,-25.6143989789504,
-10.2512529447611));
#90887=CARTESIAN_POINT('Ctrl Pts',(-0.566620766544608,-25.6087420717409,
-10.2526789006053));
#90888=CARTESIAN_POINT('Ctrl Pts',(-0.573704306571406,-25.602809065489,
-10.2540425086271));
#90889=CARTESIAN_POINT('Ctrl Pts',(-0.581145473669519,-25.5965765192272,
-10.2554749612015));
#90890=CARTESIAN_POINT('Ctrl Pts',(-0.588350320822431,-25.5900372592432,
-10.2568385890757));
#90891=CARTESIAN_POINT('Ctrl Pts',(-0.595190181936405,-25.583125162139,
-10.258115490506));
#90892=CARTESIAN_POINT('Ctrl Pts',(-0.601870189660219,-25.5763746066417,
-10.2593625496604));
#90893=CARTESIAN_POINT('Ctrl Pts',(-0.608201257607,-25.5692663939245,-10.2605267740838));
#90894=CARTESIAN_POINT('Ctrl Pts',(-0.614019955468735,-25.561757524453,
-10.261584913393));
#90895=CARTESIAN_POINT('Ctrl Pts',(-0.619257719139411,-25.5549983345689,
-10.2625374089107));
#90896=CARTESIAN_POINT('Ctrl Pts',(-0.624079449617989,-25.5479136958671,
-10.2634038182789));
#90897=CARTESIAN_POINT('Ctrl Pts',(-0.628342381682246,-25.5405057357972,
-10.2641635474767));
#90898=CARTESIAN_POINT('Ctrl Pts',(-0.632390115918174,-25.5334717382713,
-10.2648849246504));
#90899=CARTESIAN_POINT('Ctrl Pts',(-0.6359336164384,-25.5261456012722,-10.265510058591));
#90900=CARTESIAN_POINT('Ctrl Pts',(-0.638836694515535,-25.518571015401,
-10.266019087808));
#90901=CARTESIAN_POINT('Ctrl Pts',(-0.641550569217845,-25.5114900907996,
-10.2664949418767));
#90902=CARTESIAN_POINT('Ctrl Pts',(-0.643704468813425,-25.5041918114808,
-10.2668692865141));
#90903=CARTESIAN_POINT('Ctrl Pts',(-0.645179709623052,-25.4967551141897,
-10.2671246377927));
#90904=CARTESIAN_POINT('Ctrl Pts',(-0.646649962504335,-25.4893435610736,
-10.2673791257046));
#90905=CARTESIAN_POINT('Ctrl Pts',(-0.647445936812433,-25.481793895823,
-10.2675153956504));
#90906=CARTESIAN_POINT('Ctrl Pts',(-0.647446102181,-25.4742356128,-10.2675153591));
#90907=CARTESIAN_POINT('Origin',(4.4311807394E-15,-25.4742356128,-7.33821278943));
#90908=CARTESIAN_POINT('Origin',(2.84607155346,-25.4742356128,5.53854202767));
#90909=CARTESIAN_POINT('Origin',(2.84607155346,-25.7742356128,5.53854202767));
#90910=CARTESIAN_POINT('Origin',(2.84607155346,-25.4742356128,5.53854202767));
#90911=CARTESIAN_POINT('Origin',(-3.18408167778E-16,-25.7742356128,0.729452270839));
#90912=CARTESIAN_POINT('Origin',(-7.06664156103,-21.0742356128,-3.23658091327));
#90913=CARTESIAN_POINT('',(-5.92940140951,-21.0742356128,-2.47090756951));
#90914=CARTESIAN_POINT('',(-6.1473421746,-20.7742356128,-2.26474786707));
#90915=CARTESIAN_POINT('Origin',(-6.14734217459869,-21.0742356128,-2.26474786707128));
#90916=CARTESIAN_POINT('',(-7.85893479751,-20.7742356128,-4.07415000213));
#90917=CARTESIAN_POINT('',(-7.00313848605,-20.7742356128,-3.1694489346));
#90918=CARTESIAN_POINT('',(-7.64099403241,-21.0742356128,-4.28030970457));
#90919=CARTESIAN_POINT('Ctrl Pts',(-7.85893479751,-20.7742356128,-4.07415000213));
#90920=CARTESIAN_POINT('Ctrl Pts',(-7.84849506278719,-20.7742356127997,
-4.08402540383888));
#90921=CARTESIAN_POINT('Ctrl Pts',(-7.83801774285179,-20.7752699441924,
-4.093860924025));
#90922=CARTESIAN_POINT('Ctrl Pts',(-7.82761030038593,-20.7773279598862,
-4.1035549090369));
#90923=CARTESIAN_POINT('Ctrl Pts',(-7.82358114562669,-20.778124703539,-4.10730785467891));
#90924=CARTESIAN_POINT('Ctrl Pts',(-7.81941960537616,-20.7791069904586,
-4.11117060042872));
#90925=CARTESIAN_POINT('Ctrl Pts',(-7.81529955037287,-20.780248032667,-4.11498346292577));
#90926=CARTESIAN_POINT('Ctrl Pts',(-7.81108729772222,-20.7814146088567,
-4.11888164878662));
#90927=CARTESIAN_POINT('Ctrl Pts',(-7.80691879648666,-20.7827471087771,
-4.12272732617575));
#90928=CARTESIAN_POINT('Ctrl Pts',(-7.80297123741338,-20.784162024816,-4.12635799991167));
#90929=CARTESIAN_POINT('Ctrl Pts',(-7.80080645801016,-20.7849379425518,
-4.12834900437225));
#90930=CARTESIAN_POINT('Ctrl Pts',(-7.79870792837904,-20.7857376710547,
-4.13027553448078));
#90931=CARTESIAN_POINT('Ctrl Pts',(-7.79670329286778,-20.7865412504096,
-4.13211228414853));
#90932=CARTESIAN_POINT('Ctrl Pts',(-7.78746760851805,-20.7902434722002,
-4.1405744909016));
#90933=CARTESIAN_POINT('Ctrl Pts',(-7.77851371633938,-20.7947647208706,
-4.14898219734389));
#90934=CARTESIAN_POINT('Ctrl Pts',(-7.76991752227422,-20.8000665345526,
-4.15726360072429));
#90935=CARTESIAN_POINT('Ctrl Pts',(-7.76561942524165,-20.8027174413937,
-4.16140430241449));
#90936=CARTESIAN_POINT('Ctrl Pts',(-7.7614106975515,-20.8055632750576,-4.16551348054201));
#90937=CARTESIAN_POINT('Ctrl Pts',(-7.7573004438439,-20.8085979712109,-4.16958252262954));
#90938=CARTESIAN_POINT('Ctrl Pts',(-7.7552453169901,-20.8101153192876,-4.1716170436733));
#90939=CARTESIAN_POINT('Ctrl Pts',(-7.7532148037416,-20.8116798704867,-4.17364153533306));
#90940=CARTESIAN_POINT('Ctrl Pts',(-7.7512100143084,-20.8132907906684,-4.17565494741259));
#90941=CARTESIAN_POINT('Ctrl Pts',(-7.7502076195918,-20.8140962507592,-4.17666165345236));
#90942=CARTESIAN_POINT('Ctrl Pts',(-7.7492116555409,-20.8149133022977,-4.17766558986963));
#90943=CARTESIAN_POINT('Ctrl Pts',(-7.7482222589582,-20.8157418364263,-4.17866662725692));
#90944=CARTESIAN_POINT('Ctrl Pts',(-7.74760225646034,-20.8162610349341,
-4.1792939244312));
#90945=CARTESIAN_POINT('Ctrl Pts',(-7.74662787134155,-20.8170898064891,
-4.18028384051793));
#90946=CARTESIAN_POINT('Ctrl Pts',(-7.74597119137793,-20.8176568705062,
-4.18095156732887));
#90947=CARTESIAN_POINT('Ctrl Pts',(-7.74557994506031,-20.8179947241348,
-4.18134939529746));
#90948=CARTESIAN_POINT('Ctrl Pts',(-7.74530086020065,-20.8182382659002,
-4.18163343684703));
#90949=CARTESIAN_POINT('Ctrl Pts',(-7.74527390710255,-20.8182617746731,
-4.181660914165));
#90950=CARTESIAN_POINT('Ctrl Pts',(-7.74515661698443,-20.8183640763354,
-4.18178048549805));
#90951=CARTESIAN_POINT('Ctrl Pts',(-7.74445013879524,-20.8189489345674,
-4.18243767221834));
#90952=CARTESIAN_POINT('Ctrl Pts',(-7.74316657846176,-20.8200431347351,
-4.18362102280022));
#90953=CARTESIAN_POINT('Ctrl Pts',(-7.74287007718748,-20.8202958939826,
-4.18389437571265));
#90954=CARTESIAN_POINT('Ctrl Pts',(-7.74254286865722,-20.8205760166097,
-4.18419572351062));
#90955=CARTESIAN_POINT('Ctrl Pts',(-7.74218526120033,-20.8208841621755,
-4.18452477453189));
#90956=CARTESIAN_POINT('Ctrl Pts',(-7.74123241232193,-20.8217052193183,
-4.18540153448337));
#90957=CARTESIAN_POINT('Ctrl Pts',(-7.74006349915141,-20.8227248080896,
-4.18647520710011));
#90958=CARTESIAN_POINT('Ctrl Pts',(-7.738686614958,-20.823959517673,-4.18773813660473));
#90959=CARTESIAN_POINT('Ctrl Pts',(-7.73783905626572,-20.8247195589639,
-4.18851554902947));
#90960=CARTESIAN_POINT('Ctrl Pts',(-7.7366212791383,-20.8258278773245,-4.18963152051371));
#90961=CARTESIAN_POINT('Ctrl Pts',(-7.73557557589417,-20.8267999372688,
-4.19058935247806));
#90962=CARTESIAN_POINT('Ctrl Pts',(-7.734922503253,-20.8274070174885,-4.19118754690298));
#90963=CARTESIAN_POINT('Ctrl Pts',(-7.73433596497018,-20.8279597364692,
-4.19172461049083));
#90964=CARTESIAN_POINT('Ctrl Pts',(-7.73394368876629,-20.8283313289077,
-4.19208368551059));
#90965=CARTESIAN_POINT('Ctrl Pts',(-7.73141359108293,-20.8307280207245,
-4.19439964265158));
#90966=CARTESIAN_POINT('Ctrl Pts',(-7.72923493859774,-20.8328997589094,
-4.19640894337873));
#90967=CARTESIAN_POINT('Ctrl Pts',(-7.72719909536861,-20.8350073074348,
-4.19830970528371));
#90968=CARTESIAN_POINT('Ctrl Pts',(-7.72595070836115,-20.8362996644096,
-4.1994752598964));
#90969=CARTESIAN_POINT('Ctrl Pts',(-7.72475647671546,-20.8375688873218,
-4.20059957015176));
#90970=CARTESIAN_POINT('Ctrl Pts',(-7.72357219194332,-20.8388597509998,
-4.20172462996783));
#90971=CARTESIAN_POINT('Ctrl Pts',(-7.72045660051683,-20.8422557279664,
-4.20468441362771));
#90972=CARTESIAN_POINT('Ctrl Pts',(-7.71733482311445,-20.8458756638456,
-4.20768719738774));
#90973=CARTESIAN_POINT('Ctrl Pts',(-7.71434994951472,-20.8495600603431,
-4.21059110535395));
#90974=CARTESIAN_POINT('Ctrl Pts',(-7.71136507591499,-20.8532444568406,
-4.21349501332017));
#90975=CARTESIAN_POINT('Ctrl Pts',(-7.70851723702915,-20.8569927769074,
-4.21629992165792));
#90976=CARTESIAN_POINT('Ctrl Pts',(-7.70592253659978,-20.8606057200984,
-4.21888948174501));
#90977=CARTESIAN_POINT('Ctrl Pts',(-7.70351882668188,-20.8639527220423,
-4.22128842969056));
#90978=CARTESIAN_POINT('Ctrl Pts',(-7.70102646930738,-20.867518906612,-4.22367269782641));
#90979=CARTESIAN_POINT('Ctrl Pts',(-7.69859503733839,-20.8711137133317,
-4.22591514901058));
#90980=CARTESIAN_POINT('Ctrl Pts',(-7.69610053773627,-20.8748017638493,
-4.22821576595484));
#90981=CARTESIAN_POINT('Ctrl Pts',(-7.69367034678098,-20.8785195625902,
-4.23036694169355));
#90982=CARTESIAN_POINT('Ctrl Pts',(-7.6914354950889,-20.8820242700916,-4.23226022490153));
#90983=CARTESIAN_POINT('Ctrl Pts',(-7.69114582996405,-20.8824785246354,
-4.23250561841858));
#90984=CARTESIAN_POINT('Ctrl Pts',(-7.6908594050254,-20.8829291561293,-4.23274671865086));
#90985=CARTESIAN_POINT('Ctrl Pts',(-7.69057646979513,-20.8833755998666,
-4.23298332330633));
#90986=CARTESIAN_POINT('Ctrl Pts',(-7.68827966874672,-20.8869997241689,
-4.23490402374441));
#90987=CARTESIAN_POINT('Ctrl Pts',(-7.68612525160318,-20.8906940503882,
-4.23685135783739));
#90988=CARTESIAN_POINT('Ctrl Pts',(-7.68411554461339,-20.8944545039745,
-4.23882312508471));
#90989=CARTESIAN_POINT('Ctrl Pts',(-7.6831106911185,-20.8963347307677,-4.23980900870837));
#90990=CARTESIAN_POINT('Ctrl Pts',(-7.68214201293391,-20.8982314871563,
-4.2408010027283));
#90991=CARTESIAN_POINT('Ctrl Pts',(-7.68120978772197,-20.9001442498646,
-4.24179884449155));
#90992=CARTESIAN_POINT('Ctrl Pts',(-7.68072489377046,-20.9011391672474,
-4.24231786868159));
#90993=CARTESIAN_POINT('Ctrl Pts',(-7.68003169248704,-20.9026139354804,
-4.24309349704736));
#90994=CARTESIAN_POINT('Ctrl Pts',(-7.67947389717516,-20.9038295405041,
-4.24372468740508));
#90995=CARTESIAN_POINT('Ctrl Pts',(-7.67895931191554,-20.9049509777292,
-4.24430698210563));
#90996=CARTESIAN_POINT('Ctrl Pts',(-7.67855809536675,-20.9058500061099,
-4.2447681200575));
#90997=CARTESIAN_POINT('Ctrl Pts',(-7.67852273949611,-20.9059300251565,
-4.2448096590329));
#90998=CARTESIAN_POINT('Ctrl Pts',(-7.67842273446044,-20.9061563611928,
-4.24492715314753));
#90999=CARTESIAN_POINT('Ctrl Pts',(-7.67792313080382,-20.9071520128035,
-4.24538789360321));
#91000=CARTESIAN_POINT('Ctrl Pts',(-7.67704431333244,-20.9089356457351,
-4.24617259752016));
#91001=CARTESIAN_POINT('Ctrl Pts',(-7.67662816010833,-20.9097802632117,
-4.24654418442602));
#91002=CARTESIAN_POINT('Ctrl Pts',(-7.6761274306967,-20.9108019927213,-4.24698798304712));
#91003=CARTESIAN_POINT('Ctrl Pts',(-7.67554682098165,-20.9120049371452,
-4.24749955134125));
#91004=CARTESIAN_POINT('Ctrl Pts',(-7.6746434607252,-20.9138765768287,-4.2482954912875));
#91005=CARTESIAN_POINT('Ctrl Pts',(-7.67354621288957,-20.9161866189024,
-4.24925597389064));
#91006=CARTESIAN_POINT('Ctrl Pts',(-7.6722810160251,-20.9189561339372,-4.25035646274137));
#91007=CARTESIAN_POINT('Ctrl Pts',(-7.67164475994857,-20.9203488980353,
-4.25090988864534));
#91008=CARTESIAN_POINT('Ctrl Pts',(-7.67077313411016,-20.9222878700344,
-4.25166542252786));
#91009=CARTESIAN_POINT('Ctrl Pts',(-7.66996638151831,-20.9241313941136,
-4.25236283993768));
#91010=CARTESIAN_POINT('Ctrl Pts',(-7.66916890448114,-20.9259537224649,
-4.25305223886278));
#91011=CARTESIAN_POINT('Ctrl Pts',(-7.66843406290105,-20.927681993207,-4.25368556383537));
#91012=CARTESIAN_POINT('Ctrl Pts',(-7.66801806851435,-20.9286697585403,
-4.25404343038915));
#91013=CARTESIAN_POINT('Ctrl Pts',(-7.66521378196361,-20.9353284470419,
-4.25645586766188));
#91014=CARTESIAN_POINT('Ctrl Pts',(-7.66287302397626,-20.9415795983916,
-4.25855395966484));
#91015=CARTESIAN_POINT('Ctrl Pts',(-7.66088643169644,-20.9474577204314,
-4.26044222711536));
#91016=CARTESIAN_POINT('Ctrl Pts',(-7.66050174766622,-20.9485959608743,
-4.26080787151073));
#91017=CARTESIAN_POINT('Ctrl Pts',(-7.66013042505954,-20.9497203243416,
-4.26116557117456));
#91018=CARTESIAN_POINT('Ctrl Pts',(-7.65977178445987,-20.9508312089874,
-4.2615159765629));
#91019=CARTESIAN_POINT('Ctrl Pts',(-7.65756104553905,-20.9576789443666,
-4.26367595184394));
#91020=CARTESIAN_POINT('Ctrl Pts',(-7.65556299823219,-20.9646428172267,
-4.26568628175605));
#91021=CARTESIAN_POINT('Ctrl Pts',(-7.65378344616355,-20.9717031898789,
-4.2675414763972));
#91022=CARTESIAN_POINT('Ctrl Pts',(-7.65289367012923,-20.975233376205,-4.26846907371778));
#91023=CARTESIAN_POINT('Ctrl Pts',(-7.65205850085302,-20.9787876792683,
-4.26935790335033));
#91024=CARTESIAN_POINT('Ctrl Pts',(-7.65127856258358,-20.9823635907031,
-4.27020737479072));
#91025=CARTESIAN_POINT('Ctrl Pts',(-7.65088859344886,-20.9841515464204,
-4.27063211051092));
#91026=CARTESIAN_POINT('Ctrl Pts',(-7.65051243100888,-20.9859449036594,
-4.27104700768289));
#91027=CARTESIAN_POINT('Ctrl Pts',(-7.65015014678754,-20.9877433462015,
-4.27145199864907));
#91028=CARTESIAN_POINT('Ctrl Pts',(-7.64994370704688,-20.9887681493536,
-4.27168277389431));
#91029=CARTESIAN_POINT('Ctrl Pts',(-7.64962911607452,-20.9903748845687,
-4.27203903130631));
#91030=CARTESIAN_POINT('Ctrl Pts',(-7.64940168679224,-20.9915725880104,
-4.2722981831617));
#91031=CARTESIAN_POINT('Ctrl Pts',(-7.64922999698933,-20.9924767524425,
-4.27249382081456));
#91032=CARTESIAN_POINT('Ctrl Pts',(-7.64910620270052,-20.9931470874676,
-4.2726357998818));
#91033=CARTESIAN_POINT('Ctrl Pts',(-7.64910499597593,-20.9931536117467,
-4.27263718936608));
#91034=CARTESIAN_POINT('Ctrl Pts',(-7.64910091505347,-20.9931756756687,
-4.27264188834849));
#91035=CARTESIAN_POINT('Ctrl Pts',(-7.64890512371104,-20.9940939717512,
-4.27281659316766));
#91036=CARTESIAN_POINT('Ctrl Pts',(-7.64853633164759,-20.9959155521025,
-4.27314360550097));
#91037=CARTESIAN_POINT('Ctrl Pts',(-7.64839811038513,-20.9965982705251,
-4.27326616794748));
#91038=CARTESIAN_POINT('Ctrl Pts',(-7.6482359556156,-20.9974080097675,-4.27340977700282));
#91039=CARTESIAN_POINT('Ctrl Pts',(-7.64805218413761,-20.9983455875219,
-4.27357224110587));
#91040=CARTESIAN_POINT('Ctrl Pts',(-7.64771513545709,-21.000065165274,-4.27387021069376));
#91041=CARTESIAN_POINT('Ctrl Pts',(-7.64730487789276,-21.002214682967,-4.27423207276858));
#91042=CARTESIAN_POINT('Ctrl Pts',(-7.64684216014807,-21.0048007089235,
-4.27463820022418));
#91043=CARTESIAN_POINT('Ctrl Pts',(-7.64659282098928,-21.0061942097002,
-4.27485704525293));
#91044=CARTESIAN_POINT('Ctrl Pts',(-7.64623883424678,-21.0082340176968,
-4.27516695562776));
#91045=CARTESIAN_POINT('Ctrl Pts',(-7.64593356616682,-21.010082740552,-4.27543315195173));
#91046=CARTESIAN_POINT('Ctrl Pts',(-7.645672324926,-21.0116648340767,-4.275660956503));
#91047=CARTESIAN_POINT('Ctrl Pts',(-7.64544537182912,-21.0131064775254,
-4.27585806285514));
#91048=CARTESIAN_POINT('Ctrl Pts',(-7.64532585637403,-21.0138760210362,
-4.27596172879676));
#91049=CARTESIAN_POINT('Ctrl Pts',(-7.64459396626892,-21.0185885603524,
-4.27659655947077));
#91050=CARTESIAN_POINT('Ctrl Pts',(-7.64394117298286,-21.0234810301987,
-4.27719038206959));
#91051=CARTESIAN_POINT('Ctrl Pts',(-7.64340440880833,-21.0282841408939,
-4.27770630625303));
#91052=CARTESIAN_POINT('Ctrl Pts',(-7.6431808694144,-21.0302844317194,-4.27792116667917));
#91053=CARTESIAN_POINT('Ctrl Pts',(-7.64297700046929,-21.0322691066079,
-4.27812294541838));
#91054=CARTESIAN_POINT('Ctrl Pts',(-7.64279355523369,-21.0342183284971,
-4.27831078875905));
#91055=CARTESIAN_POINT('Ctrl Pts',(-7.64154568509503,-21.0474777395748,
-4.27958857662201));
#91056=CARTESIAN_POINT('Ctrl Pts',(-7.6409439068007,-21.060856640496,-4.28025671451936));
#91057=CARTESIAN_POINT('Ctrl Pts',(-7.64099403240862,-21.0742356128,-4.28030970457131));
#91058=CARTESIAN_POINT('',(-6.78519772096,-21.0742356128,-3.37560863704));
#91059=CARTESIAN_POINT('Origin',(-0.00234331738835,-21.0742356128,3.08191746407));
#91060=CARTESIAN_POINT('',(-5.92101866809,-21.0742356128,-2.06782739988));
#91061=CARTESIAN_POINT('Ctrl Pts',(-5.92101866809097,-21.0742356128,-2.06782739988085));
#91062=CARTESIAN_POINT('Ctrl Pts',(-5.92101866809097,-21.0620465312503,
-2.06782739988085));
#91063=CARTESIAN_POINT('Ctrl Pts',(-5.92158831198356,-21.0500039224024,
-2.06829775848026));
#91064=CARTESIAN_POINT('Ctrl Pts',(-5.92269655478147,-21.0380655899987,
-2.0692329656236));
#91065=CARTESIAN_POINT('Ctrl Pts',(-5.92380273941395,-21.0261494287864,
-2.07016643595348));
#91066=CARTESIAN_POINT('Ctrl Pts',(-5.92544565218085,-21.0143360094162,
-2.07156313341593));
#91067=CARTESIAN_POINT('Ctrl Pts',(-5.92763287787142,-21.0025880579166,
-2.07345107416981));
#91068=CARTESIAN_POINT('Ctrl Pts',(-5.9288398742164,-20.9961050806079,-2.07449291342733));
#91069=CARTESIAN_POINT('Ctrl Pts',(-5.93021329816248,-20.9896422204813,
-2.07568493338501));
#91070=CARTESIAN_POINT('Ctrl Pts',(-5.93175919989028,-20.9831957718637,
-2.07703601509382));
#91071=CARTESIAN_POINT('Ctrl Pts',(-5.93467897629011,-20.9710202317257,
-2.07958783091541));
#91072=CARTESIAN_POINT('Ctrl Pts',(-5.93821952912064,-20.9589055336624,
-2.08269623846277));
#91073=CARTESIAN_POINT('Ctrl Pts',(-5.94245564556774,-20.9468902378141,
-2.08640923248926));
#91074=CARTESIAN_POINT('Ctrl Pts',(-5.94340905434637,-20.9441859947455,
-2.08724490382741));
#91075=CARTESIAN_POINT('Ctrl Pts',(-5.94439779365108,-20.9414869503422,
-2.08811128428384));
#91076=CARTESIAN_POINT('Ctrl Pts',(-5.9454228766398,-20.9387938528172,-2.08900905987206));
#91077=CARTESIAN_POINT('Ctrl Pts',(-5.9482127051728,-20.9314644166643,-2.09145241321985));
#91078=CARTESIAN_POINT('Ctrl Pts',(-5.95127145415772,-20.9241793796424,
-2.09412782900737));
#91079=CARTESIAN_POINT('Ctrl Pts',(-5.95461804302441,-20.9169637237184,
-2.0970488446907));
#91080=CARTESIAN_POINT('Ctrl Pts',(-5.95610946992881,-20.9137480244477,
-2.09835061241654));
#91081=CARTESIAN_POINT('Ctrl Pts',(-5.9577600186495,-20.9103349058525,-2.09978982587361));
#91082=CARTESIAN_POINT('Ctrl Pts',(-5.95944053176509,-20.9070148772698,
-2.10125414170714));
#91083=CARTESIAN_POINT('Ctrl Pts',(-5.9611755033533,-20.9035872603059,-2.10276590995446));
#91084=CARTESIAN_POINT('Ctrl Pts',(-5.96294225821851,-20.9002591792144,
-2.10430429923713));
#91085=CARTESIAN_POINT('Ctrl Pts',(-5.96456266631968,-20.897317568035,-2.10571435869351));
#91086=CARTESIAN_POINT('Ctrl Pts',(-5.96489459080275,-20.8967150082419,
-2.10600319534881));
#91087=CARTESIAN_POINT('Ctrl Pts',(-5.9652202685808,-20.8961285551481,-2.10628655506147));
#91088=CARTESIAN_POINT('Ctrl Pts',(-5.96553802050222,-20.895560516182,-2.10656297715136));
#91089=CARTESIAN_POINT('Ctrl Pts',(-5.96943999050983,-20.8885850398452,
-2.10995741989574));
#91090=CARTESIAN_POINT('Ctrl Pts',(-5.97377445859389,-20.8813246189463,
-2.11388641840716));
#91091=CARTESIAN_POINT('Ctrl Pts',(-5.97868787468633,-20.8738973043163,
-2.11839084933764));
#91092=CARTESIAN_POINT('Ctrl Pts',(-5.98341610951698,-20.8667499170259,
-2.12272551320837));
#91093=CARTESIAN_POINT('Ctrl Pts',(-5.98868100137614,-20.8594476500422,
-2.1275935338901));
#91094=CARTESIAN_POINT('Ctrl Pts',(-5.99461331171819,-20.8521424468673,
-2.13303105290131));
#91095=CARTESIAN_POINT('Ctrl Pts',(-6.00021350704609,-20.8452462188665,
-2.13816415734227));
#91096=CARTESIAN_POINT('Ctrl Pts',(-6.00640901896054,-20.8383473719427,
-2.14380526705499));
#91097=CARTESIAN_POINT('Ctrl Pts',(-6.01330255816048,-20.8316182518332,
-2.14997766062494));
#91098=CARTESIAN_POINT('Ctrl Pts',(-6.01774519911283,-20.8272815731396,
-2.15395554885515));
#91099=CARTESIAN_POINT('Ctrl Pts',(-6.02247760495861,-20.8230162934579,
-2.15815395116255));
#91100=CARTESIAN_POINT('Ctrl Pts',(-6.02752376872349,-20.8188791385191,
-2.16257579879535));
#91101=CARTESIAN_POINT('Ctrl Pts',(-6.03497120631767,-20.8127732718332,
-2.16910183239843));
#91102=CARTESIAN_POINT('Ctrl Pts',(-6.04312863302932,-20.806943602497,-2.17609415913291));
#91103=CARTESIAN_POINT('Ctrl Pts',(-6.05196187418653,-20.8016209760895,
-2.18359488576368));
#91104=CARTESIAN_POINT('Ctrl Pts',(-6.06049325274665,-20.7964802423534,
-2.19083928645694));
#91105=CARTESIAN_POINT('Ctrl Pts',(-6.06965539423694,-20.7918131204054,
-2.19855821334899));
#91106=CARTESIAN_POINT('Ctrl Pts',(-6.07938360613618,-20.7878444413393,
-2.20676096030881));
#91107=CARTESIAN_POINT('Ctrl Pts',(-6.08886726552373,-20.7839755288535,
-2.2147575026349));
#91108=CARTESIAN_POINT('Ctrl Pts',(-6.09888915179127,-20.7807710925393,
-2.22321405218668));
#91109=CARTESIAN_POINT('Ctrl Pts',(-6.10935206214159,-20.7784460175651,
-2.23210793494573));
#91110=CARTESIAN_POINT('Ctrl Pts',(-6.11948454120585,-20.7761943712536,
-2.24072093819615));
#91111=CARTESIAN_POINT('Ctrl Pts',(-6.13003068944631,-20.7747681652049,
-2.24974413303381));
#91112=CARTESIAN_POINT('Ctrl Pts',(-6.14086459511848,-20.7743582551055,
-2.25912546437508));
#91113=CARTESIAN_POINT('Ctrl Pts',(-6.14301298428552,-20.7742769689615,
-2.26098580461026));
#91114=CARTESIAN_POINT('Ctrl Pts',(-6.14517256622352,-20.7742356128001,
-2.26286012548388));
#91115=CARTESIAN_POINT('Ctrl Pts',(-6.1473421746,-20.7742356128,-2.26474786707));
#91116=CARTESIAN_POINT('',(-7.75696851341,-21.0742356128,1.89180060423));
#91117=CARTESIAN_POINT('Origin',(-0.00234331738835,-21.0742356128,3.08191746407));
#91118=CARTESIAN_POINT('',(-8.05349668264,-20.7742356128,1.84629187045));
#91119=CARTESIAN_POINT('Origin',(-8.05349668264169,-21.0742356128,1.84629187044922));
#91120=CARTESIAN_POINT('Origin',(-0.00234331738835,-20.7742356128,3.08191746407));
#91121=CARTESIAN_POINT('Origin',(-8.59172680003,-21.0742356128,1.84629187045));
#91122=CARTESIAN_POINT('',(-8.05349668264,-21.0742356128,2.14629187045));
#91123=CARTESIAN_POINT('Ctrl Pts',(-8.05349668264,-21.0742356128,2.14629187045));
#91124=CARTESIAN_POINT('Ctrl Pts',(-8.05349668264,-21.0616661505988,2.14629187045));
#91125=CARTESIAN_POINT('Ctrl Pts',(-8.05351323889987,-21.0492324805558,
2.1455062899062));
#91126=CARTESIAN_POINT('Ctrl Pts',(-8.05353196047696,-21.0369022763782,
2.14395984318408));
#91127=CARTESIAN_POINT('Ctrl Pts',(-8.05355061584828,-21.0246156759339,
2.14241886521572));
#91128=CARTESIAN_POINT('Ctrl Pts',(-8.05357142124933,-21.0124306137542,
2.14012220955366));
#91129=CARTESIAN_POINT('Ctrl Pts',(-8.05358013787175,-21.0003207612194,
2.13704364553627));
#91130=CARTESIAN_POINT('Ctrl Pts',(-8.05358466303609,-20.9940340288004,
2.1354454338193));
#91131=CARTESIAN_POINT('Ctrl Pts',(-8.05358593017351,-20.9877677679401,
2.13363567327742));
#91132=CARTESIAN_POINT('Ctrl Pts',(-8.05358194708828,-20.9815205327896,
2.13160558189524));
#91133=CARTESIAN_POINT('Ctrl Pts',(-8.05357646511694,-20.9729223828324,
2.12881154105794));
#91134=CARTESIAN_POINT('Ctrl Pts',(-8.0535671003131,-20.9644930322314,2.12564711986058));
#91135=CARTESIAN_POINT('Ctrl Pts',(-8.05355653390898,-20.9561289564286,
2.12206499771362));
#91136=CARTESIAN_POINT('Ctrl Pts',(-8.05354614300608,-20.94790380257,2.1185423723222));
#91137=CARTESIAN_POINT('Ctrl Pts',(-8.05353459008704,-20.9397410562187,
2.11461550731705));
#91138=CARTESIAN_POINT('Ctrl Pts',(-8.05352442499017,-20.9315661832454,
2.11019608388846));
#91139=CARTESIAN_POINT('Ctrl Pts',(-8.05351471672478,-20.9237586987363,
2.1059752745779));
#91140=CARTESIAN_POINT('Ctrl Pts',(-8.05350627434382,-20.9159395752215,
2.10130478889639));
#91141=CARTESIAN_POINT('Ctrl Pts',(-8.05350131912569,-20.908074923903,2.09607302559444));
#91142=CARTESIAN_POINT('Ctrl Pts',(-8.05349811070886,-20.9029827001034,
2.09268555061026));
#91143=CARTESIAN_POINT('Ctrl Pts',(-8.05349636422765,-20.8978720151952,
2.08906207723948));
#91144=CARTESIAN_POINT('Ctrl Pts',(-8.05349668264,-20.8927430724885,2.08516517957281));
#91145=CARTESIAN_POINT('Ctrl Pts',(-8.05349728076221,-20.8831086015271,
2.07784504566683));
#91146=CARTESIAN_POINT('Ctrl Pts',(-8.05347983282803,-20.8735442883448,
2.06966063490902));
#91147=CARTESIAN_POINT('Ctrl Pts',(-8.05346690182125,-20.8642170348392,
2.06051651168285));
#91148=CARTESIAN_POINT('Ctrl Pts',(-8.05345984899157,-20.8591297642566,
2.05552912401669));
#91149=CARTESIAN_POINT('Ctrl Pts',(-8.05345413987088,-20.8541138227069,
2.05025646025968));
#91150=CARTESIAN_POINT('Ctrl Pts',(-8.05345343537466,-20.8492024318137,
2.04468558873566));
#91151=CARTESIAN_POINT('Ctrl Pts',(-8.05345243729745,-20.8422443428754,
2.03679319727835));
#91152=CARTESIAN_POINT('Ctrl Pts',(-8.05345966742439,-20.8354966553014,
2.02830258366614));
#91153=CARTESIAN_POINT('Ctrl Pts',(-8.05347058591999,-20.8290738365618,
2.0191956109293));
#91154=CARTESIAN_POINT('Ctrl Pts',(-8.05347604516779,-20.825862427192,2.01464212456088));
#91155=CARTESIAN_POINT('Ctrl Pts',(-8.05348223770851,-20.8227325395361,
2.00993486590606));
#91156=CARTESIAN_POINT('Ctrl Pts',(-8.05348734675697,-20.8197001322682,
2.0050737622086));
#91157=CARTESIAN_POINT('Ctrl Pts',(-8.05348963342434,-20.8183429114868,
2.00289806799087));
#91158=CARTESIAN_POINT('Ctrl Pts',(-8.05349171593753,-20.81682014971,2.00038693537785));
#91159=CARTESIAN_POINT('Ctrl Pts',(-8.05349333125322,-20.8153894858194,
1.99794503575545));
#91160=CARTESIAN_POINT('Ctrl Pts',(-8.0534950936214,-20.8138285794693,1.99528083443472));
#91161=CARTESIAN_POINT('Ctrl Pts',(-8.05349629985619,-20.8123773614345,
1.99269936191406));
#91162=CARTESIAN_POINT('Ctrl Pts',(-8.05349660833629,-20.8113116696654,
1.99075986042202));
#91163=CARTESIAN_POINT('Ctrl Pts',(-8.05349664883622,-20.8111717564355,
1.9905052258963));
#91164=CARTESIAN_POINT('Ctrl Pts',(-8.05349667386182,-20.8110384236002,
1.99026169002046));
#91165=CARTESIAN_POINT('Ctrl Pts',(-8.05349668264,-20.8109122481073,1.99003054167983));
#91166=CARTESIAN_POINT('Ctrl Pts',(-8.05349692473061,-20.8074324937806,
1.98365577412581));
#91167=CARTESIAN_POINT('Ctrl Pts',(-8.05349705981208,-20.8037803081111,
1.97642146393256));
#91168=CARTESIAN_POINT('Ctrl Pts',(-8.05349712335962,-20.8001488318908,
1.96826086868649));
#91169=CARTESIAN_POINT('Ctrl Pts',(-8.05349718345239,-20.7967147809143,
1.96054392428884));
#91170=CARTESIAN_POINT('Ctrl Pts',(-8.05349717957771,-20.7932995376926,
1.95199778390212));
#91171=CARTESIAN_POINT('Ctrl Pts',(-8.0534971417338,-20.7901088517368,1.94258301047705));
#91172=CARTESIAN_POINT('Ctrl Pts',(-8.05349710520334,-20.7870289057441,
1.93349499802954));
#91173=CARTESIAN_POINT('Ctrl Pts',(-8.0534970370207,-20.784158518396,1.92359673510507));
#91174=CARTESIAN_POINT('Ctrl Pts',(-8.05349696416779,-20.781719287374,1.91288165464604));
#91175=CARTESIAN_POINT('Ctrl Pts',(-8.0534968953135,-20.7794139366638,1.9027546850711));
#91176=CARTESIAN_POINT('Ctrl Pts',(-8.05349682228755,-20.7774942735949,
1.89189752857833));
#91177=CARTESIAN_POINT('Ctrl Pts',(-8.05349676786842,-20.7761741033937,
1.88034090289527));
#91178=CARTESIAN_POINT('Ctrl Pts',(-8.05349671718391,-20.7749445324848,
1.86957737351649));
#91179=CARTESIAN_POINT('Ctrl Pts',(-8.05349668264,-20.7742356128,1.85820684501475));
#91180=CARTESIAN_POINT('Ctrl Pts',(-8.05349668264,-20.7742356128,1.84629187045));
#91181=CARTESIAN_POINT('',(-11.0596214465,-21.0742356128,2.14629187045));
#91182=CARTESIAN_POINT('',(-9.55655906459,-21.0742356128,2.14629187045));
#91183=CARTESIAN_POINT('',(-11.0596214465,-20.7742356128,1.84629187045));
#91184=CARTESIAN_POINT('Ctrl Pts',(-11.0596214465,-20.7742356128,1.84629187045));
#91185=CARTESIAN_POINT('Ctrl Pts',(-11.0596214465,-20.7742356128,1.85761625667422));
#91186=CARTESIAN_POINT('Ctrl Pts',(-11.059642963506,-20.7748745883609,1.86818502268977));
#91187=CARTESIAN_POINT('Ctrl Pts',(-11.0596632830869,-20.7759101728573,
1.87794517806547));
#91188=CARTESIAN_POINT('Ctrl Pts',(-11.0596805287041,-20.7767890932354,
1.88622880869402));
#91189=CARTESIAN_POINT('Ctrl Pts',(-11.0596969117872,-20.777953966298,1.89393130523717));
#91190=CARTESIAN_POINT('Ctrl Pts',(-11.0596985458026,-20.7792742044041,
1.90104374308561));
#91191=CARTESIAN_POINT('Ctrl Pts',(-11.0597003254466,-20.7807121061485,
1.90879006304244));
#91192=CARTESIAN_POINT('Ctrl Pts',(-11.059690915806,-20.7823340171186,1.91583863354018));
#91193=CARTESIAN_POINT('Ctrl Pts',(-11.0596791895441,-20.7839989800967,
1.92220430050639));
#91194=CARTESIAN_POINT('Ctrl Pts',(-11.0596733264131,-20.7848314615858,
1.92538713398949));
#91195=CARTESIAN_POINT('Ctrl Pts',(-11.0596670744678,-20.785675165982,1.92839953863267));
#91196=CARTESIAN_POINT('Ctrl Pts',(-11.0596624003455,-20.7865152326722,
1.93124469770798));
#91197=CARTESIAN_POINT('Ctrl Pts',(-11.0596597538015,-20.7869908884821,
1.93285566081342));
#91198=CARTESIAN_POINT('Ctrl Pts',(-11.0596574856804,-20.7873370464992,
1.93399191036223));
#91199=CARTESIAN_POINT('Ctrl Pts',(-11.0596562333712,-20.7877657305251,
1.93537052417471));
#91200=CARTESIAN_POINT('Ctrl Pts',(-11.0596552739482,-20.788094155239,1.9364267119953));
#91201=CARTESIAN_POINT('Ctrl Pts',(-11.0596549107504,-20.7884712476927,
1.93762513492828));
#91202=CARTESIAN_POINT('Ctrl Pts',(-11.0596554303936,-20.7890114782493,
1.93928215526398));
#91203=CARTESIAN_POINT('Ctrl Pts',(-11.059658976655,-20.7926982362845,1.95059035129758));
#91204=CARTESIAN_POINT('Ctrl Pts',(-11.0596541534426,-20.7968715153589,
1.9611181067061));
#91205=CARTESIAN_POINT('Ctrl Pts',(-11.0596471209352,-20.8013436976379,
1.97091130167637));
#91206=CARTESIAN_POINT('Ctrl Pts',(-11.0596396610574,-20.8060876576077,
1.98129963605465));
#91207=CARTESIAN_POINT('Ctrl Pts',(-11.0596297152047,-20.8111677980098,
1.99086227742229));
#91208=CARTESIAN_POINT('Ctrl Pts',(-11.059624636264,-20.8164139319331,1.99968020401865));
#91209=CARTESIAN_POINT('Ctrl Pts',(-11.0596215642414,-20.819587082183,2.0050137708685));
#91210=CARTESIAN_POINT('Ctrl Pts',(-11.0596202727764,-20.822822013273,2.01007530969174));
#91211=CARTESIAN_POINT('Ctrl Pts',(-11.0596223889592,-20.8260898529763,
2.01488511432867));
#91212=CARTESIAN_POINT('Ctrl Pts',(-11.0596274412372,-20.8338916523628,
2.02636827576629));
#91213=CARTESIAN_POINT('Ctrl Pts',(-11.059647255111,-20.8421947911733,2.03687551725596));
#91214=CARTESIAN_POINT('Ctrl Pts',(-11.0596612382408,-20.8507666748555,
2.04644589557552));
#91215=CARTESIAN_POINT('Ctrl Pts',(-11.0596719237107,-20.8573170399532,
2.05375927900922));
#91216=CARTESIAN_POINT('Ctrl Pts',(-11.0596792042956,-20.8640250667126,
2.06052666622852));
#91217=CARTESIAN_POINT('Ctrl Pts',(-11.0596738908863,-20.8708019000932,
2.0667793406934));
#91218=CARTESIAN_POINT('Ctrl Pts',(-11.0596677575872,-20.8786244381344,
2.07399683906081));
#91219=CARTESIAN_POINT('Ctrl Pts',(-11.0596503856799,-20.8865395212126,
2.08053044995971));
#91220=CARTESIAN_POINT('Ctrl Pts',(-11.0596353586119,-20.8944454799549,
2.08644912753701));
#91221=CARTESIAN_POINT('Ctrl Pts',(-11.0596291584308,-20.8977074852617,
2.08889117894348));
#91222=CARTESIAN_POINT('Ctrl Pts',(-11.0596238733896,-20.9011756458164,
2.09137844049239));
#91223=CARTESIAN_POINT('Ctrl Pts',(-11.0596207646266,-20.9045941052338,
2.09372218167052));
#91224=CARTESIAN_POINT('Ctrl Pts',(-11.0596174417513,-20.9082480068714,
2.09622734516174));
#91225=CARTESIAN_POINT('Ctrl Pts',(-11.0596166052546,-20.9118447609928,
2.09856830978726));
#91226=CARTESIAN_POINT('Ctrl Pts',(-11.0596197952121,-20.9150376476084,
2.10056732714775));
#91227=CARTESIAN_POINT('Ctrl Pts',(-11.0596208540094,-20.9160974171127,
2.10123083258726));
#91228=CARTESIAN_POINT('Ctrl Pts',(-11.0596223563935,-20.9171124635461,
2.10185707248893));
#91229=CARTESIAN_POINT('Ctrl Pts',(-11.0596243586796,-20.9180695616067,
2.10244058595469));
#91230=CARTESIAN_POINT('Ctrl Pts',(-11.0596517158804,-20.9311463762198,
2.11041312056716));
#91231=CARTESIAN_POINT('Ctrl Pts',(-11.0598122508444,-20.9446114029323,
2.11725326253638));
#91232=CARTESIAN_POINT('Ctrl Pts',(-11.0599398380114,-20.9583708107472,
2.12301438063896));
#91233=CARTESIAN_POINT('Ctrl Pts',(-11.059985476179,-20.9632925765907,2.12507514333156));
#91234=CARTESIAN_POINT('Ctrl Pts',(-11.0600259384965,-20.9684653521836,
2.12708203867674));
#91235=CARTESIAN_POINT('Ctrl Pts',(-11.0600554539948,-20.9736656141531,
2.12893241137108));
#91236=CARTESIAN_POINT('Ctrl Pts',(-11.060085860925,-20.9790229352646,2.13083866931689));
#91237=CARTESIAN_POINT('Ctrl Pts',(-11.0601046498154,-20.9844089944274,
2.13257846615161));
#91238=CARTESIAN_POINT('Ctrl Pts',(-11.0601055108586,-20.9895605965473,
2.13409413177296));
#91239=CARTESIAN_POINT('Ctrl Pts',(-11.0601061505986,-20.9933881462091,
2.13522024464062));
#91240=CARTESIAN_POINT('Ctrl Pts',(-11.0600968937575,-20.9970858075619,
2.13622396439941));
#91241=CARTESIAN_POINT('Ctrl Pts',(-11.0600751524104,-21.0005418908902,
2.13709977156528));
#91242=CARTESIAN_POINT('Ctrl Pts',(-11.0600142322725,-21.0102259768093,
2.13955381883132));
#91243=CARTESIAN_POINT('Ctrl Pts',(-11.0599332901061,-21.0197415078409,
2.14145488072622));
#91244=CARTESIAN_POINT('Ctrl Pts',(-11.0598566502278,-21.0291627743857,
2.14288660950867));
#91245=CARTESIAN_POINT('Ctrl Pts',(-11.059778127918,-21.0388154464452,2.14435350446906));
#91246=CARTESIAN_POINT('Ctrl Pts',(-11.0597041218377,-21.0483700448158,
2.14532786081222));
#91247=CARTESIAN_POINT('Ctrl Pts',(-11.0596607930529,-21.057924127132,2.14584810129039));
#91248=CARTESIAN_POINT('Ctrl Pts',(-11.0596361636607,-21.0633549565775,
2.14614382171796));
#91249=CARTESIAN_POINT('Ctrl Pts',(-11.0596214465,-21.0687858631891,2.14629187045));
#91250=CARTESIAN_POINT('Ctrl Pts',(-11.0596214465,-21.0742356128,2.14629187045));
#91251=CARTESIAN_POINT('',(-9.55655906459,-20.7742356128,1.84629187045));
#91252=CARTESIAN_POINT('Origin',(2.84607155346,-21.0742356128,5.53854202767));
#91253=CARTESIAN_POINT('',(-8.08214906615,-21.0742356128,-4.27458799822));
#91254=CARTESIAN_POINT('Ctrl Pts',(-7.85893479751,-20.7742356128,-4.07415000213));
#91255=CARTESIAN_POINT('Ctrl Pts',(-7.86867005783962,-20.774235612798,-4.08289189880141));
#91256=CARTESIAN_POINT('Ctrl Pts',(-7.87794459209518,-20.7750912521639,
-4.0912908295309));
#91257=CARTESIAN_POINT('Ctrl Pts',(-7.88671096678694,-20.7765812278629,
-4.09925710494256));
#91258=CARTESIAN_POINT('Ctrl Pts',(-7.89592146767705,-20.7781466894116,
-4.10762697154646));
#91259=CARTESIAN_POINT('Ctrl Pts',(-7.90457129324857,-20.7804115075564,
-4.11551947771955));
#91260=CARTESIAN_POINT('Ctrl Pts',(-7.91264842931803,-20.7831317256994,
-4.12286860916846));
#91261=CARTESIAN_POINT('Ctrl Pts',(-7.91818651298307,-20.7849968416928,
-4.12790753688732));
#91262=CARTESIAN_POINT('Ctrl Pts',(-7.92345628776262,-20.7870763568834,
-4.13269182999611));
#91263=CARTESIAN_POINT('Ctrl Pts',(-7.92846334501722,-20.7892977054482,
-4.1372085828105));
#91264=CARTESIAN_POINT('Ctrl Pts',(-7.93615415887783,-20.7927096852726,
-4.14414629160502));
#91265=CARTESIAN_POINT('Ctrl Pts',(-7.94321492459647,-20.7964557545231,
-4.15047134353813));
#91266=CARTESIAN_POINT('Ctrl Pts',(-7.94965916493774,-20.8003139394615,
-4.15622441062207));
#91267=CARTESIAN_POINT('Ctrl Pts',(-7.9512841305117,-20.8012868109515,-4.15767509145658));
#91268=CARTESIAN_POINT('Ctrl Pts',(-7.95287000622591,-20.8022670254849,
-4.15908950458363));
#91269=CARTESIAN_POINT('Ctrl Pts',(-7.95441720769774,-20.8032514563752,
-4.16046848329981));
#91270=CARTESIAN_POINT('Ctrl Pts',(-7.95825873131789,-20.8056956852532,
-4.16389232913134));
#91271=CARTESIAN_POINT('Ctrl Pts',(-7.96186133808005,-20.8081655857621,
-4.16709855052187));
#91272=CARTESIAN_POINT('Ctrl Pts',(-7.96523109252315,-20.8106188105178,
-4.17010529982328));
#91273=CARTESIAN_POINT('Ctrl Pts',(-7.9669159697447,-20.8118454228956,-4.17160867447399));
#91274=CARTESIAN_POINT('Ctrl Pts',(-7.96827678400785,-20.8128676208252,
-4.17282213945004));
#91275=CARTESIAN_POINT('Ctrl Pts',(-7.96971581084777,-20.813975090629,-4.1741107736294));
#91276=CARTESIAN_POINT('Ctrl Pts',(-7.97102627021838,-20.8149836153776,
-4.17528427692258));
#91277=CARTESIAN_POINT('Ctrl Pts',(-7.97240169868035,-20.8160629485353,
-4.17652021395837));
#91278=CARTESIAN_POINT('Ctrl Pts',(-7.97412962130567,-20.8174693670533,
-4.1780796833385));
#91279=CARTESIAN_POINT('Ctrl Pts',(-7.97429914555349,-20.8176073489502,
-4.1782326808569));
#91280=CARTESIAN_POINT('Ctrl Pts',(-7.97447204595328,-20.8177485150464,
-4.17838877747379));
#91281=CARTESIAN_POINT('Ctrl Pts',(-7.97464858184815,-20.8178931330592,
-4.17854820882513));
#91282=CARTESIAN_POINT('Ctrl Pts',(-7.98332468641013,-20.8250005884708,
-4.18638368656571));
#91283=CARTESIAN_POINT('Ctrl Pts',(-7.99131018115002,-20.8326239943172,
-4.19356432373331));
#91284=CARTESIAN_POINT('Ctrl Pts',(-7.99863186617331,-20.8405310579859,
-4.20011451649722));
#91285=CARTESIAN_POINT('Ctrl Pts',(-8.00464991219655,-20.8470302549488,
-4.20549843582576));
#91286=CARTESIAN_POINT('Ctrl Pts',(-8.01022032314814,-20.8537217587971,
-4.21045717841229));
#91287=CARTESIAN_POINT('Ctrl Pts',(-8.01537097958385,-20.8604961122412,
-4.21501600509421));
#91288=CARTESIAN_POINT('Ctrl Pts',(-8.0192422021813,-20.8655877021119,-4.21844240968732));
#91289=CARTESIAN_POINT('Ctrl Pts',(-8.02297330630799,-20.8708622671668,
-4.22173188947109));
#91290=CARTESIAN_POINT('Ctrl Pts',(-8.02646659080307,-20.8761580355519,
-4.22480987956169));
#91291=CARTESIAN_POINT('Ctrl Pts',(-8.03018669861847,-20.8817976647851,
-4.22808772738883));
#91292=CARTESIAN_POINT('Ctrl Pts',(-8.03363674440835,-20.8874607571514,
-4.23112541073459));
#91293=CARTESIAN_POINT('Ctrl Pts',(-8.03673703076693,-20.8929161654381,
-4.23386733271056));
#91294=CARTESIAN_POINT('Ctrl Pts',(-8.03931139776239,-20.8974461415163,
-4.23614412672976));
#91295=CARTESIAN_POINT('Ctrl Pts',(-8.04164554775715,-20.9018319174455,
-4.23821784132976));
#91296=CARTESIAN_POINT('Ctrl Pts',(-8.04371227855687,-20.9059300251781,
-4.24007321236907));
#91297=CARTESIAN_POINT('Ctrl Pts',(-8.04883156724945,-20.9160810310949,
-4.24466896329285));
#91298=CARTESIAN_POINT('Ctrl Pts',(-8.05332097862139,-20.9263165631395,
-4.24869954377612));
#91299=CARTESIAN_POINT('Ctrl Pts',(-8.05726683881383,-20.9365856343797,
-4.25224235137789));
#91300=CARTESIAN_POINT('Ctrl Pts',(-8.06136720484735,-20.9472568059001,
-4.25592388271582));
#91301=CARTESIAN_POINT('Ctrl Pts',(-8.06488109853223,-20.9579649933757,
-4.25907912474788));
#91302=CARTESIAN_POINT('Ctrl Pts',(-8.0678827527923,-20.968700015227,-4.26177459981986));
#91303=CARTESIAN_POINT('Ctrl Pts',(-8.07101172145835,-20.979890360314,-4.26458440278501));
#91304=CARTESIAN_POINT('Ctrl Pts',(-8.07358451687653,-20.9911107636718,
-4.26689500558006));
#91305=CARTESIAN_POINT('Ctrl Pts',(-8.0756538546644,-21.0023865074548,-4.26875358985655));
#91306=CARTESIAN_POINT('Ctrl Pts',(-8.07781579187343,-21.0141668220013,
-4.27069534268541));
#91307=CARTESIAN_POINT('Ctrl Pts',(-8.07942866747217,-21.026008635305,-4.27214413248312));
#91308=CARTESIAN_POINT('Ctrl Pts',(-8.08051195256235,-21.0379645200357,
-4.27311726631233));
#91309=CARTESIAN_POINT('Ctrl Pts',(-8.08159523765254,-21.0499204047663,
-4.27409040014153));
#91310=CARTESIAN_POINT('Ctrl Pts',(-8.08214906618287,-21.0619916709181,
-4.27458799824952));
#91311=CARTESIAN_POINT('Ctrl Pts',(-8.08214906618287,-21.0742356128,-4.27458799824952));
#91312=CARTESIAN_POINT('Origin',(2.84607155346,-20.7742356128,5.53854202767));
#91313=CARTESIAN_POINT('',(-11.3495744826,-21.0742356128,1.76930332028));
#91314=CARTESIAN_POINT('Origin',(-11.059621446593,-21.0742356128,1.8462918704235));
#91315=CARTESIAN_POINT('Origin',(2.84607155346,-21.0742356128,5.53854202767));
#91316=CARTESIAN_POINT('Origin',(-7.85893479751,-21.0742356128,-4.07415000213));
#91317=CARTESIAN_POINT('Origin',(-7.85893479751,-21.0742356128,-4.07415000213));
#91318=CARTESIAN_POINT('Origin',(-7.86219292935,-23.1742356128,-4.51414908377));
#91319=CARTESIAN_POINT('',(-5.92940140951,-22.8742356128,-2.47090756951));
#91320=CARTESIAN_POINT('',(-5.92940140951,-22.1242356128,-2.47090756951));
#91321=CARTESIAN_POINT('',(-7.64099403241,-22.8742356128,-4.28030970457));
#91322=CARTESIAN_POINT('',(-7.64099403241,-22.1242356128,-4.28030970457));
#91323=CARTESIAN_POINT('',(-6.88866980649,-22.8742356128,-3.48499366825));
#91324=CARTESIAN_POINT('Origin',(-6.1473421746,-21.0742356128,-2.26474786707));
#91325=CARTESIAN_POINT('Origin',(-6.1473421746,-21.0742356128,-2.26474786707));
#91326=CARTESIAN_POINT('Origin',(-0.00234331738835,-21.2742356128,3.08191746407));
#91327=CARTESIAN_POINT('',(-7.75696851341,-22.8742356128,1.89180060423));
#91328=CARTESIAN_POINT('',(-7.75696851341,-22.1242356128,1.89180060423));
#91329=CARTESIAN_POINT('',(-5.92101866809,-22.8742356128,-2.06782739988));
#91330=CARTESIAN_POINT('',(-5.92101866809,-22.1242356128,-2.06782739988));
#91331=CARTESIAN_POINT('Origin',(-0.00234331738837,-22.8742356128,3.08191746407));
#91332=CARTESIAN_POINT('Origin',(-8.05349668264,-21.0742356128,1.84629187045));
#91333=CARTESIAN_POINT('Origin',(-8.05349668264,-21.0742356128,1.84629187045));
#91334=CARTESIAN_POINT('Origin',(-11.4443506127,-23.1742356128,2.14629187045));
#91335=CARTESIAN_POINT('',(-8.05349668264,-22.8742356128,2.14629187045));
#91336=CARTESIAN_POINT('',(-11.0596214465,-22.8742356128,2.14629187045));
#91337=CARTESIAN_POINT('',(-6.6707290414,-22.8742356128,2.14629187045));
#91338=CARTESIAN_POINT('',(-11.0596214465,-22.1242356128,2.14629187045));
#91339=CARTESIAN_POINT('',(-8.05349668264,-22.1242356128,2.14629187045));
#91340=CARTESIAN_POINT('Origin',(-11.0596214465,-21.0742356128,1.84629187045));
#91341=CARTESIAN_POINT('Origin',(-11.0596214465,-21.0742356128,1.84629187045));
#91342=CARTESIAN_POINT('Origin',(2.84607155346,-21.2742356128,5.53854202767));
#91343=CARTESIAN_POINT('',(-11.3495744826,-22.8742356128,1.76930332028));
#91344=CARTESIAN_POINT('',(-8.08214906615,-22.8742356128,-4.27458799822));
#91345=CARTESIAN_POINT('Origin',(2.84607155346,-22.8742356128,5.53854202767));
#91346=CARTESIAN_POINT('',(-8.08214906615,-22.1242356128,-4.27458799822));
#91347=CARTESIAN_POINT('',(-11.3495744826,-22.1242356128,1.76930332028));
#91348=CARTESIAN_POINT('Origin',(-7.85893479751,-22.1242356128,-4.07415000213));
#91349=CARTESIAN_POINT('Origin',(-7.85893479751,-22.8742356128,-4.07415000213));
#91350=CARTESIAN_POINT('Origin',(-6.6707290414,-22.8742356128,-3.69115337069));
#91351=CARTESIAN_POINT('',(-7.42305326732,-23.1742356128,-4.48646940701));
#91352=CARTESIAN_POINT('Origin',(-7.42305326732,-22.8742356128,-4.48646940701));
#91353=CARTESIAN_POINT('',(-5.71146064442,-23.1742356128,-2.67706727196));
#91354=CARTESIAN_POINT('',(-6.56725695587,-23.1742356128,-3.58176833949));
#91355=CARTESIAN_POINT('Origin',(-5.71146064442,-22.8742356128,-2.67706727196));
#91356=CARTESIAN_POINT('Origin',(-6.1473421746,-22.1242356128,-2.26474786707));
#91357=CARTESIAN_POINT('Origin',(-6.1473421746,-22.8742356128,-2.26474786707));
#91358=CARTESIAN_POINT('Origin',(-0.00234331738837,-22.8742356128,3.08191746407));
#91359=CARTESIAN_POINT('',(-5.69469516158,-23.1742356128,-1.87090693268));
#91360=CARTESIAN_POINT('Origin',(-5.69469516158,-22.8742356128,-1.87090693268));
#91361=CARTESIAN_POINT('',(-7.46044034417,-23.1742356128,1.93730933801));
#91362=CARTESIAN_POINT('Origin',(-0.00234331738835,-23.1742356128,3.08191746407));
#91363=CARTESIAN_POINT('Origin',(-7.46044034417,-22.8742356128,1.93730933801));
#91364=CARTESIAN_POINT('Origin',(-8.05349668264,-22.1242356128,1.84629187045));
#91365=CARTESIAN_POINT('Origin',(-8.05349668264,-22.8742356128,1.84629187045));
#91366=CARTESIAN_POINT('Origin',(-6.6707290414,-22.8742356128,2.44629187045));
#91367=CARTESIAN_POINT('',(-8.05349668264,-23.1742356128,2.44629187045));
#91368=CARTESIAN_POINT('Origin',(-8.05349668264,-22.8742356128,2.44629187045));
#91369=CARTESIAN_POINT('',(-11.0596214465,-23.1742356128,2.44629187045));
#91370=CARTESIAN_POINT('',(-9.55655906459,-23.1742356128,2.44629187045));
#91371=CARTESIAN_POINT('Origin',(-11.0596214465,-22.8742356128,2.44629187045));
#91372=CARTESIAN_POINT('Origin',(-11.0596214465,-22.1242356128,1.84629187045));
#91373=CARTESIAN_POINT('Origin',(-11.0596214465,-22.8742356128,1.84629187045));
#91374=CARTESIAN_POINT('Origin',(2.84607155346,-22.8742356128,5.53854202767));
#91375=CARTESIAN_POINT('',(-11.6395275187,-23.1742356128,1.69231477012));
#91376=CARTESIAN_POINT('Origin',(-11.6395275187,-22.8742356128,1.69231477012));
#91377=CARTESIAN_POINT('',(-8.30536333479,-23.1742356128,-4.4750259943));
#91378=CARTESIAN_POINT('Origin',(2.84607155346,-23.1742356128,5.53854202767));
#91379=CARTESIAN_POINT('Origin',(-8.30536333479,-22.8742356128,-4.4750259943));
#91380=CARTESIAN_POINT('Origin',(-7.85893479751,-22.8742356128,-4.07415000213));
#91381=CARTESIAN_POINT('Origin',(-7.85893479751,-23.1742356128,-4.07415000213));
#91382=CARTESIAN_POINT('Origin',(-3.41821282746,-21.0742356128,8.06979469543));
#91383=CARTESIAN_POINT('',(-3.62188020465,-21.0742356128,7.84952304616));
#91384=CARTESIAN_POINT('',(-3.41821282746,-20.7742356128,8.06979469543));
#91385=CARTESIAN_POINT('Origin',(-3.41821282746,-21.0742356128,8.06979469543));
#91386=CARTESIAN_POINT('',(-3.58772315463,-21.0742356128,8.31731489457));
#91387=CARTESIAN_POINT('Origin',(-3.41821282746,-21.0742356128,8.06979469543));
#91388=CARTESIAN_POINT('Origin',(-3.41821282746,-21.0742356128,8.06979469543));
#91389=CARTESIAN_POINT('Origin',(-6.1473421746,-22.8742356128,-2.26474786707));
#91390=CARTESIAN_POINT('Origin',(-6.1473421746,-23.1742356128,-2.26474786707));
#91391=CARTESIAN_POINT('Origin',(-8.05349668264,-22.8742356128,1.84629187045));
#91392=CARTESIAN_POINT('Origin',(-8.05349668264,-23.1742356128,1.84629187045));
#91393=CARTESIAN_POINT('Origin',(-11.0596214465,-22.8742356128,1.84629187045));
#91394=CARTESIAN_POINT('Origin',(-11.0596214465,-23.1742356128,1.84629187045));
#91395=CARTESIAN_POINT('Ctrl Pts',(2.55692631419833E-13,-23.1742356128,
-6.35119542306));
#91396=CARTESIAN_POINT('Ctrl Pts',(2.55692631419833E-13,-23.1742356128,
-6.35119542306));
#91397=CARTESIAN_POINT('Ctrl Pts',(2.55692631419833E-13,-23.1742356128,
-6.35119542306));
#91398=CARTESIAN_POINT('Ctrl Pts',(2.55692631419833E-13,-23.1742356128,
-6.35119542306));
#91399=CARTESIAN_POINT('Ctrl Pts',(2.55692631419833E-13,-23.1742356128,
-6.35119542306));
#91400=CARTESIAN_POINT('Ctrl Pts',(2.55692631419833E-13,-23.1742356128,
-6.35119542306));
#91401=CARTESIAN_POINT('Ctrl Pts',(0.0693760469986,-23.1744148412,-6.42641803012));
#91402=CARTESIAN_POINT('Ctrl Pts',(0.0416634461355,-23.1744158772939,-6.42685288131863));
#91403=CARTESIAN_POINT('Ctrl Pts',(0.0138942651446,-23.1744164026919,-6.42707339217563));
#91404=CARTESIAN_POINT('Ctrl Pts',(-0.0138942622373,-23.1744164026919,-6.42707339217563));
#91405=CARTESIAN_POINT('Ctrl Pts',(-0.0416634441983,-23.1744158772939,-6.42685288131863));
#91406=CARTESIAN_POINT('Ctrl Pts',(-0.0693760469997,-23.1744148412,-6.42641803012));
#91407=CARTESIAN_POINT('Ctrl Pts',(0.139040717811,-23.1404071843,-6.49840377124));
#91408=CARTESIAN_POINT('Ctrl Pts',(0.0832786080695,-23.1440517726,-6.49672753331));
#91409=CARTESIAN_POINT('Ctrl Pts',(0.0277352763853,-23.1458041293,-6.49588968315));
#91410=CARTESIAN_POINT('Ctrl Pts',(-0.0277352847943,-23.1458041293,-6.49588968315));
#91411=CARTESIAN_POINT('Ctrl Pts',(-0.0832786136747,-23.1440517726,-6.49672753331));
#91412=CARTESIAN_POINT('Ctrl Pts',(-0.13904071781,-23.1404071843,-6.49840377124));
#91413=CARTESIAN_POINT('Ctrl Pts',(0.206909891011,-23.0789305063,-6.56242231995));
#91414=CARTESIAN_POINT('Ctrl Pts',(0.124968889226,-23.0969576242,-6.57247555688));
#91415=CARTESIAN_POINT('Ctrl Pts',(0.0417906073157,-23.1061050685,-6.57744690499));
#91416=CARTESIAN_POINT('Ctrl Pts',(-0.0417906059394,-23.1061050685,-6.57744690499));
#91417=CARTESIAN_POINT('Ctrl Pts',(-0.124968888301,-23.0969576242,-6.57247555688));
#91418=CARTESIAN_POINT('Ctrl Pts',(-0.206909891012,-23.0789305063,-6.56242231995));
#91419=CARTESIAN_POINT('Ctrl Pts',(0.247420066333,-22.976056074,-6.59957097409));
#91420=CARTESIAN_POINT('Ctrl Pts',(0.150569899025,-22.9846635857,-6.62490497029));
#91421=CARTESIAN_POINT('Ctrl Pts',(0.0505568500284,-22.9890723968,-6.63785003768));
#91422=CARTESIAN_POINT('Ctrl Pts',(-0.050556853062,-22.9890723968,-6.63785003768));
#91423=CARTESIAN_POINT('Ctrl Pts',(-0.150569901037,-22.9846635857,-6.62490497029));
#91424=CARTESIAN_POINT('Ctrl Pts',(-0.247420066332,-22.976056074,-6.59957097409));
#91425=CARTESIAN_POINT('Ctrl Pts',(0.246934114499,-22.8742356112,-6.59919568243));
#91426=CARTESIAN_POINT('Ctrl Pts',(0.150218834034,-22.8742356274,-6.62384117741));
#91427=CARTESIAN_POINT('Ctrl Pts',(0.0504288433358,-22.8742356357,-6.63642072129));
#91428=CARTESIAN_POINT('Ctrl Pts',(-0.0504288433346,-22.8742356357,-6.63642072129));
#91429=CARTESIAN_POINT('Ctrl Pts',(-0.150218834033,-22.8742356274,-6.62384117741));
#91430=CARTESIAN_POINT('Ctrl Pts',(-0.246934114499,-22.8742356112,-6.59919568243));
#91431=CARTESIAN_POINT('',(-0.246934184021341,-22.8742356128,-6.5991954979861));
#91432=CARTESIAN_POINT('Origin',(-1.7193597103E-13,-22.8742356128,-5.63016324424));
#91433=CARTESIAN_POINT('Ctrl Pts',(-0.246934184771513,-22.8742356128,-6.5991954978134));
#91434=CARTESIAN_POINT('Ctrl Pts',(-0.246934148859527,-22.8894270636949,
-6.5991955069647));
#91435=CARTESIAN_POINT('Ctrl Pts',(-0.245832550213217,-22.9049462154072,
-6.59828338132465));
#91436=CARTESIAN_POINT('Ctrl Pts',(-0.243597179910913,-22.9205953175446,
-6.59632674366846));
#91437=CARTESIAN_POINT('Ctrl Pts',(-0.241426171250814,-22.9357938447094,
-6.59442644227684));
#91438=CARTESIAN_POINT('Ctrl Pts',(-0.238185574552008,-22.9511146303327,
-6.59154030865736));
#91439=CARTESIAN_POINT('Ctrl Pts',(-0.233855755675857,-22.9663366921647,
-6.58757377565012));
#91440=CARTESIAN_POINT('Ctrl Pts',(-0.231751034635713,-22.9737361226557,
-6.58564564754233));
#91441=CARTESIAN_POINT('Ctrl Pts',(-0.229389104734593,-22.9811116449574,
-6.58346269236169));
#91442=CARTESIAN_POINT('Ctrl Pts',(-0.226768764028958,-22.9884347304813,
-6.58101708621562));
#91443=CARTESIAN_POINT('Ctrl Pts',(-0.221564610785134,-23.0029788159899,
-6.57615996624994));
#91444=CARTESIAN_POINT('Ctrl Pts',(-0.215340314283273,-23.0173176761779,
-6.57026416175073));
#91445=CARTESIAN_POINT('Ctrl Pts',(-0.208096029442936,-23.0312064758602,
-6.5632974320514));
#91446=CARTESIAN_POINT('Ctrl Pts',(-0.205901552518285,-23.0354137442222,
-6.56118703359214));
#91447=CARTESIAN_POINT('Ctrl Pts',(-0.203613572566933,-23.0395795323824,
-6.55897865797242));
#91448=CARTESIAN_POINT('Ctrl Pts',(-0.201232350872621,-23.0436965948026,
-6.55667221971715));
#91449=CARTESIAN_POINT('Ctrl Pts',(-0.19611136189576,-23.0525506344417,
-6.551712057919));
#91450=CARTESIAN_POINT('Ctrl Pts',(-0.190558945505526,-23.0611795166653,
-6.54629773499068));
#91451=CARTESIAN_POINT('Ctrl Pts',(-0.184579755856799,-23.0695085808111,
-6.54043512283862));
#91452=CARTESIAN_POINT('Ctrl Pts',(-0.181590161032435,-23.073673112884,
-6.53750381676259));
#91453=CARTESIAN_POINT('Ctrl Pts',(-0.178493887542788,-23.0777627441734,
-6.53446049681495));
#91454=CARTESIAN_POINT('Ctrl Pts',(-0.175291824842479,-23.0817677673643,
-6.53130691713594));
#91455=CARTESIAN_POINT('Ctrl Pts',(-0.173690793492324,-23.0837702789598,
-6.52973012729644));
#91456=CARTESIAN_POINT('Ctrl Pts',(-0.172063316107631,-23.0857516428652,
-6.52812577757538));
#91457=CARTESIAN_POINT('Ctrl Pts',(-0.170409517042958,-23.0877106510946,
-6.5264941352391));
#91458=CARTESIAN_POINT('Ctrl Pts',(-0.169513596563035,-23.0887719139955,
-6.52561021782966));
#91459=CARTESIAN_POINT('Ctrl Pts',(-0.16832213036844,-23.0901574536878,
-6.52443867090292));
#91460=CARTESIAN_POINT('Ctrl Pts',(-0.167302169472591,-23.0913259294168,
-6.52343072184713));
#91461=CARTESIAN_POINT('Ctrl Pts',(-0.166439362407042,-23.0923143684041,
-6.52257807585787));
#91462=CARTESIAN_POINT('Ctrl Pts',(-0.165699629296992,-23.0931490318436,
-6.52184402288916));
#91463=CARTESIAN_POINT('Ctrl Pts',(-0.165369287155041,-23.0935194071582,
-6.52151762661803));
#91464=CARTESIAN_POINT('Ctrl Pts',(-0.161836338647704,-23.0974805030916,
-6.51802687847412));
#91465=CARTESIAN_POINT('Ctrl Pts',(-0.157587882532729,-23.1019181705425,
-6.51393902538029));
#91466=CARTESIAN_POINT('Ctrl Pts',(-0.152602238932102,-23.1066909261856,
-6.50915125144019));
#91467=CARTESIAN_POINT('Ctrl Pts',(-0.147737241770845,-23.1113481870159,
-6.50447933573719));
#91468=CARTESIAN_POINT('Ctrl Pts',(-0.142170055788602,-23.1163247933947,
-6.49914001872231));
#91469=CARTESIAN_POINT('Ctrl Pts',(-0.135881001461339,-23.1214407035688,
-6.49303298020319));
#91470=CARTESIAN_POINT('Ctrl Pts',(-0.129869686747692,-23.1263306829684,
-6.48719564304621));
#91471=CARTESIAN_POINT('Ctrl Pts',(-0.123198620014974,-23.1313478806465,
-6.48065594156337));
#91472=CARTESIAN_POINT('Ctrl Pts',(-0.115854507961916,-23.1362887742648,
-6.47333550793134));
#91473=CARTESIAN_POINT('Ctrl Pts',(-0.1130506684961,-23.1381751115679,-6.47054070842717));
#91474=CARTESIAN_POINT('Ctrl Pts',(-0.110148788302281,-23.1400498356338,
-6.46763228559098));
#91475=CARTESIAN_POINT('Ctrl Pts',(-0.107148401110344,-23.1418997756208,
-6.46460672780985));
#91476=CARTESIAN_POINT('Ctrl Pts',(-0.0998500822266901,-23.1463996788256,
-6.45724718249954));
#91477=CARTESIAN_POINT('Ctrl Pts',(-0.0919682950176149,-23.1507554091233,
-6.44919239150519));
#91478=CARTESIAN_POINT('Ctrl Pts',(-0.0835018169479741,-23.1547520216881,
-6.44041063626865));
#91479=CARTESIAN_POINT('Ctrl Pts',(-0.0753232474895919,-23.1586127265988,
-6.43192751086777));
#91480=CARTESIAN_POINT('Ctrl Pts',(-0.0665989231761761,-23.1621379113261,
-6.42276530222363));
#91481=CARTESIAN_POINT('Ctrl Pts',(-0.0573371151123641,-23.1651037243234,
-6.41292977338023));
#91482=CARTESIAN_POINT('Ctrl Pts',(-0.0485532283374504,-23.1679164975296,
-6.40360177056086));
#91483=CARTESIAN_POINT('Ctrl Pts',(-0.0392858230691978,-23.1702255396838,
-6.39366771310547));
#91484=CARTESIAN_POINT('Ctrl Pts',(-0.0295520826905258,-23.1718197203897,
-6.38317190916846));
#91485=CARTESIAN_POINT('Ctrl Pts',(-0.0201296495668507,-23.1733629155545,
-6.37301178502005));
#91486=CARTESIAN_POINT('Ctrl Pts',(-0.0102701699337132,-23.1742356128018,
-6.36232486459476));
#91487=CARTESIAN_POINT('Ctrl Pts',(2.3805464551794E-13,-23.1742356128,-6.35119542306));
#91488=CARTESIAN_POINT('Origin',(2.84607155346,-22.8742356128,5.53854202767));
#91489=CARTESIAN_POINT('',(-0.45,-23.1742356128,-6.23438845923));
#91490=CARTESIAN_POINT('Origin',(2.84607155346,-23.1742356128,5.53854202767));
#91491=CARTESIAN_POINT('',(-0.530881036642,-22.8742356128,-6.52327988851));
#91492=CARTESIAN_POINT('Origin',(-0.45,-22.8742356128,-6.23438845923));
#91493=CARTESIAN_POINT('Origin',(2.84607155346,-22.8742356128,5.53854202767));
#91494=CARTESIAN_POINT('Origin',(2.93915231795E-16,-20.7742356128,0.729452270839));
#91495=CARTESIAN_POINT('Ctrl Pts',(-3.39394702409,-22.8742356071,-7.27665075406));
#91496=CARTESIAN_POINT('Ctrl Pts',(-3.3939470242,-22.8742356096,-7.39921133184));
#91497=CARTESIAN_POINT('Ctrl Pts',(-3.45653492108,-22.8742356121,-7.52177190961));
#91498=CARTESIAN_POINT('Ctrl Pts',(-3.58353228733,-22.8742356136,-7.59954001295));
#91499=CARTESIAN_POINT('Ctrl Pts',(-3.72114892405,-22.8742356136,-7.59957667728));
#91500=CARTESIAN_POINT('Ctrl Pts',(-3.83031550589,-22.8742356125,-7.54386534431));
#91501=CARTESIAN_POINT('Ctrl Pts',(-3.39394702409,-22.9689887672,-7.27665074537));
#91502=CARTESIAN_POINT('Ctrl Pts',(-3.3939470273,-22.9472590608,-7.39921132275));
#91503=CARTESIAN_POINT('Ctrl Pts',(-3.45653492596,-22.9255293543,-7.52177190012));
#91504=CARTESIAN_POINT('Ctrl Pts',(-3.5835322914,-22.9117412055,-7.59954000419));
#91505=CARTESIAN_POINT('Ctrl Pts',(-3.72114892639,-22.9117347492,-7.59957667094));
#91506=CARTESIAN_POINT('Ctrl Pts',(-3.83031550688,-22.9216122395,-7.54386534051));
#91507=CARTESIAN_POINT('Ctrl Pts',(-3.39394702409,-23.0638368546,-7.29765903263));
#91508=CARTESIAN_POINT('Ctrl Pts',(-3.39394703709,-23.0202773024,-7.41438252872));
#91509=CARTESIAN_POINT('Ctrl Pts',(-3.45551763217,-22.9767177502,-7.53110602482));
#91510=CARTESIAN_POINT('Ctrl Pts',(-3.58040884259,-22.9491120295,-7.6059738358));
#91511=CARTESIAN_POINT('Ctrl Pts',(-3.71667793436,-22.9491723593,-7.60786209828));
#91512=CARTESIAN_POINT('Ctrl Pts',(-3.82588511173,-22.969036255,-7.55663051616));
#91513=CARTESIAN_POINT('Ctrl Pts',(-3.39394702409,-23.1509380315,-7.33965594802));
#91514=CARTESIAN_POINT('Ctrl Pts',(-3.39394697957,-23.0896047046,-7.44484208723));
#91515=CARTESIAN_POINT('Ctrl Pts',(-3.45348987378,-23.0282713776,-7.55002822643));
#91516=CARTESIAN_POINT('Ctrl Pts',(-3.57418338496,-22.9885124598,-7.61911093785));
#91517=CARTESIAN_POINT('Ctrl Pts',(-3.70775302124,-22.9865706365,-7.62456986686));
#91518=CARTESIAN_POINT('Ctrl Pts',(-3.81702777332,-23.0125868459,-7.58214937101));
#91519=CARTESIAN_POINT('Ctrl Pts',(-3.39394702409,-23.3144960216,-7.46222952989));
#91520=CARTESIAN_POINT('Ctrl Pts',(-3.39394707642,-23.2249734796,-7.53850326899));
#91521=CARTESIAN_POINT('Ctrl Pts',(-3.4480237922,-23.1354509376,-7.6147770081));
#91522=CARTESIAN_POINT('Ctrl Pts',(-3.55743149517,-23.0743105508,-7.66795137089));
#91523=CARTESIAN_POINT('Ctrl Pts',(-3.68302539363,-23.0640733183,-7.67932532721));
#91524=CARTESIAN_POINT('Ctrl Pts',(-3.79142259861,-23.0943657893,-7.65641303197));
#91525=CARTESIAN_POINT('Ctrl Pts',(-3.39394702409,-23.4183511293,-7.6347947685));
#91526=CARTESIAN_POINT('Ctrl Pts',(-3.39394696259,-23.319135779,-7.67899068739));
#91527=CARTESIAN_POINT('Ctrl Pts',(-3.44128745287,-23.2199204287,-7.72318660628));
#91528=CARTESIAN_POINT('Ctrl Pts',(-3.53685705407,-23.1477285443,-7.75602607095));
#91529=CARTESIAN_POINT('Ctrl Pts',(-3.65117651028,-23.1252941134,-7.76773938497));
#91530=CARTESIAN_POINT('Ctrl Pts',(-3.75606800489,-23.1462934039,-7.76036589659));
#91531=CARTESIAN_POINT('Ctrl Pts',(-3.39394702409,-23.4554260016,-7.73594528854));
#91532=CARTESIAN_POINT('Ctrl Pts',(-3.39394732526,-23.3552502828,-7.7641726908));
#91533=CARTESIAN_POINT('Ctrl Pts',(-3.43768548772,-23.255074564,-7.79240009306));
#91534=CARTESIAN_POINT('Ctrl Pts',(-3.52588291425,-23.1798234897,-7.81406109398));
#91535=CARTESIAN_POINT('Ctrl Pts',(-3.63360843235,-23.151042617,-7.82338875536));
#91536=CARTESIAN_POINT('Ctrl Pts',(-3.73562880641,-23.1648309328,-7.82105608415));
#91537=CARTESIAN_POINT('Ctrl Pts',(-3.39394702409,-23.4742356128,-7.84128512581));
#91538=CARTESIAN_POINT('Ctrl Pts',(-3.39394702409,-23.3758453918,-7.85470223468));
#91539=CARTESIAN_POINT('Ctrl Pts',(-3.43421150493,-23.2774551707,-7.86811934354));
#91540=CARTESIAN_POINT('Ctrl Pts',(-3.51532352314,-23.2014862199,-7.87872422454));
#91541=CARTESIAN_POINT('Ctrl Pts',(-3.61626901029,-23.167728681,-7.88399310977));
#91542=CARTESIAN_POINT('Ctrl Pts',(-3.71465923135,-23.1742356128,-7.88399310977));
#91543=CARTESIAN_POINT('Ctrl Pts',(-3.39394702409,-23.4742356128,-7.94679080481));
#91544=CARTESIAN_POINT('Ctrl Pts',(-3.39394702409,-23.3799878332,-7.94679080481));
#91545=CARTESIAN_POINT('Ctrl Pts',(-3.4309580406,-23.2857400536,-7.94679080481));
#91546=CARTESIAN_POINT('Ctrl Pts',(-3.50545146488,-23.2112466293,-7.94679080481));
#91547=CARTESIAN_POINT('Ctrl Pts',(-3.59969924449,-23.1742356128,-7.94679080481));
#91548=CARTESIAN_POINT('Ctrl Pts',(-3.69394702409,-23.1742356128,-7.94679080481));
#91549=CARTESIAN_POINT('',(-3.8303155059,-22.8742356128,-7.54386534442));
#91550=CARTESIAN_POINT('',(-3.69394702409,-23.1742356128,-7.94679080481));
#91551=CARTESIAN_POINT('Ctrl Pts',(-3.8303155059,-22.8742356128,-7.54386534442));
#91552=CARTESIAN_POINT('Ctrl Pts',(-3.83031550688,-22.9216122395,-7.54386534051));
#91553=CARTESIAN_POINT('Ctrl Pts',(-3.82588511173,-22.969036255,-7.55663051616));
#91554=CARTESIAN_POINT('Ctrl Pts',(-3.81702777332,-23.0125868459,-7.58214937101));
#91555=CARTESIAN_POINT('Ctrl Pts',(-3.79142259861,-23.0943657893,-7.65641303197));
#91556=CARTESIAN_POINT('Ctrl Pts',(-3.75606800489,-23.1462934039,-7.76036589659));
#91557=CARTESIAN_POINT('Ctrl Pts',(-3.73562880641,-23.1648309328,-7.82105608415));
#91558=CARTESIAN_POINT('Ctrl Pts',(-3.71465923135,-23.1742356128,-7.88399310977));
#91559=CARTESIAN_POINT('Ctrl Pts',(-3.69394702409,-23.1742356128,-7.94679080481));
#91560=CARTESIAN_POINT('Origin',(-3.69182573245668,-23.4721143211804,-7.94679080481));
#91561=CARTESIAN_POINT('Ctrl Pts',(-3.8303155058534,-22.8742356128,-7.54386534432868));
#91562=CARTESIAN_POINT('Ctrl Pts',(-3.81518314929505,-22.8742356128939,
-7.55158788853908));
#91563=CARTESIAN_POINT('Ctrl Pts',(-3.79939056241824,-22.8742356129764,
-7.55802229157615));
#91564=CARTESIAN_POINT('Ctrl Pts',(-3.78316997118284,-22.8742356130436,
-7.5630658635742));
#91565=CARTESIAN_POINT('Ctrl Pts',(-3.76665552522089,-22.874235613112,-7.56820080569857));
#91566=CARTESIAN_POINT('Ctrl Pts',(-3.74969782981516,-22.8742356131644,
-7.57189413383619));
#91567=CARTESIAN_POINT('Ctrl Pts',(-3.73255167002916,-22.8742356131991,
-7.57409096118322));
#91568=CARTESIAN_POINT('Ctrl Pts',(-3.71493679959741,-22.8742356132347,
-7.5763478414154));
#91569=CARTESIAN_POINT('Ctrl Pts',(-3.69712349521037,-22.8742356132514,
-7.57702531075057));
#91570=CARTESIAN_POINT('Ctrl Pts',(-3.67939142268828,-22.8742356132509,
-7.57611921848549));
#91571=CARTESIAN_POINT('Ctrl Pts',(-3.66143051624416,-22.8742356132503,
-7.57520143302174));
#91572=CARTESIAN_POINT('Ctrl Pts',(-3.64355349380092,-22.8742356132319,
-7.57265914646795));
#91573=CARTESIAN_POINT('Ctrl Pts',(-3.62604663418343,-22.8742356132015,
-7.56854219910733));
#91574=CARTESIAN_POINT('Ctrl Pts',(-3.60828649605848,-22.8742356131707,
-7.56436569027734));
#91575=CARTESIAN_POINT('Ctrl Pts',(-3.59090790575233,-22.8742356131275,
-7.55856885321304));
#91576=CARTESIAN_POINT('Ctrl Pts',(-3.57419660503199,-22.8742356130833,
-7.55125591270884));
#91577=CARTESIAN_POINT('Ctrl Pts',(-3.56154804494767,-22.8742356130498,
-7.54572084581559));
#91578=CARTESIAN_POINT('Ctrl Pts',(-3.54928154903051,-22.8742356130158,
-7.53931835010142));
#91579=CARTESIAN_POINT('Ctrl Pts',(-3.53751294855566,-22.8742356129882,
-7.53211173026943));
#91580=CARTESIAN_POINT('Ctrl Pts',(-3.52194460449692,-22.8742356129516,
-7.52257829957095));
#91581=CARTESIAN_POINT('Ctrl Pts',(-3.50723469779423,-22.8742356128951,
-7.51162760824219));
#91582=CARTESIAN_POINT('Ctrl Pts',(-3.49363196674743,-22.8742356128088,
-7.49943703911464));
#91583=CARTESIAN_POINT('Ctrl Pts',(-3.48014654190352,-22.8742356127232,
-7.48735159809485));
#91584=CARTESIAN_POINT('Ctrl Pts',(-3.46774980238245,-22.8742356126084,
-7.47404796167307));
#91585=CARTESIAN_POINT('Ctrl Pts',(-3.45665074877321,-22.8742356124454,
-7.45973758957544));
#91586=CARTESIAN_POINT('Ctrl Pts',(-3.44579169741472,-22.8742356122859,
-7.4457366602135));
#91587=CARTESIAN_POINT('Ctrl Pts',(-3.43617519122419,-22.8742356120803,
-7.4307724949923));
#91588=CARTESIAN_POINT('Ctrl Pts',(-3.42795843215071,-22.8742356118008,
-7.41507410196173));
#91589=CARTESIAN_POINT('Ctrl Pts',(-3.41986382836557,-22.8742356115254,
-7.39960909069516));
#91590=CARTESIAN_POINT('Ctrl Pts',(-3.41312801722337,-22.8742356111781,
-7.38343188314801));
#91591=CARTESIAN_POINT('Ctrl Pts',(-3.40785807822884,-22.8742356107227,
-7.36678603675321));
#91592=CARTESIAN_POINT('Ctrl Pts',(-3.40271733726589,-22.8742356102784,
-7.35054828058307));
#91593=CARTESIAN_POINT('Ctrl Pts',(-3.39897168837945,-22.8742356097309,
-7.33386493486951));
#91594=CARTESIAN_POINT('Ctrl Pts',(-3.39667506741503,-22.8742356090388,
-7.31698039369392));
#91595=CARTESIAN_POINT('Ctrl Pts',(-3.39485783558188,-22.8742356084911,
-7.30362027629198));
#91596=CARTESIAN_POINT('Ctrl Pts',(-3.3939470241021,-22.8742356078525,-7.29013459097236));
#91597=CARTESIAN_POINT('Ctrl Pts',(-3.39394702409,-22.8742356071,-7.27665075406));
#91598=CARTESIAN_POINT('Origin',(2.84607155346,-22.8742356128,5.53854202767));
#91599=CARTESIAN_POINT('',(-6.53717906469,-22.8742356128,-5.76093294477));
#91600=CARTESIAN_POINT('Origin',(2.84607155346,-22.8742356128,5.53854202767));
#91601=CARTESIAN_POINT('',(-6.72883656293,-23.1742356128,-5.99173026574));
#91602=CARTESIAN_POINT('Origin',(-6.72883656293,-22.8742356128,-5.99173026574));
#91603=CARTESIAN_POINT('Origin',(2.84607155346,-23.1742356128,5.53854202767));
#91604=CARTESIAN_POINT('Origin',(1.35123173137E-15,-21.2742356128,-3.80469754864));
#91605=CARTESIAN_POINT('',(-0.11480502971,-19.4742356128,-4.08186140839));
#91606=CARTESIAN_POINT('Origin',(1.61893433855E-15,-19.4742356128,-3.80469754864));
#91607=CARTESIAN_POINT('',(-0.11480502971,-23.0742356128,-4.08186140839));
#91608=CARTESIAN_POINT('',(-0.11480502971,-21.2742356128,-4.08186140839));
#91609=CARTESIAN_POINT('Origin',(1.12255033962E-15,-23.0742356128,-3.80469754864));
#91610=CARTESIAN_POINT('Origin',(-3.1295913978,-23.1742356128,-2.83309600707));
#91611=CARTESIAN_POINT('',(-3.32093311398,-19.4742356128,-2.75383967318));
#91612=CARTESIAN_POINT('',(-3.32093311398,-23.0742356128,-2.75383967318));
#91613=CARTESIAN_POINT('',(-3.32093311398,-21.2742356128,-2.75383967318));
#91614=CARTESIAN_POINT('',(0.0382683432365,-23.0742356128,-4.14526647551));
#91615=CARTESIAN_POINT('',(0.0382683432365,-19.4742356128,-4.14526647551));
#91616=CARTESIAN_POINT('Origin',(4.78632831116E-15,-22.5742356128,-7.33821278943));
#91617=CARTESIAN_POINT('',(-0.647446102181,-19.6742356128,-10.2675153591));
#91618=CARTESIAN_POINT('',(-0.647446102181,-20.0742356128,-10.2675153591));
#91619=CARTESIAN_POINT('Origin',(-4.16333634234434E-16,-19.6742356129479,
-7.33819410486897));
#91620=CARTESIAN_POINT('Origin',(2.84607155346,-20.0742356128,5.53854202767));
#91621=CARTESIAN_POINT('',(-3.81744045688,-22.8742356128,-9.21387212773));
#91622=CARTESIAN_POINT('Ctrl Pts',(-3.81744045688,-22.8742356128,-9.21387212773));
#91623=CARTESIAN_POINT('Ctrl Pts',(-3.78438300100211,-22.8742356128,-9.22880383666651));
#91624=CARTESIAN_POINT('Ctrl Pts',(-3.75125472648156,-22.876873984767,-9.24363320588492));
#91625=CARTESIAN_POINT('Ctrl Pts',(-3.71838012225711,-22.8821739340745,
-9.25821762563378));
#91626=CARTESIAN_POINT('Ctrl Pts',(-3.6865095776919,-22.8873120117665,-9.27235660648325));
#91627=CARTESIAN_POINT('Ctrl Pts',(-3.65487745148123,-22.8949539427161,
-9.28626544525872));
#91628=CARTESIAN_POINT('Ctrl Pts',(-3.62382288627738,-22.9051278862397,
-9.29980564138486));
#91629=CARTESIAN_POINT('Ctrl Pts',(-3.59982416043969,-22.9129902304622,
-9.31026939936978));
#91630=CARTESIAN_POINT('Ctrl Pts',(-3.57617118781195,-22.9223651478789,
-9.32051284720793));
#91631=CARTESIAN_POINT('Ctrl Pts',(-3.55303923210181,-22.9332555735994,
-9.33046796299208));
#91632=CARTESIAN_POINT('Ctrl Pts',(-3.52731510523081,-22.9453663824053,
-9.34153865086025));
#91633=CARTESIAN_POINT('Ctrl Pts',(-3.50223264779224,-22.9593502627365,
-9.35225383201401));
#91634=CARTESIAN_POINT('Ctrl Pts',(-3.47806004814019,-22.9751863932197,
-9.36251314034884));
#91635=CARTESIAN_POINT('Ctrl Pts',(-3.45499124406393,-22.990299397063,-9.37230397697133));
#91636=CARTESIAN_POINT('Ctrl Pts',(-3.43275123888764,-23.0070999540256,
-9.38167960517042));
#91637=CARTESIAN_POINT('Ctrl Pts',(-3.41159767393858,-23.0255307665745,
-9.39054653772574));
#91638=CARTESIAN_POINT('Ctrl Pts',(-3.39154598669303,-23.0430015281129,
-9.39895159658247));
#91639=CARTESIAN_POINT('Ctrl Pts',(-3.37247065010445,-23.061937444689,-9.40689954920998));
#91640=CARTESIAN_POINT('Ctrl Pts',(-3.35461163146646,-23.0822474209105,
-9.41430534116002));
#91641=CARTESIAN_POINT('Ctrl Pts',(-3.34903427425971,-23.0885902102061,
-9.41661816405032));
#91642=CARTESIAN_POINT('Ctrl Pts',(-3.34357569434173,-23.0950666709068,
-9.41887806947029));
#91643=CARTESIAN_POINT('Ctrl Pts',(-3.33824360900109,-23.1016730489955,
-9.42108235584647));
#91644=CARTESIAN_POINT('Ctrl Pts',(-3.32258626090874,-23.1210722811451,
-9.42755511029096));
#91645=CARTESIAN_POINT('Ctrl Pts',(-3.30801838438582,-23.1415942623807,
-9.43354874753964));
#91646=CARTESIAN_POINT('Ctrl Pts',(-3.29472253386083,-23.1631172221777,
-9.43900011480726));
#91647=CARTESIAN_POINT('Ctrl Pts',(-3.28136620602029,-23.1847380810018,
-9.44447627808608));
#91648=CARTESIAN_POINT('Ctrl Pts',(-3.26929464819255,-23.2073686497991,
-9.44940485150287));
#91649=CARTESIAN_POINT('Ctrl Pts',(-3.25868404771759,-23.2308337864388,
-9.45372543317535));
#91650=CARTESIAN_POINT('Ctrl Pts',(-3.24835603008727,-23.253673996612,-9.45793094857403));
#91651=CARTESIAN_POINT('Ctrl Pts',(-3.23941312735556,-23.2773043321175,
-9.46156012110628));
#91652=CARTESIAN_POINT('Ctrl Pts',(-3.23199421260798,-23.3015220020268,
-9.46456562543563));
#91653=CARTESIAN_POINT('Ctrl Pts',(-3.22751779279442,-23.3161344434833,
-9.46637908462574));
#91654=CARTESIAN_POINT('Ctrl Pts',(-3.22359568701309,-23.3309599547749,
-9.46796566933521));
#91655=CARTESIAN_POINT('Ctrl Pts',(-3.22025193761968,-23.3459477027596,
-9.46931721244178));
#91656=CARTESIAN_POINT('Ctrl Pts',(-3.21506416160153,-23.3692009644169,
-9.47141411089046));
#91657=CARTESIAN_POINT('Ctrl Pts',(-3.21127189271638,-23.3928404899255,
-9.47294403759531));
#91658=CARTESIAN_POINT('Ctrl Pts',(-3.20893196554164,-23.4166584893515,
-9.47388782994456));
#91659=CARTESIAN_POINT('Ctrl Pts',(-3.20705389182888,-23.4357753059324,
-9.47464533710999));
#91660=CARTESIAN_POINT('Ctrl Pts',(-3.20611087685479,-23.4550065968702,
-9.47502544136242));
#91661=CARTESIAN_POINT('Ctrl Pts',(-3.20611087388,-23.4742356128,-9.47502544833));
#91662=CARTESIAN_POINT('',(-13.018207968,-22.8742356128,8.75735407375));
#91663=CARTESIAN_POINT('Origin',(2.84607155346,-22.8742356128,5.53854202767));
#91664=CARTESIAN_POINT('',(-12.9732844032,-22.9031898545,8.9713386779));
#91665=CARTESIAN_POINT('Origin',(-12.9922058324069,-23.4864244001328,8.73196264121582));
#91666=CARTESIAN_POINT('',(-12.9732844032,-19.6742356128,8.9713386779));
#91667=CARTESIAN_POINT('',(-12.9732844032,-21.2742356128,8.9713386779));
#91668=CARTESIAN_POINT('',(-11.5410914269,-19.6742356128,-1.88073402204));
#91669=CARTESIAN_POINT('Origin',(2.84607155346,-19.6742356128,5.53854202767));
#91670=CARTESIAN_POINT('',(-11.5410915433775,-22.0742358826999,-1.880733914433));
#91671=CARTESIAN_POINT('',(-11.5410914269,-21.2742356128,-1.88073402204));
#91672=CARTESIAN_POINT('',(-11.2053401891,-22.6742356128,-2.49849372966));
#91673=CARTESIAN_POINT('Ctrl Pts',(-11.2053401891,-22.6742356128,-2.49849372966));
#91674=CARTESIAN_POINT('Ctrl Pts',(-11.2150383685076,-22.6742356128,-2.48153808629711));
#91675=CARTESIAN_POINT('Ctrl Pts',(-11.2249897894519,-22.6738663548581,
-2.46406918052205));
#91676=CARTESIAN_POINT('Ctrl Pts',(-11.2351241182894,-22.6729000605474,
-2.44619729884691));
#91677=CARTESIAN_POINT('Ctrl Pts',(-11.2369260237553,-22.6727282513405,
-2.44301963984323));
#91678=CARTESIAN_POINT('Ctrl Pts',(-11.2387336971335,-22.6725376931046,
-2.43982928294016));
#91679=CARTESIAN_POINT('Ctrl Pts',(-11.2405467261739,-22.6723272624817,
-2.43662689819009));
#91680=CARTESIAN_POINT('Ctrl Pts',(-11.2503196279632,-22.6711929630497,
-2.41936485166077));
#91681=CARTESIAN_POINT('Ctrl Pts',(-11.2602458476986,-22.6694750423375,
-2.40175690044939));
#91682=CARTESIAN_POINT('Ctrl Pts',(-11.2702378606974,-22.6669990989714,
-2.38395208224529));
#91683=CARTESIAN_POINT('Ctrl Pts',(-11.2725244303702,-22.6664325047313,
-2.37987763224816));
#91684=CARTESIAN_POINT('Ctrl Pts',(-11.2748144198167,-22.665826417789,-2.37579294242994));
#91685=CARTESIAN_POINT('Ctrl Pts',(-11.2771067403129,-22.6651791086157,
-2.37169991214447));
#91686=CARTESIAN_POINT('Ctrl Pts',(-11.2875627511759,-22.6622265233383,
-2.35303028492714));
#91687=CARTESIAN_POINT('Ctrl Pts',(-11.2980683420681,-22.658419074168,-2.33418470244293));
#91688=CARTESIAN_POINT('Ctrl Pts',(-11.3085232390998,-22.6536382160094,
-2.31534181654695));
#91689=CARTESIAN_POINT('Ctrl Pts',(-11.311982469164,-22.6520563651097,-2.30910723793846));
#91690=CARTESIAN_POINT('Ctrl Pts',(-11.3154361566497,-22.6503683749809,
-2.30287299222311));
#91691=CARTESIAN_POINT('Ctrl Pts',(-11.3188807244952,-22.6485711953677,
-2.29664559899274));
#91692=CARTESIAN_POINT('Ctrl Pts',(-11.3296723127873,-22.6429407583018,
-2.27713561489883));
#91693=CARTESIAN_POINT('Ctrl Pts',(-11.3403771745526,-22.6362330411102,
-2.25768738349784));
#91694=CARTESIAN_POINT('Ctrl Pts',(-11.350894153497,-22.6283844511168,-2.23848952894692));
#91695=CARTESIAN_POINT('Ctrl Pts',(-11.3538790481232,-22.6261568899304,
-2.23304085654893));
#91696=CARTESIAN_POINT('Ctrl Pts',(-11.356848858058,-22.6238377439721,-2.22761230160938));
#91697=CARTESIAN_POINT('Ctrl Pts',(-11.3598014066801,-22.6214262928633,
-2.22220802156407));
#91698=CARTESIAN_POINT('Ctrl Pts',(-11.3700755207974,-22.6130350597113,
-2.20340250910257));
#91699=CARTESIAN_POINT('Ctrl Pts',(-11.380144070066,-22.6035189145293,-2.18488415807147));
#91700=CARTESIAN_POINT('Ctrl Pts',(-11.3899200358009,-22.5928768230476,
-2.16682324106742));
#91701=CARTESIAN_POINT('Ctrl Pts',(-11.3995284381226,-22.582417140672,-2.1490718943892));
#91702=CARTESIAN_POINT('Ctrl Pts',(-11.4088538998602,-22.5708701456172,
-2.13176302103624));
#91703=CARTESIAN_POINT('Ctrl Pts',(-11.4178296800987,-22.5582763477247,
-2.11503479986363));
#91704=CARTESIAN_POINT('Ctrl Pts',(-11.41987788432,-22.5554025396189,-2.11121754806936));
#91705=CARTESIAN_POINT('Ctrl Pts',(-11.4219079567884,-22.5524743831754,
-2.10743041339639));
#91706=CARTESIAN_POINT('Ctrl Pts',(-11.4239192477556,-22.5494926390321,
-2.1036748141767));
#91707=CARTESIAN_POINT('Ctrl Pts',(-11.43417381845,-22.5342902110344,-2.08452688464914));
#91708=CARTESIAN_POINT('Ctrl Pts',(-11.4439376612349,-22.5176830774906,
-2.06620306707214));
#91709=CARTESIAN_POINT('Ctrl Pts',(-11.4531160015901,-22.4997822076498,
-2.04890684167093));
#91710=CARTESIAN_POINT('Ctrl Pts',(-11.4604919004757,-22.4853967086597,
-2.03500724711187));
#91711=CARTESIAN_POINT('Ctrl Pts',(-11.4674900183935,-22.4701767234614,
-2.02177078277232));
#91712=CARTESIAN_POINT('Ctrl Pts',(-11.4740689030204,-22.4541987893081,
-2.00928995557508));
#91713=CARTESIAN_POINT('Ctrl Pts',(-11.4825434750249,-22.4336168576976,
-1.99321281260074));
#91714=CARTESIAN_POINT('Ctrl Pts',(-11.490322094781,-22.4117772815337,-1.97839019854048));
#91715=CARTESIAN_POINT('Ctrl Pts',(-11.497328194312,-22.388875007061,-1.96499799149759));
#91716=CARTESIAN_POINT('Ctrl Pts',(-11.5044353732041,-22.3656423137493,
-1.95141257056642));
#91717=CARTESIAN_POINT('Ctrl Pts',(-11.5107475618039,-22.3413165292408,
-1.93929939008369));
#91718=CARTESIAN_POINT('Ctrl Pts',(-11.516202430633,-22.3161381940112,-1.92880681486341));
#91719=CARTESIAN_POINT('Ctrl Pts',(-11.5217404470366,-22.2905760699918,
-1.91815430322522));
#91720=CARTESIAN_POINT('Ctrl Pts',(-11.5263947864914,-22.2641357626773,
-1.90917247603084));
#91721=CARTESIAN_POINT('Ctrl Pts',(-11.5301185510954,-22.2370988916848,
-1.90197624996427));
#91722=CARTESIAN_POINT('Ctrl Pts',(-11.5312011327901,-22.2292386683008,
-1.89988414602147));
#91723=CARTESIAN_POINT('Ctrl Pts',(-11.5322051805355,-22.2213281837172,
-1.89794268745646));
#91724=CARTESIAN_POINT('Ctrl Pts',(-11.5331298302645,-22.2133747150666,
-1.8961540158936));
#91725=CARTESIAN_POINT('Ctrl Pts',(-11.5363534362541,-22.18564654041,-1.88991817092117));
#91726=CARTESIAN_POINT('Ctrl Pts',(-11.538610065403,-22.1573952246849,-1.88554404014394));
#91727=CARTESIAN_POINT('Ctrl Pts',(-11.5398768288808,-22.1289373239018,
-1.88308865866385));
#91728=CARTESIAN_POINT('Ctrl Pts',(-11.5406859896255,-22.1107594899229,
-1.88152025355765));
#91729=CARTESIAN_POINT('Ctrl Pts',(-11.5410916389492,-22.0924976615588,
-1.88073379444023));
#91730=CARTESIAN_POINT('Ctrl Pts',(-11.5410916355629,-22.0742358827,-1.88073379476507));
#91731=CARTESIAN_POINT('',(-10.9558455155,-22.6742356128,-2.9197793747));
#91732=CARTESIAN_POINT('Origin',(2.84607155346,-22.6742356128,5.53854202767));
#91733=CARTESIAN_POINT('',(-10.5755260945836,-22.0742355256,-3.51114483648484));
#91734=CARTESIAN_POINT('Ctrl Pts',(-10.5755260924509,-22.0742355256,-3.51114484417453));
#91735=CARTESIAN_POINT('Ctrl Pts',(-10.5755260822369,-22.1031469614448,
-3.51114486448172));
#91736=CARTESIAN_POINT('Ctrl Pts',(-10.5767677418046,-22.1320579213261,
-3.50930400549702));
#91737=CARTESIAN_POINT('Ctrl Pts',(-10.5792325785806,-22.1606355884888,
-3.50564573524642));
#91738=CARTESIAN_POINT('Ctrl Pts',(-10.5800163561132,-22.1697228163623,
-3.50448246550852));
#91739=CARTESIAN_POINT('Ctrl Pts',(-10.5809235534889,-22.1787763809613,
-3.50313572368826));
#91740=CARTESIAN_POINT('Ctrl Pts',(-10.5819528553846,-22.1877857466703,
-3.50160709265196));
#91741=CARTESIAN_POINT('Ctrl Pts',(-10.5851501398811,-22.2157712244254,
-3.49685875950131));
#91742=CARTESIAN_POINT('Ctrl Pts',(-10.5895274155016,-22.2433280808745,
-3.49035326238203));
#91743=CARTESIAN_POINT('Ctrl Pts',(-10.5950216821739,-22.2701519594831,
-3.48216748914416));
#91744=CARTESIAN_POINT('Ctrl Pts',(-10.6005159488462,-22.2969758380917,
-3.47398171590629));
#91745=CARTESIAN_POINT('Ctrl Pts',(-10.6071270982676,-22.3230660301722,
-3.46411560723739));
#91746=CARTESIAN_POINT('Ctrl Pts',(-10.6147618810049,-22.3481448348233,
-3.45268519075675));
#91747=CARTESIAN_POINT('Ctrl Pts',(-10.622080654927,-22.3721856108078,-3.44172788693613));
#91748=CARTESIAN_POINT('Ctrl Pts',(-10.6303374421656,-22.3952935640885,
-3.42933684581246));
#91749=CARTESIAN_POINT('Ctrl Pts',(-10.6394305448135,-22.4172536196382,
-3.41564103111459));
#91750=CARTESIAN_POINT('Ctrl Pts',(-10.6482304239307,-22.4385055335036,
-3.40238686271707));
#91751=CARTESIAN_POINT('Ctrl Pts',(-10.6578134256327,-22.4586820254219,
-3.38791074678206));
#91752=CARTESIAN_POINT('Ctrl Pts',(-10.6680658047925,-22.4776185689882,
-3.37236187144591));
#91753=CARTESIAN_POINT('Ctrl Pts',(-10.6695640249749,-22.4803858400104,
-3.37008965360454));
#91754=CARTESIAN_POINT('Ctrl Pts',(-10.6710765029368,-22.4831266918782,
-3.36779458436639));
#91755=CARTESIAN_POINT('Ctrl Pts',(-10.6726028459052,-22.4858406750051,
-3.36547718891772));
#91756=CARTESIAN_POINT('Ctrl Pts',(-10.6822657120498,-22.5030221710496,
-3.35080638262523));
#91757=CARTESIAN_POINT('Ctrl Pts',(-10.6924829158915,-22.5191257906813,
-3.33524243824076));
#91758=CARTESIAN_POINT('Ctrl Pts',(-10.7031594665192,-22.5340498367433,
-3.31891032579949));
#91759=CARTESIAN_POINT('Ctrl Pts',(-10.7138348392274,-22.5489722362692,
-3.30258001524302));
#91760=CARTESIAN_POINT('Ctrl Pts',(-10.7249691157714,-22.5627148211697,
-3.28548218570648));
#91761=CARTESIAN_POINT('Ctrl Pts',(-10.7364505099692,-22.5752141494242,
-3.26777236884611));
#91762=CARTESIAN_POINT('Ctrl Pts',(-10.7411978244337,-22.5803823581624,
-3.26044973291037));
#91763=CARTESIAN_POINT('Ctrl Pts',(-10.7460043143161,-22.5853385080984,
-3.25302278904938));
#91764=CARTESIAN_POINT('Ctrl Pts',(-10.7508614475812,-22.5900803309822,
-3.24550376429458));
#91765=CARTESIAN_POINT('Ctrl Pts',(-10.7627069683827,-22.6016446341505,
-3.22716645311171));
#91766=CARTESIAN_POINT('Ctrl Pts',(-10.7748560071437,-22.6119277933076,
-3.20827751126036));
#91767=CARTESIAN_POINT('Ctrl Pts',(-10.7871852725812,-22.620935663889,-3.18901744575809));
#91768=CARTESIAN_POINT('Ctrl Pts',(-10.7903745404317,-22.6232657712414,
-3.18403535594777));
#91769=CARTESIAN_POINT('Ctrl Pts',(-10.7935758339048,-22.6255107998843,
-3.17902851552711));
#91770=CARTESIAN_POINT('Ctrl Pts',(-10.7967869569923,-22.6276714019374,
-3.17400020894282));
#91771=CARTESIAN_POINT('Ctrl Pts',(-10.8086005850894,-22.6356201938167,
-3.15550121580946));
#91772=CARTESIAN_POINT('Ctrl Pts',(-10.8205463051744,-22.6424216610541,
-3.1367127417122));
#91773=CARTESIAN_POINT('Ctrl Pts',(-10.8325097037303,-22.6481359064699,
-3.11780970742615));
#91774=CARTESIAN_POINT('Ctrl Pts',(-10.836369413317,-22.6499794735557,-3.1117110873466));
#91775=CARTESIAN_POINT('Ctrl Pts',(-10.8402309498401,-22.65171026809,-3.10560060707827));
#91776=CARTESIAN_POINT('Ctrl Pts',(-10.8440904541677,-22.6533314735688,
-3.09948429558307));
#91777=CARTESIAN_POINT('Ctrl Pts',(-10.8558666365666,-22.658278122103,-3.08082210643566));
#91778=CARTESIAN_POINT('Ctrl Pts',(-10.8676229787536,-22.6621918852187,
-3.06210658929104));
#91779=CARTESIAN_POINT('Ctrl Pts',(-10.8792423341283,-22.6652063814963,
-3.04352515477537));
#91780=CARTESIAN_POINT('Ctrl Pts',(-10.8901782818038,-22.6680435762026,
-3.02603661181894));
#91781=CARTESIAN_POINT('Ctrl Pts',(-10.9009927099857,-22.6700845210861,
-3.00866714751034));
#91782=CARTESIAN_POINT('Ctrl Pts',(-10.9115939386224,-22.6714920197301,
-2.99156911371207));
#91783=CARTESIAN_POINT('Ctrl Pts',(-10.9122564291068,-22.6715799769367,
-2.99050062579606));
#91784=CARTESIAN_POINT('Ctrl Pts',(-10.9129180895067,-22.671665477032,-2.98943319573186));
#91785=CARTESIAN_POINT('Ctrl Pts',(-10.9135788984978,-22.6717485664354,
-2.98836685977345));
#91786=CARTESIAN_POINT('Ctrl Pts',(-10.9246016135353,-22.6731345506286,
-2.9705796965187));
#91787=CARTESIAN_POINT('Ctrl Pts',(-10.9353804297876,-22.6738503295624,
-2.95310776326213));
#91788=CARTESIAN_POINT('Ctrl Pts',(-10.9458478020495,-22.6741130911883,
-2.93607201666157));
#91789=CARTESIAN_POINT('Ctrl Pts',(-10.9492132620403,-22.6741975740668,
-2.93059469893909));
#91790=CARTESIAN_POINT('Ctrl Pts',(-10.9525465530167,-22.6742356128,-2.92516247667494));
#91791=CARTESIAN_POINT('Ctrl Pts',(-10.9558455155,-22.6742356128,-2.9197793747));
#91792=CARTESIAN_POINT('',(-10.575526102,-19.6742356128,-3.51114482323));
#91793=CARTESIAN_POINT('',(-10.575526102,-21.2742356128,-3.51114482323));
#91794=CARTESIAN_POINT('Origin',(2.84607155346,-19.6742356128,5.53854202767));
#91795=CARTESIAN_POINT('Origin',(-5.88314991338E-17,-21.2742356128,5.26360209032));
#91796=CARTESIAN_POINT('',(-0.11480502971,-19.4742356128,5.54076595007));
#91797=CARTESIAN_POINT('Origin',(3.14260590599E-16,-19.4742356128,5.26360209032));
#91798=CARTESIAN_POINT('',(-0.11480502971,-23.0742356128,5.54076595007));
#91799=CARTESIAN_POINT('Origin',(-1.5436783271E-16,-23.0742356128,5.26360209032));
#91800=CARTESIAN_POINT('',(-0.11480502971,-21.2742356128,5.54076595007));
#91801=CARTESIAN_POINT('Origin',(-0.306146745892,-23.1742356128,5.46150961618));
#91802=CARTESIAN_POINT('',(-3.28628885403,-23.0742356128,4.22709433719));
#91803=CARTESIAN_POINT('',(0.0382683432365,-23.0742356128,5.60417101718));
#91804=CARTESIAN_POINT('',(-3.32093311400686,-23.0738037252489,4.21274421484887));
#91805=CARTESIAN_POINT('Origin',(-2.99360273116386,-22.7074961024392,4.3483288972549));
#91806=CARTESIAN_POINT('',(-3.32093311398,-19.4742356128,4.21274421486));
#91807=CARTESIAN_POINT('',(-3.32093311398,-21.2742356128,4.21274421486));
#91808=CARTESIAN_POINT('',(0.0382683432365,-19.4742356128,5.60417101718));
#91809=CARTESIAN_POINT('Origin',(-3.20612808427,-21.2742356128,3.93558035511));
#91810=CARTESIAN_POINT('',(-3.48329194402,-19.4742356128,4.05038538482));
#91811=CARTESIAN_POINT('Origin',(-3.20612808427,-19.4742356128,3.93558035511));
#91812=CARTESIAN_POINT('',(-3.48329194413303,-23.0738037264187,4.05038538486682));
#91813=CARTESIAN_POINT('Ctrl Pts',(-3.32093311408565,-23.0738037279965,
4.21274421481624));
#91814=CARTESIAN_POINT('Ctrl Pts',(-3.32649953892796,-23.0736167080344,
4.21043852615111));
#91815=CARTESIAN_POINT('Ctrl Pts',(-3.33218472035755,-23.0733915385147,
4.20788283100398));
#91816=CARTESIAN_POINT('Ctrl Pts',(-3.33779803563545,-23.0731489797998,
4.2051381487545));
#91817=CARTESIAN_POINT('Ctrl Pts',(-3.3433941674316,-23.0729071636055,4.20240186852682));
#91818=CARTESIAN_POINT('Ctrl Pts',(-3.34891808664344,-23.0726490695311,
4.19947790246271));
#91819=CARTESIAN_POINT('Ctrl Pts',(-3.3541921005032,-23.0723930661155,4.19647738284274));
#91820=CARTESIAN_POINT('Ctrl Pts',(-3.35966736019967,-23.0721272941207,
4.19336236938608));
#91821=CARTESIAN_POINT('Ctrl Pts',(-3.36487256382545,-23.0718643619847,
4.1901655261768));
#91822=CARTESIAN_POINT('Ctrl Pts',(-3.36963320621352,-23.0716096917244,
4.18706010956818));
#91823=CARTESIAN_POINT('Ctrl Pts',(-3.3704732769902,-23.0715647521919,4.18651212265178));
#91824=CARTESIAN_POINT('Ctrl Pts',(-3.37129957700738,-23.0715200233368,
4.18596708260654));
#91825=CARTESIAN_POINT('Ctrl Pts',(-3.37211124092873,-23.0714754752609,
4.18542605817892));
#91826=CARTESIAN_POINT('Ctrl Pts',(-3.37925430544364,-23.0710834290309,
4.18066476192198));
#91827=CARTESIAN_POINT('Ctrl Pts',(-3.38676214200264,-23.0707665220959,
4.17521843173161));
#91828=CARTESIAN_POINT('Ctrl Pts',(-3.39449455836696,-23.0705326312762,
4.16896150743035));
#91829=CARTESIAN_POINT('Ctrl Pts',(-3.39765144005647,-23.0704371416373,
4.16640701879075));
#91830=CARTESIAN_POINT('Ctrl Pts',(-3.40103633252313,-23.07035052779,4.16355761839104));
#91831=CARTESIAN_POINT('Ctrl Pts',(-3.40439681524113,-23.0702861543674,
4.16059166666122));
#91832=CARTESIAN_POINT('Ctrl Pts',(-3.40775272380699,-23.0702218685672,
4.15762975206403));
#91833=CARTESIAN_POINT('Ctrl Pts',(-3.41108364310168,-23.070179967768,4.15455185397879));
#91834=CARTESIAN_POINT('Ctrl Pts',(-3.41417028014852,-23.0701613960827,
4.15157738913841));
#91835=CARTESIAN_POINT('Ctrl Pts',(-3.41556346404581,-23.0701530135705,
4.15023483526642));
#91836=CARTESIAN_POINT('Ctrl Pts',(-3.41690737724349,-23.0701491978883,
4.14891389157001));
#91837=CARTESIAN_POINT('Ctrl Pts',(-3.41818426505082,-23.0701491888037,
4.14763700853578));
#91838=CARTESIAN_POINT('Ctrl Pts',(-3.4263619288722,-23.0701491306227,4.13945937528304));
#91839=CARTESIAN_POINT('Ctrl Pts',(-3.43407663369041,-23.0703076690209,
4.13081108398498));
#91840=CARTESIAN_POINT('Ctrl Pts',(-3.44127024360413,-23.0706011962246,
4.12174976949149));
#91841=CARTESIAN_POINT('Ctrl Pts',(-3.44816625075039,-23.0708825800805,
4.11306332551536));
#91842=CARTESIAN_POINT('Ctrl Pts',(-3.45458303810648,-23.0712882536269,
4.10399736533341));
#91843=CARTESIAN_POINT('Ctrl Pts',(-3.4604744230075,-23.0717516366824,4.09460399601809));
#91844=CARTESIAN_POINT('Ctrl Pts',(-3.46583461881877,-23.0721732394048,
4.08605756768185));
#91845=CARTESIAN_POINT('Ctrl Pts',(-3.47075949094676,-23.0726427185181,
4.07724017642156));
#91846=CARTESIAN_POINT('Ctrl Pts',(-3.4752236042024,-23.0730692325225,4.06819151220635));
#91847=CARTESIAN_POINT('Ctrl Pts',(-3.47810595867232,-23.0733446208196,
4.06234903997189));
#91848=CARTESIAN_POINT('Ctrl Pts',(-3.48079639531383,-23.0736013142645,
4.05641016936358));
#91849=CARTESIAN_POINT('Ctrl Pts',(-3.48329194424607,-23.0738037257,4.05038538491364));
#91850=CARTESIAN_POINT('',(-3.48329194402,-21.2742356128,4.05038538482));
#91851=CARTESIAN_POINT('Origin',(-3.56254827791,-23.1742356128,3.85904366864));
#91852=CARTESIAN_POINT('',(-3.49764208328952,-23.0742356036667,4.0157410839798));
#91853=CARTESIAN_POINT('Origin',(-3.61516698256916,-22.7188054056451,3.73201086501446));
#91854=CARTESIAN_POINT('',(-4.7969635569,-23.0742356128,0.878901560502));
#91855=CARTESIAN_POINT('',(-3.72150316839,-23.0742356128,3.47529261624));
#91856=CARTESIAN_POINT('',(-4.81131367924113,-23.0738037252489,0.844257300522139));
#91857=CARTESIAN_POINT('Origin',(-4.67572895257626,-22.7074959741112,1.17158778382924));
#91858=CARTESIAN_POINT('',(-4.81131367923,-19.4742356128,0.844257300549));
#91859=CARTESIAN_POINT('',(-4.81131367923,-21.2742356128,0.844257300549));
#91860=CARTESIAN_POINT('',(-4.02322090503,-19.4742356128,2.74688156443));
#91861=CARTESIAN_POINT('Origin',(-4.53414981948,-21.2742356128,0.729452270839));
#91862=CARTESIAN_POINT('',(-4.81131367923,-19.4742356128,0.614647241129));
#91863=CARTESIAN_POINT('Origin',(-4.53414981948,-19.4742356128,0.729452270839));
#91864=CARTESIAN_POINT('',(-4.81131367935289,-23.0738037265127,0.61464724109448));
#91865=CARTESIAN_POINT('Ctrl Pts',(-4.81131367927376,-23.0738037279964,
0.844257300443346));
#91866=CARTESIAN_POINT('Ctrl Pts',(-4.81361936799537,-23.0736167080296,
0.838690875456146));
#91867=CARTESIAN_POINT('Ctrl Pts',(-4.81583224901354,-23.0733915385045,
0.832863695608802));
#91868=CARTESIAN_POINT('Ctrl Pts',(-4.81786067891667,-23.0731489797839,
0.826953698746072));
#91869=CARTESIAN_POINT('Ctrl Pts',(-4.81988289938928,-23.0729071635841,
0.821061793568343));
#91870=CARTESIAN_POINT('Ctrl Pts',(-4.82172134391612,-23.0726490695041,
0.815088236474101));
#91871=CARTESIAN_POINT('Ctrl Pts',(-4.82332894712803,-23.0723930660825,
0.809237257609517));
#91872=CARTESIAN_POINT('Ctrl Pts',(-4.82499789326136,-23.0721272940827,
0.803163017100496));
#91873=CARTESIAN_POINT('Ctrl Pts',(-4.82641801853694,-23.0718643619411,
0.797221872695268));
#91874=CARTESIAN_POINT('Ctrl Pts',(-4.82758843991301,-23.0716096916733,
0.791659728914695));
#91875=CARTESIAN_POINT('Ctrl Pts',(-4.82779497430443,-23.0715647521585,
0.790678224300857));
#91876=CARTESIAN_POINT('Ctrl Pts',(-4.8279938550574,-23.0715200233209,0.78970854082669));
#91877=CARTESIAN_POINT('Ctrl Pts',(-4.82818522600442,-23.0714754752622,
0.788752046093464));
#91878=CARTESIAN_POINT('Ctrl Pts',(-4.82986939051381,-23.0710834290264,
0.780334391751288));
#91879=CARTESIAN_POINT('Ctrl Pts',(-4.83132709564776,-23.0707665220907,
0.771174412539057));
#91880=CARTESIAN_POINT('Ctrl Pts',(-4.83237042608539,-23.0705326312721,
0.761282454889659));
#91881=CARTESIAN_POINT('Ctrl Pts',(-4.8327963823021,-23.0704371416318,0.757243906119096));
#91882=CARTESIAN_POINT('Ctrl Pts',(-4.83317503237506,-23.0703505277842,
0.752835595290697));
#91883=CARTESIAN_POINT('Ctrl Pts',(-4.83345400791012,-23.0702861543619,
0.748362130534413));
#91884=CARTESIAN_POINT('Ctrl Pts',(-4.83373260371525,-23.0702218685622,
0.743894754873028));
#91885=CARTESIAN_POINT('Ctrl Pts',(-4.83391151672308,-23.0701799677641,
0.739363036592918));
#91886=CARTESIAN_POINT('Ctrl Pts',(-4.83399083444416,-23.0701613960804,
0.735077190299951));
#91887=CARTESIAN_POINT('Ctrl Pts',(-4.83402663527135,-23.0701530135698,
0.73314273176506));
#91888=CARTESIAN_POINT('Ctrl Pts',(-4.83404287715848,-23.0701491978883,
0.731258393567419));
#91889=CARTESIAN_POINT('Ctrl Pts',(-4.83404288053355,-23.0701491888037,
0.729452605050674));
#91890=CARTESIAN_POINT('Ctrl Pts',(-4.83404290214876,-23.0701491306227,
0.717887663578479));
#91891=CARTESIAN_POINT('Ctrl Pts',(-4.8333827568176,-23.0703076690209,0.706317278061772));
#91892=CARTESIAN_POINT('Ctrl Pts',(-4.83206209024346,-23.0706011962248,
0.694823310783213));
#91893=CARTESIAN_POINT('Ctrl Pts',(-4.83079606021932,-23.0708825800807,
0.683804853925016));
#91894=CARTESIAN_POINT('Ctrl Pts',(-4.82892281214912,-23.0712882536273,
0.672856898147235));
#91895=CARTESIAN_POINT('Ctrl Pts',(-4.82644653522177,-23.071751636683,0.662048944789373));
#91896=CARTESIAN_POINT('Ctrl Pts',(-4.8241935285967,-23.0721732394055,0.652215476549306));
#91897=CARTESIAN_POINT('Ctrl Pts',(-4.82144110192226,-23.0726427185188,
0.642498228916228));
#91898=CARTESIAN_POINT('Ctrl Pts',(-4.81819933485018,-23.0730692325233,
0.632943252331222));
#91899=CARTESIAN_POINT('Ctrl Pts',(-4.81610621550821,-23.0733446208201,
0.626773868209116));
#91900=CARTESIAN_POINT('Ctrl Pts',(-4.81380922582505,-23.0736013142647,
0.620672026540791));
#91901=CARTESIAN_POINT('Ctrl Pts',(-4.81131367946162,-23.0738037257,0.614647241033059));
#91902=CARTESIAN_POINT('',(-4.81131367923,-21.2742356128,0.614647241129));
#91903=CARTESIAN_POINT('Origin',(-4.73205734534,-23.1742356128,0.423305524947));
#91904=CARTESIAN_POINT('',(-4.80666892645645,-23.0740393995008,0.603433815990868));
#91905=CARTESIAN_POINT('Ctrl Pts',(-4.81131367925832,-23.0738037283007,
0.614647241182803));
#91906=CARTESIAN_POINT('Ctrl Pts',(-4.80976568786345,-23.0738979005228,
0.610910059368051));
#91907=CARTESIAN_POINT('Ctrl Pts',(-4.80821741312739,-23.0739763495673,
0.607172193515546));
#91908=CARTESIAN_POINT('Ctrl Pts',(-4.80666892647,-23.0740393981,0.603433816023));
#91909=CARTESIAN_POINT('',(-4.79748444904916,-23.0742356281333,0.581260526068347));
#91910=CARTESIAN_POINT('Ctrl Pts',(-4.80666892644968,-23.0740394002012,
0.603433815974802));
#91911=CARTESIAN_POINT('Ctrl Pts',(-4.80360593375962,-23.0741641147023,
0.596039097464416));
#91912=CARTESIAN_POINT('Ctrl Pts',(-4.800544079459,-23.0742356283685,0.588647127288019));
#91913=CARTESIAN_POINT('Ctrl Pts',(-4.79748444904758,-23.0742356358,0.581260526069004));
#91914=CARTESIAN_POINT('',(-3.48329194402,-23.0742356128,-2.59148084314));
#91915=CARTESIAN_POINT('',(-6.0279343243,-23.0742356128,3.55182930271));
#91916=CARTESIAN_POINT('',(-3.48329194402,-19.4742356128,-2.59148084314));
#91917=CARTESIAN_POINT('',(-3.48329194402,-21.2742356128,-2.59148084314));
#91918=CARTESIAN_POINT('',(-5.72621658766,-19.4742356128,2.8234182509));
#91919=CARTESIAN_POINT('Origin',(-3.20612808427,-21.2742356128,-2.47667581343));
#91920=CARTESIAN_POINT('Origin',(-3.20612808427,-19.4742356128,-2.47667581343));
#91921=CARTESIAN_POINT('Origin',(-3.20612808427,-23.0742356128,-2.47667581343));
#91922=CARTESIAN_POINT('Origin',(-9.38771846805,-25.4742356128,12.7721409138));
#91923=CARTESIAN_POINT('',(-9.57074430825,-25.4742356128,13.0098414435));
#91924=CARTESIAN_POINT('Origin',(-9.38771846805,-25.4742356128,12.7721409138));
#91925=CARTESIAN_POINT('Origin',(-9.38771846805,-25.4742356128,12.7721409138));
#91926=CARTESIAN_POINT('Origin',(-2.72521192632E-16,-25.4742356128,0.580061096523));
#91927=CARTESIAN_POINT('',(-12.4158608431,-25.4742356128,10.1688558911));
#91928=CARTESIAN_POINT('Origin',(-2.72521192632E-16,-25.4742356128,0.580061096523));
#91929=CARTESIAN_POINT('Origin',(-12.1784264826,-25.4742356128,9.98548488886));
#91930=CARTESIAN_POINT('Origin',(2.4183046301E-16,-21.2742356128,0.580061096523));
#91931=CARTESIAN_POINT('',(-12.4158607189067,-19.6742356128,10.1688560519572));
#91932=CARTESIAN_POINT('',(-3.109463736,-19.6742356128,15.9563357222));
#91933=CARTESIAN_POINT('Origin',(-8.94493678676E-16,-19.6742356128,0.580061096523));
#91934=CARTESIAN_POINT('',(-12.4158608431,-21.2742356128,10.1688558911));
#91935=CARTESIAN_POINT('',(-9.57074430825,-23.4742356128,13.0098414435));
#91936=CARTESIAN_POINT('',(-9.57074430825,-22.5741587422,13.0098414435));
#91937=CARTESIAN_POINT('',(-9.06991786753072,-22.874235391647,13.3798726563422));
#91938=CARTESIAN_POINT('Ctrl Pts',(-9.0699178675,-22.8742351711,13.3798726563));
#91939=CARTESIAN_POINT('Ctrl Pts',(-9.22406041417,-22.8742363569,13.2706476151));
#91940=CARTESIAN_POINT('Ctrl Pts',(-9.3768173424,-22.9427255764,13.1589191215));
#91941=CARTESIAN_POINT('Ctrl Pts',(-9.5056235281,-23.0835945845,13.0599834668));
#91942=CARTESIAN_POINT('Ctrl Pts',(-9.57074430825,-23.2789184576,13.0098414435));
#91943=CARTESIAN_POINT('Ctrl Pts',(-9.57074430825,-23.4742356128,13.0098414435));
#91944=CARTESIAN_POINT('Origin',(4.58869751468E-17,-22.8742356128,0.580061096523));
#91945=CARTESIAN_POINT('',(-2.49776595187,-21.2742356128,16.0674673138));
#91946=CARTESIAN_POINT('Origin',(-1.97861558624E-15,-21.2742356128,0.580061096523));
#91947=CARTESIAN_POINT('',(-3.10946375819683,-20.6742355012,15.9563357201048));
#91948=CARTESIAN_POINT('Ctrl Pts',(-3.10946378033221,-20.6742355012,15.9563357204339));
#91949=CARTESIAN_POINT('Ctrl Pts',(-3.10946378735857,-20.7002248449885,
15.95633571906));
#91950=CARTESIAN_POINT('Ctrl Pts',(-3.10773833558802,-20.7262145171259,
15.9566848789689));
#91951=CARTESIAN_POINT('Ctrl Pts',(-3.10431023879153,-20.7519525807421,
15.9573769620387));
#91952=CARTESIAN_POINT('Ctrl Pts',(-3.10395560128583,-20.7546151901211,
15.9574485582124));
#91953=CARTESIAN_POINT('Ctrl Pts',(-3.10358278308959,-20.7572751232837,
15.9575238125558));
#91954=CARTESIAN_POINT('Ctrl Pts',(-3.10319183705832,-20.7599321129217,
15.9576027102366));
#91955=CARTESIAN_POINT('Ctrl Pts',(-3.099307134996,-20.7863337446062,15.9583866905278));
#91956=CARTESIAN_POINT('Ctrl Pts',(-3.0936290098475,-20.8124388627447,15.9595314025541));
#91957=CARTESIAN_POINT('Ctrl Pts',(-3.08623683217655,-20.8379928558938,
15.9610147519107));
#91958=CARTESIAN_POINT('Ctrl Pts',(-3.07851101700349,-20.8647001993577,
15.9625650505474));
#91959=CARTESIAN_POINT('Ctrl Pts',(-3.06891341716237,-20.8908050127768,
15.9644850853575));
#91960=CARTESIAN_POINT('Ctrl Pts',(-3.05758035100362,-20.9160480560527,
15.9667371363132));
#91961=CARTESIAN_POINT('Ctrl Pts',(-3.04602935090593,-20.9417765209943,
15.9690324940253));
#91962=CARTESIAN_POINT('Ctrl Pts',(-3.03267630960258,-20.9666092779845,
15.9716725056088));
#91963=CARTESIAN_POINT('Ctrl Pts',(-3.01770170425029,-20.9903114039395,
15.9746078088576));
#91964=CARTESIAN_POINT('Ctrl Pts',(-3.0026101605923,-21.0141986223484,15.9775660342055));
#91965=CARTESIAN_POINT('Ctrl Pts',(-2.98587257741445,-21.0369370503983,
15.9808238878688));
#91966=CARTESIAN_POINT('Ctrl Pts',(-2.9676965498713,-21.058332813913,15.9843255532809));
#91967=CARTESIAN_POINT('Ctrl Pts',(-2.96474362937427,-21.0618088203441,
15.9848944421399));
#91968=CARTESIAN_POINT('Ctrl Pts',(-2.96175277307212,-21.0652494956996,
15.9854697605075));
#91969=CARTESIAN_POINT('Ctrl Pts',(-2.95872490069565,-21.0686541357244,
15.9860512642797));
#91970=CARTESIAN_POINT('Ctrl Pts',(-2.93804665294392,-21.0919054426437,
15.9900225277859));
#91971=CARTESIAN_POINT('Ctrl Pts',(-2.91564036809565,-21.1134718480583,
15.9942823225078));
#91972=CARTESIAN_POINT('Ctrl Pts',(-2.89181128846758,-21.1331574400962,
15.9987514051654));
#91973=CARTESIAN_POINT('Ctrl Pts',(-2.87100351620025,-21.1503470807564,
16.0026538493904));
#91974=CARTESIAN_POINT('Ctrl Pts',(-2.8491109162229,-21.1661037147375,16.0067158795856));
#91975=CARTESIAN_POINT('Ctrl Pts',(-2.82633684712334,-21.1803292052124,
16.010887082969));
#91976=CARTESIAN_POINT('Ctrl Pts',(-2.79803654352825,-21.1980065775549,
16.016070448383));
#91977=CARTESIAN_POINT('Ctrl Pts',(-2.76837177274804,-21.2133225213693,
16.0214227358652));
#91978=CARTESIAN_POINT('Ctrl Pts',(-2.73773014859016,-21.2261403216352,
16.0268536353127));
#91979=CARTESIAN_POINT('Ctrl Pts',(-2.7149562079203,-21.235666964912,16.0308900721922));
#91980=CARTESIAN_POINT('Ctrl Pts',(-2.69164267896409,-21.2438149588589,
16.0349700557871));
#91981=CARTESIAN_POINT('Ctrl Pts',(-2.66794852457163,-21.2505464024847,
16.0390594036265));
#91982=CARTESIAN_POINT('Ctrl Pts',(-2.6320530991438,-21.2607441934119,16.0452545553078));
#91983=CARTESIAN_POINT('Ctrl Pts',(-2.59528016107295,-21.2676884801428,
16.051471061566));
#91984=CARTESIAN_POINT('Ctrl Pts',(-2.55817677954374,-21.2713011763122,
16.0576035767246));
#91985=CARTESIAN_POINT('Ctrl Pts',(-2.53810797210176,-21.2732552435907,
16.0609205861394));
#91986=CARTESIAN_POINT('Ctrl Pts',(-2.51794240601556,-21.2742356128,16.0642133111923));
#91987=CARTESIAN_POINT('Ctrl Pts',(-2.49776595187,-21.2742356128,16.0674673138));
#91988=CARTESIAN_POINT('',(-3.109463736,-22.4223864096,15.9563357222));
#91989=CARTESIAN_POINT('Origin',(-9.38771846805,-22.5741587422,12.7721409138));
#91990=CARTESIAN_POINT('',(-9.18405109086,-23.4742356128,12.9924125631));
#91991=CARTESIAN_POINT('Origin',(-9.38771846805,-23.4742356128,12.7721409138));
#91992=CARTESIAN_POINT('',(-9.18405109086,-24.4742356128,12.9924125631));
#91993=CARTESIAN_POINT('Origin',(-3.88971125292,-23.1742356128,8.09716475273));
#91994=CARTESIAN_POINT('',(-5.19285862192,-22.8742356128,9.30207971851));
#91995=CARTESIAN_POINT('',(-6.46706166421,-22.8742356128,10.4802322066));
#91996=CARTESIAN_POINT('',(-5.19285862192,-21.0742356128,9.30207971851));
#91997=CARTESIAN_POINT('',(-5.19285862192,-21.9742356128,9.30207971851));
#91998=CARTESIAN_POINT('',(-8.34854625295,-21.0742356128,12.2198888201));
#91999=CARTESIAN_POINT('',(-6.71750298683,-21.0742356128,10.7117950404));
#92000=CARTESIAN_POINT('',(-8.34854625295,-22.8742356128,12.2198888201));
#92001=CARTESIAN_POINT('',(-8.34854625295,-21.9742356128,12.2198888201));
#92002=CARTESIAN_POINT('',(-8.78908955148,-23.4742356128,12.6272235745));
#92003=CARTESIAN_POINT('Origin',(-8.78908955139227,-22.8742356128972,12.627223574425));
#92004=CARTESIAN_POINT('',(-6.87439641858,-23.4742356128,10.8568617063));
#92005=CARTESIAN_POINT('Origin',(-4.98919124473,-21.9742356128,9.52235136777));
#92006=CARTESIAN_POINT('',(-4.80552303981,-22.8742356128,9.28514683472));
#92007=CARTESIAN_POINT('Origin',(-4.98919124473,-22.8742356128,9.52235136777));
#92008=CARTESIAN_POINT('',(-4.80552303981,-21.0742356128,9.28514683472));
#92009=CARTESIAN_POINT('',(-4.80552303981,-21.2742356128,9.28514683472));
#92010=CARTESIAN_POINT('Origin',(-4.98919124473,-21.0742356128,9.52235136777));
#92011=CARTESIAN_POINT('Origin',(-0.00234331738835,-21.2742356128,3.08191746407));
#92012=CARTESIAN_POINT('',(-1.01141425905,-21.0742356128,10.8621723381));
#92013=CARTESIAN_POINT('',(-1.01141425905,-22.8742356128,10.8621723381));
#92014=CARTESIAN_POINT('',(-1.01141425905,-21.9742356128,10.8621723381));
#92015=CARTESIAN_POINT('Origin',(-0.00234331738803,-21.0742356128,3.08191746407));
#92016=CARTESIAN_POINT('Origin',(-0.00234331738803,-22.8742356128,3.08191746407));
#92017=CARTESIAN_POINT('Origin',(-1.05,-21.9742356128,11.1596805575));
#92018=CARTESIAN_POINT('',(-0.75,-22.8742356128,11.1596805575));
#92019=CARTESIAN_POINT('Origin',(-1.05,-22.8742356128,11.1596805575));
#92020=CARTESIAN_POINT('',(-0.75,-21.0742356128,11.1596805575));
#92021=CARTESIAN_POINT('',(-0.75,-21.9742356128,11.1596805575));
#92022=CARTESIAN_POINT('Origin',(-1.05,-21.0742356128,11.1596805575));
#92023=CARTESIAN_POINT('Origin',(-0.75,-23.1742356128,-8.70195642562));
#92024=CARTESIAN_POINT('',(-0.75,-21.0742356128,14.92922515));
#92025=CARTESIAN_POINT('',(-0.75,-22.8742356128,14.92922515));
#92026=CARTESIAN_POINT('',(-0.75,-21.9742356128,14.92922515));
#92027=CARTESIAN_POINT('',(-0.75,-21.0742356128,12.1167294155));
#92028=CARTESIAN_POINT('',(-0.75,-22.8742356128,2.93538176615));
#92029=CARTESIAN_POINT('Origin',(-8.14487887576,-21.9742356128,12.4401604693));
#92030=CARTESIAN_POINT('',(-8.31471092647,-22.8742356128,12.6874600337));
#92031=CARTESIAN_POINT('Ctrl Pts',(-8.31471092647,-22.8742356128,12.6874600337));
#92032=CARTESIAN_POINT('Ctrl Pts',(-8.32883744679105,-22.8742356128,12.6777586987252));
#92033=CARTESIAN_POINT('Ctrl Pts',(-8.34213871713093,-22.87423561284,12.6668454324847));
#92034=CARTESIAN_POINT('Ctrl Pts',(-8.35440983412802,-22.8742356129023,
12.65487775851));
#92035=CARTESIAN_POINT('Ctrl Pts',(-8.36739587231599,-22.8742356129683,
12.6422128420811));
#92036=CARTESIAN_POINT('Ctrl Pts',(-8.37922775178076,-22.8742356130598,
12.6283672875421));
#92037=CARTESIAN_POINT('Ctrl Pts',(-8.38970962078642,-22.8742356131585,
12.6135677349304));
#92038=CARTESIAN_POINT('Ctrl Pts',(-8.4000338934081,-22.8742356132558,12.5989906956869));
#92039=CARTESIAN_POINT('Ctrl Pts',(-8.40904851996284,-22.8742356133604,
12.5834888008467));
#92040=CARTESIAN_POINT('Ctrl Pts',(-8.4166128270163,-22.8742356134502,12.5673088581972));
#92041=CARTESIAN_POINT('Ctrl Pts',(-8.42435033379277,-22.8742356135419,
12.550758443862));
#92042=CARTESIAN_POINT('Ctrl Pts',(-8.43057011020167,-22.8742356136185,
12.5334991192691));
#92043=CARTESIAN_POINT('Ctrl Pts',(-8.43517222719556,-22.8742356136446,
12.5158179803121));
#92044=CARTESIAN_POINT('Ctrl Pts',(-8.43977434418945,-22.8742356136708,
12.4981368413551));
#92045=CARTESIAN_POINT('Ctrl Pts',(-8.44275875512409,-22.8742356136469,
12.4800345388221));
#92046=CARTESIAN_POINT('Ctrl Pts',(-8.44407743450015,-22.8742356135222,
12.4618116758578));
#92047=CARTESIAN_POINT('Ctrl Pts',(-8.44539020172562,-22.8742356133981,
12.4436705130489));
#92048=CARTESIAN_POINT('Ctrl Pts',(-8.44505217626979,-22.8742356132917,
12.4254099092049));
#92049=CARTESIAN_POINT('Ctrl Pts',(-8.44306743009479,-22.8742356132021,
12.4073301787109));
#92050=CARTESIAN_POINT('Ctrl Pts',(-8.44111043587038,-22.8742356131139,
12.3895032502093));
#92051=CARTESIAN_POINT('Ctrl Pts',(-8.43755252343825,-22.8742356130421,
12.3718527651297));
#92052=CARTESIAN_POINT('Ctrl Pts',(-8.43244743182453,-22.8742356129856,
12.3546611841392));
#92053=CARTESIAN_POINT('Ctrl Pts',(-8.42740525448748,-22.8742356129299,
12.337681469255));
#92054=CARTESIAN_POINT('Ctrl Pts',(-8.42085385627011,-22.8742356128891,
12.3211499566653));
#92055=CARTESIAN_POINT('Ctrl Pts',(-8.41289301572016,-22.8742356128608,
12.3053251052911));
#92056=CARTESIAN_POINT('Ctrl Pts',(-8.40484005245799,-22.8742356128322,
12.2893171290043));
#92057=CARTESIAN_POINT('Ctrl Pts',(-8.39534470099704,-22.8742356128163,
12.2740328873715));
#92058=CARTESIAN_POINT('Ctrl Pts',(-8.38456053591612,-22.8742356128083,
12.259716988749));
#92059=CARTESIAN_POINT('Ctrl Pts',(-8.37377637083519,-22.8742356128002,
12.2454010901265));
#92060=CARTESIAN_POINT('Ctrl Pts',(-8.36170335091807,-22.8742356128,12.2320541243705));
#92061=CARTESIAN_POINT('Ctrl Pts',(-8.34854625295,-22.8742356128,12.2198888201));
#92062=CARTESIAN_POINT('',(-8.31471092647,-21.0742356128,12.6874600337));
#92063=CARTESIAN_POINT('Origin',(-8.14487887576,-21.0742356128,12.4401604693));
#92064=CARTESIAN_POINT('',(-8.31471092647,-22.5742356128,12.6874600337));
#92065=CARTESIAN_POINT('Origin',(-1.05,-21.9742356128,14.92922515));
#92066=CARTESIAN_POINT('',(-1.07189396011,-22.8742356128,15.2284251743));
#92067=CARTESIAN_POINT('Origin',(-1.05,-22.8742356128,14.92922515));
#92068=CARTESIAN_POINT('',(-1.07189396011,-21.0742356128,15.2284251743));
#92069=CARTESIAN_POINT('',(-1.07189396011,-22.5742356128,15.2284251743));
#92070=CARTESIAN_POINT('Origin',(-1.05,-21.0742356128,14.92922515));
#92071=CARTESIAN_POINT('Origin',(2.4183046301E-16,-21.2742356128,0.580061096523));
#92072=CARTESIAN_POINT('Origin',(2.71042223425E-15,-22.8742356128,0.580061096523));
#92073=CARTESIAN_POINT('Origin',(-1.51003344041E-15,-21.0742356128,0.580061096523));
#92074=CARTESIAN_POINT('Origin',(-0.45,-22.8742356128,2.93538176615));
#92075=CARTESIAN_POINT('',(-0.75,-22.8742356128,-6.23438845923));
#92076=CARTESIAN_POINT('Origin',(-0.45,-22.8742356128,-6.23438845923));
#92077=CARTESIAN_POINT('',(-0.45,-23.1742356128,-4.99584562937));
#92078=CARTESIAN_POINT('',(-0.45,-23.1742356128,-5.6151170443));
#92079=CARTESIAN_POINT('',(-0.75,-22.8742356128,-4.99584562937));
#92080=CARTESIAN_POINT('Origin',(-0.45,-22.8742356128,-4.99584562937));
#92081=CARTESIAN_POINT('',(-0.75,-22.8742356128,-5.6151170443));
#92082=CARTESIAN_POINT('Origin',(-7.40416713263E-16,-22.8742356128,0.729452270839));
#92083=CARTESIAN_POINT('',(-0.935307608221,-23.1742356128,5.53218022249));
#92084=CARTESIAN_POINT('',(-0.992653804111,-22.8742356128,5.82664824081));
#92085=CARTESIAN_POINT('Origin',(-0.935307608221,-22.8742356128,5.53218022249));
#92086=CARTESIAN_POINT('',(-1.19254592572,-22.8742356128,5.78361912069));
#92087=CARTESIAN_POINT('Origin',(3.67394039744E-17,-22.8742356128,0.729452270839));
#92088=CARTESIAN_POINT('',(-1.12365184404,-23.1742356128,5.49163692002));
#92089=CARTESIAN_POINT('Origin',(-1.12365184404,-22.8742356128,5.49163692002));
#92090=CARTESIAN_POINT('Origin',(-3.42702565972E-16,-23.1742356128,0.729452270839));
#92091=CARTESIAN_POINT('Origin',(-1.05,-22.8742356128,6.12111625914));
#92092=CARTESIAN_POINT('',(-0.45,-23.1742356128,6.12111625914));
#92093=CARTESIAN_POINT('',(-0.75,-22.8742356128,6.12111625914));
#92094=CARTESIAN_POINT('Origin',(-0.45,-22.8742356128,6.12111625914));
#92095=CARTESIAN_POINT('Origin',(-1.05,-22.8742356128,6.12111625914));
#92096=CARTESIAN_POINT('Origin',(-1.05,-23.1742356128,6.12111625914));
#92097=CARTESIAN_POINT('Origin',(-0.45,-22.8742356128,2.93538176615));
#92098=CARTESIAN_POINT('',(-0.45,-23.1742356128,9.0358656718));
#92099=CARTESIAN_POINT('',(-0.75,-22.8742356128,9.0358656718));
#92100=CARTESIAN_POINT('Origin',(-0.45,-22.8742356128,9.0358656718));
#92101=CARTESIAN_POINT('',(-0.75,-22.8742356128,7.57849096547));
#92102=CARTESIAN_POINT('',(-0.45,-23.1742356128,7.57849096547));
#92103=CARTESIAN_POINT('Origin',(-1.05,-22.8742356128,9.0358656718));
#92104=CARTESIAN_POINT('',(-1.15397857793,-23.1742356128,9.62678737163));
#92105=CARTESIAN_POINT('',(-1.10198928897,-22.8742356128,9.33132652171));
#92106=CARTESIAN_POINT('Origin',(-1.15397857793,-22.8742356128,9.62678737163));
#92107=CARTESIAN_POINT('Origin',(-1.05,-22.8742356128,9.0358656718));
#92108=CARTESIAN_POINT('Origin',(-1.05,-23.1742356128,9.0358656718));
#92109=CARTESIAN_POINT('Origin',(-0.00234331738835,-22.8742356128,3.08191746407));
#92110=CARTESIAN_POINT('',(-3.7572334818,-23.1742356128,8.56483509371));
#92111=CARTESIAN_POINT('',(-3.58772315463,-22.8742356128,8.31731489457));
#92112=CARTESIAN_POINT('Origin',(-3.7572334818,-22.8742356128,8.56483509371));
#92113=CARTESIAN_POINT('Origin',(-0.00234331738835,-22.8742356128,3.08191746407));
#92114=CARTESIAN_POINT('Origin',(-0.00234331738835,-23.1742356128,3.08191746407));
#92115=CARTESIAN_POINT('Origin',(-1.2614400074,-22.8742356128,6.07560132137));
#92116=CARTESIAN_POINT('',(-1.46510738459,-22.8742356128,5.8553296721));
#92117=CARTESIAN_POINT('Origin',(-1.2614400074,-22.8742356128,6.07560132137));
#92118=CARTESIAN_POINT('',(-1.66877476178,-23.1742356128,5.63505802284));
#92119=CARTESIAN_POINT('Origin',(-1.66877476178,-22.8742356128,5.63505802284));
#92120=CARTESIAN_POINT('Origin',(-1.2614400074,-23.1742356128,6.07560132137));
#92121=CARTESIAN_POINT('Origin',(-3.41821282746,-22.8742356128,8.06979469543));
#92122=CARTESIAN_POINT('',(-3.82554758184,-23.1742356128,7.6292513969));
#92123=CARTESIAN_POINT('',(-3.62188020465,-22.8742356128,7.84952304616));
#92124=CARTESIAN_POINT('Origin',(-3.82554758184,-22.8742356128,7.6292513969));
#92125=CARTESIAN_POINT('Origin',(-3.41821282746,-22.8742356128,8.06979469543));
#92126=CARTESIAN_POINT('Origin',(-3.41821282746,-23.1742356128,8.06979469543));
#92127=CARTESIAN_POINT('Origin',(-6.6707290414,-22.8742356128,10.2599605573));
#92128=CARTESIAN_POINT('',(-2.54349379462,-22.8742356128,6.85242635913));
#92129=CARTESIAN_POINT('',(-2.74716117181,-23.1742356128,6.63215470987));
#92130=CARTESIAN_POINT('Origin',(-0.00234331738835,-22.8742356128,3.08191746407));
#92131=CARTESIAN_POINT('',(-6.21380646358,-22.8742356128,1.78497474518));
#92132=CARTESIAN_POINT('',(-6.50747329887,-23.1742356128,1.72365761992));
#92133=CARTESIAN_POINT('Origin',(-6.50747329887,-22.8742356128,1.72365761992));
#92134=CARTESIAN_POINT('',(-6.03449750111,-23.1742356128,0.293602240855));
#92135=CARTESIAN_POINT('Origin',(-0.00234331738835,-23.1742356128,3.08191746407));
#92136=CARTESIAN_POINT('',(-5.76218263052,-22.8742356128,0.419477620705));
#92137=CARTESIAN_POINT('Origin',(-6.03449750111,-22.8742356128,0.293602240855));
#92138=CARTESIAN_POINT('Origin',(-0.00234331738835,-22.8742356128,3.08191746407));
#92139=CARTESIAN_POINT('Ctrl Pts',(-4.88987240374,-23.1742356097,0.542992178472));
#92140=CARTESIAN_POINT('Ctrl Pts',(-4.86084787859,-23.1742356067,0.555014532813));
#92141=CARTESIAN_POINT('Ctrl Pts',(-4.83182335285,-23.1618986036,0.567036885942));
#92142=CARTESIAN_POINT('Ctrl Pts',(-4.80888237522,-23.137067473,0.576539351728));
#92143=CARTESIAN_POINT('Ctrl Pts',(-4.79748446133,-23.1056515569,0.581260521919));
#92144=CARTESIAN_POINT('Ctrl Pts',(-4.79748444899,-23.0742356355,0.58126052593));
#92145=CARTESIAN_POINT('Ctrl Pts',(-4.89332536714,-23.1742356121,0.548536687929));
#92146=CARTESIAN_POINT('Ctrl Pts',(-4.86410343804,-23.1745712361,0.560640808584));
#92147=CARTESIAN_POINT('Ctrl Pts',(-4.83473862243,-23.1624020478,0.572744367244));
#92148=CARTESIAN_POINT('Ctrl Pts',(-4.81143971624,-23.1374948049,0.582274826956));
#92149=CARTESIAN_POINT('Ctrl Pts',(-4.79983297467,-23.1058652194,0.58693034427));
#92150=CARTESIAN_POINT('Ctrl Pts',(-4.79977917182,-23.07423563,0.586800476896));
#92151=CARTESIAN_POINT('Ctrl Pts',(-4.89674616735,-23.1741819495,0.554055341853));
#92152=CARTESIAN_POINT('Ctrl Pts',(-4.86733644658,-23.174853061,0.566241584166));
#92153=CARTESIAN_POINT('Ctrl Pts',(-4.83763986632,-23.1628553414,0.578430209837));
#92154=CARTESIAN_POINT('Ctrl Pts',(-4.81398926394,-23.1378767526,0.587995632443));
#92155=CARTESIAN_POINT('Ctrl Pts',(-4.80217889215,-23.1060383,0.59259390235));
#92156=CARTESIAN_POINT('Ctrl Pts',(-4.80207503274,-23.0741998456,0.592343175471));
#92157=CARTESIAN_POINT('Ctrl Pts',(-4.90013262037,-23.1740815975,0.559548447604));
#92158=CARTESIAN_POINT('Ctrl Pts',(-4.87054456006,-23.1750868242,0.571816367149));
#92159=CARTESIAN_POINT('Ctrl Pts',(-4.84052526678,-23.1632633043,0.584093271995));
#92160=CARTESIAN_POINT('Ctrl Pts',(-4.816529999,-23.1382178393,0.593700396416));
#92161=CARTESIAN_POINT('Ctrl Pts',(-4.8045217228,-23.1061753876,0.59825000772));
#92162=CARTESIAN_POINT('Ctrl Pts',(-4.80437168194,-23.074132936,0.597887777111));
#92163=CARTESIAN_POINT('Ctrl Pts',(-4.9034828985,-23.1739412939,0.565017049189));
#92164=CARTESIAN_POINT('Ctrl Pts',(-4.87372566794,-23.1752779938,0.577365441326));
#92165=CARTESIAN_POINT('Ctrl Pts',(-4.84339318826,-23.1636304163,0.589733124501));
#92166=CARTESIAN_POINT('Ctrl Pts',(-4.81906111591,-23.1385222645,0.599388337029));
#92167=CARTESIAN_POINT('Ctrl Pts',(-4.80686117712,-23.1062808323,0.603897950179));
#92168=CARTESIAN_POINT('Ctrl Pts',(-4.80666892648,-23.0740394002,0.603433816048));
#92169=CARTESIAN_POINT('',(-4.90348289994913,-23.1739412934337,0.565017049040251));
#92170=CARTESIAN_POINT('Origin',(-4.8983948094157,-23.0747913407119,0.56545239354252));
#92171=CARTESIAN_POINT('',(-4.88987240399273,-23.17423561125,0.542992182694935));
#92172=CARTESIAN_POINT('Ctrl Pts',(-4.9034828985,-23.1739412939,0.565017049189));
#92173=CARTESIAN_POINT('Ctrl Pts',(-4.89901586077995,-23.1741283653771,
0.557725581051751));
#92174=CARTESIAN_POINT('Ctrl Pts',(-4.89447635549808,-23.1742356128882,
0.550384858685629));
#92175=CARTESIAN_POINT('Ctrl Pts',(-4.88987240449,-23.1742356097,0.542992182489001));
#92176=CARTESIAN_POINT('Origin',(-4.8892191322679,-23.0749427012436,0.543262776949538));
#92177=CARTESIAN_POINT('Origin',(-5.48986775992,-22.8742356128,0.545353000555));
#92178=CARTESIAN_POINT('',(-5.1900363009,-22.8742356128,0.55540766038));
#92179=CARTESIAN_POINT('Origin',(-4.89020484189,-22.8742356128,0.565462320206));
#92180=CARTESIAN_POINT('Origin',(-5.48986775992,-22.8742356128,0.545353000555));
#92181=CARTESIAN_POINT('Origin',(-5.48986775992,-23.1742356128,0.545353000555));
#92182=CARTESIAN_POINT('Ctrl Pts',(-4.91026666705,-23.1735877712,0.882730576443));
#92183=CARTESIAN_POINT('Ctrl Pts',(-4.88018105031,-23.1755928789,0.870218178727));
#92184=CARTESIAN_POINT('Ctrl Pts',(-4.84922086626,-23.1643051888,0.857678480686));
#92185=CARTESIAN_POINT('Ctrl Pts',(-4.82420272303,-23.13907693,0.847951337039));
#92186=CARTESIAN_POINT('Ctrl Pts',(-4.81160444157,-23.1064403276,0.843555347761));
#92187=CARTESIAN_POINT('Ctrl Pts',(-4.81131367923,-23.073803724,0.844257300549));
#92188=CARTESIAN_POINT('Ctrl Pts',(-4.90607244846,-23.1738495633,0.889624687643));
#92189=CARTESIAN_POINT('Ctrl Pts',(-4.87618496465,-23.1754360605,0.877215340784));
#92190=CARTESIAN_POINT('Ctrl Pts',(-4.84561274758,-23.1639199413,0.864783368054));
#92191=CARTESIAN_POINT('Ctrl Pts',(-4.82102256688,-23.1387632801,0.855100421724));
#92192=CARTESIAN_POINT('Ctrl Pts',(-4.80867334759,-23.1063707663,0.8506316329));
#92193=CARTESIAN_POINT('Ctrl Pts',(-4.80844479873,-23.0739782513,0.85118339076));
#92194=CARTESIAN_POINT('Ctrl Pts',(-4.90188345783,-23.1740438603,0.89651618735));
#92195=CARTESIAN_POINT('Ctrl Pts',(-4.87220155195,-23.1752205389,0.884207133034));
#92196=CARTESIAN_POINT('Ctrl Pts',(-4.84201706368,-23.1634854888,0.871880564251));
#92197=CARTESIAN_POINT('Ctrl Pts',(-4.81784840655,-23.1384044972,0.862242184947));
#92198=CARTESIAN_POINT('Ctrl Pts',(-4.80574358799,-23.1062561396,0.857704695525));
#92199=CARTESIAN_POINT('Ctrl Pts',(-4.80557512116,-23.0741077812,0.85811140527));
#92200=CARTESIAN_POINT('Ctrl Pts',(-4.89770009156,-23.1741721033,0.903404516156));
#92201=CARTESIAN_POINT('Ctrl Pts',(-4.86823079014,-23.1749477659,0.891193246426));
#92202=CARTESIAN_POINT('Ctrl Pts',(-4.83843359789,-23.1630030668,0.878969965755));
#92203=CARTESIAN_POINT('Ctrl Pts',(-4.81468020651,-23.1380016463,0.869376522739));
#92204=CARTESIAN_POINT('Ctrl Pts',(-4.802815301,-23.1060974606,0.864774202654));
#92205=CARTESIAN_POINT('Ctrl Pts',(-4.80270489088,-23.0741932746,0.865040754137));
#92206=CARTESIAN_POINT('Ctrl Pts',(-4.89352269524,-23.1742356128,0.91028919283));
#92207=CARTESIAN_POINT('Ctrl Pts',(-4.86427263762,-23.1746190563,0.898173422263));
#92208=CARTESIAN_POINT('Ctrl Pts',(-4.83486214645,-23.162473773,0.886051492275));
#92209=CARTESIAN_POINT('Ctrl Pts',(-4.81151792338,-23.1375556813,0.876503354045));
#92210=CARTESIAN_POINT('Ctrl Pts',(-4.79988860489,-23.1058956471,0.871839869986));
#92211=CARTESIAN_POINT('Ctrl Pts',(-4.79983432123,-23.0742356128,0.871970922337));
#92212=CARTESIAN_POINT('Ctrl Pts',(-4.88935151015,-23.1742356128,0.917169903738));
#92213=CARTESIAN_POINT('Ctrl Pts',(-4.86032697863,-23.1742356128,0.90514754914));
#92214=CARTESIAN_POINT('Ctrl Pts',(-4.83130244711,-23.1618986073,0.893125194543));
#92215=CARTESIAN_POINT('Ctrl Pts',(-4.80836146378,-23.1370674659,0.883622728112));
#92216=CARTESIAN_POINT('Ctrl Pts',(-4.7969635569,-23.1056515394,0.878901560502));
#92217=CARTESIAN_POINT('Ctrl Pts',(-4.7969635569,-23.0742356128,0.878901560502));
#92218=CARTESIAN_POINT('',(-4.88935151015,-23.1742356128,0.917169903738));
#92219=CARTESIAN_POINT('Origin',(-4.88869823765389,-23.0749427099031,0.916899309412879));
#92220=CARTESIAN_POINT('',(-4.91026667169405,-23.1735877810644,0.882730576328867));
#92221=CARTESIAN_POINT('Origin',(-4.78300704958758,-22.686919287924,1.13838380064551));
#92222=CARTESIAN_POINT('Origin',(-4.90303610019935,-23.0745775166647,0.882230481220324));
#92223=CARTESIAN_POINT('Ctrl Pts',(-4.91032411032826,-23.1735838288474,
0.882801380280842));
#92224=CARTESIAN_POINT('Ctrl Pts',(-4.88022671384046,-23.1756160163728,
0.870279875408482));
#92225=CARTESIAN_POINT('Ctrl Pts',(-4.84924393654162,-23.1643433388717,
0.857726517801697));
#92226=CARTESIAN_POINT('Ctrl Pts',(-4.82420252529952,-23.1391099370352,
0.847986365762712));
#92227=CARTESIAN_POINT('Ctrl Pts',(-4.81159271910536,-23.1064573061117,
0.843583836626828));
#92228=CARTESIAN_POINT('Ctrl Pts',(-4.81130199410985,-23.0738046752881,
0.844285506864908));
#92229=CARTESIAN_POINT('Ctrl Pts',(-4.94434742826404,-23.171453756981,0.826898793291758));
#92230=CARTESIAN_POINT('Ctrl Pts',(-4.91067807699736,-23.1770055230639,
0.818105216460323));
#92231=CARTESIAN_POINT('Ctrl Pts',(-4.87457600571307,-23.167652358011,0.809242452726758));
#92232=CARTESIAN_POINT('Ctrl Pts',(-4.8445619038014,-23.1418126887911,0.802685366669083));
#92233=CARTESIAN_POINT('Ctrl Pts',(-4.8293242397813,-23.1071017824707,0.800486968739525));
#92234=CARTESIAN_POINT('Ctrl Pts',(-4.82875126200463,-23.0723908765014,
0.802171370483634));
#92235=CARTESIAN_POINT('Ctrl Pts',(-4.96420776206773,-23.1658532222896,
0.763665118766352));
#92236=CARTESIAN_POINT('Ctrl Pts',(-4.92841514195084,-23.174432018286,0.760045081408559));
#92237=CARTESIAN_POINT('Ctrl Pts',(-4.88880992409556,-23.1670369908996,
0.756370657617406));
#92238=CARTESIAN_POINT('Ctrl Pts',(-4.85536837092642,-23.1410196792605,
0.753866960469878));
#92239=CARTESIAN_POINT('Ctrl Pts',(-4.83885806030122,-23.1048418671394,
0.753535150521697));
#92240=CARTESIAN_POINT('Ctrl Pts',(-4.83896248410945,-23.0686637734685,
0.754906483839526));
#92241=CARTESIAN_POINT('Ctrl Pts',(-4.9642104382863,-23.1658530695551,0.695241429168574));
#92242=CARTESIAN_POINT('Ctrl Pts',(-4.92841670517027,-23.1744321920304,
0.698861429442802));
#92243=CARTESIAN_POINT('Ctrl Pts',(-4.88881020696589,-23.1670369970505,
0.702535807890803));
#92244=CARTESIAN_POINT('Ctrl Pts',(-4.85536781453051,-23.141018906302,0.705039301384199));
#92245=CARTESIAN_POINT('Ctrl Pts',(-4.83885769137182,-23.1048402717239,
0.705370657456912));
#92246=CARTESIAN_POINT('Ctrl Pts',(-4.83896308256911,-23.0686617900272,
0.703998762393385));
#92247=CARTESIAN_POINT('Ctrl Pts',(-4.94434734509692,-23.1714537621886,
0.632005686936182));
#92248=CARTESIAN_POINT('Ctrl Pts',(-4.91067802717319,-23.1770055181565,
0.640799265178577));
#92249=CARTESIAN_POINT('Ctrl Pts',(-4.87457599443822,-23.167652357672,0.649662030565025));
#92250=CARTESIAN_POINT('Ctrl Pts',(-4.84456191778467,-23.1418127111943,
0.656219122931779));
#92251=CARTESIAN_POINT('Ctrl Pts',(-4.82932424873922,-23.107101829449,0.658417534179115));
#92252=CARTESIAN_POINT('Ctrl Pts',(-4.82875124236076,-23.0723909352002,
0.656733148919665));
#92253=CARTESIAN_POINT('Ctrl Pts',(-4.91032411262656,-23.1735838286412,
0.576103162589323));
#92254=CARTESIAN_POINT('Ctrl Pts',(-4.88022671491257,-23.1756160164777,
0.588624667473674));
#92255=CARTESIAN_POINT('Ctrl Pts',(-4.84924393621136,-23.1643433387761,
0.601178025081577));
#92256=CARTESIAN_POINT('Ctrl Pts',(-4.82420252410613,-23.1391099360228,
0.61091817693581));
#92257=CARTESIAN_POINT('Ctrl Pts',(-4.81159271820302,-23.1064573042801,
0.615320705592525));
#92258=CARTESIAN_POINT('Ctrl Pts',(-4.81130199435762,-23.0738046729465,
0.614619034738959));
#92259=CARTESIAN_POINT('',(-4.91026668200588,-23.1735877855957,0.576173964916216));
#92260=CARTESIAN_POINT('Ctrl Pts',(-4.91026667429727,-23.1735877859444,
0.882730577727296));
#92261=CARTESIAN_POINT('Ctrl Pts',(-4.91879411776458,-23.1730555309431,
0.868713877246766));
#92262=CARTESIAN_POINT('Ctrl Pts',(-4.92622758773466,-23.1722660176644,
0.854117529858202));
#92263=CARTESIAN_POINT('Ctrl Pts',(-4.93243211502344,-23.171462420821,0.839089304309771));
#92264=CARTESIAN_POINT('Ctrl Pts',(-4.93811142443016,-23.1707268490523,
0.825333229309873));
#92265=CARTESIAN_POINT('Ctrl Pts',(-4.9427623803931,-23.1699802976463,0.811215540434539));
#92266=CARTESIAN_POINT('Ctrl Pts',(-4.94629784193977,-23.1693715096677,
0.796856553293824));
#92267=CARTESIAN_POINT('Ctrl Pts',(-4.94857306719722,-23.1689797277838,
0.787615912494103));
#92268=CARTESIAN_POINT('Ctrl Pts',(-4.95038657496731,-23.1686442133483,
0.778275464280113));
#92269=CARTESIAN_POINT('Ctrl Pts',(-4.95171571795756,-23.1683929962434,
0.768868428703813));
#92270=CARTESIAN_POINT('Ctrl Pts',(-4.95361365836277,-23.1680342725415,
0.7554357182697));
#92271=CARTESIAN_POINT('Ctrl Pts',(-4.95454013240377,-23.1678467144829,
0.741880779640089));
#92272=CARTESIAN_POINT('Ctrl Pts',(-4.95448697348868,-23.1678572110641,
0.7283291771088));
#92273=CARTESIAN_POINT('Ctrl Pts',(-4.95447471934027,-23.1678596307272,
0.725205273086987));
#92274=CARTESIAN_POINT('Ctrl Pts',(-4.95441038067712,-23.1678723584511,
0.722081549228793));
#92275=CARTESIAN_POINT('Ctrl Pts',(-4.95429380538934,-23.1678953318367,
0.718959547665966));
#92276=CARTESIAN_POINT('Ctrl Pts',(-4.9537680339869,-23.1679989451272,0.70487886923606));
#92277=CARTESIAN_POINT('Ctrl Pts',(-4.95214944036737,-23.1683220299151,
0.690852161339055));
#92278=CARTESIAN_POINT('Ctrl Pts',(-4.94950342663415,-23.1688041380817,
0.676996407633137));
#92279=CARTESIAN_POINT('Ctrl Pts',(-4.94672280729924,-23.1693107716162,
0.662435796638999));
#92280=CARTESIAN_POINT('Ctrl Pts',(-4.94280686905793,-23.1699924763006,
0.648064082382267));
#92281=CARTESIAN_POINT('Ctrl Pts',(-4.93782902584385,-23.1707193115796,
0.6340127869156));
#92282=CARTESIAN_POINT('Ctrl Pts',(-4.93252157779082,-23.1714942738113,
0.619031093527582));
#92283=CARTESIAN_POINT('Ctrl Pts',(-4.92600560665533,-23.1723197923502,
0.604413876753238));
#92284=CARTESIAN_POINT('Ctrl Pts',(-4.91838360323196,-23.1729819475197,
0.590313280824429));
#92285=CARTESIAN_POINT('Ctrl Pts',(-4.91580296743621,-23.173206138095,0.585539141982699));
#92286=CARTESIAN_POINT('Ctrl Pts',(-4.91309574645361,-23.173411204469,0.580824151361539));
#92287=CARTESIAN_POINT('Ctrl Pts',(-4.91026668277928,-23.173587785389,0.576173965249023));
#92288=CARTESIAN_POINT('Origin',(-4.90303611057442,-23.0745775160784,0.576674065905074));
#92289=CARTESIAN_POINT('Ctrl Pts',(-4.90348290199,-23.1739412927,0.565017048926));
#92290=CARTESIAN_POINT('Ctrl Pts',(-4.87372566996,-23.1752779928,0.577365441579));
#92291=CARTESIAN_POINT('Ctrl Pts',(-4.84339318716,-23.1636304143,0.589733124946));
#92292=CARTESIAN_POINT('Ctrl Pts',(-4.81906111615,-23.1385222628,0.599388337346));
#92293=CARTESIAN_POINT('Ctrl Pts',(-4.80686117638,-23.1062808303,0.603897950601));
#92294=CARTESIAN_POINT('Ctrl Pts',(-4.80666892647,-23.0740393981,0.603433816023));
#92295=CARTESIAN_POINT('Ctrl Pts',(-4.90574226327,-23.1738467182,0.568735011834));
#92296=CARTESIAN_POINT('Ctrl Pts',(-4.87587305899,-23.175403149,0.581137165172));
#92297=CARTESIAN_POINT('Ctrl Pts',(-4.84533146364,-23.163872265,0.593561421472));
#92298=CARTESIAN_POINT('Ctrl Pts',(-4.82077291013,-23.13872269,0.603240740434));
#92299=CARTESIAN_POINT('Ctrl Pts',(-4.80844177844,-23.1063495195,0.607713860274));
#92300=CARTESIAN_POINT('Ctrl Pts',(-4.80821741307,-23.0739763492,0.607172193377));
#92301=CARTESIAN_POINT('Ctrl Pts',(-4.90800356168,-23.1737290414,0.572454037538));
#92302=CARTESIAN_POINT('Ctrl Pts',(-4.87802484771,-23.1755082749,0.584910832115));
#92303=CARTESIAN_POINT('Ctrl Pts',(-4.84727399761,-23.164097327,0.597392404899));
#92304=CARTESIAN_POINT('Ctrl Pts',(-4.82248677013,-23.1389076984,0.607095701029));
#92305=CARTESIAN_POINT('Ctrl Pts',(-4.81002287785,-23.1064027985,0.611530970941));
#92306=CARTESIAN_POINT('Ctrl Pts',(-4.80976568781,-23.0738978985,0.610910059239));
#92307=CARTESIAN_POINT('Ctrl Pts',(-4.91026668053,-23.173587786,0.576173964221));
#92308=CARTESIAN_POINT('Ctrl Pts',(-4.88018105713,-23.1755928936,0.588686362821));
#92309=CARTESIAN_POINT('Ctrl Pts',(-4.84922086635,-23.164305202,0.601226061781));
#92310=CARTESIAN_POINT('Ctrl Pts',(-4.82420271933,-23.1390769396,0.610953205986));
#92311=CARTESIAN_POINT('Ctrl Pts',(-4.81160443804,-23.1064403339,0.615349194972));
#92312=CARTESIAN_POINT('Ctrl Pts',(-4.81131367927,-23.0738037283,0.614647241211));
#92313=CARTESIAN_POINT('Ctrl Pts',(-4.91026668053,-23.173587786,0.576173964221));
#92314=CARTESIAN_POINT('Ctrl Pts',(-4.90800356173676,-23.1737290413966,
0.572454037692303));
#92315=CARTESIAN_POINT('Ctrl Pts',(-4.90574226337073,-23.1738467181957,
0.568735011999752));
#92316=CARTESIAN_POINT('Ctrl Pts',(-4.90348290200454,-23.1739412926994,
0.56501704894993));
#92317=CARTESIAN_POINT('Origin',(3.67394039744E-17,-22.8742356128,0.729452270839));
#92318=CARTESIAN_POINT('',(-4.79074910795,-23.1742356128,1.72429853244));
#92319=CARTESIAN_POINT('Origin',(-3.42702565972E-16,-23.1742356128,0.729452270839));
#92320=CARTESIAN_POINT('',(-5.08448267152,-22.8742356128,1.78529520144));
#92321=CARTESIAN_POINT('Origin',(-4.79074910795,-22.8742356128,1.72429853244));
#92322=CARTESIAN_POINT('Origin',(3.67394039744E-17,-22.8742356128,0.729452270839));
#92323=CARTESIAN_POINT('Origin',(-5.92013962829,-22.8742356128,1.84629187045));
#92324=CARTESIAN_POINT('',(-5.92013962829,-22.8742356128,2.14629187045));
#92325=CARTESIAN_POINT('',(-5.92013962829,-23.1742356128,2.44629187045));
#92326=CARTESIAN_POINT('Origin',(-5.92013962829,-22.8742356128,2.44629187045));
#92327=CARTESIAN_POINT('Origin',(-5.92013962829,-23.1742356128,1.84629187045));
#92328=CARTESIAN_POINT('Origin',(-5.92013962829,-22.8742356128,1.84629187045));
#92329=CARTESIAN_POINT('Origin',(-5.3782162351,-22.8742356128,1.84629187045));
#92330=CARTESIAN_POINT('',(-5.3782162351,-23.1742356128,2.44629187045));
#92331=CARTESIAN_POINT('Origin',(-5.3782162351,-23.1742356128,1.84629187045));
#92332=CARTESIAN_POINT('',(-5.3782162351,-22.8742356128,2.14629187045));
#92333=CARTESIAN_POINT('Origin',(-5.3782162351,-22.8742356128,2.44629187045));
#92334=CARTESIAN_POINT('Origin',(-5.3782162351,-22.8742356128,1.84629187045));
#92335=CARTESIAN_POINT('Origin',(-6.6707290414,-22.8742356128,2.44629187045));
#92336=CARTESIAN_POINT('',(-5.6491779317,-23.1742356128,2.44629187045));
#92337=CARTESIAN_POINT('',(-5.6491779317,-22.8742356128,2.14629187045));
#92338=CARTESIAN_POINT('Ctrl Pts',(-3.36369872841,-23.1735877712,4.30991925785));
#92339=CARTESIAN_POINT('Ctrl Pts',(-3.35127258606,-23.1755928789,4.27979791296));
#92340=CARTESIAN_POINT('Ctrl Pts',(-3.33824733549,-23.1643051888,4.24903885135));
#92341=CARTESIAN_POINT('Ctrl Pts',(-3.327434966,-23.13907693,4.22447022338));
#92342=CARTESIAN_POINT('Ctrl Pts',(-3.32163506958,-23.1064403276,4.21245345931));
#92343=CARTESIAN_POINT('Ctrl Pts',(-3.32093311398,-23.073803724,4.21274421486));
#92344=CARTESIAN_POINT('Ctrl Pts',(-3.35585809522,-23.1738495633,4.31182837022));
#92345=CARTESIAN_POINT('Ctrl Pts',(-3.34349918606,-23.1754360605,4.28191999443));
#92346=CARTESIAN_POINT('Ctrl Pts',(-3.33067209627,-23.1639199413,4.2515114402));
#92347=CARTESIAN_POINT('Ctrl Pts',(-3.32013108976,-23.1387632801,4.22727667967));
#92348=CARTESIAN_POINT('Ctrl Pts',(-3.31455878394,-23.1063707663,4.21538455208));
#92349=CARTESIAN_POINT('Ctrl Pts',(-3.31400702377,-23.0739782513,4.21561309536));
#92350=CARTESIAN_POINT('Ctrl Pts',(-3.34802300536,-23.1740438603,4.31373933271));
#92351=CARTESIAN_POINT('Ctrl Pts',(-3.33573854421,-23.1752205389,4.28404724001));
#92352=CARTESIAN_POINT('Ctrl Pts',(-3.32311108825,-23.1634854888,4.2539873833));
#92353=CARTESIAN_POINT('Ctrl Pts',(-3.31283663026,-23.1384044972,4.23008219858));
#92354=CARTESIAN_POINT('Ctrl Pts',(-3.30748572051,-23.1062561396,4.21831430975));
#92355=CARTESIAN_POINT('Ctrl Pts',(-3.30707900926,-23.0741077812,4.21848277293));
#92356=CARTESIAN_POINT('Ctrl Pts',(-3.34019413469,-23.1741721033,4.31565203007));
#92357=CARTESIAN_POINT('Ctrl Pts',(-3.32799086345,-23.1749477659,4.28617941556));
#92358=CARTESIAN_POINT('Ctrl Pts',(-3.31556423141,-23.1630030668,4.25646645421));
#92359=CARTESIAN_POINT('Ctrl Pts',(-3.3055516359,-23.1380016463,4.23288668148));
#92360=CARTESIAN_POINT('Ctrl Pts',(-3.30041621249,-23.1060974606,4.22124259459));
#92361=CARTESIAN_POINT('Ctrl Pts',(-3.30014966039,-23.0741932746,4.22135300321));
#92362=CARTESIAN_POINT('Ctrl Pts',(-3.33237206787,-23.1742356128,4.31756636636));
#92363=CARTESIAN_POINT('Ctrl Pts',(-3.3202562973,-23.1746190563,4.28831630874));
#92364=CARTESIAN_POINT('Ctrl Pts',(-3.30803143845,-23.162473773,4.2589484521));
#92365=CARTESIAN_POINT('Ctrl Pts',(-3.29827613331,-23.1375556813,4.23569004038));
#92366=CARTESIAN_POINT('Ctrl Pts',(-3.29335054454,-23.1058956471,4.22416928921));
#92367=CARTESIAN_POINT('Ctrl Pts',(-3.29321949219,-23.0742356128,4.22422357287));
#92368=CARTESIAN_POINT('Ctrl Pts',(-3.32455719726,-23.1742356128,4.31948229044));
#92369=CARTESIAN_POINT('Ctrl Pts',(-3.31253484266,-23.1742356128,4.29045775892));
#92370=CARTESIAN_POINT('Ctrl Pts',(-3.30051248807,-23.1618986073,4.2614332274));
#92371=CARTESIAN_POINT('Ctrl Pts',(-3.29101002164,-23.1370674659,4.23849224407));
#92372=CARTESIAN_POINT('Ctrl Pts',(-3.28628885403,-23.1056515394,4.22709433719));
#92373=CARTESIAN_POINT('Ctrl Pts',(-3.28628885403,-23.0742356128,4.22709433719));
#92374=CARTESIAN_POINT('',(-3.32455719726,-23.1742356128,4.31948229044));
#92375=CARTESIAN_POINT('Origin',(-3.32428660293348,-23.0749427099053,4.31882901794046));
#92376=CARTESIAN_POINT('',(-3.36369873177259,-23.1735877810642,4.30991926105255));
#92377=CARTESIAN_POINT('Origin',(-3.09293905505095,-22.6869204620332,4.40070704808497));
#92378=CARTESIAN_POINT('Origin',(-3.3589395662952,-23.0745775166517,4.30445285428866));
#92379=CARTESIAN_POINT('Ctrl Pts',(-3.36368928106124,-23.1735838288475,
4.31000994225207));
#92380=CARTESIAN_POINT('Ctrl Pts',(-3.35126124891729,-23.1756160163725,
4.27987382809444));
#92381=CARTESIAN_POINT('Ctrl Pts',(-3.33822968127554,-23.1643433388712,
4.2490891318676));
#92382=CARTESIAN_POINT('Ctrl Pts',(-3.32741005713184,-23.1391099370348,
4.22449485261762));
#92383=CARTESIAN_POINT('Ctrl Pts',(-3.32160663587613,-23.1064573061115,
4.21246531493779));
#92384=CARTESIAN_POINT('Ctrl Pts',(-3.32090490647545,-23.0738046752881,
4.2127558971094));
#92385=CARTESIAN_POINT('Ctrl Pts',(-3.42727649823542,-23.1714537569812,
4.29453896273396));
#92386=CARTESIAN_POINT('Ctrl Pts',(-3.40968666944009,-23.1770055230636,
4.26451313832345));
#92387=CARTESIAN_POINT('Ctrl Pts',(-3.39042557036629,-23.1676523580104,
4.23271819857054));
#92388=CARTESIAN_POINT('Ctrl Pts',(-3.37383895538399,-23.1418126887906,
4.20685846356792));
#92389=CARTESIAN_POINT('Ctrl Pts',(-3.36461880191793,-23.1071017824704,
4.19452930592906));
#92390=CARTESIAN_POINT('Ctrl Pts',(-3.36302259354816,-23.0723908765014,
4.1953152013499));
#92391=CARTESIAN_POINT('Ctrl Pts',(-3.48603283499412,-23.1658532222902,
4.26386937938429));
#92392=CARTESIAN_POINT('Ctrl Pts',(-3.46328338356492,-23.1744320182858,
4.23600042202927));
#92393=CARTESIAN_POINT('Ctrl Pts',(-3.43787647541882,-23.167036990899,4.20539709393266));
#92394=CARTESIAN_POINT('Ctrl Pts',(-3.41600010763765,-23.14101967926,4.17997996368029));
#92395=CARTESIAN_POINT('Ctrl Pts',(-3.40456018010292,-23.1048418671392,
4.1680707860097));
#92396=CARTESIAN_POINT('Ctrl Pts',(-3.40366433978954,-23.0686637734687,
4.16911430388931));
#92397=CARTESIAN_POINT('Ctrl Pts',(-3.5344175822824,-23.1658530695554,4.21548841685241));
#92398=CARTESIAN_POINT('Ctrl Pts',(-3.50654786413253,-23.1744321920302,
4.1927381521826));
#92399=CARTESIAN_POINT('Ctrl Pts',(-3.47594366275913,-23.1670369970499,
4.16733030664708));
#92400=CARTESIAN_POINT('Ctrl Pts',(-3.45052608305801,-23.1410189063015,
4.14545320139491));
#92401=CARTESIAN_POINT('Ctrl Pts',(-3.43861735888675,-23.1048402717236,
4.13401308548029));
#92402=CARTESIAN_POINT('Ctrl Pts',(-3.4396619580288,-23.0686617900272,4.13311753200938));
#92403=CARTESIAN_POINT('Ctrl Pts',(-3.56508667654552,-23.1714537621884,
4.15672866682488));
#92404=CARTESIAN_POINT('Ctrl Pts',(-3.53506087470362,-23.1770055181561,
4.13913886260155));
#92405=CARTESIAN_POINT('Ctrl Pts',(-3.50326596105016,-23.1676523576714,
4.1198777919475));
#92406=CARTESIAN_POINT('Ctrl Pts',(-3.4774062394318,-23.1418127111937,4.10329119928901));
#92407=CARTESIAN_POINT('Ctrl Pts',(-3.46507706882468,-23.1071018294486,
4.09407105167612));
#92408=CARTESIAN_POINT('Ctrl Pts',(-3.46586293236865,-23.0723909351999,
4.09247483475298));
#92409=CARTESIAN_POINT('Ctrl Pts',(-3.58055767219067,-23.1735838286411,
4.09314155437213));
#92410=CARTESIAN_POINT('Ctrl Pts',(-3.55042155715734,-23.1756160164775,
4.08071352136631));
#92411=CARTESIAN_POINT('Ctrl Pts',(-3.51963685995032,-23.1643433387759,
4.06768195273836));
#92412=CARTESIAN_POINT('Ctrl Pts',(-3.49504258020861,-23.1391099360226,
4.05686232785297));
#92413=CARTESIAN_POINT('Ctrl Pts',(-3.48301304307739,-23.1064573042799,
4.05105890645977));
#92414=CARTESIAN_POINT('Ctrl Pts',(-3.48330362649208,-23.0738046729463,
4.05035717743438));
#92415=CARTESIAN_POINT('',(-3.58046699781502,-23.1735877854623,4.09315100955954));
#92416=CARTESIAN_POINT('Ctrl Pts',(-3.36369873262431,-23.1735877859441,
4.30991926388135));
#92417=CARTESIAN_POINT('Ctrl Pts',(-3.37963984968545,-23.1730555309427,
4.3060377730225));
#92418=CARTESIAN_POINT('Ctrl Pts',(-3.39521728292792,-23.1722660176641,
4.30097285382577));
#92419=CARTESIAN_POINT('Ctrl Pts',(-3.41023110644254,-23.1714624208208,
4.29473355694982));
#92420=CARTESIAN_POINT('Ctrl Pts',(-3.42397399855252,-23.1707268490521,
4.28902242122716));
#92421=CARTESIAN_POINT('Ctrl Pts',(-3.43724543459262,-23.1699802976461,
4.28232843018724));
#92422=CARTESIAN_POINT('Ctrl Pts',(-3.44989872060649,-23.1693715096676,
4.27467504184132));
#92423=CARTESIAN_POINT('Ctrl Pts',(-3.4580416675809,-23.1689797277841,4.26974974928039));
#92424=CARTESIAN_POINT('Ctrl Pts',(-3.46592870548895,-23.1686442133489,
4.26442739865431));
#92425=CARTESIAN_POINT('Ctrl Pts',(-3.4735203301526,-23.1683929962441,4.25871546603301));
#92426=CARTESIAN_POINT('Ctrl Pts',(-3.48436073732317,-23.168034272542,4.25055915192515));
#92427=CARTESIAN_POINT('Ctrl Pts',(-3.49460064242592,-23.1678467144834,
4.24162947897747));
#92428=CARTESIAN_POINT('Ctrl Pts',(-3.50414548344453,-23.1678572110644,
4.23200945990114));
#92429=CARTESIAN_POINT('Ctrl Pts',(-3.50634575216987,-23.1678596307274,
4.22979186119314));
#92430=CARTESIAN_POINT('Ctrl Pts',(-3.50850906418678,-23.1678723584513,
4.22753756056653));
#92431=CARTESIAN_POINT('Ctrl Pts',(-3.51063422148549,-23.1678953318369,
4.22524754091519));
#92432=CARTESIAN_POINT('Ctrl Pts',(-3.52021898816255,-23.1679989451271,
4.21491922119162));
#92433=CARTESIAN_POINT('Ctrl Pts',(-3.52899284990985,-23.1683220299147,
4.20385632239788));
#92434=CARTESIAN_POINT('Ctrl Pts',(-3.53691933305998,-23.168804138081,4.19218781074263));
#92435=CARTESIAN_POINT('Ctrl Pts',(-3.54524904504247,-23.169310771615,4.17992570918867));
#92436=CARTESIAN_POINT('Ctrl Pts',(-3.55264239516412,-23.1699924762988,
4.16699438610174));
#92437=CARTESIAN_POINT('Ctrl Pts',(-3.55905829477961,-23.1707193115775,
4.15353875310712));
#92438=CARTESIAN_POINT('Ctrl Pts',(-3.56589901925505,-23.1714942738086,
4.13919216362241));
#92439=CARTESIAN_POINT('Ctrl Pts',(-3.57162746497981,-23.1723197923469,
4.12424874315674));
#92440=CARTESIAN_POINT('Ctrl Pts',(-3.57620852167135,-23.1729819475165,
4.10888854586347));
#92441=CARTESIAN_POINT('Ctrl Pts',(-3.57775956255688,-23.173206138093,4.10368793482203));
#92442=CARTESIAN_POINT('Ctrl Pts',(-3.57917927008932,-23.173411204468,4.09843963864397));
#92443=CARTESIAN_POINT('Ctrl Pts',(-3.58046699811946,-23.1735877853888,
4.0931510103795));
#92444=CARTESIAN_POINT('Origin',(-3.57500058690307,-23.0745775160831,4.08839184830127));
#92445=CARTESIAN_POINT('Ctrl Pts',(-3.59003004342,-23.1742356021,4.05400943362));
#92446=CARTESIAN_POINT('Ctrl Pts',(-3.56100550691,-23.1742356,4.04198707509));
#92447=CARTESIAN_POINT('Ctrl Pts',(-3.53198097115,-23.1618985927,4.02996471716));
#92448=CARTESIAN_POINT('Ctrl Pts',(-3.50903998578,-23.1370674502,4.020462249));
#92449=CARTESIAN_POINT('Ctrl Pts',(-3.49764207994,-23.1056515239,4.01574108184));
#92450=CARTESIAN_POINT('Ctrl Pts',(-3.49764208329,-23.0742355991,4.01574108398));
#92451=CARTESIAN_POINT('Ctrl Pts',(-3.58811407486,-23.1742356053,4.06182447384));
#92452=CARTESIAN_POINT('Ctrl Pts',(-3.55886400839,-23.1746190551,4.04970869805));
#92453=CARTESIAN_POINT('Ctrl Pts',(-3.52949614106,-23.1624737743,4.03748383221));
#92454=CARTESIAN_POINT('Ctrl Pts',(-3.50623772102,-23.1375556797,4.02772852035));
#92455=CARTESIAN_POINT('Ctrl Pts',(-3.49471696821,-23.1058956405,4.02280292775));
#92456=CARTESIAN_POINT('Ctrl Pts',(-3.49477125586,-23.0742356024,4.0226718745));
#92457=CARTESIAN_POINT('Ctrl Pts',(-3.5861997009,-23.1741720972,4.06964669163));
#92458=CARTESIAN_POINT('Ctrl Pts',(-3.5567270736,-23.1749477738,4.05744341379));
#92459=CARTESIAN_POINT('Ctrl Pts',(-3.52701409515,-23.1630030812,4.04501677108));
#92460=CARTESIAN_POINT('Ctrl Pts',(-3.50343430799,-23.138001656,4.03500416396));
#92461=CARTESIAN_POINT('Ctrl Pts',(-3.49179021707,-23.1060974603,4.02986873261));
#92462=CARTESIAN_POINT('Ctrl Pts',(-3.49190063063,-23.0741932655,4.02960217686));
#92463=CARTESIAN_POINT('Ctrl Pts',(-3.5842870025,-23.1740438599,4.07747556494));
#92464=CARTESIAN_POINT('Ctrl Pts',(-3.55459489737,-23.1752205531,4.0651910977));
#92465=CARTESIAN_POINT('Ctrl Pts',(-3.52453502353,-23.1634855096,4.05256363124));
#92466=CARTESIAN_POINT('Ctrl Pts',(-3.50062982413,-23.1384045129,4.04228916144));
#92467=CARTESIAN_POINT('Ctrl Pts',(-3.48886193116,-23.1062561443,4.03693824347));
#92468=CARTESIAN_POINT('Ctrl Pts',(-3.48903039927,-23.074107776,4.03653152834));
#92469=CARTESIAN_POINT('Ctrl Pts',(-3.58237606919,-23.1738495698,4.08531053381));
#92470=CARTESIAN_POINT('Ctrl Pts',(-3.55246768452,-23.1754360753,4.07295161995));
#92471=CARTESIAN_POINT('Ctrl Pts',(-3.52205911864,-23.1639199594,4.06012452288));
#92472=CARTESIAN_POINT('Ctrl Pts',(-3.49782434849,-23.1387632939,4.04958350869));
#92473=CARTESIAN_POINT('Ctrl Pts',(-3.48593221864,-23.1063707724,4.04401119803));
#92474=CARTESIAN_POINT('Ctrl Pts',(-3.48616076587,-23.0739782508,4.0434594362));
#92475=CARTESIAN_POINT('Ctrl Pts',(-3.58046699728,-23.1735877856,4.09315100795));
#92476=CARTESIAN_POINT('Ctrl Pts',(-3.55034564706,-23.1755928932,4.08072486167));
#92477=CARTESIAN_POINT('Ctrl Pts',(-3.51958658013,-23.1643052014,4.06769960726));
#92478=CARTESIAN_POINT('Ctrl Pts',(-3.49501794889,-23.1390769393,4.05688723526));
#92479=CARTESIAN_POINT('Ctrl Pts',(-3.48300118522,-23.1064403336,4.05108733867));
#92480=CARTESIAN_POINT('Ctrl Pts',(-3.48329194402,-23.073803728,4.05038538482));
#92481=CARTESIAN_POINT('',(-3.59003004166812,-23.17423560745,4.05400943566779));
#92482=CARTESIAN_POINT('Origin',(-3.66997333637772,-22.6950817829913,3.82597648379911));
#92483=CARTESIAN_POINT('Origin',(-3.58937676056356,-23.0749427241466,4.05373884035109));
#92484=CARTESIAN_POINT('Origin',(9.24917823675E-16,-22.8742356128,0.729452270839));
#92485=CARTESIAN_POINT('',(-2.95028784657,-23.1742356128,4.63288636429));
#92486=CARTESIAN_POINT('Origin',(-3.42702565972E-16,-23.1742356128,0.729452270839));
#92487=CARTESIAN_POINT('',(-3.13117783752,-22.8742356128,4.87221628548));
#92488=CARTESIAN_POINT('Origin',(-2.95028784657,-22.8742356128,4.63288636429));
#92489=CARTESIAN_POINT('',(-4.2092958712,-22.8742356128,3.77060280966));
#92490=CARTESIAN_POINT('Origin',(3.67394039744E-17,-22.8742356128,0.729452270839));
#92491=CARTESIAN_POINT('',(-3.96612236541,-23.1742356128,3.59491374888));
#92492=CARTESIAN_POINT('Origin',(-3.96612236541,-22.8742356128,3.59491374888));
#92493=CARTESIAN_POINT('Origin',(-3.42702565972E-16,-23.1742356128,0.729452270839));
#92494=CARTESIAN_POINT('Origin',(-3.31206782846,-22.8742356128,5.11154620667));
#92495=CARTESIAN_POINT('',(-2.90473307408,-23.1742356128,5.55208950519));
#92496=CARTESIAN_POINT('',(-3.10840045127,-22.8742356128,5.33181785593));
#92497=CARTESIAN_POINT('Origin',(-2.90473307408,-22.8742356128,5.55208950519));
#92498=CARTESIAN_POINT('Origin',(-3.31206782846,-22.8742356128,5.11154620667));
#92499=CARTESIAN_POINT('Origin',(-3.31206782846,-23.1742356128,5.11154620667));
#92500=CARTESIAN_POINT('Origin',(-6.6707290414,-22.8742356128,9.03420135995));
#92501=CARTESIAN_POINT('',(-4.51260368036,-23.1742356128,7.03875740065));
#92502=CARTESIAN_POINT('',(-4.71627105755,-22.8742356128,6.81848575139));
#92503=CARTESIAN_POINT('Origin',(-4.51260368036,-22.8742356128,7.03875740065));
#92504=CARTESIAN_POINT('',(-3.91233575441,-22.8742356128,6.07515180366));
#92505=CARTESIAN_POINT('',(-3.70866837722,-23.1742356128,6.29542345292));
#92506=CARTESIAN_POINT('Origin',(-4.91993843473,-22.8742356128,6.59821410213));
#92507=CARTESIAN_POINT('',(-5.40800342362,-23.1742356128,6.94720201972));
#92508=CARTESIAN_POINT('',(-5.16397092918,-22.8742356128,6.77270806092));
#92509=CARTESIAN_POINT('Origin',(-5.40800342362,-22.8742356128,6.94720201972));
#92510=CARTESIAN_POINT('Origin',(-4.91993843473,-22.8742356128,6.59821410213));
#92511=CARTESIAN_POINT('Origin',(-4.91993843473,-23.1742356128,6.59821410213));
#92512=CARTESIAN_POINT('Origin',(-0.00234331738835,-22.8742356128,3.08191746407));
#92513=CARTESIAN_POINT('',(-6.57948381998,-23.1742356128,4.03207991826));
#92514=CARTESIAN_POINT('',(-6.28256615006,-22.8742356128,3.98918589435));
#92515=CARTESIAN_POINT('Origin',(-6.57948381998,-22.8742356128,4.03207991826));
#92516=CARTESIAN_POINT('Origin',(-0.00234331738835,-22.8742356128,3.08191746407));
#92517=CARTESIAN_POINT('Origin',(-0.00234331738835,-23.1742356128,3.08191746407));
#92518=CARTESIAN_POINT('Origin',(-4.452469377,-22.8742356128,3.94629187045));
#92519=CARTESIAN_POINT('',(-4.452469377,-22.8742356128,3.64629187045));
#92520=CARTESIAN_POINT('Origin',(-4.452469377,-22.8742356128,3.94629187045));
#92521=CARTESIAN_POINT('',(-4.452469377,-23.1742356128,3.34629187045));
#92522=CARTESIAN_POINT('Origin',(-4.452469377,-22.8742356128,3.34629187045));
#92523=CARTESIAN_POINT('Origin',(-4.452469377,-23.1742356128,3.94629187045));
#92524=CARTESIAN_POINT('Origin',(-5.98564848014,-22.8742356128,3.94629187045));
#92525=CARTESIAN_POINT('',(-5.98564848014,-23.1742356128,3.34629187045));
#92526=CARTESIAN_POINT('',(-5.98564848014,-22.8742356128,3.64629187045));
#92527=CARTESIAN_POINT('Origin',(-5.98564848014,-22.8742356128,3.34629187045));
#92528=CARTESIAN_POINT('Origin',(-5.98564848014,-22.8742356128,3.94629187045));
#92529=CARTESIAN_POINT('Origin',(-5.98564848014,-23.1742356128,3.94629187045));
#92530=CARTESIAN_POINT('Origin',(-6.6707290414,-22.8742356128,3.34629187045));
#92531=CARTESIAN_POINT('',(-5.21905892857,-22.8742356128,3.64629187045));
#92532=CARTESIAN_POINT('',(-5.21905892857,-23.1742356128,3.34629187045));
#92533=CARTESIAN_POINT('Origin',(-4.1372329486,-21.0742356128,5.87450964899));
#92534=CARTESIAN_POINT('',(-3.31206782846,-20.7742356128,5.11154620667));
#92535=CARTESIAN_POINT('',(-3.10840045127,-21.0742356128,5.33181785593));
#92536=CARTESIAN_POINT('Ctrl Pts',(-3.31206782846,-20.7742356128,5.11154620667));
#92537=CARTESIAN_POINT('Ctrl Pts',(-3.29933521826663,-20.7742356127999,
5.12531686098549));
#92538=CARTESIAN_POINT('Ctrl Pts',(-3.28660287019773,-20.775999501442,5.13908723180644));
#92539=CARTESIAN_POINT('Ctrl Pts',(-3.27409353932531,-20.7794964191287,
5.15261640363735));
#92540=CARTESIAN_POINT('Ctrl Pts',(-3.26210247220447,-20.7828484589079,
5.16558505952856));
#92541=CARTESIAN_POINT('Ctrl Pts',(-3.25031672255145,-20.7877924035019,
5.1783316591539));
#92542=CARTESIAN_POINT('Ctrl Pts',(-3.23892583382867,-20.7942487422808,
5.19065120625108));
#92543=CARTESIAN_POINT('Ctrl Pts',(-3.22753797140324,-20.800703365759,5.20296748032772));
#92544=CARTESIAN_POINT('Ctrl Pts',(-3.21654515523054,-20.8086693535063,
5.21485650144502));
#92545=CARTESIAN_POINT('Ctrl Pts',(-3.2061240830046,-20.8180186608397,5.22612716637859));
#92546=CARTESIAN_POINT('Ctrl Pts',(-3.19570270992945,-20.8273682380811,
5.23739815668853));
#92547=CARTESIAN_POINT('Ctrl Pts',(-3.18585347586854,-20.8381008902533,
5.24805036353882));
#92548=CARTESIAN_POINT('Ctrl Pts',(-3.17673470576069,-20.8500440916057,
5.25791255432522));
#92549=CARTESIAN_POINT('Ctrl Pts',(-3.17554748033519,-20.8515990460721,
5.25919656998899));
#92550=CARTESIAN_POINT('Ctrl Pts',(-3.17437260707132,-20.8531744629905,
5.26046722646361));
#92551=CARTESIAN_POINT('Ctrl Pts',(-3.17321040762789,-20.8547699110405,
5.26172417586659));
#92552=CARTESIAN_POINT('Ctrl Pts',(-3.16700069378047,-20.8632945028438,
5.26844014545107));
#92553=CARTESIAN_POINT('Ctrl Pts',(-3.16115327543625,-20.8723916371716,
5.2747642828771));
#92554=CARTESIAN_POINT('Ctrl Pts',(-3.15571375996958,-20.8819903575583,
5.28064726256438));
#92555=CARTESIAN_POINT('Ctrl Pts',(-3.15299400223624,-20.8867897177517,
5.28358875240802));
#92556=CARTESIAN_POINT('Ctrl Pts',(-3.15037611880697,-20.8917143566616,
5.28642006250033));
#92557=CARTESIAN_POINT('Ctrl Pts',(-3.14786523424292,-20.896754634957,5.28913565049302));
#92558=CARTESIAN_POINT('Ctrl Pts',(-3.14680766159051,-20.8988775762351,
5.29027944325729));
#92559=CARTESIAN_POINT('Ctrl Pts',(-3.14562334882535,-20.9013206204291,
5.29156030880195));
#92560=CARTESIAN_POINT('Ctrl Pts',(-3.14450250481394,-20.9037103020532,
5.2927725312126));
#92561=CARTESIAN_POINT('Ctrl Pts',(-3.14326498842998,-20.9063487335674,
5.2941109378766));
#92562=CARTESIAN_POINT('Ctrl Pts',(-3.14210503148785,-20.9089219096235,
5.29536546195516));
#92563=CARTESIAN_POINT('Ctrl Pts',(-3.14123879647682,-20.910887453468,5.29630231800518));
#92564=CARTESIAN_POINT('Ctrl Pts',(-3.14102688301432,-20.911368298962,5.29653150801353));
#92565=CARTESIAN_POINT('Ctrl Pts',(-3.14083239185809,-20.9118126387024,
5.29674185533738));
#92566=CARTESIAN_POINT('Ctrl Pts',(-3.14065826128173,-20.9122123369602,
5.29693018215616));
#92567=CARTESIAN_POINT('Ctrl Pts',(-3.1375970523511,-20.9192390171794,5.30024096049042));
#92568=CARTESIAN_POINT('Ctrl Pts',(-3.13478628520643,-20.9264540360834,
5.30338356310924));
#92569=CARTESIAN_POINT('Ctrl Pts',(-3.13223592512423,-20.9338322706568,
5.30634721230281));
#92570=CARTESIAN_POINT('Ctrl Pts',(-3.13096074508313,-20.9375213879435,
5.30782903689959));
#92571=CARTESIAN_POINT('Ctrl Pts',(-3.129750643895,-20.9412512918604,5.3092661479207));
#92572=CARTESIAN_POINT('Ctrl Pts',(-3.12860673216448,-20.9450187312842,
5.31065734421785));
#92573=CARTESIAN_POINT('Ctrl Pts',(-3.12803477629922,-20.9469024509962,
5.31135294236643));
#92574=CARTESIAN_POINT('Ctrl Pts',(-3.12747936638829,-20.948795553409,5.31203706335906));
#92575=CARTESIAN_POINT('Ctrl Pts',(-3.12694063242266,-20.950697626295,5.31270956660706));
#92576=CARTESIAN_POINT('Ctrl Pts',(-3.12663283447761,-20.9517843484305,
5.31309379171811));
#92577=CARTESIAN_POINT('Ctrl Pts',(-3.12619161680522,-20.9533813143145,
5.31365170209757));
#92578=CARTESIAN_POINT('Ctrl Pts',(-3.12585743559154,-20.9546204589871,
5.31407645693962));
#92579=CARTESIAN_POINT('Ctrl Pts',(-3.12560670461402,-20.9555501700011,
5.31439514390465));
#92580=CARTESIAN_POINT('Ctrl Pts',(-3.12541480694582,-20.9562775177554,
5.31464041022965));
#92581=CARTESIAN_POINT('Ctrl Pts',(-3.12537458248023,-20.9564303402735,
5.3146920888797));
#92582=CARTESIAN_POINT('Ctrl Pts',(-3.12522435030849,-20.957001108796,5.31488510066286));
#92583=CARTESIAN_POINT('Ctrl Pts',(-3.12479964436627,-20.9584280758291,
5.31532581148723));
#92584=CARTESIAN_POINT('Ctrl Pts',(-3.12412770189941,-20.9607278021972,
5.31598476355186));
#92585=CARTESIAN_POINT('Ctrl Pts',(-3.12396023830268,-20.9613009471733,
5.31614898964004));
#92586=CARTESIAN_POINT('Ctrl Pts',(-3.12377757874227,-20.9619283916087,
5.31632659765268));
#92587=CARTESIAN_POINT('Ctrl Pts',(-3.1235804670171,-20.9626105622649,5.31651678315158));
#92588=CARTESIAN_POINT('Ctrl Pts',(-3.12311253766171,-20.9642299873657,
5.31696827013355));
#92589=CARTESIAN_POINT('Ctrl Pts',(-3.12243241818589,-20.9666119834499,
5.31761216570488));
#92590=CARTESIAN_POINT('Ctrl Pts',(-3.12174493077351,-20.969121675404,5.31825518911771));
#92591=CARTESIAN_POINT('Ctrl Pts',(-3.12109418479046,-20.9714972417466,
5.31886384739328));
#92592=CARTESIAN_POINT('Ctrl Pts',(-3.1204372075556,-20.9739871819659,5.31947132386135));
#92593=CARTESIAN_POINT('Ctrl Pts',(-3.11991259420517,-20.9760333492218,
5.31995167406521));
#92594=CARTESIAN_POINT('Ctrl Pts',(-3.11982119675865,-20.9763898297845,
5.32003536004467));
#92595=CARTESIAN_POINT('Ctrl Pts',(-3.11973373269842,-20.9767327986748,
5.32011527847067));
#92596=CARTESIAN_POINT('Ctrl Pts',(-3.11965084049907,-20.9770592586797,
5.32019086546073));
#92597=CARTESIAN_POINT('Ctrl Pts',(-3.11873221172192,-20.980677157076,5.32102853637301));
#92598=CARTESIAN_POINT('Ctrl Pts',(-3.11800394114676,-20.9837595200313,
5.32169404058884));
#92599=CARTESIAN_POINT('Ctrl Pts',(-3.11737165618863,-20.9865959563919,
5.32228942746157));
#92600=CARTESIAN_POINT('Ctrl Pts',(-3.11667947524101,-20.9897010867334,
5.32294121498944));
#92601=CARTESIAN_POINT('Ctrl Pts',(-3.11610269286778,-20.9925119721021,
5.32350857546106));
#92602=CARTESIAN_POINT('Ctrl Pts',(-3.11555570510201,-20.9954279844329,
5.32408406940618));
#92603=CARTESIAN_POINT('Ctrl Pts',(-3.11544778770807,-20.9960032961146,
5.32419761089772));
#92604=CARTESIAN_POINT('Ctrl Pts',(-3.11534113468803,-20.9965827453735,
5.32431135583329));
#92605=CARTESIAN_POINT('Ctrl Pts',(-3.11523524285449,-20.9971694629971,
5.32442584825116));
#92606=CARTESIAN_POINT('Ctrl Pts',(-3.11209966050602,-21.0145428652934,
5.32781610406697));
#92607=CARTESIAN_POINT('Ctrl Pts',(-3.110027452273,-21.0323321591983,5.3300569564894));
#92608=CARTESIAN_POINT('Ctrl Pts',(-3.10905193709402,-21.0502512911575,
5.33111237020608));
#92609=CARTESIAN_POINT('Ctrl Pts',(-3.10861763232592,-21.0582289880891,
5.33158224624629));
#92610=CARTESIAN_POINT('Ctrl Pts',(-3.1084002383703,-21.066232297709,5.33181765908384));
#92611=CARTESIAN_POINT('Ctrl Pts',(-3.10840045126752,-21.0742356128,5.33181785593268));
#92612=CARTESIAN_POINT('',(-4.71627105755,-21.0742356128,6.81848575139));
#92613=CARTESIAN_POINT('',(-3.91233575441,-21.0742356128,6.07515180366));
#92614=CARTESIAN_POINT('',(-4.91993843473,-20.7742356128,6.59821410213));
#92615=CARTESIAN_POINT('Ctrl Pts',(-4.91993843473,-20.7742356128,6.59821410213));
#92616=CARTESIAN_POINT('Ctrl Pts',(-4.91101807800614,-20.7742356128001,
6.60786170359966));
#92617=CARTESIAN_POINT('Ctrl Pts',(-4.90252339602707,-20.7750985628785,
6.61712968289017));
#92618=CARTESIAN_POINT('Ctrl Pts',(-4.8944934572549,-20.7766036070835,6.62592256231193));
#92619=CARTESIAN_POINT('Ctrl Pts',(-4.88605462232259,-20.7781852903283,
6.63516318794124));
#92620=CARTESIAN_POINT('Ctrl Pts',(-4.87812882597999,-20.7804752394698,
6.64387935631824));
#92621=CARTESIAN_POINT('Ctrl Pts',(-4.87072223708168,-20.7832292456085,
6.65200261974273));
#92622=CARTESIAN_POINT('Ctrl Pts',(-4.86531045478571,-20.7852415189868,
6.65793805558096));
#92623=CARTESIAN_POINT('Ctrl Pts',(-4.86017499035168,-20.7875018067851,
6.66355789937889));
#92624=CARTESIAN_POINT('Ctrl Pts',(-4.85530752896798,-20.7899222629677,
6.66884704557737));
#92625=CARTESIAN_POINT('Ctrl Pts',(-4.84828146203815,-20.7934161349884,
6.67648180469773));
#92626=CARTESIAN_POINT('Ctrl Pts',(-4.84182598167012,-20.7972434179056,
6.68344575129118));
#92627=CARTESIAN_POINT('Ctrl Pts',(-4.8359312132666,-20.8011818445937,6.68978189067321));
#92628=CARTESIAN_POINT('Ctrl Pts',(-4.83433051190638,-20.8022513089942,
6.69150244460053));
#92629=CARTESIAN_POINT('Ctrl Pts',(-4.8327710384092,-20.8033292152502,6.69317683282407));
#92630=CARTESIAN_POINT('Ctrl Pts',(-4.83125236393977,-20.8044116620105,
6.69480616639989));
#92631=CARTESIAN_POINT('Ctrl Pts',(-4.82769667927255,-20.8069460032574,
6.69862093811689));
#92632=CARTESIAN_POINT('Ctrl Pts',(-4.82436526487051,-20.8095049076771,
6.70218957148497));
#92633=CARTESIAN_POINT('Ctrl Pts',(-4.82125350553739,-20.812044273078,6.70553206549793));
#92634=CARTESIAN_POINT('Ctrl Pts',(-4.81969762587084,-20.8133139557784,
6.70720331250441));
#92635=CARTESIAN_POINT('Ctrl Pts',(-4.81843122123371,-20.8143803798034,
6.7085628667989));
#92636=CARTESIAN_POINT('Ctrl Pts',(-4.81709937825491,-20.8155303534285,
6.70999899677484));
#92637=CARTESIAN_POINT('Ctrl Pts',(-4.81587928901512,-20.8165838338074,
6.71131462238422));
#92638=CARTESIAN_POINT('Ctrl Pts',(-4.81460418147319,-20.8177075259004,
6.71269462123414));
#92639=CARTESIAN_POINT('Ctrl Pts',(-4.81301644753763,-20.8191595577754,
6.71442100155403));
#92640=CARTESIAN_POINT('Ctrl Pts',(-4.81287101948364,-20.8192925562364,
6.71457912888554));
#92641=CARTESIAN_POINT('Ctrl Pts',(-4.81272298219209,-20.8194283405095,
6.7147401475396));
#92642=CARTESIAN_POINT('Ctrl Pts',(-4.81257214682211,-20.8195671295471,
6.71490426436397));
#92643=CARTESIAN_POINT('Ctrl Pts',(-4.80473608843389,-20.8267773681179,
6.72343030847733));
#92644=CARTESIAN_POINT('Ctrl Pts',(-4.79752989742272,-20.8344866681735,
6.73123516492522));
#92645=CARTESIAN_POINT('Ctrl Pts',(-4.79092681315199,-20.8424631101107,
6.7383485989656));
#92646=CARTESIAN_POINT('Ctrl Pts',(-4.78541183125531,-20.8491251381994,
6.74428983163013));
#92647=CARTESIAN_POINT('Ctrl Pts',(-4.78031680760064,-20.8559741803587,
6.74974956049137));
#92648=CARTESIAN_POINT('Ctrl Pts',(-4.77561385480444,-20.8628961108439,
6.75475842594953));
#92649=CARTESIAN_POINT('Ctrl Pts',(-4.77223310973378,-20.8678719809795,
6.75835907812297));
#92650=CARTESIAN_POINT('Ctrl Pts',(-4.76896166073005,-20.8730320642035,
6.76182963192853));
#92651=CARTESIAN_POINT('Ctrl Pts',(-4.76589273431812,-20.8782133062045,
6.76508294196168));
#92652=CARTESIAN_POINT('Ctrl Pts',(-4.76261503962766,-20.88374700989,6.76855756324314));
#92653=CARTESIAN_POINT('Ctrl Pts',(-4.75956871210815,-20.8893043149753,
6.77178399636243));
#92654=CARTESIAN_POINT('Ctrl Pts',(-4.75683198223358,-20.8946499026989,
6.77469430090779));
#92655=CARTESIAN_POINT('Ctrl Pts',(-4.75429868506137,-20.899598130286,6.77738827021165));
#92656=CARTESIAN_POINT('Ctrl Pts',(-4.75202989571111,-20.9043638139079,
6.77981219865064));
#92657=CARTESIAN_POINT('Ctrl Pts',(-4.75006304874771,-20.9087436757408,
6.78193882013059));
#92658=CARTESIAN_POINT('Ctrl Pts',(-4.74555434167549,-20.9187838641179,
6.78681378675738));
#92659=CARTESIAN_POINT('Ctrl Pts',(-4.74160660860021,-20.9288814156251,
6.7910825342297));
#92660=CARTESIAN_POINT('Ctrl Pts',(-4.73813954370417,-20.9389926751171,
6.79483177943904));
#92661=CARTESIAN_POINT('Ctrl Pts',(-4.73453775139493,-20.9494968501952,
6.79872671736649));
#92662=CARTESIAN_POINT('Ctrl Pts',(-4.73145429815306,-20.9600166233867,
6.80206143894353));
#92663=CARTESIAN_POINT('Ctrl Pts',(-4.72882070162607,-20.9705491771698,
6.80490985719644));
#92664=CARTESIAN_POINT('Ctrl Pts',(-4.72607730103734,-20.9815208708038,
6.80787703619746));
#92665=CARTESIAN_POINT('Ctrl Pts',(-4.72382167411467,-20.9925073236551,
6.8103169231494));
#92666=CARTESIAN_POINT('Ctrl Pts',(-4.72200555539,-21.0035411667321,6.81228154610962));
#92667=CARTESIAN_POINT('Ctrl Pts',(-4.72009746998151,-21.0151337540938,
6.81434565587991));
#92668=CARTESIAN_POINT('Ctrl Pts',(-4.7186740823484,-21.0267797209318,6.81588563580126));
#92669=CARTESIAN_POINT('Ctrl Pts',(-4.71771751058766,-21.0385403140574,
6.81692062577603));
#92670=CARTESIAN_POINT('Ctrl Pts',(-4.71676093882692,-21.050300907183,6.8179556157508));
#92671=CARTESIAN_POINT('Ctrl Pts',(-4.7162710575463,-21.0621774370813,6.818485751394));
#92672=CARTESIAN_POINT('Ctrl Pts',(-4.7162710575463,-21.0742356128,6.818485751394));
#92673=CARTESIAN_POINT('',(-4.1160031316,-20.7742356128,5.8548801544));
#92674=CARTESIAN_POINT('Origin',(-2.31985562646,-21.0742356128,7.05423263334));
#92675=CARTESIAN_POINT('',(-1.46510738459,-21.0742356128,5.8553296721));
#92676=CARTESIAN_POINT('',(-2.54349379462,-21.0742356128,6.85242635913));
#92677=CARTESIAN_POINT('',(-1.2614400074,-20.7742356128,6.07560132137));
#92678=CARTESIAN_POINT('Origin',(-1.26144000740192,-21.0742356128,6.07560132136512));
#92679=CARTESIAN_POINT('',(-2.33982641743,-20.7742356128,7.0726980084));
#92680=CARTESIAN_POINT('Origin',(-0.00234331738835,-21.0742356128,3.08191746407));
#92681=CARTESIAN_POINT('',(-6.21380646358,-21.0742356128,1.78497474518));
#92682=CARTESIAN_POINT('',(-5.92013962829,-20.7742356128,1.84629187045));
#92683=CARTESIAN_POINT('Ctrl Pts',(-6.21380646358263,-21.0742356128,1.78497474517945));
#92684=CARTESIAN_POINT('Ctrl Pts',(-6.21380646358263,-21.0638291242201,
1.78497474517945));
#92685=CARTESIAN_POINT('Ctrl Pts',(-6.21327417566471,-21.0536166921391,
1.78505315888558));
#92686=CARTESIAN_POINT('Ctrl Pts',(-6.21224803590314,-21.0435122709929,
1.7852283036963));
#92687=CARTESIAN_POINT('Ctrl Pts',(-6.2112178215814,-21.0333677275616,1.78540414396596));
#92688=CARTESIAN_POINT('Ctrl Pts',(-6.20968970505262,-21.0233311229344,
1.78567751866417));
#92689=CARTESIAN_POINT('Ctrl Pts',(-6.20765173862219,-21.0133172081608,
1.78607754692084));
#92690=CARTESIAN_POINT('Ctrl Pts',(-6.20633833173915,-21.0068635471027,
1.78633535286792));
#92691=CARTESIAN_POINT('Ctrl Pts',(-6.20481214385547,-21.0004193812891,
1.78664597516925));
#92692=CARTESIAN_POINT('Ctrl Pts',(-6.20305914183912,-20.9939650457512,
1.78701943793744));
#92693=CARTESIAN_POINT('Ctrl Pts',(-6.20017203893198,-20.9833350916946,
1.78763451164169));
#92694=CARTESIAN_POINT('Ctrl Pts',(-6.1966691290526,-20.9726827259468,1.78840119577086));
#92695=CARTESIAN_POINT('Ctrl Pts',(-6.19245514538327,-20.9619932754936,
1.7893188173187));
#92696=CARTESIAN_POINT('Ctrl Pts',(-6.19142746403405,-20.9593863957033,
1.78954260142048));
#92697=CARTESIAN_POINT('Ctrl Pts',(-6.19035731493665,-20.956777469529,1.78977539984786));
#92698=CARTESIAN_POINT('Ctrl Pts',(-6.18924298052752,-20.9541666224691,
1.79001727404038));
#92699=CARTESIAN_POINT('Ctrl Pts',(-6.18640116205152,-20.947508339864,1.79063411091049));
#92700=CARTESIAN_POINT('Ctrl Pts',(-6.18327258049845,-20.9408382928993,
1.79130942869506));
#92701=CARTESIAN_POINT('Ctrl Pts',(-6.17982938053887,-20.934169877643,1.79204407797328));
#92702=CARTESIAN_POINT('Ctrl Pts',(-6.17831560267499,-20.9312381572896,
1.79236706119474));
#92703=CARTESIAN_POINT('Ctrl Pts',(-6.17688544243804,-20.9285769855239,
1.79267133246466));
#92704=CARTESIAN_POINT('Ctrl Pts',(-6.17535411987191,-20.9258272802483,
1.79299524597198));
#92705=CARTESIAN_POINT('Ctrl Pts',(-6.17391712939085,-20.9232469615133,
1.7932992058541));
#92706=CARTESIAN_POINT('Ctrl Pts',(-6.17239097810791,-20.9205884555348,
1.79362047868821));
#92707=CARTESIAN_POINT('Ctrl Pts',(-6.17058626019263,-20.9175771306239,
1.79399842408086));
#92708=CARTESIAN_POINT('Ctrl Pts',(-6.16993973029997,-20.9164983406618,
1.79413382086064));
#92709=CARTESIAN_POINT('Ctrl Pts',(-6.16925708304517,-20.9153745097185,
1.79427656745455));
#92710=CARTESIAN_POINT('Ctrl Pts',(-6.16852821746026,-20.9141939713519,
1.79442876434852));
#92711=CARTESIAN_POINT('Ctrl Pts',(-6.16226859189097,-20.9040553006583,
1.79573585798662));
#92712=CARTESIAN_POINT('Ctrl Pts',(-6.15517323883986,-20.8939067913336,
1.79721736722423));
#92713=CARTESIAN_POINT('Ctrl Pts',(-6.14713178957169,-20.8839003131641,
1.79888899627398));
#92714=CARTESIAN_POINT('Ctrl Pts',(-6.14250264364114,-20.8781399774145,
1.79985128734304));
#92715=CARTESIAN_POINT('Ctrl Pts',(-6.13756008361075,-20.872427578217,1.8008765606857));
#92716=CARTESIAN_POINT('Ctrl Pts',(-6.13228512614383,-20.8667997672481,
1.8019674021234));
#92717=CARTESIAN_POINT('Ctrl Pts',(-6.12756782361308,-20.86176691398,1.80294292260997));
#92718=CARTESIAN_POINT('Ctrl Pts',(-6.12271663472741,-20.8569369691441,
1.80394169722641));
#92719=CARTESIAN_POINT('Ctrl Pts',(-6.11760803373886,-20.8521972192353,
1.80499799326209));
#92720=CARTESIAN_POINT('Ctrl Pts',(-6.11234437566273,-20.8473136076668,
1.80608635016675));
#92721=CARTESIAN_POINT('Ctrl Pts',(-6.10680731541783,-20.8425247796987,
1.80723580224648));
#92722=CARTESIAN_POINT('Ctrl Pts',(-6.1008263123872,-20.837754257854,1.80849112969859));
#92723=CARTESIAN_POINT('Ctrl Pts',(-6.09543622633937,-20.8334550586889,
1.80962243208224));
#92724=CARTESIAN_POINT('Ctrl Pts',(-6.08968498885813,-20.8291706338078,
1.81083984845462));
#92725=CARTESIAN_POINT('Ctrl Pts',(-6.08342555190955,-20.8248881944549,
1.81218069347538));
#92726=CARTESIAN_POINT('Ctrl Pts',(-6.08273932768923,-20.8244187091593,
1.81232769077506));
#92727=CARTESIAN_POINT('Ctrl Pts',(-6.08204697635262,-20.8239492959192,
1.81247617541911));
#92728=CARTESIAN_POINT('Ctrl Pts',(-6.08134829036222,-20.823479974991,1.81262619935616));
#92729=CARTESIAN_POINT('Ctrl Pts',(-6.07084476035318,-20.8164245502068,
1.81488154860675));
#92730=CARTESIAN_POINT('Ctrl Pts',(-6.05949429674607,-20.8097986564887,
1.81725014952178));
#92731=CARTESIAN_POINT('Ctrl Pts',(-6.04732674889071,-20.8038283905592,
1.81977071506763));
#92732=CARTESIAN_POINT('Ctrl Pts',(-6.04124297496303,-20.8008432575944,
1.82103099784056));
#92733=CARTESIAN_POINT('Ctrl Pts',(-6.03495585748087,-20.7980223837757,
1.82232960162766));
#92734=CARTESIAN_POINT('Ctrl Pts',(-6.02847522956622,-20.7953955144343,
1.82367335937379));
#92735=CARTESIAN_POINT('Ctrl Pts',(-6.02583793509647,-20.7943265087641,
1.82422020219816));
#92736=CARTESIAN_POINT('Ctrl Pts',(-6.0228510692185,-20.7931653163342,1.82484135358158));
#92737=CARTESIAN_POINT('Ctrl Pts',(-6.01989947204153,-20.7920763253463,
1.82545656126346));
#92738=CARTESIAN_POINT('Ctrl Pts',(-6.0167298538359,-20.7909068955583,1.82611721153239));
#92739=CARTESIAN_POINT('Ctrl Pts',(-6.01360113456556,-20.7898210851413,
1.82677095962912));
#92740=CARTESIAN_POINT('Ctrl Pts',(-6.01101145633295,-20.788960047348,1.82731391901932));
#92741=CARTESIAN_POINT('Ctrl Pts',(-6.01008678157446,-20.7886526037809,
1.82750778899));
#92742=CARTESIAN_POINT('Ctrl Pts',(-6.00923099123423,-20.7883732746121,
1.82768750069863));
#92743=CARTESIAN_POINT('Ctrl Pts',(-6.00846713791962,-20.7881270953015,
1.82784824664587));
#92744=CARTESIAN_POINT('Ctrl Pts',(-6.0026023396212,-20.7862369522931,1.82908243983431));
#92745=CARTESIAN_POINT('Ctrl Pts',(-5.99587512952763,-20.7842726880881,
1.83049099473282));
#92746=CARTESIAN_POINT('Ctrl Pts',(-5.98825586153528,-20.7824167003156,
1.8320826743304));
#92747=CARTESIAN_POINT('Ctrl Pts',(-5.98084399712823,-20.7806112342623,
1.83363102692392));
#92748=CARTESIAN_POINT('Ctrl Pts',(-5.97258700545796,-20.7789084592162,
1.83535287478211));
#92749=CARTESIAN_POINT('Ctrl Pts',(-5.96347756599724,-20.7775200828796,
1.83725209508735));
#92750=CARTESIAN_POINT('Ctrl Pts',(-5.95480118246376,-20.7761977089138,
1.83906102788216));
#92751=CARTESIAN_POINT('Ctrl Pts',(-5.94535068955056,-20.7751610722981,
1.8410310343364));
#92752=CARTESIAN_POINT('Ctrl Pts',(-5.93515058418323,-20.7746277752809,
1.84315899601206));
#92753=CARTESIAN_POINT('Ctrl Pts',(-5.93031300926584,-20.7743748500236,
1.84416821833444));
#92754=CARTESIAN_POINT('Ctrl Pts',(-5.92530735504451,-20.7742356127999,
1.84521285807765));
#92755=CARTESIAN_POINT('Ctrl Pts',(-5.92013962829,-20.7742356128,1.84629187045));
#92756=CARTESIAN_POINT('',(-5.76218263052,-21.0742356128,0.419477620705));
#92757=CARTESIAN_POINT('Origin',(-0.00234331738835,-21.0742356128,3.08191746407));
#92758=CARTESIAN_POINT('',(-5.48986775992,-20.7742356128,0.545353000555));
#92759=CARTESIAN_POINT('Ctrl Pts',(-5.76218263051847,-21.0742356128,0.419477620705708));
#92760=CARTESIAN_POINT('Ctrl Pts',(-5.76218263051847,-21.0700542173555,
0.419477620705718));
#92761=CARTESIAN_POINT('Ctrl Pts',(-5.76208822882541,-21.0658728234983,
0.419481774388309));
#92762=CARTESIAN_POINT('Ctrl Pts',(-5.76189949703241,-21.0616950856527,
0.419490058448013));
#92763=CARTESIAN_POINT('Ctrl Pts',(-5.76180351272392,-21.0595703918119,
0.419494271515295));
#92764=CARTESIAN_POINT('Ctrl Pts',(-5.76170596844914,-21.0578162530132,
0.419502972865373));
#92765=CARTESIAN_POINT('Ctrl Pts',(-5.76157699842966,-21.0558688871039,
0.419508645330075));
#92766=CARTESIAN_POINT('Ctrl Pts',(-5.76145237759245,-21.0539871911022,
0.419514126505492));
#92767=CARTESIAN_POINT('Ctrl Pts',(-5.7612993086323,-21.0519248572092,0.41951636520272));
#92768=CARTESIAN_POINT('Ctrl Pts',(-5.76105052573855,-21.0491764894493,
0.419527231998826));
#92769=CARTESIAN_POINT('Ctrl Pts',(-5.76054427759769,-21.0435838377684,
0.419549344834819));
#92770=CARTESIAN_POINT('Ctrl Pts',(-5.75995086462676,-21.0380043491261,
0.4197570049967));
#92771=CARTESIAN_POINT('Ctrl Pts',(-5.75927114796157,-21.0324468066016,
0.420149699187728));
#92772=CARTESIAN_POINT('Ctrl Pts',(-5.75893128962897,-21.0296680353393,
0.42034604628324));
#92773=CARTESIAN_POINT('Ctrl Pts',(-5.75856986164284,-21.0268947495701,
0.420588648987048));
#92774=CARTESIAN_POINT('Ctrl Pts',(-5.75818700380084,-21.0241280412191,
0.420877413809454));
#92775=CARTESIAN_POINT('Ctrl Pts',(-5.75800935278482,-21.0228442525758,
0.421011404441123));
#92776=CARTESIAN_POINT('Ctrl Pts',(-5.75774710432639,-21.0209676723318,
0.421231939899458));
#92777=CARTESIAN_POINT('Ctrl Pts',(-5.75750471561971,-21.0193269715218,
0.421435552712598));
#92778=CARTESIAN_POINT('Ctrl Pts',(-5.75722472950835,-21.0174317782761,
0.421670748322804));
#92779=CARTESIAN_POINT('Ctrl Pts',(-5.75697461782143,-21.0158507644803,
0.42188180568687));
#92780=CARTESIAN_POINT('Ctrl Pts',(-5.75697430408476,-21.0158487352453,
0.42188208656193));
#92781=CARTESIAN_POINT('Ctrl Pts',(-5.75697391849401,-21.0158462412614,
0.421882431764879));
#92782=CARTESIAN_POINT('Ctrl Pts',(-5.75681273469604,-21.0149286495503,
0.421957097869057));
#92783=CARTESIAN_POINT('Ctrl Pts',(-5.75646751532521,-21.0131012056486,
0.422116826131579));
#92784=CARTESIAN_POINT('Ctrl Pts',(-5.75611606673489,-21.0112407869194,
0.422279436568426));
#92785=CARTESIAN_POINT('Ctrl Pts',(-5.75557395522215,-21.0084370054318,
0.422530172355905));
#92786=CARTESIAN_POINT('Ctrl Pts',(-5.75476782901722,-21.0047090998318,
0.422902939748514));
#92787=CARTESIAN_POINT('Ctrl Pts',(-5.75396170281228,-21.0009811942318,
0.423275707141123));
#92788=CARTESIAN_POINT('Ctrl Pts',(-5.75289137553641,-20.9963284789036,
0.423770592291697));
#92789=CARTESIAN_POINT('Ctrl Pts',(-5.75143609421341,-20.9907917516533,
0.424443412285836));
#92790=CARTESIAN_POINT('Ctrl Pts',(-5.75003801615353,-20.98547265852,0.42508978550398));
#92791=CARTESIAN_POINT('Ctrl Pts',(-5.748284064558,-20.9793370244532,0.42590065187824));
#92792=CARTESIAN_POINT('Ctrl Pts',(-5.74602953787445,-20.9724505880868,
0.426942898528165));
#92793=CARTESIAN_POINT('Ctrl Pts',(-5.74383550469501,-20.9657489287159,
0.427957179595572));
#92794=CARTESIAN_POINT('Ctrl Pts',(-5.74116676451505,-20.9583354833729,
0.429190883969123));
#92795=CARTESIAN_POINT('Ctrl Pts',(-5.73786227189959,-20.9503096563882,
0.430718453591819));
#92796=CARTESIAN_POINT('Ctrl Pts',(-5.73474618032658,-20.9427414107469,
0.432158930960783));
#92797=CARTESIAN_POINT('Ctrl Pts',(-5.73106397875205,-20.9346282631776,
0.433861082610605));
#92798=CARTESIAN_POINT('Ctrl Pts',(-5.7266659725094,-20.926095961081,0.435894103682038));
#92799=CARTESIAN_POINT('Ctrl Pts',(-5.72244512364354,-20.9179073511426,
0.437845232036613));
#92800=CARTESIAN_POINT('Ctrl Pts',(-5.71756421491754,-20.9093323848096,
0.440101462659826));
#92801=CARTESIAN_POINT('Ctrl Pts',(-5.71188791964413,-20.9005271966043,
0.442725349212077));
#92802=CARTESIAN_POINT('Ctrl Pts',(-5.70643988023259,-20.8920760836763,
0.445243723725645));
#92803=CARTESIAN_POINT('Ctrl Pts',(-5.70025837439386,-20.8834128049173,
0.448101132492726));
#92804=CARTESIAN_POINT('Ctrl Pts',(-5.69323182479467,-20.8747203666876,
0.451349151232407));
#92805=CARTESIAN_POINT('Ctrl Pts',(-5.68647772309588,-20.8663649696347,
0.454471231077957));
#92806=CARTESIAN_POINT('Ctrl Pts',(-5.67894210952565,-20.8579827361327,
0.457954554149233));
#92807=CARTESIAN_POINT('Ctrl Pts',(-5.67054418362936,-20.8497784476017,
0.461836469810334));
#92808=CARTESIAN_POINT('Ctrl Pts',(-5.6624554326642,-20.8418762051202,0.465575470301429));
#92809=CARTESIAN_POINT('Ctrl Pts',(-5.6535660256726,-20.8341393286479,0.469684563567774));
#92810=CARTESIAN_POINT('Ctrl Pts',(-5.64383110675435,-20.8267879818355,
0.474184483903669));
#92811=CARTESIAN_POINT('Ctrl Pts',(-5.63418816478761,-20.8195060916333,
0.478641888327719));
#92812=CARTESIAN_POINT('Ctrl Pts',(-5.62371480691348,-20.8126028174762,
0.48348314188324));
#92813=CARTESIAN_POINT('Ctrl Pts',(-5.61240580309607,-20.8063250428812,
0.488710662141486));
#92814=CARTESIAN_POINT('Ctrl Pts',(-5.6019057715892,-20.8004963393009,0.4935642397245));
#92815=CARTESIAN_POINT('Ctrl Pts',(-5.5906851835362,-20.7952075582835,0.498750885402041));
#92816=CARTESIAN_POINT('Ctrl Pts',(-5.57877932195408,-20.7906767474455,
0.504254289919316));
#92817=CARTESIAN_POINT('Ctrl Pts',(-5.5671865239154,-20.7862650738648,0.509612982917204));
#92818=CARTESIAN_POINT('Ctrl Pts',(-5.55494366255547,-20.7825726642816,
0.515272159292754));
#92819=CARTESIAN_POINT('Ctrl Pts',(-5.54212646457403,-20.7798115878137,
0.521196815032388));
#92820=CARTESIAN_POINT('Ctrl Pts',(-5.52976210381069,-20.7771480613867,
0.526912150089981));
#92821=CARTESIAN_POINT('Ctrl Pts',(-5.51686313783045,-20.7753519171367,
0.532874599206211));
#92822=CARTESIAN_POINT('Ctrl Pts',(-5.5035416480442,-20.7746140611604,0.539032353698168));
#92823=CARTESIAN_POINT('Ctrl Pts',(-5.49902989564469,-20.7743641624234,
0.54111787596711));
#92824=CARTESIAN_POINT('Ctrl Pts',(-5.49447006936149,-20.7742356128,0.543225619674669));
#92825=CARTESIAN_POINT('Ctrl Pts',(-5.48986775992,-20.7742356128,0.545353000555));
#92826=CARTESIAN_POINT('Origin',(-0.00234331738835,-20.7742356128,3.08191746407));
#92827=CARTESIAN_POINT('Origin',(-5.48986775992,-21.0742356128,0.545353000555));
#92828=CARTESIAN_POINT('',(-5.1900363009,-21.0742356128,0.55540766038));
#92829=CARTESIAN_POINT('Origin',(-5.48986775992,-21.0742356128,0.545353000555));
#92830=CARTESIAN_POINT('Origin',(-5.48986775992,-21.0742356128,0.545353000555));
#92831=CARTESIAN_POINT('Origin',(1.47842115491E-15,-21.0742356128,0.729452270839));
#92832=CARTESIAN_POINT('',(-5.08448267152,-21.0742356128,1.78529520144));
#92833=CARTESIAN_POINT('',(-5.3782162351,-20.7742356128,1.84629187045));
#92834=CARTESIAN_POINT('Ctrl Pts',(-5.08448267152607,-21.0742356128,1.78529520144126));
#92835=CARTESIAN_POINT('Ctrl Pts',(-5.08448267152607,-21.0614130940682,
1.78529520144126));
#92836=CARTESIAN_POINT('Ctrl Pts',(-5.08528146803515,-21.0485906280905,
1.78549730909642));
#92837=CARTESIAN_POINT('Ctrl Pts',(-5.08687246330687,-21.0358733936431,
1.7859002586259));
#92838=CARTESIAN_POINT('Ctrl Pts',(-5.08766796094273,-21.0295147764195,
1.78610173339064));
#92839=CARTESIAN_POINT('Ctrl Pts',(-5.08866130593276,-21.0231824345426,
1.78635337671675));
#92840=CARTESIAN_POINT('Ctrl Pts',(-5.08985043859178,-21.0168894102148,
1.78665479764093));
#92841=CARTESIAN_POINT('Ctrl Pts',(-5.0903951219712,-21.0140068842564,1.78679286379055));
#92842=CARTESIAN_POINT('Ctrl Pts',(-5.09092718216906,-21.0113881381866,
1.78693799787711));
#92843=CARTESIAN_POINT('Ctrl Pts',(-5.0915147214932,-21.0086827022826,1.78708833999566));
#92844=CARTESIAN_POINT('Ctrl Pts',(-5.09207204900295,-21.00611638239,1.78723095138369));
#92845=CARTESIAN_POINT('Ctrl Pts',(-5.09267924627531,-21.0034718705681,
1.78737821109546));
#92846=CARTESIAN_POINT('Ctrl Pts',(-5.09342319728476,-21.0004534336218,
1.78756269841702));
#92847=CARTESIAN_POINT('Ctrl Pts',(-5.0936071767023,-20.9997069728143,1.7876083222142));
#92848=CARTESIAN_POINT('Ctrl Pts',(-5.09379967401835,-20.9989376697526,
1.78765640532237));
#92849=CARTESIAN_POINT('Ctrl Pts',(-5.09400233909841,-20.9981411165267,
1.78770783716017));
#92850=CARTESIAN_POINT('Ctrl Pts',(-5.09709097517254,-20.9860015657566,
1.7884916635083));
#92851=CARTESIAN_POINT('Ctrl Pts',(-5.10094234956947,-20.974063720211,1.78935051102611));
#92852=CARTESIAN_POINT('Ctrl Pts',(-5.1055271132446,-20.9624169074904,1.79028097896789));
#92853=CARTESIAN_POINT('Ctrl Pts',(-5.10654181896996,-20.9598392200921,
1.7904869113157));
#92854=CARTESIAN_POINT('Ctrl Pts',(-5.1075923771993,-20.9572759311037,1.79069622721775));
#92855=CARTESIAN_POINT('Ctrl Pts',(-5.10867832162472,-20.9547282358368,
1.79090865953936));
#92856=CARTESIAN_POINT('Ctrl Pts',(-5.11167461524405,-20.9476987388446,
1.79149479414705));
#92857=CARTESIAN_POINT('Ctrl Pts',(-5.11494087661384,-20.9407862593262,
1.79210608868242));
#92858=CARTESIAN_POINT('Ctrl Pts',(-5.11846765793979,-20.9340111008953,
1.79274037257807));
#92859=CARTESIAN_POINT('Ctrl Pts',(-5.11985187154921,-20.9313519435392,
1.79298932036345));
#92860=CARTESIAN_POINT('Ctrl Pts',(-5.1211267858793,-20.928986911576,1.79323158599076));
#92861=CARTESIAN_POINT('Ctrl Pts',(-5.12245944386044,-20.9265929771404,
1.79347032304439));
#92862=CARTESIAN_POINT('Ctrl Pts',(-5.12371441533186,-20.9243385956984,
1.79369514306253));
#92863=CARTESIAN_POINT('Ctrl Pts',(-5.12502075047096,-20.922058421466,1.79391703398184));
#92864=CARTESIAN_POINT('Ctrl Pts',(-5.12654632236385,-20.9194925254243,
1.79416863251517));
#92865=CARTESIAN_POINT('Ctrl Pts',(-5.12752829683552,-20.9178409189536,
1.79433058052822));
#92866=CARTESIAN_POINT('Ctrl Pts',(-5.12860157962051,-20.9160710796194,
1.79450533697522));
#92867=CARTESIAN_POINT('Ctrl Pts',(-5.12981865714979,-20.914117158484,1.7947096656124));
#92868=CARTESIAN_POINT('Ctrl Pts',(-5.13493442695431,-20.9059041971033,
1.79556852484454));
#92869=CARTESIAN_POINT('Ctrl Pts',(-5.14041852996597,-20.897943240988,1.79661719636324));
#92870=CARTESIAN_POINT('Ctrl Pts',(-5.14624478500792,-20.8902716071521,
1.79785127829691));
#92871=CARTESIAN_POINT('Ctrl Pts',(-5.1491579125289,-20.8864357902341,1.79846831926374));
#92872=CARTESIAN_POINT('Ctrl Pts',(-5.15215653588352,-20.8826722651419,
1.79913170401791));
#92873=CARTESIAN_POINT('Ctrl Pts',(-5.15523710145265,-20.8789854927669,
1.79984085770605));
#92874=CARTESIAN_POINT('Ctrl Pts',(-5.15677738423722,-20.8771421065794,
1.80019543455013));
#92875=CARTESIAN_POINT('Ctrl Pts',(-5.15833814960495,-20.8753179065473,
1.80056145300697));
#92876=CARTESIAN_POINT('Ctrl Pts',(-5.15991893697881,-20.8735134363296,
1.80093883851198));
#92877=CARTESIAN_POINT('Ctrl Pts',(-5.16070933066575,-20.8726112012207,
1.80112753126449));
#92878=CARTESIAN_POINT('Ctrl Pts',(-5.1615047296844,-20.871713898423,1.80131906574349));
#92879=CARTESIAN_POINT('Ctrl Pts',(-5.16230507536263,-20.8708215951015,
1.80151343250699));
#92880=CARTESIAN_POINT('Ctrl Pts',(-5.16286595087811,-20.8701962764435,
1.80164964309903));
#92881=CARTESIAN_POINT('Ctrl Pts',(-5.16381117101369,-20.8691535012779,
1.80187989131107));
#92882=CARTESIAN_POINT('Ctrl Pts',(-5.16433869641073,-20.8685768123516,
1.80201031399209));
#92883=CARTESIAN_POINT('Ctrl Pts',(-5.16456392748109,-20.8683305905301,
1.80206599896994));
#92884=CARTESIAN_POINT('Ctrl Pts',(-5.16471247623231,-20.8681689155371,
1.80210294211167));
#92885=CARTESIAN_POINT('Ctrl Pts',(-5.1647208930014,-20.8681597501726,1.80210502009182));
#92886=CARTESIAN_POINT('Ctrl Pts',(-5.16478496730456,-20.8680899770403,
1.80212083912267));
#92887=CARTESIAN_POINT('Ctrl Pts',(-5.16543415713941,-20.8673822152715,
1.80225950119297));
#92888=CARTESIAN_POINT('Ctrl Pts',(-5.1666860085911,-20.8660564184847,1.8025153204794));
#92889=CARTESIAN_POINT('Ctrl Pts',(-5.1676325256999,-20.8650539917672,1.80270874385327));
#92890=CARTESIAN_POINT('Ctrl Pts',(-5.16892428264733,-20.8636986921275,
1.80296985397145));
#92891=CARTESIAN_POINT('Ctrl Pts',(-5.17058106734596,-20.8620092639083,
1.80330799035701));
#92892=CARTESIAN_POINT('Ctrl Pts',(-5.1725050808472,-20.8600473416948,1.80370066598446));
#92893=CARTESIAN_POINT('Ctrl Pts',(-5.17492098970874,-20.8576352118099,
1.8041932137294));
#92894=CARTESIAN_POINT('Ctrl Pts',(-5.17787468853171,-20.8548243854623,
1.80479514724455));
#92895=CARTESIAN_POINT('Ctrl Pts',(-5.1792155093237,-20.8535484211087,1.80506839276513));
#92896=CARTESIAN_POINT('Ctrl Pts',(-5.18096220677253,-20.851916394557,1.80541625744203));
#92897=CARTESIAN_POINT('Ctrl Pts',(-5.18272412749508,-20.8503133827491,
1.80577433408361));
#92898=CARTESIAN_POINT('Ctrl Pts',(-5.18455593116523,-20.8486467907875,
1.80614661309585));
#92899=CARTESIAN_POINT('Ctrl Pts',(-5.18640420676291,-20.8470119466033,
1.80652993493292));
#92900=CARTESIAN_POINT('Ctrl Pts',(-5.1877915946851,-20.8458061052139,1.80681508756679));
#92901=CARTESIAN_POINT('Ctrl Pts',(-5.18800943258993,-20.8456167724702,
1.8068598602301));
#92902=CARTESIAN_POINT('Ctrl Pts',(-5.18821584645905,-20.8454379528746,
1.80690215364221));
#92903=CARTESIAN_POINT('Ctrl Pts',(-5.18840893352295,-20.8452711264075,
1.80694149257333));
#92904=CARTESIAN_POINT('Ctrl Pts',(-5.1936202871629,-20.8407685372677,1.80800323683386));
#92905=CARTESIAN_POINT('Ctrl Pts',(-5.19865361893382,-20.8367359737122,
1.80903280841691));
#92906=CARTESIAN_POINT('Ctrl Pts',(-5.2034457792482,-20.8331144155368,1.81001714106857));
#92907=CARTESIAN_POINT('Ctrl Pts',(-5.20584185940539,-20.8313036364491,
1.8105093073944));
#92908=CARTESIAN_POINT('Ctrl Pts',(-5.20817788729427,-20.8295956268,1.81099021388227));
#92909=CARTESIAN_POINT('Ctrl Pts',(-5.21044732529831,-20.8279832426908,
1.81145850828711));
#92910=CARTESIAN_POINT('Ctrl Pts',(-5.21158204430033,-20.8271770506363,
1.81169265548952));
#92911=CARTESIAN_POINT('Ctrl Pts',(-5.21270012169541,-20.8263947736905,
1.81192365088883));
#92912=CARTESIAN_POINT('Ctrl Pts',(-5.21380082865156,-20.8256355352479,
1.81215134374786));
#92913=CARTESIAN_POINT('Ctrl Pts',(-5.2145476908534,-20.8251203695249,1.81230584008232));
#92914=CARTESIAN_POINT('Ctrl Pts',(-5.21576632620745,-20.8242901399562,
1.81255684264991));
#92915=CARTESIAN_POINT('Ctrl Pts',(-5.21648082540202,-20.8238087349836,
1.81270562152336));
#92916=CARTESIAN_POINT('Ctrl Pts',(-5.2168193373676,-20.8235806572688,1.81277610925697));
#92917=CARTESIAN_POINT('Ctrl Pts',(-5.21704411632927,-20.8234301284241,
1.81282312096779));
#92918=CARTESIAN_POINT('Ctrl Pts',(-5.21705013203587,-20.8234260963392,
1.8128243686639));
#92919=CARTESIAN_POINT('Ctrl Pts',(-5.21712543227981,-20.8233756256304,
1.81283998641723));
#92920=CARTESIAN_POINT('Ctrl Pts',(-5.21794283507666,-20.8228205263349,
1.81302715496386));
#92921=CARTESIAN_POINT('Ctrl Pts',(-5.21951437433468,-20.8217883955223,
1.81336586433952));
#92922=CARTESIAN_POINT('Ctrl Pts',(-5.22109550447098,-20.8207499657638,
1.81370664080983));
#92923=CARTESIAN_POINT('Ctrl Pts',(-5.22344024804095,-20.8192284429785,
1.81420110808858));
#92924=CARTESIAN_POINT('Ctrl Pts',(-5.22658729860372,-20.8172915736929,
1.81485262134387));
#92925=CARTESIAN_POINT('Ctrl Pts',(-5.22971685572864,-20.8153654708383,
1.81550051304735));
#92926=CARTESIAN_POINT('Ctrl Pts',(-5.23364039011882,-20.8130282348166,
1.81630427268963));
#92927=CARTESIAN_POINT('Ctrl Pts',(-5.23841592276139,-20.8103901583995,
1.81728413247834));
#92928=CARTESIAN_POINT('Ctrl Pts',(-5.2430438977556,-20.8078335950578,1.81823371589435));
#92929=CARTESIAN_POINT('Ctrl Pts',(-5.24847286282806,-20.8049942587288,
1.8193494472573));
#92930=CARTESIAN_POINT('Ctrl Pts',(-5.25476408162235,-20.8020181237148,
1.8206558715834));
#92931=CARTESIAN_POINT('Ctrl Pts',(-5.26085974723718,-20.7991344974314,
1.82192168765233));
#92932=CARTESIAN_POINT('Ctrl Pts',(-5.26775980090195,-20.7961293482283,
1.82332050551907));
#92933=CARTESIAN_POINT('Ctrl Pts',(-5.27551754699974,-20.7931746130028,
1.82489808968304));
#92934=CARTESIAN_POINT('Ctrl Pts',(-5.28273403840939,-20.7904260284135,
1.82636560646225));
#92935=CARTESIAN_POINT('Ctrl Pts',(-5.2906934607079,-20.7877214605548,1.82798843561937));
#92936=CARTESIAN_POINT('Ctrl Pts',(-5.29942286128885,-20.7852385908721,
1.82978958090487));
#92937=CARTESIAN_POINT('Ctrl Pts',(-5.30778785157575,-20.7828593690015,
1.83151553707779));
#92938=CARTESIAN_POINT('Ctrl Pts',(-5.31686057569694,-20.7806841633692,
1.83340582143119));
#92939=CARTESIAN_POINT('Ctrl Pts',(-5.3266394453264,-20.7789010890687,1.83545887229495));
#92940=CARTESIAN_POINT('Ctrl Pts',(-5.33583825993341,-20.7772237817169,
1.83739014196007));
#92941=CARTESIAN_POINT('Ctrl Pts',(-5.34566235646555,-20.7758941532551,
1.8394657905466));
#92942=CARTESIAN_POINT('Ctrl Pts',(-5.35607973455985,-20.7750893176935,
1.84165835473634));
#92943=CARTESIAN_POINT('Ctrl Pts',(-5.36318972295453,-20.7745400075454,
1.84315480670367));
#92944=CARTESIAN_POINT('Ctrl Pts',(-5.37057545291419,-20.7742356128,1.84470518673479));
#92945=CARTESIAN_POINT('Ctrl Pts',(-5.3782162351,-20.7742356128,1.84629187045));
#92946=CARTESIAN_POINT('Origin',(1.126325016E-16,-20.7742356128,0.729452270839));
#92947=CARTESIAN_POINT('Origin',(2.57175827821E-16,-21.0742356128,0.729452270839));
#92948=CARTESIAN_POINT('Origin',(-5.92013962829,-21.0742356128,1.84629187045));
#92949=CARTESIAN_POINT('',(-5.92013962829,-21.0742356128,2.14629187045));
#92950=CARTESIAN_POINT('Origin',(-5.92013962829,-21.0742356128,1.84629187045));
#92951=CARTESIAN_POINT('Origin',(-5.92013962829,-21.0742356128,1.84629187045));
#92952=CARTESIAN_POINT('Origin',(-5.3782162351,-21.0742356128,1.84629187045));
#92953=CARTESIAN_POINT('',(-5.3782162351,-21.0742356128,2.14629187045));
#92954=CARTESIAN_POINT('Origin',(-5.3782162351,-21.0742356128,1.84629187045));
#92955=CARTESIAN_POINT('Origin',(-5.3782162351,-21.0742356128,1.84629187045));
#92956=CARTESIAN_POINT('Origin',(-3.31206782846,-21.0742356128,5.11154620667));
#92957=CARTESIAN_POINT('',(-3.13117783752,-21.0742356128,4.87221628548));
#92958=CARTESIAN_POINT('Origin',(-3.31206782846,-21.0742356128,5.11154620667));
#92959=CARTESIAN_POINT('Origin',(-3.31206782846,-21.0742356128,5.11154620667));
#92960=CARTESIAN_POINT('Origin',(-5.60029074364,-21.0742356128,1.84629187045));
#92961=CARTESIAN_POINT('',(-5.6491779317,-20.7742356128,1.84629187045));
#92962=CARTESIAN_POINT('',(-5.6491779317,-21.0742356128,2.14629187045));
#92963=CARTESIAN_POINT('Origin',(1.47842115491E-15,-21.0742356128,0.729452270839));
#92964=CARTESIAN_POINT('',(-4.2092958712,-21.0742356128,3.77060280966));
#92965=CARTESIAN_POINT('',(-4.452469377,-20.7742356128,3.94629187045));
#92966=CARTESIAN_POINT('Ctrl Pts',(-4.20929587120239,-21.0742356128,3.77060280966173));
#92967=CARTESIAN_POINT('Ctrl Pts',(-4.20929587120239,-21.0567670633141,
3.77060280966173));
#92968=CARTESIAN_POINT('Ctrl Pts',(-4.21053420664878,-21.039288104426,3.7714875497586));
#92969=CARTESIAN_POINT('Ctrl Pts',(-4.21302952672439,-21.0219367655753,
3.77327918596831));
#92970=CARTESIAN_POINT('Ctrl Pts',(-4.21552484680001,-21.0045854267246,
3.77507082217803));
#92971=CARTESIAN_POINT('Ctrl Pts',(-4.21927769717971,-20.9873595047338,
3.77776973840221));
#92972=CARTESIAN_POINT('Ctrl Pts',(-4.22434041182606,-20.9704316655761,
3.78142247514592));
#92973=CARTESIAN_POINT('Ctrl Pts',(-4.2290076878942,-20.9548260262887,3.78478990388288));
#92974=CARTESIAN_POINT('Ctrl Pts',(-4.23478878393056,-20.9394753388172,
3.78897006104767));
#92975=CARTESIAN_POINT('Ctrl Pts',(-4.24173245519993,-20.9245813330018,
3.79399759136516));
#92976=CARTESIAN_POINT('Ctrl Pts',(-4.24232076312392,-20.9233194268283,
3.79442355276356));
#92977=CARTESIAN_POINT('Ctrl Pts',(-4.24291741501226,-20.9220608303557,
3.79485559592467));
#92978=CARTESIAN_POINT('Ctrl Pts',(-4.24352243904187,-20.9208056843632,
3.79529374087375));
#92979=CARTESIAN_POINT('Ctrl Pts',(-4.24637370724739,-20.9148906170492,
3.79735856590814));
#92980=CARTESIAN_POINT('Ctrl Pts',(-4.2494837284245,-20.9089093610656,3.79961172647346));
#92981=CARTESIAN_POINT('Ctrl Pts',(-4.25278436811486,-20.9030443905848,
3.8020023595835));
#92982=CARTESIAN_POINT('Ctrl Pts',(-4.25609549745106,-20.8971607808496,
3.80440059027976));
#92983=CARTESIAN_POINT('Ctrl Pts',(-4.25959825927427,-20.8913947792768,
3.80693702485545));
#92984=CARTESIAN_POINT('Ctrl Pts',(-4.26318787729757,-20.8859011249233,
3.80953429455957));
#92985=CARTESIAN_POINT('Ctrl Pts',(-4.26574097359176,-20.8819937931457,
3.81138158850939));
#92986=CARTESIAN_POINT('Ctrl Pts',(-4.26833719887337,-20.8782235763595,
3.81325907226093));
#92987=CARTESIAN_POINT('Ctrl Pts',(-4.27092931133313,-20.8746352746839,
3.81513200774992));
#92988=CARTESIAN_POINT('Ctrl Pts',(-4.27772396722458,-20.8652293266398,
3.82004149850395));
#92989=CARTESIAN_POINT('Ctrl Pts',(-4.28525987940435,-20.8559988435105,
3.82547188896741));
#92990=CARTESIAN_POINT('Ctrl Pts',(-4.29358234259888,-20.8471407335453,
3.83147537999488));
#92991=CARTESIAN_POINT('Ctrl Pts',(-4.29734859711526,-20.8431320769874,
3.83419220489007));
#92992=CARTESIAN_POINT('Ctrl Pts',(-4.30127563429279,-20.8392002484946,
3.83702618686642));
#92993=CARTESIAN_POINT('Ctrl Pts',(-4.30536586453391,-20.8353663275283,
3.83998090287142));
#92994=CARTESIAN_POINT('Ctrl Pts',(-4.31193016316833,-20.8292133726383,
3.84472284576788));
#92995=CARTESIAN_POINT('Ctrl Pts',(-4.31891569582986,-20.8233125443284,
3.84977500785908));
#92996=CARTESIAN_POINT('Ctrl Pts',(-4.32632635631929,-20.8177620044615,
3.85513691010998));
#92997=CARTESIAN_POINT('Ctrl Pts',(-4.330031686564,-20.8149867345281,3.85781786123542));
#92998=CARTESIAN_POINT('Ctrl Pts',(-4.33384315336668,-20.8122992204208,
3.86057600867429));
#92999=CARTESIAN_POINT('Ctrl Pts',(-4.3377602566725,-20.8097127162401,3.86340969540574));
#93000=CARTESIAN_POINT('Ctrl Pts',(-4.33948117149357,-20.8085763782291,
3.8646546289992));
#93001=CARTESIAN_POINT('Ctrl Pts',(-4.3414979467098,-20.8072824582389,3.86611317481211));
#93002=CARTESIAN_POINT('Ctrl Pts',(-4.34345078725751,-20.8060737953689,
3.86752521019504));
#93003=CARTESIAN_POINT('Ctrl Pts',(-4.34561904450574,-20.8047318056033,
3.86909300637654));
#93004=CARTESIAN_POINT('Ctrl Pts',(-4.34770824252956,-20.8034950021666,
3.87060329056719));
#93005=CARTESIAN_POINT('Ctrl Pts',(-4.34920034244517,-20.8026314786707,
3.87168154390545));
#93006=CARTESIAN_POINT('Ctrl Pts',(-4.34942324250476,-20.8025024796428,
3.87184262074142));
#93007=CARTESIAN_POINT('Ctrl Pts',(-4.34963278664701,-20.8023817233861,
3.87199403392379));
#93008=CARTESIAN_POINT('Ctrl Pts',(-4.34982722465402,-20.8022700347198,
3.87213451813516));
#93009=CARTESIAN_POINT('Ctrl Pts',(-4.35516377370196,-20.7992046255698,
3.87599025033482));
#93010=CARTESIAN_POINT('Ctrl Pts',(-4.36125806845615,-20.7959906141422,
3.88039336313273));
#93011=CARTESIAN_POINT('Ctrl Pts',(-4.36815945129353,-20.7928434952946,
3.8853795348017));
#93012=CARTESIAN_POINT('Ctrl Pts',(-4.37448994688551,-20.789956708333,3.88995324684102));
#93013=CARTESIAN_POINT('Ctrl Pts',(-4.38150021419207,-20.7871267873611,
3.89501804152803));
#93014=CARTESIAN_POINT('Ctrl Pts',(-4.38921284910019,-20.7845634272244,
3.90059026672928));
#93015=CARTESIAN_POINT('Ctrl Pts',(-4.39666085655732,-20.7820880182831,
3.9059713038646));
#93016=CARTESIAN_POINT('Ctrl Pts',(-4.40476457688503,-20.7798615624639,
3.91182606547739));
#93017=CARTESIAN_POINT('Ctrl Pts',(-4.41351920705256,-20.7781089820743,
3.91815110222087));
#93018=CARTESIAN_POINT('Ctrl Pts',(-4.42183641148545,-20.7764439694917,
3.9241601080423));
#93019=CARTESIAN_POINT('Ctrl Pts',(-4.43074160378321,-20.7752072573721,
3.93059392855731));
#93020=CARTESIAN_POINT('Ctrl Pts',(-4.44019906484498,-20.7746177736591,
3.93742677551188));
#93021=CARTESIAN_POINT('Ctrl Pts',(-4.44419274238802,-20.7743688476681,
3.94031213631424));
#93022=CARTESIAN_POINT('Ctrl Pts',(-4.44828445852957,-20.7742356127999,
3.94326833220267));
#93023=CARTESIAN_POINT('Ctrl Pts',(-4.452469377,-20.7742356128,3.94629187045));
#93024=CARTESIAN_POINT('Origin',(2.57175827821E-16,-21.0742356128,0.729452270839));
#93025=CARTESIAN_POINT('Origin',(1.126325016E-16,-20.7742356128,0.729452270839));
#93026=CARTESIAN_POINT('Origin',(-1.05,-22.8742356128,-4.99584562937));
#93027=CARTESIAN_POINT('',(-0.972828518105,-23.1742356128,-4.40082919062));
#93028=CARTESIAN_POINT('Origin',(-1.05,-23.1742356128,-4.99584562937));
#93029=CARTESIAN_POINT('',(-1.01141425905,-22.8742356128,-4.69833741));
#93030=CARTESIAN_POINT('Origin',(-0.972828518105,-22.8742356128,-4.40082919062));
#93031=CARTESIAN_POINT('Origin',(-1.05,-22.8742356128,-4.99584562937));
#93032=CARTESIAN_POINT('Origin',(-0.00234331738835,-22.8742356128,3.08191746407));
#93033=CARTESIAN_POINT('',(-4.23842172091,-23.1742356128,-3.16219806837));
#93034=CARTESIAN_POINT('Origin',(-0.00234331738835,-23.1742356128,3.08191746407));
#93035=CARTESIAN_POINT('',(-4.40684492179,-22.8742356128,-3.41045927235));
#93036=CARTESIAN_POINT('Origin',(-4.23842172091,-22.8742356128,-3.16219806837));
#93037=CARTESIAN_POINT('Origin',(-0.00234331738835,-22.8742356128,3.08191746407));
#93038=CARTESIAN_POINT('Origin',(-6.34552156645,-22.8742356128,-5.5301356238));
#93039=CARTESIAN_POINT('',(-6.56346233154,-22.8742356128,-5.32397592135));
#93040=CARTESIAN_POINT('',(-6.78140309663,-23.1742356128,-5.11781621891));
#93041=CARTESIAN_POINT('Origin',(-6.78140309663,-22.8742356128,-5.11781621891));
#93042=CARTESIAN_POINT('Origin',(-6.34552156645,-23.1742356128,-5.5301356238));
#93043=CARTESIAN_POINT('Origin',(-6.34552156645,-22.8742356128,-5.5301356238));
#93044=CARTESIAN_POINT('Origin',(-4.57526812267,-22.8742356128,-3.65872047634));
#93045=CARTESIAN_POINT('',(-5.01114965285,-23.1742356128,-3.24640107146));
#93046=CARTESIAN_POINT('Origin',(-4.57526812267,-23.1742356128,-3.65872047634));
#93047=CARTESIAN_POINT('',(-4.79320888776,-22.8742356128,-3.4525607739));
#93048=CARTESIAN_POINT('Origin',(-5.01114965285,-22.8742356128,-3.24640107146));
#93049=CARTESIAN_POINT('Origin',(-4.57526812267,-22.8742356128,-3.65872047634));
#93050=CARTESIAN_POINT('Origin',(-1.2614400074,-21.0742356128,6.07560132137));
#93051=CARTESIAN_POINT('',(-1.19254592572,-21.0742356128,5.78361912069));
#93052=CARTESIAN_POINT('Origin',(-1.2614400074,-21.0742356128,6.07560132137));
#93053=CARTESIAN_POINT('Origin',(-1.2614400074,-21.0742356128,6.07560132137));
#93054=CARTESIAN_POINT('Origin',(-1.71825752818E-13,-21.9742356128,-5.63016324424));
#93055=CARTESIAN_POINT('',(-0.246933912590001,-21.0742356137361,-6.5991955009251));
#93056=CARTESIAN_POINT('Origin',(-1.72570291390173E-13,-21.0742355071906,
-5.63016324424002));
#93057=CARTESIAN_POINT('',(-0.246934184763,-21.3732856128,-6.59919549778));
#93058=CARTESIAN_POINT('Origin',(2.84607155346,-21.3642356128,5.53854202767));
#93059=CARTESIAN_POINT('',(-0.530881033960364,-21.0742356128,-6.52327988866722));
#93060=CARTESIAN_POINT('',(-0.530881036642,-22.1242356128,-6.52327988851));
#93061=CARTESIAN_POINT('Origin',(2.84607155346,-21.0742356128,5.53854202767));
#93062=CARTESIAN_POINT('Origin',(-0.45,-22.8742356128,-6.23438845923));
#93063=CARTESIAN_POINT('Origin',(-0.45,-22.8742356128,-6.23438845923));
#93064=CARTESIAN_POINT('Ctrl Pts',(7.715616340275E-16,-20.7742356128,-6.9673210071));
#93065=CARTESIAN_POINT('Ctrl Pts',(7.715616340275E-16,-20.7742356128,-6.9673210071));
#93066=CARTESIAN_POINT('Ctrl Pts',(7.715616340275E-16,-20.7742356128,-6.9673210071));
#93067=CARTESIAN_POINT('Ctrl Pts',(7.715616340275E-16,-20.7742356128,-6.9673210071));
#93068=CARTESIAN_POINT('Ctrl Pts',(7.715616340275E-16,-20.7742356128,-6.9673210071));
#93069=CARTESIAN_POINT('Ctrl Pts',(7.715616340275E-16,-20.7742356128,-6.9673210071));
#93070=CARTESIAN_POINT('Ctrl Pts',(0.0620789114664,-20.7727817153,-6.86712083978));
#93071=CARTESIAN_POINT('Ctrl Pts',(0.0372447941938,-20.7727814769555,-6.86710441347656));
#93072=CARTESIAN_POINT('Ctrl Pts',(0.0124139553071,-20.7727812105989,-6.8670860566289));
#93073=CARTESIAN_POINT('Ctrl Pts',(-0.0124139554138,-20.7727812105989,-6.8670860566289));
#93074=CARTESIAN_POINT('Ctrl Pts',(-0.0372447942657,-20.7727814769555,-6.86710441347656));
#93075=CARTESIAN_POINT('Ctrl Pts',(-0.0620789114664,-20.7727817153,-6.86712083978));
#93076=CARTESIAN_POINT('Ctrl Pts',(0.126706651057,-20.809097628,-6.7683471563));
#93077=CARTESIAN_POINT('Ctrl Pts',(0.0760530156428,-20.8106930399,-6.76865483887));
#93078=CARTESIAN_POINT('Ctrl Pts',(0.0253584233265,-20.8114382347,-6.76885772281));
#93079=CARTESIAN_POINT('Ctrl Pts',(-0.0253584229554,-20.8114382347,-6.76885772281));
#93080=CARTESIAN_POINT('Ctrl Pts',(-0.0760530153923,-20.8106930399,-6.76865483887));
#93081=CARTESIAN_POINT('Ctrl Pts',(-0.126706651057,-20.809097628,-6.7683471563));
#93082=CARTESIAN_POINT('Ctrl Pts',(0.185538258403,-20.8478771982,-6.68330934255));
#93083=CARTESIAN_POINT('Ctrl Pts',(0.111595913132,-20.8641740172,-6.68722155122));
#93084=CARTESIAN_POINT('Ctrl Pts',(0.0372374622574,-20.8723993359,-6.68904882319));
#93085=CARTESIAN_POINT('Ctrl Pts',(-0.0372374612746,-20.8723993359,-6.68904882319));
#93086=CARTESIAN_POINT('Ctrl Pts',(-0.111595912483,-20.8641740172,-6.68722155122));
#93087=CARTESIAN_POINT('Ctrl Pts',(-0.185538258404,-20.8478771982,-6.68330934255));
#93088=CARTESIAN_POINT('Ctrl Pts',(0.248193078621,-20.9544277624,-6.59756027965));
#93089=CARTESIAN_POINT('Ctrl Pts',(0.151037451012,-20.9653225623,-6.62292642142));
#93090=CARTESIAN_POINT('Ctrl Pts',(0.0507127937414,-20.9709039046,-6.63587730141));
#93091=CARTESIAN_POINT('Ctrl Pts',(-0.0507127941925,-20.9709039046,-6.63587730141));
#93092=CARTESIAN_POINT('Ctrl Pts',(-0.15103745131,-20.9653225623,-6.62292642142));
#93093=CARTESIAN_POINT('Ctrl Pts',(-0.248193078621,-20.9544277624,-6.59756027965));
#93094=CARTESIAN_POINT('Ctrl Pts',(0.246933661348,-21.0742356173,-6.5991953663));
#93095=CARTESIAN_POINT('Ctrl Pts',(0.15021854742,-21.0742356301,-6.62384075504));
#93096=CARTESIAN_POINT('Ctrl Pts',(0.0504287451839,-21.0742356366,-6.63642024334));
#93097=CARTESIAN_POINT('Ctrl Pts',(-0.0504287451839,-21.0742356366,-6.63642024334));
#93098=CARTESIAN_POINT('Ctrl Pts',(-0.15021854742,-21.0742356301,-6.62384075504));
#93099=CARTESIAN_POINT('Ctrl Pts',(-0.246933661348,-21.0742356173,-6.5991953663));
#93100=CARTESIAN_POINT('Ctrl Pts',(-6.57550091203307E-15,-20.7742356128,
-6.96732100709999));
#93101=CARTESIAN_POINT('Ctrl Pts',(-0.000739046140776542,-20.7742183042276,
-6.96612812943488));
#93102=CARTESIAN_POINT('Ctrl Pts',(-0.00213178760716483,-20.7741874385235,
-6.96388034917257));
#93103=CARTESIAN_POINT('Ctrl Pts',(-0.00418474029193665,-20.7742053701667,
-6.9605765338024));
#93104=CARTESIAN_POINT('Ctrl Pts',(-0.00641465514642071,-20.774224847497,
-6.95698793333194));
#93105=CARTESIAN_POINT('Ctrl Pts',(-0.00942378940812995,-20.7743021658575,
-6.95215281744824));
#93106=CARTESIAN_POINT('Ctrl Pts',(-0.0132219688318108,-20.7745826669425,
-6.94607879927397));
#93107=CARTESIAN_POINT('Ctrl Pts',(-0.0170201482554917,-20.7748631680274,
-6.94000478109969));
#93108=CARTESIAN_POINT('Ctrl Pts',(-0.0216078184058048,-20.7753481037327,
-6.93269120520879));
#93109=CARTESIAN_POINT('Ctrl Pts',(-0.0269904576317545,-20.7762314335538,
-6.9241638748923));
#93110=CARTESIAN_POINT('Ctrl Pts',(-0.0323089928856136,-20.777104243452,
-6.91573809991356));
#93111=CARTESIAN_POINT('Ctrl Pts',(-0.0383968143842043,-20.7783663975252,
-6.9061281889125));
#93112=CARTESIAN_POINT('Ctrl Pts',(-0.0452340558275931,-20.7802380903564,
-6.8953994038545));
#93113=CARTESIAN_POINT('Ctrl Pts',(-0.0485017240992391,-20.7811326135833,
-6.89027188118068));
#93114=CARTESIAN_POINT('Ctrl Pts',(-0.051940429322601,-20.7821668181412,
-6.88488924067781));
#93115=CARTESIAN_POINT('Ctrl Pts',(-0.0555471514172319,-20.7833679719454,
-6.87926140234126));
#93116=CARTESIAN_POINT('Ctrl Pts',(-0.0595526878616734,-20.7847019436826,
-6.87301126413569));
#93117=CARTESIAN_POINT('Ctrl Pts',(-0.063127261239606,-20.7860232276961,
-6.86746021183157));
#93118=CARTESIAN_POINT('Ctrl Pts',(-0.0664331293085701,-20.7873256017318,
-6.86234415039677));
#93119=CARTESIAN_POINT('Ctrl Pts',(-0.0700590269614373,-20.7887540540658,
-6.85673282085748));
#93120=CARTESIAN_POINT('Ctrl Pts',(-0.0733617729652654,-20.7901604262365,
-6.85164463855104));
#93121=CARTESIAN_POINT('Ctrl Pts',(-0.0765514209480796,-20.7915988864223,
-6.84674347698261));
#93122=CARTESIAN_POINT('Ctrl Pts',(-0.0785513039528601,-20.7925007891069,
-6.84367048906131));
#93123=CARTESIAN_POINT('Ctrl Pts',(-0.0805066452710636,-20.7934164265047,
-6.84067126660403));
#93124=CARTESIAN_POINT('Ctrl Pts',(-0.0824682378119286,-20.7943690054015,
-6.83766549654366));
#93125=CARTESIAN_POINT('Ctrl Pts',(-0.0920786456764894,-20.7990359642781,
-6.82293936171931));
#93126=CARTESIAN_POINT('Ctrl Pts',(-0.100960528456615,-20.8041428102936,
-6.80948841419464));
#93127=CARTESIAN_POINT('Ctrl Pts',(-0.109114333331388,-20.8094053876005,
-6.797269946806));
#93128=CARTESIAN_POINT('Ctrl Pts',(-0.114438108000665,-20.8128414246644,
-6.78929227648152));
#93129=CARTESIAN_POINT('Ctrl Pts',(-0.119451716877995,-20.8163450388597,
-6.78183955514836));
#93130=CARTESIAN_POINT('Ctrl Pts',(-0.12415772521919,-20.8198442769267,
-6.77489576919354));
#93131=CARTESIAN_POINT('Ctrl Pts',(-0.130114551502564,-20.824273583417,
-6.76610638258755));
#93132=CARTESIAN_POINT('Ctrl Pts',(-0.135577437715922,-20.82869661386,-6.7581295295839));
#93133=CARTESIAN_POINT('Ctrl Pts',(-0.140483820768466,-20.8329959479912,
-6.75092075220541));
#93134=CARTESIAN_POINT('Ctrl Pts',(-0.142937012294739,-20.8351456150569,
-6.74731636351616));
#93135=CARTESIAN_POINT('Ctrl Pts',(-0.145262555217202,-20.8372633999559,
-6.74390296005163));
#93136=CARTESIAN_POINT('Ctrl Pts',(-0.147467464851545,-20.8393348214145,
-6.74067276188158));
#93137=CARTESIAN_POINT('Ctrl Pts',(-0.148569919668717,-20.8403705321438,
-6.73905766279656));
#93138=CARTESIAN_POINT('Ctrl Pts',(-0.149642232430758,-20.84139465963,-6.73748836687227));
#93139=CARTESIAN_POINT('Ctrl Pts',(-0.150684903317464,-20.8424055801115,
-6.73596387258709));
#93140=CARTESIAN_POINT('Ctrl Pts',(-0.15131977036796,-20.8430211148047,
-6.73503563031748));
#93141=CARTESIAN_POINT('Ctrl Pts',(-0.151588988504639,-20.8432845686164,
-6.73464223535714));
#93142=CARTESIAN_POINT('Ctrl Pts',(-0.152141066761498,-20.8438275612463,
-6.73383575971623));
#93143=CARTESIAN_POINT('Ctrl Pts',(-0.152495691609109,-20.8441763499845,
-6.73331772391659));
#93144=CARTESIAN_POINT('Ctrl Pts',(-0.152967046458675,-20.844640439587,
-6.73262921807131));
#93145=CARTESIAN_POINT('Ctrl Pts',(-0.153724483183895,-20.8453971487028,
-6.73152382693266));
#93146=CARTESIAN_POINT('Ctrl Pts',(-0.165819652379691,-20.8574806990291,
-6.71387232892058));
#93147=CARTESIAN_POINT('Ctrl Pts',(-0.176794399150034,-20.8706467710759,
-6.69801435723457));
#93148=CARTESIAN_POINT('Ctrl Pts',(-0.186589072833805,-20.8845898753631,
-6.68394159693474));
#93149=CARTESIAN_POINT('Ctrl Pts',(-0.196711292295833,-20.8989992539839,
-6.66939822644683));
#93150=CARTESIAN_POINT('Ctrl Pts',(-0.205572200092412,-20.9142354112887,
-6.65676360713048));
#93151=CARTESIAN_POINT('Ctrl Pts',(-0.213142751347805,-20.9299280505707,
-6.64602128475438));
#93152=CARTESIAN_POINT('Ctrl Pts',(-0.220146036668008,-20.9444448310021,
-6.63608389102129));
#93153=CARTESIAN_POINT('Ctrl Pts',(-0.226045896532328,-20.9593494493265,
-6.62776573152344));
#93154=CARTESIAN_POINT('Ctrl Pts',(-0.230849786453082,-20.9743672314828,
-6.62103443567695));
#93155=CARTESIAN_POINT('Ctrl Pts',(-0.235484211608852,-20.9888552377771,
-6.61454059686787));
#93156=CARTESIAN_POINT('Ctrl Pts',(-0.239099720633237,-21.0034475477172,
-6.60952261522757));
#93157=CARTESIAN_POINT('Ctrl Pts',(-0.241718744711677,-21.0179417593159,
-6.60594163792155));
#93158=CARTESIAN_POINT('Ctrl Pts',(-0.244248413806021,-21.0319414622701,
-6.60248283519685));
#93159=CARTESIAN_POINT('Ctrl Pts',(-0.245849619786232,-21.0458498424135,
-6.60036330646126));
#93160=CARTESIAN_POINT('Ctrl Pts',(-0.246540851867042,-21.0595316198178,
-6.59955630271868));
#93161=CARTESIAN_POINT('Ctrl Pts',(-0.24679002646896,-21.0644636123177,
-6.59926539487183));
#93162=CARTESIAN_POINT('Ctrl Pts',(-0.246920851074132,-21.0693665923741,
-6.59914522303046));
#93163=CARTESIAN_POINT('Ctrl Pts',(-0.246933661366624,-21.0742356155283,
-6.59919536627582));
#93164=CARTESIAN_POINT('Origin',(2.84607155346,-21.0742356128,5.53854202767));
#93165=CARTESIAN_POINT('',(-1.05,-20.7742356128,-6.68100624476));
#93166=CARTESIAN_POINT('Ctrl Pts',(-1.05,-20.7742356128,-6.68100624476));
#93167=CARTESIAN_POINT('Ctrl Pts',(-1.03625292470594,-20.7740159455194,
-6.67687310983531));
#93168=CARTESIAN_POINT('Ctrl Pts',(-1.02237382634443,-20.7742867438727,
-6.67269596024792));
#93169=CARTESIAN_POINT('Ctrl Pts',(-1.00846284537523,-20.7749590260321,
-6.6685054782835));
#93170=CARTESIAN_POINT('Ctrl Pts',(-0.993968393349887,-20.7756595058564,
-6.66413923409621));
#93171=CARTESIAN_POINT('Ctrl Pts',(-0.979438879191048,-20.7767959613459,
-6.65975837854857));
#93172=CARTESIAN_POINT('Ctrl Pts',(-0.96494582937768,-20.7783083760812,
-6.65538485104873));
#93173=CARTESIAN_POINT('Ctrl Pts',(-0.949182506410178,-20.7799533495161,
-6.65062799673753));
#93174=CARTESIAN_POINT('Ctrl Pts',(-0.933461830247863,-20.782042980466,
-6.64587966075301));
#93175=CARTESIAN_POINT('Ctrl Pts',(-0.917834461394271,-20.7845474988965,
-6.64115542515622));
#93176=CARTESIAN_POINT('Ctrl Pts',(-0.908284964982968,-20.7860779478152,
-6.63826856228761));
#93177=CARTESIAN_POINT('Ctrl Pts',(-0.898769536443018,-20.7877642505962,
-6.63539046214858));
#93178=CARTESIAN_POINT('Ctrl Pts',(-0.889294615397127,-20.7896072434251,
-6.63252311810195));
#93179=CARTESIAN_POINT('Ctrl Pts',(-0.871011378197203,-20.7931635659407,
-6.62699016103724));
#93180=CARTESIAN_POINT('Ctrl Pts',(-0.852879229238803,-20.797300044157,
-6.62149721776252));
#93181=CARTESIAN_POINT('Ctrl Pts',(-0.834927156599105,-20.8020715544452,
-6.61605309569464));
#93182=CARTESIAN_POINT('Ctrl Pts',(-0.817519370509437,-20.8066983979351,
-6.61077403325401));
#93183=CARTESIAN_POINT('Ctrl Pts',(-0.800278528149882,-20.811923828354,
-6.60554014165193));
#93184=CARTESIAN_POINT('Ctrl Pts',(-0.783241385589988,-20.8178396330701,
-6.60036265094451));
#93185=CARTESIAN_POINT('Ctrl Pts',(-0.766995111590773,-20.8234808246023,
-6.5954255006938));
#93186=CARTESIAN_POINT('Ctrl Pts',(-0.75093240170514,-20.8297509634394,
-6.59053912116687));
#93187=CARTESIAN_POINT('Ctrl Pts',(-0.735123129947809,-20.8367492310671,
-6.58572501216975));
#93188=CARTESIAN_POINT('Ctrl Pts',(-0.721365830513912,-20.8428391550528,
-6.58153575285423));
#93189=CARTESIAN_POINT('Ctrl Pts',(-0.707800285523294,-20.8494811269749,
-6.57740117455926));
#93190=CARTESIAN_POINT('Ctrl Pts',(-0.694511943633331,-20.8567437051301,
-6.57334766925701));
#93191=CARTESIAN_POINT('Ctrl Pts',(-0.681861691477839,-20.8636575432691,
-6.56948880826353));
#93192=CARTESIAN_POINT('Ctrl Pts',(-0.669462246162125,-20.8711341867228,
-6.56570329210059));
#93193=CARTESIAN_POINT('Ctrl Pts',(-0.657430144764881,-20.8792291148818,
-6.56202717171159));
#93194=CARTESIAN_POINT('Ctrl Pts',(-0.646106591108891,-20.8868473480003,
-6.55856753111379));
#93195=CARTESIAN_POINT('Ctrl Pts',(-0.635108251855433,-20.8950134147344,
-6.55520473747399));
#93196=CARTESIAN_POINT('Ctrl Pts',(-0.624574744850416,-20.9037661637504,
-6.55198202898773));
#93197=CARTESIAN_POINT('Ctrl Pts',(-0.615767147388661,-20.9110847794763,
-6.5492873595799));
#93198=CARTESIAN_POINT('Ctrl Pts',(-0.607285106257906,-20.9188135257316,
-6.54669080698833));
#93199=CARTESIAN_POINT('Ctrl Pts',(-0.599236493259071,-20.9269691201472,
-6.54422580515893));
#93200=CARTESIAN_POINT('Ctrl Pts',(-0.590128979800226,-20.9361976898294,
-6.54143650005251));
#93201=CARTESIAN_POINT('Ctrl Pts',(-0.581575283606785,-20.9459732020675,
-6.53881527683606));
#93202=CARTESIAN_POINT('Ctrl Pts',(-0.573774149863334,-20.9563085906836,
-6.53642377787523));
#93203=CARTESIAN_POINT('Ctrl Pts',(-0.56627503412483,-20.9662438485556,
-6.53412486491134));
#93204=CARTESIAN_POINT('Ctrl Pts',(-0.559471283802019,-20.9766965655441,
-6.53203821531165));
#93205=CARTESIAN_POINT('Ctrl Pts',(-0.553583731234507,-20.9876651913132,
-6.53023237010088));
#93206=CARTESIAN_POINT('Ctrl Pts',(-0.547811914458446,-20.9984181990356,
-6.52846202366864));
#93207=CARTESIAN_POINT('Ctrl Pts',(-0.542920470100945,-21.0096671438262,
-6.52696149994591));
#93208=CARTESIAN_POINT('Ctrl Pts',(-0.539162633367657,-21.0213962266405,
-6.52580944852247));
#93209=CARTESIAN_POINT('Ctrl Pts',(-0.535502136482079,-21.0328214891412,
-6.52468723887186));
#93210=CARTESIAN_POINT('Ctrl Pts',(-0.532917204308461,-21.0447024126547,
-6.5238956579284));
#93211=CARTESIAN_POINT('Ctrl Pts',(-0.531686808004321,-21.0570093207758,
-6.52352140235709));
#93212=CARTESIAN_POINT('Ctrl Pts',(-0.53112156681897,-21.062663085592,-6.52334947022267));
#93213=CARTESIAN_POINT('Ctrl Pts',(-0.530842835073694,-21.068406533619,
-6.52326581257046));
#93214=CARTESIAN_POINT('Ctrl Pts',(-0.530881032646531,-21.0742356128,-6.52327988721974));
#93215=CARTESIAN_POINT('Origin',(2.84607155346,-20.7742356128,5.53854202767));
#93216=CARTESIAN_POINT('Origin',(-2.45,-20.1742356128,10.7304528845));
#93217=CARTESIAN_POINT('',(-2.45,-19.6742356128,10.4304528845));
#93218=CARTESIAN_POINT('',(-2.75,-19.6742356128,10.7304528845));
#93219=CARTESIAN_POINT('Origin',(-2.45,-19.6742356128,10.7304528845));
#93220=CARTESIAN_POINT('',(-2.75,-20.6742356128,10.7304528845));
#93221=CARTESIAN_POINT('',(-2.75,-20.1742356128,10.7304528845));
#93222=CARTESIAN_POINT('',(-2.45,-20.6742356128,10.4304528845));
#93223=CARTESIAN_POINT('Origin',(-2.45,-20.6742356128,10.7304528845));
#93224=CARTESIAN_POINT('',(-2.45,-20.1742356128,10.4304528845));
#93225=CARTESIAN_POINT('Origin',(1.47842115491E-15,-21.0742356128,0.729452270839));
#93226=CARTESIAN_POINT('',(-0.992653804111,-21.0742356128,5.82664824081));
#93227=CARTESIAN_POINT('Origin',(2.57175827821E-16,-21.0742356128,0.729452270839));
#93228=CARTESIAN_POINT('',(-1.05,-20.7742356128,6.12111625914));
#93229=CARTESIAN_POINT('Origin',(-1.04999999999979,-21.0742356128,6.12111625913628));
#93230=CARTESIAN_POINT('Origin',(1.126325016E-16,-20.7742356128,0.729452270839));
#93231=CARTESIAN_POINT('Origin',(9.79717439318E-17,-22.3742356128,0.729452270839));
#93232=CARTESIAN_POINT('',(-10.7000575594,-22.3742356128,-2.76302312605));
#93233=CARTESIAN_POINT('',(-10.9449284019,-22.3742356128,-2.34954507713));
#93234=CARTESIAN_POINT('Origin',(-11.0821857629,-22.3742356128,-2.71007990903));
#93235=CARTESIAN_POINT('Origin',(2.84607155346,-22.3742356128,5.53854202767));
#93236=CARTESIAN_POINT('Origin',(2.84607155346,-19.6742356128,5.53854202767));
#93237=CARTESIAN_POINT('',(-11.2744572343,-19.3742356128,-1.7432341771));
#93238=CARTESIAN_POINT('Origin',(-11.2744572343,-19.6742356128,-1.7432341771));
#93239=CARTESIAN_POINT('',(-12.6801076867,-19.3742356128,8.90771939699));
#93240=CARTESIAN_POINT('Origin',(-12.6801076867,-19.6742356128,8.90771939699));
#93241=CARTESIAN_POINT('Origin',(2.84607155346,-19.3742356128,5.53854202767));
#93242=CARTESIAN_POINT('Origin',(-8.94493678676E-16,-19.6742356128,0.580061096523));
#93243=CARTESIAN_POINT('',(-12.1784262599,-19.3742356128,9.98548517727));
#93244=CARTESIAN_POINT('Origin',(-12.1784262599,-19.6742356128,9.98548517727));
#93245=CARTESIAN_POINT('',(-3.05,-19.3742356128,15.662287998));
#93246=CARTESIAN_POINT('Origin',(-3.05,-19.6742356128,15.662287998));
#93247=CARTESIAN_POINT('Origin',(1.21374489213E-15,-19.3742356128,0.580061096523));
#93248=CARTESIAN_POINT('Origin',(-1.01908995768E-15,-19.4742356128,-4.23765442876));
#93249=CARTESIAN_POINT('',(3.35920145722,-19.3742356128,-2.84622762644));
#93250=CARTESIAN_POINT('Origin',(3.35920145722,-19.4742356128,-2.84622762644));
#93251=CARTESIAN_POINT('',(0.153073372946,-19.3742356128,-4.17424936164));
#93252=CARTESIAN_POINT('',(1.75613741508,-19.3742356128,-3.51023849404));
#93253=CARTESIAN_POINT('Origin',(0.153073372946,-19.4742356128,-4.17424936164));
#93254=CARTESIAN_POINT('Origin',(-1.62738508975E-15,-19.4742356128,5.69655897044));
#93255=CARTESIAN_POINT('',(0.153073372946,-19.3742356128,5.63315390332));
#93256=CARTESIAN_POINT('Origin',(0.153073372946,-19.4742356128,5.63315390332));
#93257=CARTESIAN_POINT('',(3.35920145722,-19.3742356128,4.30513216811));
#93258=CARTESIAN_POINT('',(1.75613741508,-19.3742356128,4.96914303572));
#93259=CARTESIAN_POINT('Origin',(3.35920145722,-19.4742356128,4.30513216811));
#93260=CARTESIAN_POINT('Origin',(3.20612808427,-19.4742356128,3.93558035511));
#93261=CARTESIAN_POINT('',(3.57567989727,-19.3742356128,4.08865372805));
#93262=CARTESIAN_POINT('Origin',(3.20612808427,-19.3742356128,3.93558035511));
#93263=CARTESIAN_POINT('Origin',(3.57567989727,-19.4742356128,4.08865372805));
#93264=CARTESIAN_POINT('Origin',(4.11560885829,-19.4742356128,2.78514990766));
#93265=CARTESIAN_POINT('',(4.90370163248,-19.3742356128,0.882525643785));
#93266=CARTESIAN_POINT('',(4.23969076488,-19.3742356128,2.48558968592));
#93267=CARTESIAN_POINT('Origin',(4.90370163248,-19.4742356128,0.882525643785));
#93268=CARTESIAN_POINT('Origin',(4.53414981948,-19.4742356128,0.729452270839));
#93269=CARTESIAN_POINT('',(4.90370163248,-19.3742356128,0.576378897893));
#93270=CARTESIAN_POINT('Origin',(4.53414981948,-19.3742356128,0.729452270839));
#93271=CARTESIAN_POINT('Origin',(4.90370163248,-19.4742356128,0.576378897893));
#93272=CARTESIAN_POINT('Origin',(5.81860454091,-19.4742356128,2.78514990766));
#93273=CARTESIAN_POINT('',(3.57567989727,-19.3742356128,-2.62974918638));
#93274=CARTESIAN_POINT('',(4.23969076488,-19.3742356128,-1.02668514424));
#93275=CARTESIAN_POINT('Origin',(3.57567989727,-19.4742356128,-2.62974918638));
#93276=CARTESIAN_POINT('Origin',(3.20612808427,-19.4742356128,-2.47667581343));
#93277=CARTESIAN_POINT('Origin',(3.20612808427,-19.3742356128,-2.47667581343));
#93278=CARTESIAN_POINT('Origin',(1.61893433855E-15,-19.4742356128,-3.80469754864));
#93279=CARTESIAN_POINT('',(-0.153073372946,-19.3742356128,-4.17424936164));
#93280=CARTESIAN_POINT('Origin',(1.57762160836E-15,-19.3742356128,-3.80469754864));
#93281=CARTESIAN_POINT('Origin',(-0.153073372946,-19.4742356128,-4.17424936164));
#93282=CARTESIAN_POINT('Origin',(-1.01908995768E-15,-19.4742356128,-4.23765442876));
#93283=CARTESIAN_POINT('',(-3.35920145722,-19.3742356128,-2.84622762644));
#93284=CARTESIAN_POINT('',(-1.75613741508,-19.3742356128,-3.51023849404));
#93285=CARTESIAN_POINT('Origin',(-3.35920145722,-19.4742356128,-2.84622762644));
#93286=CARTESIAN_POINT('Origin',(3.14260590599E-16,-19.4742356128,5.26360209032));
#93287=CARTESIAN_POINT('',(-0.153073372946,-19.3742356128,5.63315390332));
#93288=CARTESIAN_POINT('Origin',(-0.153073372946,-19.4742356128,5.63315390332));
#93289=CARTESIAN_POINT('Origin',(1.87729180512E-16,-19.3742356128,5.26360209032));
#93290=CARTESIAN_POINT('Origin',(-1.62738508975E-15,-19.4742356128,5.69655897044));
#93291=CARTESIAN_POINT('',(-3.35920145722,-19.3742356128,4.30513216811));
#93292=CARTESIAN_POINT('Origin',(-3.35920145722,-19.4742356128,4.30513216811));
#93293=CARTESIAN_POINT('',(-1.75613741508,-19.3742356128,4.96914303572));
#93294=CARTESIAN_POINT('Origin',(-3.20612808427,-19.4742356128,3.93558035511));
#93295=CARTESIAN_POINT('',(-3.57567989727,-19.3742356128,4.08865372805));
#93296=CARTESIAN_POINT('Origin',(-3.57567989727,-19.4742356128,4.08865372805));
#93297=CARTESIAN_POINT('Origin',(-3.20612808427,-19.3742356128,3.93558035511));
#93298=CARTESIAN_POINT('Origin',(-4.11560885829,-19.4742356128,2.78514990766));
#93299=CARTESIAN_POINT('',(-4.90370163248,-19.3742356128,0.882525643785));
#93300=CARTESIAN_POINT('Origin',(-4.90370163248,-19.4742356128,0.882525643785));
#93301=CARTESIAN_POINT('',(-4.23969076488,-19.3742356128,2.48558968592));
#93302=CARTESIAN_POINT('Origin',(-4.53414981948,-19.4742356128,0.729452270839));
#93303=CARTESIAN_POINT('',(-4.90370163248,-19.3742356128,0.576378897893));
#93304=CARTESIAN_POINT('Origin',(-4.90370163248,-19.4742356128,0.576378897893));
#93305=CARTESIAN_POINT('Origin',(-4.53414981948,-19.3742356128,0.729452270839));
#93306=CARTESIAN_POINT('Origin',(-5.81860454091,-19.4742356128,2.78514990766));
#93307=CARTESIAN_POINT('',(-3.57567989727,-19.3742356128,-2.62974918638));
#93308=CARTESIAN_POINT('Origin',(-3.57567989727,-19.4742356128,-2.62974918638));
#93309=CARTESIAN_POINT('',(-4.23969076488,-19.3742356128,-1.02668514424));
#93310=CARTESIAN_POINT('Origin',(-3.20612808427,-19.4742356128,-2.47667581343));
#93311=CARTESIAN_POINT('Origin',(-3.20612808427,-19.3742356128,-2.47667581343));
#93312=CARTESIAN_POINT('Origin',(4.65365783676E-16,-19.3742356128,0.729452270839));
#93313=CARTESIAN_POINT('Origin',(-10.0415172382,-19.3742356128,8.33514586886));
#93314=CARTESIAN_POINT('',(-3.05,-19.3742356128,10.7304528845));
#93315=CARTESIAN_POINT('',(-3.05,-19.3742356128,2.96634320571));
#93316=CARTESIAN_POINT('',(-2.45,-19.3742356128,10.1304528845));
#93317=CARTESIAN_POINT('Origin',(-2.45,-19.3742356128,10.7304528845));
#93318=CARTESIAN_POINT('',(-6.6707290414,-19.3742356128,10.1304528845));
#93319=CARTESIAN_POINT('',(-10.3267865236,-19.3742356128,-3.3434289261));
#93320=CARTESIAN_POINT('Origin',(2.84607155346,-19.3742356128,5.53854202767));
#93321=CARTESIAN_POINT('Origin',(-11.0821857629,-19.3742356128,-2.71007990903));
#93322=CARTESIAN_POINT('Ctrl Pts',(1.13381424745833E-15,-19.3742356128,
-10.0919881826));
#93323=CARTESIAN_POINT('Ctrl Pts',(1.13381424745833E-15,-19.3742356128,
-10.0919881826));
#93324=CARTESIAN_POINT('Ctrl Pts',(1.13381424745833E-15,-19.3742356128,
-10.0919881826));
#93325=CARTESIAN_POINT('Ctrl Pts',(1.13381424745833E-15,-19.3742356128,
-10.0919881826));
#93326=CARTESIAN_POINT('Ctrl Pts',(1.13381424745833E-15,-19.3742356128,
-10.0919881826));
#93327=CARTESIAN_POINT('Ctrl Pts',(1.13381424745833E-15,-19.3742356128,
-10.0919881826));
#93328=CARTESIAN_POINT('Ctrl Pts',(-0.0415097842719,-19.3742356128,-10.1079379349));
#93329=CARTESIAN_POINT('Ctrl Pts',(-0.0249058705631,-19.3742356128,-10.1079379349));
#93330=CARTESIAN_POINT('Ctrl Pts',(-0.0083019552457,-19.3742356128,-10.1079379261));
#93331=CARTESIAN_POINT('Ctrl Pts',(0.0083019552457,-19.3742356128,-10.1079379261));
#93332=CARTESIAN_POINT('Ctrl Pts',(0.0249058705631,-19.3742356128,-10.1079379349));
#93333=CARTESIAN_POINT('Ctrl Pts',(0.0415097842719,-19.3742356128,-10.1079379349));
#93334=CARTESIAN_POINT('Ctrl Pts',(-0.0833222863185,-19.3764713196,-10.1232737584));
#93335=CARTESIAN_POINT('Ctrl Pts',(-0.0499933690234,-19.3759012652,-10.1232736299));
#93336=CARTESIAN_POINT('Ctrl Pts',(-0.0166644595934,-19.3756162324,-10.1232735872));
#93337=CARTESIAN_POINT('Ctrl Pts',(0.0166644595551,-19.3756162324,-10.1232735872));
#93338=CARTESIAN_POINT('Ctrl Pts',(0.0499933689979,-19.3759012652,-10.1232736299));
#93339=CARTESIAN_POINT('Ctrl Pts',(0.0833222863185,-19.3764713196,-10.1232737584));
#93340=CARTESIAN_POINT('Ctrl Pts',(-0.125363533497,-19.3807247797,-10.1376350659));
#93341=CARTESIAN_POINT('Ctrl Pts',(-0.0752314126451,-19.3789864318,-10.1378539929));
#93342=CARTESIAN_POINT('Ctrl Pts',(-0.025079356408,-19.378117295,-10.1379634778));
#93343=CARTESIAN_POINT('Ctrl Pts',(0.0250793561827,-19.378117295,-10.1379634778));
#93344=CARTESIAN_POINT('Ctrl Pts',(0.0752314124954,-19.3789864318,-10.1378539929));
#93345=CARTESIAN_POINT('Ctrl Pts',(0.125363533497,-19.3807247797,-10.1376350659));
#93346=CARTESIAN_POINT('Ctrl Pts',(-0.214270880278,-19.3937598094,-10.1664794265));
#93347=CARTESIAN_POINT('Ctrl Pts',(-0.128662254182,-19.3884633982,-10.1680588961));
#93348=CARTESIAN_POINT('Ctrl Pts',(-0.0429040381187,-19.3858130556,-10.1688486495));
#93349=CARTESIAN_POINT('Ctrl Pts',(0.0429040383692,-19.3858130556,-10.1688486495));
#93350=CARTESIAN_POINT('Ctrl Pts',(0.128662254349,-19.3884633982,-10.1680588961));
#93351=CARTESIAN_POINT('Ctrl Pts',(0.214270880278,-19.3937598094,-10.1664794265));
#93352=CARTESIAN_POINT('Ctrl Pts',(-0.302878944992,-19.4154221962,-10.1917028607));
#93353=CARTESIAN_POINT('Ctrl Pts',(-0.182097857803,-19.4049779364,-10.197316357));
#93354=CARTESIAN_POINT('Ctrl Pts',(-0.0607613296063,-19.3997406668,-10.2001306891));
#93355=CARTESIAN_POINT('Ctrl Pts',(0.0607613293279,-19.3997406668,-10.2001306891));
#93356=CARTESIAN_POINT('Ctrl Pts',(0.182097857618,-19.4049779364,-10.197316357));
#93357=CARTESIAN_POINT('Ctrl Pts',(0.302878944991,-19.4154221962,-10.1917028607));
#93358=CARTESIAN_POINT('Ctrl Pts',(-0.349011853831,-19.4292028661,-10.2039820431));
#93359=CARTESIAN_POINT('Ctrl Pts',(-0.209987919386,-19.4158427429,-10.2126719835));
#93360=CARTESIAN_POINT('Ctrl Pts',(-0.070093390793,-19.4091363298,-10.2170325701));
#93361=CARTESIAN_POINT('Ctrl Pts',(0.070093395411,-19.4091363298,-10.2170325701));
#93362=CARTESIAN_POINT('Ctrl Pts',(0.209987922457,-19.4158427429,-10.2126719835));
#93363=CARTESIAN_POINT('Ctrl Pts',(0.349011853831,-19.4292028661,-10.2039820431));
#93364=CARTESIAN_POINT('Ctrl Pts',(-0.414201204383,-19.4525352086,-10.2201075969));
#93365=CARTESIAN_POINT('Ctrl Pts',(-0.249526732723,-19.4351881568,-10.2348601694));
#93366=CARTESIAN_POINT('Ctrl Pts',(-0.0833448932135,-19.4264619682,-10.24227702));
#93367=CARTESIAN_POINT('Ctrl Pts',(0.0833448912668,-19.4264619682,-10.24227702));
#93368=CARTESIAN_POINT('Ctrl Pts',(0.249526731429,-19.4351881568,-10.2348601694));
#93369=CARTESIAN_POINT('Ctrl Pts',(0.414201204383,-19.4525352086,-10.2201075969));
#93370=CARTESIAN_POINT('Ctrl Pts',(-0.476889168989,-19.4827229707,-10.2341511354));
#93371=CARTESIAN_POINT('Ctrl Pts',(-0.287745576237,-19.4629708985,-10.2572820885));
#93372=CARTESIAN_POINT('Ctrl Pts',(-0.0961879175727,-19.453011347,-10.2689444929));
#93373=CARTESIAN_POINT('Ctrl Pts',(0.0961879183933,-19.453011347,-10.2689444929));
#93374=CARTESIAN_POINT('Ctrl Pts',(0.287745576783,-19.4629708985,-10.2572820885));
#93375=CARTESIAN_POINT('Ctrl Pts',(0.476889168989,-19.4827229707,-10.2341511354));
#93376=CARTESIAN_POINT('Ctrl Pts',(-0.495216410211,-19.492424266,-10.2381345523));
#93377=CARTESIAN_POINT('Ctrl Pts',(-0.298936557215,-19.4721609989,-10.2639381086));
#93378=CARTESIAN_POINT('Ctrl Pts',(-0.0999515182904,-19.4619368311,-10.2769563707));
#93379=CARTESIAN_POINT('Ctrl Pts',(0.09995152576,-19.4619368311,-10.2769563707));
#93380=CARTESIAN_POINT('Ctrl Pts',(0.298936562175,-19.4721609989,-10.2639381086));
#93381=CARTESIAN_POINT('Ctrl Pts',(0.495216410211,-19.492424266,-10.2381345523));
#93382=CARTESIAN_POINT('Ctrl Pts',(-0.548607288051,-19.5230709178,-10.2493705418));
#93383=CARTESIAN_POINT('Ctrl Pts',(-0.331601042239,-19.50197069,-10.2837483093));
#93384=CARTESIAN_POINT('Ctrl Pts',(-0.110947746796,-19.4913020672,-10.3011245839));
#93385=CARTESIAN_POINT('Ctrl Pts',(0.110947732078,-19.4913020672,-10.3011245839));
#93386=CARTESIAN_POINT('Ctrl Pts',(0.331601032464,-19.50197069,-10.2837483093));
#93387=CARTESIAN_POINT('Ctrl Pts',(0.548607288052,-19.5230709178,-10.2493705418));
#93388=CARTESIAN_POINT('Ctrl Pts',(-0.596976385661,-19.562200797,-10.2586626864));
#93389=CARTESIAN_POINT('Ctrl Pts',(-0.361343872845,-19.5433606575,-10.3026842693));
#93390=CARTESIAN_POINT('Ctrl Pts',(-0.120986572931,-19.5338129691,-10.3249810452));
#93391=CARTESIAN_POINT('Ctrl Pts',(0.120986601929,-19.5338129691,-10.3249810452));
#93392=CARTESIAN_POINT('Ctrl Pts',(0.36134389211,-19.5433606575,-10.3026842693));
#93393=CARTESIAN_POINT('Ctrl Pts',(0.596976385661,-19.562200797,-10.2586626864));
#93394=CARTESIAN_POINT('Ctrl Pts',(-0.628284771894,-19.5926160239,-10.2642394886));
#93395=CARTESIAN_POINT('Ctrl Pts',(-0.380691753868,-19.576871863,-10.3156638409));
#93396=CARTESIAN_POINT('Ctrl Pts',(-0.127533759232,-19.5688752663,-10.3417537086));
#93397=CARTESIAN_POINT('Ctrl Pts',(0.127533760988,-19.5688752663,-10.3417537086));
#93398=CARTESIAN_POINT('Ctrl Pts',(0.380691755013,-19.576871863,-10.3156638409));
#93399=CARTESIAN_POINT('Ctrl Pts',(0.628284771894,-19.5926160239,-10.2642394886));
#93400=CARTESIAN_POINT('Ctrl Pts',(-0.647446102181,-19.633156143,-10.2675153591));
#93401=CARTESIAN_POINT('Ctrl Pts',(-0.392565377877,-19.6252559631,-10.3238501103));
#93402=CARTESIAN_POINT('Ctrl Pts',(-0.131557494297,-19.6212431604,-10.3524631664));
#93403=CARTESIAN_POINT('Ctrl Pts',(0.131557494286,-19.6212431604,-10.3524631664));
#93404=CARTESIAN_POINT('Ctrl Pts',(0.392565377877,-19.6252559631,-10.3238501103));
#93405=CARTESIAN_POINT('Ctrl Pts',(0.647446102181,-19.633156143,-10.2675153591));
#93406=CARTESIAN_POINT('Ctrl Pts',(-0.647446102181,-19.6742356128,-10.2675153591));
#93407=CARTESIAN_POINT('Ctrl Pts',(-0.392565377877,-19.6742356128,-10.3238501103));
#93408=CARTESIAN_POINT('Ctrl Pts',(-0.131557494527,-19.6742356128,-10.3524631675));
#93409=CARTESIAN_POINT('Ctrl Pts',(0.131557494527,-19.6742356128,-10.3524631675));
#93410=CARTESIAN_POINT('Ctrl Pts',(0.392565377877,-19.6742356128,-10.3238501103));
#93411=CARTESIAN_POINT('Ctrl Pts',(0.647446102181,-19.6742356128,-10.2675153591));
#93412=CARTESIAN_POINT('Ctrl Pts',(-0.647446102181,-19.6742356128,-10.2675153591));
#93413=CARTESIAN_POINT('Ctrl Pts',(-0.647445941636813,-19.6661001011575,
-10.2675153945841));
#93414=CARTESIAN_POINT('Ctrl Pts',(-0.646542770743725,-19.6579947206812,
-10.2673610476357));
#93415=CARTESIAN_POINT('Ctrl Pts',(-0.6448617348847,-19.6500513204232,-10.2670699532246));
#93416=CARTESIAN_POINT('Ctrl Pts',(-0.643110060949621,-19.6417741340008,
-10.266766626862));
#93417=CARTESIAN_POINT('Ctrl Pts',(-0.640514331113089,-19.633672486467,
-10.266314905712));
#93418=CARTESIAN_POINT('Ctrl Pts',(-0.637226684371121,-19.6258364904321,
-10.2657366368423));
#93419=CARTESIAN_POINT('Ctrl Pts',(-0.633683129499015,-19.6173905459294,
-10.265113355927));
#93420=CARTESIAN_POINT('Ctrl Pts',(-0.629336605338115,-19.6092529554109,
-10.2643431920501));
#93421=CARTESIAN_POINT('Ctrl Pts',(-0.624378482864707,-19.6014736015796,
-10.2634539338467));
#93422=CARTESIAN_POINT('Ctrl Pts',(-0.620736150240958,-19.5957587378579,
-10.2628006675785));
#93423=CARTESIAN_POINT('Ctrl Pts',(-0.616763848379759,-19.5902357668082,
-10.2620831507));
#93424=CARTESIAN_POINT('Ctrl Pts',(-0.612533267931434,-19.5849072924126,
-10.2613118426351));
#93425=CARTESIAN_POINT('Ctrl Pts',(-0.606480198733363,-19.5772833683127,
-10.2602082633161));
#93426=CARTESIAN_POINT('Ctrl Pts',(-0.59990047287895,-19.5700585023242,
-10.2589948789287));
#93427=CARTESIAN_POINT('Ctrl Pts',(-0.592977788625539,-19.5632046643295,
-10.2576984743346));
#93428=CARTESIAN_POINT('Ctrl Pts',(-0.586303368636261,-19.556596621605,
-10.2564485619567));
#93429=CARTESIAN_POINT('Ctrl Pts',(-0.579310981101092,-19.550332062835,
-10.2551216113969));
#93430=CARTESIAN_POINT('Ctrl Pts',(-0.572123283687863,-19.544366280316,
-10.2537352999208));
#93431=CARTESIAN_POINT('Ctrl Pts',(-0.565452398298276,-19.5388294513213,
-10.2524486674376));
#93432=CARTESIAN_POINT('Ctrl Pts',(-0.558613515362534,-19.5335490260034,
-10.2511109441));
#93433=CARTESIAN_POINT('Ctrl Pts',(-0.551661093300188,-19.5284883850772,
-10.2497295965832));
#93434=CARTESIAN_POINT('Ctrl Pts',(-0.547611964544735,-19.5255410400353,
-10.2489250922103));
#93435=CARTESIAN_POINT('Ctrl Pts',(-0.543523480221757,-19.5226682993563,
-10.2481056613876));
#93436=CARTESIAN_POINT('Ctrl Pts',(-0.539398338224439,-19.5198645633611,
-10.247271538349));
#93437=CARTESIAN_POINT('Ctrl Pts',(-0.536480092791513,-19.5178811189686,
-10.2466814554502));
#93438=CARTESIAN_POINT('Ctrl Pts',(-0.533543376246939,-19.5159322357429,
-10.246084000407));
#93439=CARTESIAN_POINT('Ctrl Pts',(-0.530587106428603,-19.5140165822185,
-10.2454789413881));
#93440=CARTESIAN_POINT('Ctrl Pts',(-0.522248905685559,-19.5086134544183,
-10.2437723638863));
#93441=CARTESIAN_POINT('Ctrl Pts',(-0.513755279272081,-19.503470639622,
-10.2420051344035));
#93442=CARTESIAN_POINT('Ctrl Pts',(-0.505148889126634,-19.4985340614123,
-10.2401816464316));
#93443=CARTESIAN_POINT('Ctrl Pts',(-0.493851874114429,-19.4920541555282,
-10.2377880794837));
#93444=CARTESIAN_POINT('Ctrl Pts',(-0.482361393685303,-19.4859314445867,
-10.235297811603));
#93445=CARTESIAN_POINT('Ctrl Pts',(-0.470738754303351,-19.4801299566937,
-10.2327185873485));
#93446=CARTESIAN_POINT('Ctrl Pts',(-0.460415430607163,-19.4749770275293,
-10.2304276991958));
#93447=CARTESIAN_POINT('Ctrl Pts',(-0.44998689248508,-19.4700825616961,
-10.2280666991948));
#93448=CARTESIAN_POINT('Ctrl Pts',(-0.439477083766254,-19.4654176369213,
-10.2256374783638));
#93449=CARTESIAN_POINT('Ctrl Pts',(-0.422732203090843,-19.4579851887387,
-10.2217670927042));
#93450=CARTESIAN_POINT('Ctrl Pts',(-0.405782552671417,-19.4511239727718,
-10.2177231721969));
#93451=CARTESIAN_POINT('Ctrl Pts',(-0.388710157357095,-19.4447597442073,
-10.2135127613696));
#93452=CARTESIAN_POINT('Ctrl Pts',(-0.381260998107146,-19.4419828548953,
-10.2116756424309));
#93453=CARTESIAN_POINT('Ctrl Pts',(-0.373787812289178,-19.4393009012942,
-10.2098067387429));
#93454=CARTESIAN_POINT('Ctrl Pts',(-0.366294824663843,-19.436709133715,
-10.2079062805535));
#93455=CARTESIAN_POINT('Ctrl Pts',(-0.345601093381887,-19.4295513290432,
-10.2026576970711));
#93456=CARTESIAN_POINT('Ctrl Pts',(-0.324759283924013,-19.4230782905106,
-10.197168887497));
#93457=CARTESIAN_POINT('Ctrl Pts',(-0.303821610594384,-19.4172207371684,
-10.1914391367788));
#93458=CARTESIAN_POINT('Ctrl Pts',(-0.282246141989557,-19.4111847533106,
-10.185534848619));
#93459=CARTESIAN_POINT('Ctrl Pts',(-0.260564896862457,-19.4058026301278,
-10.1793742687788));
#93460=CARTESIAN_POINT('Ctrl Pts',(-0.238824865074793,-19.4010423842632,
-10.1729531784551));
#93461=CARTESIAN_POINT('Ctrl Pts',(-0.229060950242532,-19.3989044556871,
-10.1700693289897));
#93462=CARTESIAN_POINT('Ctrl Pts',(-0.219285416886937,-19.3968925139675,
-10.1671329286478));
#93463=CARTESIAN_POINT('Ctrl Pts',(-0.209505275647252,-19.3950061365628,
-10.1641437615851));
#93464=CARTESIAN_POINT('Ctrl Pts',(-0.186799713516908,-19.3906267254363,
-10.1572041155416));
#93465=CARTESIAN_POINT('Ctrl Pts',(-0.164070264338569,-19.3869226098162,
-10.1499848160957));
#93466=CARTESIAN_POINT('Ctrl Pts',(-0.141363992467237,-19.383901171999,
-10.1424921906684));
#93467=CARTESIAN_POINT('Ctrl Pts',(-0.1176844998854,-19.3807502313785,-10.1346784214494));
#93468=CARTESIAN_POINT('Ctrl Pts',(-0.0940309082477135,-19.3783415049,-10.126561853247));
#93469=CARTESIAN_POINT('Ctrl Pts',(-0.0704547890620564,-19.376712860041,
-10.118136804536));
#93470=CARTESIAN_POINT('Ctrl Pts',(-0.0515376158941429,-19.3754060564664,
-10.111376654396));
#93471=CARTESIAN_POINT('Ctrl Pts',(-0.0326704350502771,-19.3746020563644,
-10.1044164174881));
#93472=CARTESIAN_POINT('Ctrl Pts',(-0.0138743237156372,-19.3743346947001,
-10.0972858826397));
#93473=CARTESIAN_POINT('Ctrl Pts',(-0.00924519296368537,-19.3742688485216,
-10.0955297652409));
#93474=CARTESIAN_POINT('Ctrl Pts',(-0.00462033833946646,-19.3742356128,
-10.09376354789));
#93475=CARTESIAN_POINT('Ctrl Pts',(-1.46021229138484E-14,-19.3742356128,
-10.0919881826));
#93476=CARTESIAN_POINT('Origin',(2.84607155346,-19.6742356128,5.53854202767));
#93477=CARTESIAN_POINT('Ctrl Pts',(-10.3267865236,-19.3742356128,-3.3434289261));
#93478=CARTESIAN_POINT('Ctrl Pts',(-10.3387312196063,-19.3742356127965,
-3.3514827927929));
#93479=CARTESIAN_POINT('Ctrl Pts',(-10.3502659022817,-19.3752737080098,
-3.35929500283175));
#93480=CARTESIAN_POINT('Ctrl Pts',(-10.3612964278539,-19.3771435879029,
-3.366782731296));
#93481=CARTESIAN_POINT('Ctrl Pts',(-10.3726225546623,-19.3790635777208,
-3.37447111944563));
#93482=CARTESIAN_POINT('Ctrl Pts',(-10.3834174120365,-19.3818597256152,
-3.38181758261816));
#93483=CARTESIAN_POINT('Ctrl Pts',(-10.3936260273276,-19.3853112756837,
-3.38876386993635));
#93484=CARTESIAN_POINT('Ctrl Pts',(-10.404292680099,-19.3889176889978,-3.39602182145676));
#93485=CARTESIAN_POINT('Ctrl Pts',(-10.4143196241775,-19.393238865228,-3.40284309446403));
#93486=CARTESIAN_POINT('Ctrl Pts',(-10.4236902973134,-19.3980382520255,
-3.40919213448965));
#93487=CARTESIAN_POINT('Ctrl Pts',(-10.4288958013969,-19.4007043601279,
-3.4127190906966));
#93488=CARTESIAN_POINT('Ctrl Pts',(-10.4338995668108,-19.4035183843968,
-3.41610084279332));
#93489=CARTESIAN_POINT('Ctrl Pts',(-10.4387038417048,-19.4064428549585,
-3.41933470452082));
#93490=CARTESIAN_POINT('Ctrl Pts',(-10.4479416835707,-19.4120661378027,
-3.42555289642579));
#93491=CARTESIAN_POINT('Ctrl Pts',(-10.4564343914218,-19.4180968666509,
-3.43123772413905));
#93492=CARTESIAN_POINT('Ctrl Pts',(-10.4642110658934,-19.4243032304506,
-3.43642557350015));
#93493=CARTESIAN_POINT('Ctrl Pts',(-10.468973720738,-19.4281041827376,-3.43960275881023));
#93494=CARTESIAN_POINT('Ctrl Pts',(-10.4734684907843,-19.4319718023247,
-3.44259400325187));
#93495=CARTESIAN_POINT('Ctrl Pts',(-10.477706871939,-19.4358603802918,-3.44541093680795));
#93496=CARTESIAN_POINT('Ctrl Pts',(-10.4832863710631,-19.4409793907275,
-3.44911921073018));
#93497=CARTESIAN_POINT('Ctrl Pts',(-10.4884211141688,-19.4461343216654,
-3.45252637078225));
#93498=CARTESIAN_POINT('Ctrl Pts',(-10.4931417652086,-19.4512367616961,
-3.45566728613861));
#93499=CARTESIAN_POINT('Ctrl Pts',(-10.4955020907286,-19.4537879817114,
-3.45723774381679));
#93500=CARTESIAN_POINT('Ctrl Pts',(-10.497758968688,-19.4563263498715,-3.45874172903051));
#93501=CARTESIAN_POINT('Ctrl Pts',(-10.4999165611424,-19.4588423794387,
-3.460183992036));
#93502=CARTESIAN_POINT('Ctrl Pts',(-10.5010151617041,-19.4601234886168,
-3.46091836193272));
#93503=CARTESIAN_POINT('Ctrl Pts',(-10.5018334456779,-19.4610958633222,
-3.46146508757472));
#93504=CARTESIAN_POINT('Ctrl Pts',(-10.5027639399852,-19.4622174177238,
-3.46208908760247));
#93505=CARTESIAN_POINT('Ctrl Pts',(-10.5036608864843,-19.4632985358844,
-3.46269059008983));
#93506=CARTESIAN_POINT('Ctrl Pts',(-10.5046628965481,-19.4645174989002,
-3.4633644336224));
#93507=CARTESIAN_POINT('Ctrl Pts',(-10.5060957679725,-19.4663149543736,
-3.46433051713108));
#93508=CARTESIAN_POINT('Ctrl Pts',(-10.5163491930108,-19.4791772912472,
-3.47124367393553));
#93509=CARTESIAN_POINT('Ctrl Pts',(-10.5254908828199,-19.4929441876984,
-3.47740738103718));
#93510=CARTESIAN_POINT('Ctrl Pts',(-10.5334831428677,-19.5073425987759,
-3.48279617293412));
#93511=CARTESIAN_POINT('Ctrl Pts',(-10.5419680711657,-19.5226285735648,
-3.48851714704963));
#93512=CARTESIAN_POINT('Ctrl Pts',(-10.549157878795,-19.5386258135561,-3.49336498501857));
#93513=CARTESIAN_POINT('Ctrl Pts',(-10.5550496559692,-19.5550381187943,
-3.49733766485271));
#93514=CARTESIAN_POINT('Ctrl Pts',(-10.5611683702378,-19.5720825865791,
-3.5014633627647));
#93515=CARTESIAN_POINT('Ctrl Pts',(-10.5658877319341,-19.5895745010765,
-3.50464558914306));
#93516=CARTESIAN_POINT('Ctrl Pts',(-10.5692405803808,-19.607219645542,-3.506906418514));
#93517=CARTESIAN_POINT('Ctrl Pts',(-10.572797265971,-19.6259375303653,-3.50930469549345));
#93518=CARTESIAN_POINT('Ctrl Pts',(-10.5748167551615,-19.6448277038803,
-3.51066648913781));
#93519=CARTESIAN_POINT('Ctrl Pts',(-10.5753692578738,-19.663583483134,-3.51103905824762));
#93520=CARTESIAN_POINT('Ctrl Pts',(-10.5754740112682,-19.6671395408632,
-3.51110969659566));
#93521=CARTESIAN_POINT('Ctrl Pts',(-10.5755261020433,-19.6706908911756,
-3.51114482325917));
#93522=CARTESIAN_POINT('Ctrl Pts',(-10.5755261020433,-19.6742356128,-3.51114482325917));
#93523=CARTESIAN_POINT('Origin',(-11.0821857629,-19.6742356128,-2.71007990903));
#93524=CARTESIAN_POINT('',(-10.5566756949,-19.6742356128,-3.15068305993));
#93525=CARTESIAN_POINT('Origin',(-10.3267865236,-19.6742356128,-3.3434289261));
#93526=CARTESIAN_POINT('',(-11.2159436339,-19.6742356128,-2.03747244546));
#93527=CARTESIAN_POINT('Origin',(-11.0821857629,-19.6742356128,-2.71007990903));
#93528=CARTESIAN_POINT('Origin',(-11.2744572342983,-19.6742356128,-1.74323417709617));
#93529=CARTESIAN_POINT('Origin',(-12.5441720511,-22.5760378048,9.34841724773));
#93530=CARTESIAN_POINT('',(-12.8222448081,-25.4742356128,9.46100295649));
#93531=CARTESIAN_POINT('Origin',(-12.5441720511,-25.4742356128,9.34841724773));
#93532=CARTESIAN_POINT('',(-12.8222448231109,-23.4742356815,9.46100293550673));
#93533=CARTESIAN_POINT('',(-12.8222448081,-21.2742356128,9.46100295649));
#93534=CARTESIAN_POINT('Origin',(-12.5441720511,-23.47423564715,9.34841724773));
#93535=CARTESIAN_POINT('Origin',(-12.5441720511,-25.4742356128,9.34841724773));
#93536=CARTESIAN_POINT('Origin',(-12.5441720511,-25.4742356128,9.34841724773));
#93537=CARTESIAN_POINT('Origin',(-10.0415172382,-25.4742356128,8.33514586886));
#93538=CARTESIAN_POINT('Origin',(-10.0415172382,-25.4742356128,8.33514586886));
#93539=CARTESIAN_POINT('Origin',(-10.0415172382,-19.6742356128,8.33514586886));
#93540=CARTESIAN_POINT('Origin',(-10.0415172382,-19.6742356128,8.33514586886));
#93541=CARTESIAN_POINT('Origin',(-10.0415172382,-21.2742356128,8.33514586886));
#93542=CARTESIAN_POINT('Ctrl Pts',(-12.822244843051,-23.4742356815,9.46100291845212));
#93543=CARTESIAN_POINT('Ctrl Pts',(-12.8222448374688,-23.4526557884998,
9.46100292804296));
#93544=CARTESIAN_POINT('Ctrl Pts',(-12.8227658011016,-23.4310761714824,
9.459718249267));
#93545=CARTESIAN_POINT('Ctrl Pts',(-12.8237956782946,-23.4096767931088,
9.45716500907838));
#93546=CARTESIAN_POINT('Ctrl Pts',(-12.8249218353694,-23.3862768561876,
9.45437307473734));
#93547=CARTESIAN_POINT('Ctrl Pts',(-12.8266564446377,-23.3630965146334,
9.45006425351064));
#93548=CARTESIAN_POINT('Ctrl Pts',(-12.8289489787169,-23.3403539792507,
9.4443040829754));
#93549=CARTESIAN_POINT('Ctrl Pts',(-12.8312709606729,-23.3173193132581,
9.43846992235491));
#93550=CARTESIAN_POINT('Ctrl Pts',(-12.8341646949754,-23.2947342337854,
9.43114748157285));
#93551=CARTESIAN_POINT('Ctrl Pts',(-12.8375494613154,-23.2727938554516,
9.42244323588751));
#93552=CARTESIAN_POINT('Ctrl Pts',(-12.8410023873676,-23.250411659361,9.41356371107774));
#93553=CARTESIAN_POINT('Ctrl Pts',(-12.8449656668396,-23.2287009550523,
9.40324680779877));
#93554=CARTESIAN_POINT('Ctrl Pts',(-12.8493339497345,-23.2078282931751,
9.39163588847771));
#93555=CARTESIAN_POINT('Ctrl Pts',(-12.8533668576591,-23.1885581301571,
9.38091639762304));
#93556=CARTESIAN_POINT('Ctrl Pts',(-12.8577443119826,-23.1700021065795,
9.36909474059184));
#93557=CARTESIAN_POINT('Ctrl Pts',(-12.8623765483007,-23.1522553698924,
9.35629852758267));
#93558=CARTESIAN_POINT('Ctrl Pts',(-12.8676258737502,-23.1321444795705,
9.34179765111725));
#93559=CARTESIAN_POINT('Ctrl Pts',(-12.8732011777363,-23.1130741318264,
9.3260463447321));
#93560=CARTESIAN_POINT('Ctrl Pts',(-12.8789692176796,-23.0951288263937,
9.30924271806145));
#93561=CARTESIAN_POINT('Ctrl Pts',(-12.8847323055415,-23.0771989276877,
9.29245351794285));
#93562=CARTESIAN_POINT('Ctrl Pts',(-12.8906877245128,-23.0603914552665,
9.27461404125843));
#93563=CARTESIAN_POINT('Ctrl Pts',(-12.8967175034202,-23.0447417766193,
9.25591265355548));
#93564=CARTESIAN_POINT('Ctrl Pts',(-12.9032960762988,-23.0276677589662,
9.23550917876373));
#93565=CARTESIAN_POINT('Ctrl Pts',(-12.909961941791,-23.0119710592708,9.21408281923307));
#93566=CARTESIAN_POINT('Ctrl Pts',(-12.9165837263722,-22.997646095339,9.1918614547601));
#93567=CARTESIAN_POINT('Ctrl Pts',(-12.9229613039847,-22.9838494264575,
9.17045959928658));
#93568=CARTESIAN_POINT('Ctrl Pts',(-12.9292980187867,-22.9713240464602,
9.14832050002835));
#93569=CARTESIAN_POINT('Ctrl Pts',(-12.9354980002173,-22.9600302011921,
9.12562740036042));
#93570=CARTESIAN_POINT('Ctrl Pts',(-12.9422358704374,-22.9477565412539,
9.10096552642308));
#93571=CARTESIAN_POINT('Ctrl Pts',(-12.9488130289529,-22.9369364542937,
9.07564536621217));
#93572=CARTESIAN_POINT('Ctrl Pts',(-12.9551362385969,-22.9274915788356,
9.04986970620133));
#93573=CARTESIAN_POINT('Ctrl Pts',(-12.9614594482409,-22.9180467033774,
9.02409404619048));
#93574=CARTESIAN_POINT('Ctrl Pts',(-12.9675285501681,-22.9099757205391,
8.99786337398523));
#93575=CARTESIAN_POINT('Ctrl Pts',(-12.9732844031999,-22.9031898545,8.97133867789998));
#93576=CARTESIAN_POINT('Ctrl Pts',(-10.5755260924,-22.0742355256,-3.51114484425));
#93577=CARTESIAN_POINT('Ctrl Pts',(-10.6188297183,-22.0742355492,-3.44692120094));
#93578=CARTESIAN_POINT('Ctrl Pts',(-10.6414054613,-22.0742355727,-3.36872151284));
#93579=CARTESIAN_POINT('Ctrl Pts',(-10.6370511822,-22.0742355929,-3.28545797344));
#93580=CARTESIAN_POINT('Ctrl Pts',(-10.6064419603,-22.0742356067,-3.21003960317));
#93581=CARTESIAN_POINT('Ctrl Pts',(-10.5566756907,-22.0742356132,-3.15068306769));
#93582=CARTESIAN_POINT('Ctrl Pts',(-10.5755260601,-22.166010044,-3.51114490853));
#93583=CARTESIAN_POINT('Ctrl Pts',(-10.6188296919,-22.1536827124,-3.44692125214));
#93584=CARTESIAN_POINT('Ctrl Pts',(-10.6414054404,-22.1413553808,-3.36872155059));
#93585=CARTESIAN_POINT('Ctrl Pts',(-10.6370511655,-22.1307558548,-3.28545799936));
#93586=CARTESIAN_POINT('Ctrl Pts',(-10.6064419458,-22.1235274771,-3.21003962102));
#93587=CARTESIAN_POINT('Ctrl Pts',(-10.5566756767,-22.1201229434,-3.15068308186));
#93588=CARTESIAN_POINT('Ctrl Pts',(-10.5859201877,-22.2577874429,-3.49572587157));
#93589=CARTESIAN_POINT('Ctrl Pts',(-10.6278514281,-22.233131778,-3.43337939424));
#93590=CARTESIAN_POINT('Ctrl Pts',(-10.6489702842,-22.208476113,-3.35703447733));
#93591=CARTESIAN_POINT('Ctrl Pts',(-10.6432450252,-22.1872763848,-3.27537017178));
#93592=CARTESIAN_POINT('Ctrl Pts',(-10.6115652008,-22.1728195852,-3.20109406558));
#93593=CARTESIAN_POINT('Ctrl Pts',(-10.5611420569,-22.1660113751,-3.14236541304));
#93594=CARTESIAN_POINT('Ctrl Pts',(-10.6066865316,-22.3446142249,-3.46495847428));
#93595=CARTESIAN_POINT('Ctrl Pts',(-10.6458822742,-22.3082051755,-3.40634319147));
#93596=CARTESIAN_POINT('Ctrl Pts',(-10.6640744247,-22.271796126,-3.33367204908));
#93597=CARTESIAN_POINT('Ctrl Pts',(-10.6555763229,-22.2405343767,-3.25514874825));
#93598=CARTESIAN_POINT('Ctrl Pts',(-10.6217403852,-22.2193079256,-3.18308999607));
#93599=CARTESIAN_POINT('Ctrl Pts',(-10.5700204128,-22.2094250148,-3.125562098));
#93600=CARTESIAN_POINT('Ctrl Pts',(-10.674845259,-22.520870984,-3.36284445229));
#93601=CARTESIAN_POINT('Ctrl Pts',(-10.7051567944,-22.4603981097,-3.31661379633));
#93602=CARTESIAN_POINT('Ctrl Pts',(-10.7138373508,-22.3999252353,-3.25613169144));
#93603=CARTESIAN_POINT('Ctrl Pts',(-10.6962772721,-22.3481414788,-3.18810636174));
#93604=CARTESIAN_POINT('Ctrl Pts',(-10.6552160972,-22.313296938,-3.12357064819));
#93605=CARTESIAN_POINT('Ctrl Pts',(-10.5989042983,-22.2975531745,-3.07021211854));
#93606=CARTESIAN_POINT('Ctrl Pts',(-10.7768953898,-22.6311647495,-3.20613583022));
#93607=CARTESIAN_POINT('Ctrl Pts',(-10.7945590475,-22.5536945709,-3.178366012));
#93608=CARTESIAN_POINT('Ctrl Pts',(-10.7886824067,-22.4762243923,-3.13547322182));
#93609=CARTESIAN_POINT('Ctrl Pts',(-10.7562408317,-22.4108351721,-3.08179482002));
#93610=CARTESIAN_POINT('Ctrl Pts',(-10.7028434694,-22.368886031,-3.02683000685));
#93611=CARTESIAN_POINT('Ctrl Pts',(-10.6386344625,-22.3527003413,-2.97820952919));
#93612=CARTESIAN_POINT('Ctrl Pts',(-10.8408451958,-22.6662436275,-3.10591749488));
#93613=CARTESIAN_POINT('Ctrl Pts',(-10.8508648422,-22.5823049863,-3.08975078999));
#93614=CARTESIAN_POINT('Ctrl Pts',(-10.835946736,-22.4983663451,-3.05779148046));
#93615=CARTESIAN_POINT('Ctrl Pts',(-10.7939944577,-22.4282060593,-3.01294781655));
#93616=CARTESIAN_POINT('Ctrl Pts',(-10.7324020912,-22.3847322352,-2.96381562098));
#93617=CARTESIAN_POINT('Ctrl Pts',(-10.6626475871,-22.3702395434,-2.91797567427));
#93618=CARTESIAN_POINT('Ctrl Pts',(-10.9022658531,-22.6742356128,-3.00720831272));
#93619=CARTESIAN_POINT('Ctrl Pts',(-10.9055923018,-22.5849236589,-3.00178035997));
#93620=CARTESIAN_POINT('Ctrl Pts',(-10.8807899278,-22.495611705,-2.97883906106));
#93621=CARTESIAN_POINT('Ctrl Pts',(-10.8268747327,-22.422876423,-2.93934282537));
#93622=CARTESIAN_POINT('Ctrl Pts',(-10.7549391582,-22.3819887897,-2.89162579979));
#93623=CARTESIAN_POINT('Ctrl Pts',(-10.6791013717,-22.3742356128,-2.84444941082));
#93624=CARTESIAN_POINT('Ctrl Pts',(-10.9558455155,-22.6742356128,-2.9197793747));
#93625=CARTESIAN_POINT('Ctrl Pts',(-10.9558455155,-22.5799878332,-2.9197793747));
#93626=CARTESIAN_POINT('Ctrl Pts',(-10.9242889413,-22.4857400536,-2.90044034768));
#93627=CARTESIAN_POINT('Ctrl Pts',(-10.8607738721,-22.4112466293,-2.86151598188));
#93628=CARTESIAN_POINT('Ctrl Pts',(-10.7804157158,-22.3742356128,-2.81226955396));
#93629=CARTESIAN_POINT('Ctrl Pts',(-10.7000575594,-22.3742356128,-2.76302312605));
#93630=CARTESIAN_POINT('',(-10.5566756928877,-22.0742356130312,-3.15068306070111));
#93631=CARTESIAN_POINT('Origin',(-10.3289416669918,-22.0742354221932,-3.34331619631364));
#93632=CARTESIAN_POINT('Origin',(-10.7018663106063,-22.6721142716748,-2.76413150657896));
#93633=CARTESIAN_POINT('Ctrl Pts',(-10.5566756907,-22.0742356132,-3.15068306769));
#93634=CARTESIAN_POINT('Ctrl Pts',(-10.5566756859512,-22.0898005735048,
-3.15068307249646));
#93635=CARTESIAN_POINT('Ctrl Pts',(-10.5573215621371,-22.1049828544198,
-3.14956730460941));
#93636=CARTESIAN_POINT('Ctrl Pts',(-10.5584978473689,-22.1196224072354,
-3.14747917537089));
#93637=CARTESIAN_POINT('Ctrl Pts',(-10.5597026713832,-22.1346171417708,
-3.14534038438448));
#93638=CARTESIAN_POINT('Ctrl Pts',(-10.5614636623284,-22.1490426809088,
-3.14218291907421));
#93639=CARTESIAN_POINT('Ctrl Pts',(-10.5636517974364,-22.1627817175157,
-3.13816526443253));
#93640=CARTESIAN_POINT('Ctrl Pts',(-10.5658925822785,-22.1768513354569,
-3.13405093913847));
#93641=CARTESIAN_POINT('Ctrl Pts',(-10.5685810564944,-22.1902013580508,
-3.12903543901091));
#93642=CARTESIAN_POINT('Ctrl Pts',(-10.5715778051455,-22.2027583291733,
-3.12327540451024));
#93643=CARTESIAN_POINT('Ctrl Pts',(-10.5722285509149,-22.2054850829943,
-3.12202460955891));
#93644=CARTESIAN_POINT('Ctrl Pts',(-10.5728938380069,-22.2081746216534,
-3.12073863082624));
#93645=CARTESIAN_POINT('Ctrl Pts',(-10.5735722505496,-22.2108264835374,
-3.11941893786222));
#93646=CARTESIAN_POINT('Ctrl Pts',(-10.5767098864281,-22.2230912582412,
-3.11331540095486));
#93647=CARTESIAN_POINT('Ctrl Pts',(-10.5801400974471,-22.2345491177178,
-3.10650592289017));
#93648=CARTESIAN_POINT('Ctrl Pts',(-10.5837599834052,-22.2451819019482,
-3.09916288252606));
#93649=CARTESIAN_POINT('Ctrl Pts',(-10.5858115691318,-22.2512080775278,
-3.09500118324169));
#93650=CARTESIAN_POINT('Ctrl Pts',(-10.5879242114495,-22.2569701262268,
-3.09066763613829));
#93651=CARTESIAN_POINT('Ctrl Pts',(-10.5900806129031,-22.2624708648471,
-3.0861898087817));
#93652=CARTESIAN_POINT('Ctrl Pts',(-10.5925134060449,-22.2686766477117,
-3.08113804642784));
#93653=CARTESIAN_POINT('Ctrl Pts',(-10.5950025653009,-22.2745494339731,
-3.0759040953588));
#93654=CARTESIAN_POINT('Ctrl Pts',(-10.5975255802534,-22.2800979399819,
-3.07052547791864));
#93655=CARTESIAN_POINT('Ctrl Pts',(-10.5980937173012,-22.2813473625509,
-3.06931431116335));
#93656=CARTESIAN_POINT('Ctrl Pts',(-10.598663581943,-22.2825803644228,-3.06809579402851));
#93657=CARTESIAN_POINT('Ctrl Pts',(-10.5992350299983,-22.2837970686739,
-3.06687046288606));
#93658=CARTESIAN_POINT('Ctrl Pts',(-10.6007896133565,-22.2871070251309,
-3.06353703759118));
#93659=CARTESIAN_POINT('Ctrl Pts',(-10.6023553288436,-22.2902961983313,
-3.06015269099193));
#93660=CARTESIAN_POINT('Ctrl Pts',(-10.6039279613649,-22.2933677297212,
-3.05672524457382));
#93661=CARTESIAN_POINT('Ctrl Pts',(-10.6047142776256,-22.2949034954161,
-3.05501152136476));
#93662=CARTESIAN_POINT('Ctrl Pts',(-10.6055023240052,-22.2964098493286,
-3.05328702260517));
#93663=CARTESIAN_POINT('Ctrl Pts',(-10.6062915890173,-22.2978872035116,
-3.05155269432272));
#93664=CARTESIAN_POINT('Ctrl Pts',(-10.6067749132123,-22.2987918945979,
-3.05049063936261));
#93665=CARTESIAN_POINT('Ctrl Pts',(-10.6071177353671,-22.2994259157237,
-3.04973510754653));
#93666=CARTESIAN_POINT('Ctrl Pts',(-10.6075784274124,-22.300268624085,-3.04871832870286));
#93667=CARTESIAN_POINT('Ctrl Pts',(-10.6078700422379,-22.3008020525526,
-3.04807471484389));
#93668=CARTESIAN_POINT('Ctrl Pts',(-10.6082089738345,-22.3014187874837,
-3.04732610967217));
#93669=CARTESIAN_POINT('Ctrl Pts',(-10.6086625394533,-22.3022326923837,
-3.04632115024142));
#93670=CARTESIAN_POINT('Ctrl Pts',(-10.6133661861168,-22.3106731934043,
-3.03589934162453));
#93671=CARTESIAN_POINT('Ctrl Pts',(-10.618088525891,-22.318158006891,-3.02504352114557));
#93672=CARTESIAN_POINT('Ctrl Pts',(-10.6227349108549,-22.3247632918189,
-3.01388705341523));
#93673=CARTESIAN_POINT('Ctrl Pts',(-10.6275370085389,-22.3315899374155,
-3.00235670277379));
#93674=CARTESIAN_POINT('Ctrl Pts',(-10.6322563565154,-22.3374778766665,
-2.99050341653969));
#93675=CARTESIAN_POINT('Ctrl Pts',(-10.6368193302651,-22.3425438840508,
-2.9784373250117));
#93676=CARTESIAN_POINT('Ctrl Pts',(-10.6415727814018,-22.3478213675254,
-2.96586754494355));
#93677=CARTESIAN_POINT('Ctrl Pts',(-10.646155819192,-22.3522078165756,-2.95306559830315));
#93678=CARTESIAN_POINT('Ctrl Pts',(-10.6505367312537,-22.3558567328289,
-2.94014022159176));
#93679=CARTESIAN_POINT('Ctrl Pts',(-10.6540771116143,-22.3588055597533,
-2.92969473690327));
#93680=CARTESIAN_POINT('Ctrl Pts',(-10.6574866958116,-22.361273330863,-2.91916829324453));
#93681=CARTESIAN_POINT('Ctrl Pts',(-10.6607733565153,-22.3633442036669,
-2.9086173822976));
#93682=CARTESIAN_POINT('Ctrl Pts',(-10.6651828350991,-22.3661225462162,
-2.89446197653664));
#93683=CARTESIAN_POINT('Ctrl Pts',(-10.6693355569454,-22.3681818404446,
-2.88025185841365));
#93684=CARTESIAN_POINT('Ctrl Pts',(-10.6732963279558,-22.3697259156136,
-2.86602304448339));
#93685=CARTESIAN_POINT('Ctrl Pts',(-10.6774323877848,-22.3713383257386,
-2.8511645167987));
#93686=CARTESIAN_POINT('Ctrl Pts',(-10.6813598786535,-22.3723889750259,
-2.83628552145626));
#93687=CARTESIAN_POINT('Ctrl Pts',(-10.6851919722119,-22.3730728664481,
-2.82140498507979));
#93688=CARTESIAN_POINT('Ctrl Pts',(-10.6892557863458,-22.3737981116921,
-2.80562464644122));
#93689=CARTESIAN_POINT('Ctrl Pts',(-10.6932123001532,-22.374110482048,-2.78984241926712));
#93690=CARTESIAN_POINT('Ctrl Pts',(-10.697233260058,-22.3742040322445,-2.77405800409609));
#93691=CARTESIAN_POINT('Ctrl Pts',(-10.6981702131669,-22.3742258310561,
-2.77037996272886));
#93692=CARTESIAN_POINT('Ctrl Pts',(-10.6991108225775,-22.3742356128,-2.76670171793979));
#93693=CARTESIAN_POINT('Ctrl Pts',(-10.7000575594,-22.3742356128,-2.76302312605));
#93694=CARTESIAN_POINT('Origin',(2.84607155346,-22.6742356128,5.53854202767));
#93695=CARTESIAN_POINT('Origin',(-10.9467697490204,-22.6721143269662,-2.35059830462873));
#93696=CARTESIAN_POINT('Ctrl Pts',(-11.2053401891,-22.6742356128,-2.49849372966));
#93697=CARTESIAN_POINT('Ctrl Pts',(-11.2053401891,-22.5799878332,-2.49849372966));
#93698=CARTESIAN_POINT('Ctrl Pts',(-11.1732131726,-22.4857400536,-2.48011792621));
#93699=CARTESIAN_POINT('Ctrl Pts',(-11.1085499535,-22.4112466293,-2.44313227564));
#93700=CARTESIAN_POINT('Ctrl Pts',(-11.0267391777,-22.3742356128,-2.39633867638));
#93701=CARTESIAN_POINT('Ctrl Pts',(-10.9449284019,-22.3742356128,-2.34954507713));
#93702=CARTESIAN_POINT('Ctrl Pts',(-11.2476948874,-22.6742356128,-2.42444362923));
#93703=CARTESIAN_POINT('Ctrl Pts',(-11.2450653313,-22.5840941242,-2.429040968));
#93704=CARTESIAN_POINT('Ctrl Pts',(-11.2130113811,-22.4939526355,-2.41703302845));
#93705=CARTESIAN_POINT('Ctrl Pts',(-11.1517699452,-22.4209218727,-2.38727936284));
#93706=CARTESIAN_POINT('Ctrl Pts',(-11.0744430753,-22.3806857596,-2.34601859644));
#93707=CARTESIAN_POINT('Ctrl Pts',(-10.9959501219,-22.3742356128,-2.30169489009));
#93708=CARTESIAN_POINT('Ctrl Pts',(-11.2941946283,-22.6686213022,-2.34203463014));
#93709=CARTESIAN_POINT('Ctrl Pts',(-11.2868586676,-22.5829413188,-2.35499473105));
#93710=CARTESIAN_POINT('Ctrl Pts',(-11.2526857413,-22.4972613355,-2.35302785728));
#93711=CARTESIAN_POINT('Ctrl Pts',(-11.1928402247,-22.426280398,-2.33351209766));
#93712=CARTESIAN_POINT('Ctrl Pts',(-11.1189291588,-22.3836825181,-2.2998966476));
#93713=CARTESIAN_POINT('Ctrl Pts',(-11.043868081,-22.3714284849,-2.25918468729));
#93714=CARTESIAN_POINT('Ctrl Pts',(-11.3417981924,-22.6467118109,-2.25595171063));
#93715=CARTESIAN_POINT('Ctrl Pts',(-11.3291442479,-22.5660000486,-2.27877967267));
#93716=CARTESIAN_POINT('Ctrl Pts',(-11.2910933501,-22.4852882864,-2.28766776945));
#93717=CARTESIAN_POINT('Ctrl Pts',(-11.229550879,-22.4176465288,-2.27867532762));
#93718=CARTESIAN_POINT('Ctrl Pts',(-11.1557537306,-22.375311083,-2.25331234023));
#93719=CARTESIAN_POINT('Ctrl Pts',(-11.0817600114,-22.3604736068,-2.21745676256));
#93720=CARTESIAN_POINT('Ctrl Pts',(-11.4353537652,-22.5603047021,-2.08352845036));
#93721=CARTESIAN_POINT('Ctrl Pts',(-11.4121163918,-22.4942390833,-2.12677174602));
#93722=CARTESIAN_POINT('Ctrl Pts',(-11.3657157526,-22.4281734646,-2.15766880717));
#93723=CARTESIAN_POINT('Ctrl Pts',(-11.2994862528,-22.3717132431,-2.16962607727));
#93724=CARTESIAN_POINT('Ctrl Pts',(-11.2242843437,-22.3339703351,-2.16051799049));
#93725=CARTESIAN_POINT('Ctrl Pts',(-11.1508960681,-22.3172702763,-2.13427099913));
#93726=CARTESIAN_POINT('Ctrl Pts',(-11.5032693058,-22.4004263802,-1.95414386857));
#93727=CARTESIAN_POINT('Ctrl Pts',(-11.4721201637,-22.3564749274,-2.01366537708));
#93728=CARTESIAN_POINT('Ctrl Pts',(-11.418463566,-22.3125234745,-2.06143417372));
#93729=CARTESIAN_POINT('Ctrl Pts',(-11.3465841747,-22.2747985542,-2.0888955933));
#93730=CARTESIAN_POINT('Ctrl Pts',(-11.2678343078,-22.2492105131,-2.09172776553));
#93731=CARTESIAN_POINT('Ctrl Pts',(-11.1928782665,-22.237330862,-2.07277075552));
#93732=CARTESIAN_POINT('Ctrl Pts',(-11.5284593408,-22.2976444921,-1.90521795022));
#93733=CARTESIAN_POINT('Ctrl Pts',(-11.4944206426,-22.2676340437,-1.97094002685));
#93734=CARTESIAN_POINT('Ctrl Pts',(-11.4380739731,-22.2376235953,-2.02511044406));
#93735=CARTESIAN_POINT('Ctrl Pts',(-11.3640715597,-22.2118199507,-2.05839415541));
#93736=CARTESIAN_POINT('Ctrl Pts',(-11.283947635,-22.1942244807,-2.0655995494));
#93737=CARTESIAN_POINT('Ctrl Pts',(-11.208324537,-22.1859402315,-2.04918926595));
#93738=CARTESIAN_POINT('Ctrl Pts',(-11.5410916547,-22.1859264501,-1.88073379583));
#93739=CARTESIAN_POINT('Ctrl Pts',(-11.5055896574,-22.1709238273,-1.9495777849));
#93740=CARTESIAN_POINT('Ctrl Pts',(-11.4478685938,-22.1559212045,-2.00696368603));
#93741=CARTESIAN_POINT('Ctrl Pts',(-11.3727622471,-22.1430213573,-2.04316893107));
#93742=CARTESIAN_POINT('Ctrl Pts',(-11.2919149591,-22.1342242685,-2.05258032919));
#93743=CARTESIAN_POINT('Ctrl Pts',(-11.2159437174,-22.1300808784,-2.0374723572));
#93744=CARTESIAN_POINT('Ctrl Pts',(-11.5410916367,-22.0742358827,-1.88073379256));
#93745=CARTESIAN_POINT('Ctrl Pts',(-11.5055896399,-22.0742358104,-1.94957779219));
#93746=CARTESIAN_POINT('Ctrl Pts',(-11.4478685736,-22.0742357381,-2.00696370221));
#93747=CARTESIAN_POINT('Ctrl Pts',(-11.3727622216,-22.074235676,-2.04316895153));
#93748=CARTESIAN_POINT('Ctrl Pts',(-11.2919149284,-22.0742356336,-2.05258034776));
#93749=CARTESIAN_POINT('Ctrl Pts',(-11.2159436836,-22.0742356136,-2.03747236903));
#93750=CARTESIAN_POINT('',(-11.2159436600663,-22.0742356133472,-2.03747240750538));
#93751=CARTESIAN_POINT('Origin',(-11.2753946067519,-22.074235881436,-1.74517806931961));
#93752=CARTESIAN_POINT('Ctrl Pts',(-10.9449284019,-22.3742356128,-2.34954507713));
#93753=CARTESIAN_POINT('Ctrl Pts',(-10.9565768825276,-22.3742356128,-2.33862067127606));
#93754=CARTESIAN_POINT('Ctrl Pts',(-10.968280766592,-22.3740622680576,-2.32779191576226));
#93755=CARTESIAN_POINT('Ctrl Pts',(-10.979949755164,-22.37354310181,-2.31690595964475));
#93756=CARTESIAN_POINT('Ctrl Pts',(-10.9911689868806,-22.373043945744,-2.30643958002794));
#93757=CARTESIAN_POINT('Ctrl Pts',(-11.0023563344253,-22.372225707338,-2.29592034716022));
#93758=CARTESIAN_POINT('Ctrl Pts',(-11.0134389745054,-22.3709040042025,
-2.28524712449359));
#93759=CARTESIAN_POINT('Ctrl Pts',(-11.0238481066063,-22.3696626228676,
-2.27522252892091));
#93760=CARTESIAN_POINT('Ctrl Pts',(-11.0341647801129,-22.3679770644684,
-2.26506174680759));
#93761=CARTESIAN_POINT('Ctrl Pts',(-11.0443340519157,-22.3656632096047,
-2.25471467683243));
#93762=CARTESIAN_POINT('Ctrl Pts',(-11.0474655616257,-22.3649506847441,
-2.25152841623034));
#93763=CARTESIAN_POINT('Ctrl Pts',(-11.0505831413501,-22.3641783511552,
-2.24832476821515));
#93764=CARTESIAN_POINT('Ctrl Pts',(-11.0536853244324,-22.3633402225444,
-2.24510308453649));
#93765=CARTESIAN_POINT('Ctrl Pts',(-11.0633642697261,-22.3607252250548,
-2.23505129221736));
#93766=CARTESIAN_POINT('Ctrl Pts',(-11.0728793857902,-22.3574725336843,
-2.22483316903463));
#93767=CARTESIAN_POINT('Ctrl Pts',(-11.0821562752923,-22.3534133609767,
-2.2145039537747));
#93768=CARTESIAN_POINT('Ctrl Pts',(-11.0896802081132,-22.3501212076366,
-2.20612654217665));
#93769=CARTESIAN_POINT('Ctrl Pts',(-11.0970483562335,-22.3462982180438,
-2.19767660347488));
#93770=CARTESIAN_POINT('Ctrl Pts',(-11.1042297129877,-22.3418596791366,
-2.18920695368937));
#93771=CARTESIAN_POINT('Ctrl Pts',(-11.1122476406949,-22.3369040857435,
-2.17975065705759));
#93772=CARTESIAN_POINT('Ctrl Pts',(-11.1200316088684,-22.331181788504,-2.17027399083279));
#93773=CARTESIAN_POINT('Ctrl Pts',(-11.1276410948107,-22.3246179799789,
-2.16092525729618));
#93774=CARTESIAN_POINT('Ctrl Pts',(-11.1314458377819,-22.3213360757163,
-2.15625089052788));
#93775=CARTESIAN_POINT('Ctrl Pts',(-11.1351832582712,-22.317839173301,-2.15159900315221));
#93776=CARTESIAN_POINT('Ctrl Pts',(-11.1388218124651,-22.3141117280667,
-2.14697715269855));
#93777=CARTESIAN_POINT('Ctrl Pts',(-11.139525886561,-22.3133904532158,-2.14608280703086));
#93778=CARTESIAN_POINT('Ctrl Pts',(-11.1402262722922,-22.312660544195,-2.145189591596));
#93779=CARTESIAN_POINT('Ctrl Pts',(-11.1409228190846,-22.3119219228704,
-2.144297623045));
#93780=CARTESIAN_POINT('Ctrl Pts',(-11.1420260993752,-22.3107519995309,
-2.14288480866867));
#93781=CARTESIAN_POINT('Ctrl Pts',(-11.1431197477329,-22.3095602176583,
-2.1414751213253));
#93782=CARTESIAN_POINT('Ctrl Pts',(-11.1442033086172,-22.308346245778,-2.14006904278067));
#93783=CARTESIAN_POINT('Ctrl Pts',(-11.1452339612863,-22.3071915498336,
-2.13873162037472));
#93784=CARTESIAN_POINT('Ctrl Pts',(-11.1464488402109,-22.3057917228803,
-2.13714291255623));
#93785=CARTESIAN_POINT('Ctrl Pts',(-11.1475069745288,-22.3045370649081,
-2.13575056520196));
#93786=CARTESIAN_POINT('Ctrl Pts',(-11.1482636315973,-22.3036398765197,
-2.13475491706011));
#93787=CARTESIAN_POINT('Ctrl Pts',(-11.1489410725372,-22.3028181867498,
-2.13385890924935));
#93788=CARTESIAN_POINT('Ctrl Pts',(-11.1494233819929,-22.3022264767122,
-2.13321857299617));
#93789=CARTESIAN_POINT('Ctrl Pts',(-11.1557486448315,-22.29446647643,-2.12482086264944));
#93790=CARTESIAN_POINT('Ctrl Pts',(-11.1618495924945,-22.2858526143557,
-2.1165696985762));
#93791=CARTESIAN_POINT('Ctrl Pts',(-11.1676296764402,-22.2763188870647,
-2.10861659005254));
#93792=CARTESIAN_POINT('Ctrl Pts',(-11.1731962959871,-22.2671372500517,
-2.10095719794287));
#93793=CARTESIAN_POINT('Ctrl Pts',(-11.1784653901721,-22.2571017817321,
-2.09357457146205));
#93794=CARTESIAN_POINT('Ctrl Pts',(-11.1833374488865,-22.2461885091507,
-2.08663413877296));
#93795=CARTESIAN_POINT('Ctrl Pts',(-11.1882095076009,-22.2352752365692,
-2.07969370608386));
#93796=CARTESIAN_POINT('Ctrl Pts',(-11.1926845419211,-22.2234833193454,
-2.07319587467472));
#93797=CARTESIAN_POINT('Ctrl Pts',(-11.1966487080552,-22.2108358475213,
-2.06733170400025));
#93798=CARTESIAN_POINT('Ctrl Pts',(-11.2004710745941,-22.1986407801437,
-2.06167729674131));
#93799=CARTESIAN_POINT('Ctrl Pts',(-11.2038037915588,-22.1856447995889,
-2.05660690044393));
#93800=CARTESIAN_POINT('Ctrl Pts',(-11.2065790246433,-22.1719101123269,
-2.05231577287415));
#93801=CARTESIAN_POINT('Ctrl Pts',(-11.2092944749749,-22.1584712911741,
-2.04811708273626));
#93802=CARTESIAN_POINT('Ctrl Pts',(-11.2114758661764,-22.1443248656484,
-2.04466512644328));
#93803=CARTESIAN_POINT('Ctrl Pts',(-11.2130487391782,-22.1295766664627,
-2.04215055378544));
#93804=CARTESIAN_POINT('Ctrl Pts',(-11.2145585009443,-22.1154202360173,
-2.03973687788627));
#93805=CARTESIAN_POINT('Ctrl Pts',(-11.2155070568181,-22.1007092604967,
-2.0381878039234));
#93806=CARTESIAN_POINT('Ctrl Pts',(-11.2158247434131,-22.0855848206322,
-2.03766750097925));
#93807=CARTESIAN_POINT('Ctrl Pts',(-11.2159036934711,-22.0818261621817,
-2.03753819760833));
#93808=CARTESIAN_POINT('Ctrl Pts',(-11.2159436859039,-22.0780422089381,
-2.03747236822363));
#93809=CARTESIAN_POINT('Ctrl Pts',(-11.2159436836,-22.0742356136,-2.03747236903));
#93810=CARTESIAN_POINT('Origin',(-11.2744572343,-19.6742356128,-1.7432341771));
#93811=CARTESIAN_POINT('Origin',(-11.2744572343,-19.6742356128,-1.7432341771));
#93812=CARTESIAN_POINT('Origin',(-11.2744572343,-21.2742356128,-1.7432341771));
#93813=CARTESIAN_POINT('',(-11.2159436339,-20.8742356128,-2.03747244546));
#93814=CARTESIAN_POINT('Origin',(-10.3267865236,-21.2742356128,-3.3434289261));
#93815=CARTESIAN_POINT('Origin',(-10.3267865236,-19.6742356128,-3.3434289261));
#93816=CARTESIAN_POINT('',(-10.5566756949,-20.8742356128,-3.15068305993));
#93817=CARTESIAN_POINT('Origin',(-6.6707290414,-19.6742356128,10.1304528845));
#93818=CARTESIAN_POINT('Origin',(-2.45,-19.6742356128,10.1304528845));
#93819=CARTESIAN_POINT('',(-2.88657986403E-14,-19.6742356128,10.4304528845));
#93820=CARTESIAN_POINT('Origin',(-2.75,-19.3742356128,10.4304528845));
#93821=CARTESIAN_POINT('',(-1.375,-20.6742356128,10.4304528845));
#93822=CARTESIAN_POINT('Origin',(-1.375,-20.6742356128,10.7304528845));
#93823=CARTESIAN_POINT('',(-2.45,-20.9304376384,10.5743743079));
#93824=CARTESIAN_POINT('Origin',(-2.45,-20.6742356128,10.7304528845));
#93825=CARTESIAN_POINT('',(-1.82443078508723,-20.9742355917829,10.7304528845));
#93826=CARTESIAN_POINT('Ctrl Pts',(-2.45000000001651,-20.9304376384374,
10.5743743079454));
#93827=CARTESIAN_POINT('Ctrl Pts',(-2.44729189173785,-20.9308368579965,
10.5750296244019));
#93828=CARTESIAN_POINT('Ctrl Pts',(-2.44457723791173,-20.9312343514944,
10.5756877663935));
#93829=CARTESIAN_POINT('Ctrl Pts',(-2.33821087635373,-20.9467017934165,
10.6015224622014));
#93830=CARTESIAN_POINT('Ctrl Pts',(-2.23664227464802,-20.957470549854,10.6278009815082));
#93831=CARTESIAN_POINT('Ctrl Pts',(-2.0775138014278,-20.9680551199903,10.6682233822152));
#93832=CARTESIAN_POINT('Ctrl Pts',(-2.02332178583692,-20.9705889581146,
10.6818849323202));
#93833=CARTESIAN_POINT('Ctrl Pts',(-1.93823023557501,-20.9730684400875,
10.7029370878533));
#93834=CARTESIAN_POINT('Ctrl Pts',(-1.90756560839508,-20.973660008163,10.710444942518));
#93835=CARTESIAN_POINT('Ctrl Pts',(-1.85938817655537,-20.9741488490342,
10.722093182511));
#93836=CARTESIAN_POINT('Ctrl Pts',(-1.84191849476494,-20.9742356126494,
10.7262868288948));
#93837=CARTESIAN_POINT('Ctrl Pts',(-1.82443078250423,-20.9742356128,10.7304528736574));
#93838=CARTESIAN_POINT('',(-4.4408920985E-16,-20.9742356128,10.7304528845));
#93839=CARTESIAN_POINT('Origin',(-1.97861558624E-15,-21.2742356128,0.580061096523));
#93840=CARTESIAN_POINT('',(-2.45,-20.9742356128,15.7712943679));
#93841=CARTESIAN_POINT('Origin',(2.78569866985E-16,-20.9742356128,0.580061096523));
#93842=CARTESIAN_POINT('Origin',(-2.45000000000807,-21.2742356128,15.7712943679849));
#93843=CARTESIAN_POINT('Origin',(2.69422295812E-16,-20.9742356128,0.729452270839));
#93844=CARTESIAN_POINT('',(-1.01362101456,-20.9742356128,10.8791871183));
#93845=CARTESIAN_POINT('Origin',(-0.00234352656470205,-20.9742355812827,
3.0819174256968));
#93846=CARTESIAN_POINT('',(-0.767157287525,-20.9742356128,11.1596805575));
#93847=CARTESIAN_POINT('Origin',(-1.05,-20.9742356128,11.1596805575));
#93848=CARTESIAN_POINT('',(-0.767157287525,-20.9742356128,14.92922515));
#93849=CARTESIAN_POINT('',(-0.767157287525,-20.9742356128,12.1167294155));
#93850=CARTESIAN_POINT('',(-1.07064182355,-20.9742356128,15.2113136381));
#93851=CARTESIAN_POINT('Origin',(-1.05,-20.9742356128,14.92922515));
#93852=CARTESIAN_POINT('',(-2.45000000041083,-20.9742356123072,15.0444077749624));
#93853=CARTESIAN_POINT('Origin',(5.40116187885964E-9,-20.9742356120504,
0.58006109717732));
#93854=CARTESIAN_POINT('',(-2.45,-20.9742356128,13.3490218086));
#93855=CARTESIAN_POINT('Origin',(-3.05,-19.6742356128,15.662287998));
#93856=CARTESIAN_POINT('',(-2.75,-19.6742356128,15.662287998));
#93857=CARTESIAN_POINT('Origin',(-3.05,-19.6742356128,15.662287998));
#93858=CARTESIAN_POINT('Origin',(-3.05,-19.6742356128,15.662287998));
#93859=CARTESIAN_POINT('',(-2.97246042119851,-19.3848539651149,15.6779684221767));
#93860=CARTESIAN_POINT('Origin',(-3.05,-19.6742356128,15.662287998));
#93861=CARTESIAN_POINT('Origin',(-3.05,-19.6742356128,2.96634320571));
#93862=CARTESIAN_POINT('',(-2.75,-19.6742356128,13.1963704412));
#93863=CARTESIAN_POINT('Origin',(-3.05,-19.6742356128,10.7304528845));
#93864=CARTESIAN_POINT('Origin',(-3.05,-22.4223864096,15.662287998));
#93865=CARTESIAN_POINT('',(-2.750000005455,-20.6742356128438,15.6622879962));
#93866=CARTESIAN_POINT('Ctrl Pts',(-2.75,-20.6742356128,15.6622879962));
#93867=CARTESIAN_POINT('Ctrl Pts',(-2.75000002192,-20.6742356209121,15.7685078015738));
#93868=CARTESIAN_POINT('Ctrl Pts',(-2.79701105507061,-20.6742356114132,
15.8747276069476));
#93869=CARTESIAN_POINT('Ctrl Pts',(-2.89192095826334,-20.6742355819167,
15.9523655950137));
#93870=CARTESIAN_POINT('Ctrl Pts',(-3.00535144290051,-20.6742355416214,
15.9773898040232));
#93871=CARTESIAN_POINT('Ctrl Pts',(-3.10946375772823,-20.6742355012,15.9563357177875));
#93872=CARTESIAN_POINT('',(-2.75,-20.1742356128,15.662287998));
#93873=CARTESIAN_POINT('Origin',(-2.75,-19.3742356128,10.4304528845));
#93874=CARTESIAN_POINT('',(-2.75,-20.6742356128,13.3490218086));
#93875=CARTESIAN_POINT('Ctrl Pts',(-3.1094637805,-20.6742355012,15.9563357204));
#93876=CARTESIAN_POINT('Ctrl Pts',(-3.00535146138,-20.6742355416,15.9773898081));
#93877=CARTESIAN_POINT('Ctrl Pts',(-2.89192096986,-20.6742355819,15.9523656045));
#93878=CARTESIAN_POINT('Ctrl Pts',(-2.7970110589,-20.6742356114,15.8747276156));
#93879=CARTESIAN_POINT('Ctrl Pts',(-2.75000002192,-20.6742356209,15.7685078059));
#93880=CARTESIAN_POINT('Ctrl Pts',(-2.75000002182,-20.6742356129,15.6622879962));
#93881=CARTESIAN_POINT('Ctrl Pts',(-3.10946380353,-20.7613039297,15.9563357159));
#93882=CARTESIAN_POINT('Ctrl Pts',(-3.00535147528,-20.7455779654,15.9773898056));
#93883=CARTESIAN_POINT('Ctrl Pts',(-2.89192097435,-20.7298520012,15.9523656029));
#93884=CARTESIAN_POINT('Ctrl Pts',(-2.79701105681,-20.7183575883,15.8747276131));
#93885=CARTESIAN_POINT('Ctrl Pts',(-2.75000001886,-20.7146527462,15.7685078017));
#93886=CARTESIAN_POINT('Ctrl Pts',(-2.75000002231,-20.7177698279,15.6622879905));
#93887=CARTESIAN_POINT('Ctrl Pts',(-3.09336559174,-20.8484128662,15.9595900965));
#93888=CARTESIAN_POINT('Ctrl Pts',(-2.99245619263,-20.8169453132,15.9798833716));
#93889=CARTESIAN_POINT('Ctrl Pts',(-2.88234381849,-20.7854777603,15.9544199132));
#93890=CARTESIAN_POINT('Ctrl Pts',(-2.78979771265,-20.7624813454,15.8769278231));
#93891=CARTESIAN_POINT('Ctrl Pts',(-2.74323291398,-20.755077053,15.7712039881));
#93892=CARTESIAN_POINT('Ctrl Pts',(-2.74210499444,-20.7613240613,15.6654801511));
#93893=CARTESIAN_POINT('Ctrl Pts',(-3.0611129676,-20.9309303248,15.9661188953));
#93894=CARTESIAN_POINT('Ctrl Pts',(-2.96663575098,-20.8849847431,15.9848817048));
#93895=CARTESIAN_POINT('Ctrl Pts',(-2.86318716199,-20.8390391614,15.9585340485));
#93896=CARTESIAN_POINT('Ctrl Pts',(-2.77538294467,-20.80528071,15.8813354034));
#93897=CARTESIAN_POINT('Ctrl Pts',(-2.72969914456,-20.7940068531,15.7766097304));
#93898=CARTESIAN_POINT('Ctrl Pts',(-2.72628672053,-20.8025832991,15.6718840609));
#93899=CARTESIAN_POINT('Ctrl Pts',(-2.95857415151,-21.0968055424,15.9864129862));
#93900=CARTESIAN_POINT('Ctrl Pts',(-2.883615269,-21.0232686806,16.0006863819));
#93901=CARTESIAN_POINT('Ctrl Pts',(-2.80037813885,-20.9497318188,15.9717891925));
#93902=CARTESIAN_POINT('Ctrl Pts',(-2.72731697454,-20.8948262684,15.8954574233));
#93903=CARTESIAN_POINT('Ctrl Pts',(-2.68525006547,-20.8745215131,15.7936237677));
#93904=CARTESIAN_POINT('Ctrl Pts',(-2.67599823713,-20.8855201685,15.6917901077));
#93905=CARTESIAN_POINT('Ctrl Pts',(-2.802073414,-21.210145586,16.0157241263));
#93906=CARTESIAN_POINT('Ctrl Pts',(-2.75443180074,-21.1206683319,16.0242286253));
#93907=CARTESIAN_POINT('Ctrl Pts',(-2.69943877243,-21.0311910779,15.9921593039));
#93908=CARTESIAN_POINT('Ctrl Pts',(-2.64793358485,-20.9628100879,15.9169517332));
#93909=CARTESIAN_POINT('Ctrl Pts',(-2.61350648776,-20.9339674316,15.8187461919));
#93910=CARTESIAN_POINT('Ctrl Pts',(-2.59924369788,-20.942191106,15.7205406559));
#93911=CARTESIAN_POINT('Ctrl Pts',(-2.70443397686,-21.2527626391,16.0332525536));
#93912=CARTESIAN_POINT('Ctrl Pts',(-2.67281955818,-21.1584143796,16.038616685));
#93913=CARTESIAN_POINT('Ctrl Pts',(-2.63437509944,-21.0640661201,16.0048673446));
#93914=CARTESIAN_POINT('Ctrl Pts',(-2.59591773658,-20.9910117695,15.9302754357));
#93915=CARTESIAN_POINT('Ctrl Pts',(-2.56711899741,-20.9580670061,15.8340046748));
#93916=CARTESIAN_POINT('Ctrl Pts',(-2.55135784288,-20.9634991119,15.7377339138));
#93917=CARTESIAN_POINT('Ctrl Pts',(-2.60121936463,-21.2742356128,16.0507826341));
#93918=CARTESIAN_POINT('Ctrl Pts',(-2.58568379068,-21.1783721495,16.0532881684));
#93919=CARTESIAN_POINT('Ctrl Pts',(-2.56380921231,-21.0825086862,16.0180414277));
#93920=CARTESIAN_POINT('Ctrl Pts',(-2.53876678585,-21.0074397583,15.9440093758));
#93921=CARTESIAN_POINT('Ctrl Pts',(-2.51662240651,-20.9716977028,15.8494690665));
#93922=CARTESIAN_POINT('Ctrl Pts',(-2.50073751227,-20.9742356128,15.7549287572));
#93923=CARTESIAN_POINT('Ctrl Pts',(-2.49776595187,-21.2742356128,16.0674673138));
#93924=CARTESIAN_POINT('Ctrl Pts',(-2.49776595187,-21.1799878332,16.0674673138));
#93925=CARTESIAN_POINT('Ctrl Pts',(-2.49187306376,-21.0857400536,16.0309284411));
#93926=CARTESIAN_POINT('Ctrl Pts',(-2.4800122327,-21.0112466293,15.9573853181));
#93927=CARTESIAN_POINT('Ctrl Pts',(-2.46500611635,-20.9742356128,15.864339843));
#93928=CARTESIAN_POINT('Ctrl Pts',(-2.45,-20.9742356128,15.7712943679));
#93929=CARTESIAN_POINT('Ctrl Pts',(-2.75000002182,-20.6742356129,15.6622879962));
#93930=CARTESIAN_POINT('Ctrl Pts',(-2.75000002198767,-20.6891327288188,
15.662287996202));
#93931=CARTESIAN_POINT('Ctrl Pts',(-2.7488884673052,-20.7043898896441,15.6627908269653));
#93932=CARTESIAN_POINT('Ctrl Pts',(-2.74651746486329,-20.7198130389006,
15.6638118403573));
#93933=CARTESIAN_POINT('Ctrl Pts',(-2.74423092920776,-20.7346867396071,
15.6647964802227));
#93934=CARTESIAN_POINT('Ctrl Pts',(-2.74077278856836,-20.7497146973984,
15.6662631994214));
#93935=CARTESIAN_POINT('Ctrl Pts',(-2.73603745825241,-20.7646874654371,
15.6682067376741));
#93936=CARTESIAN_POINT('Ctrl Pts',(-2.7338400705365,-20.7716354446415,15.6691086192318));
#93937=CARTESIAN_POINT('Ctrl Pts',(-2.73136807582815,-20.778571039602,15.6701128877873));
#93938=CARTESIAN_POINT('Ctrl Pts',(-2.72861328945327,-20.7854707230258,
15.6712174187728));
#93939=CARTESIAN_POINT('Ctrl Pts',(-2.72296675191468,-20.799613134144,15.6734813967454));
#93940=CARTESIAN_POINT('Ctrl Pts',(-2.71613031669946,-20.8136044725922,
15.6761744654426));
#93941=CARTESIAN_POINT('Ctrl Pts',(-2.70806242614445,-20.8272155055718,
15.6793002985697));
#93942=CARTESIAN_POINT('Ctrl Pts',(-2.70552338278455,-20.8314990295826,
15.6802840285536));
#93943=CARTESIAN_POINT('Ctrl Pts',(-2.70286266137133,-20.8357446890429,
15.6813104484459));
#93944=CARTESIAN_POINT('Ctrl Pts',(-2.70007978559827,-20.8399448481202,
15.6823791917623));
#93945=CARTESIAN_POINT('Ctrl Pts',(-2.69426700983312,-20.8487179967928,
15.6846115462601));
#93946=CARTESIAN_POINT('Ctrl Pts',(-2.68792075017705,-20.857292667102,15.687029930608));
#93947=CARTESIAN_POINT('Ctrl Pts',(-2.68104398035804,-20.8655956668358,
15.6896343447235));
#93948=CARTESIAN_POINT('Ctrl Pts',(-2.67941833810201,-20.8675584644246,
15.6902500183246));
#93949=CARTESIAN_POINT('Ctrl Pts',(-2.67776307577371,-20.8695060866975,
15.6908760803931));
#93950=CARTESIAN_POINT('Ctrl Pts',(-2.67607832738159,-20.8714375297582,
15.6915125453967));
#93951=CARTESIAN_POINT('Ctrl Pts',(-2.67419967587668,-20.8735912688148,
15.6922222632052));
#93952=CARTESIAN_POINT('Ctrl Pts',(-2.67228435995548,-20.8757248910275,
15.6929449165403));
#93953=CARTESIAN_POINT('Ctrl Pts',(-2.67033263730239,-20.8778369880354,
15.6936804881095));
#93954=CARTESIAN_POINT('Ctrl Pts',(-2.66859870637496,-20.879713397226,15.6943339776262));
#93955=CARTESIAN_POINT('Ctrl Pts',(-2.66660548636659,-20.8818162220527,
15.6950847913152));
#93956=CARTESIAN_POINT('Ctrl Pts',(-2.66467211375905,-20.8837967669163,
15.6958131945261));
#93957=CARTESIAN_POINT('Ctrl Pts',(-2.66247767151406,-20.8860447512417,
15.696639956409));
#93958=CARTESIAN_POINT('Ctrl Pts',(-2.66036059309485,-20.8881350146166,
15.6974377084262));
#93959=CARTESIAN_POINT('Ctrl Pts',(-2.65883635900915,-20.889613008879,15.6980158102704));
#93960=CARTESIAN_POINT('Ctrl Pts',(-2.65162649322279,-20.8966041530638,
15.7007503224732));
#93961=CARTESIAN_POINT('Ctrl Pts',(-2.643585031057,-20.9037016639627,15.7037798378816));
#93962=CARTESIAN_POINT('Ctrl Pts',(-2.63461960904651,-20.9107022452566,
15.7071214036503));
#93963=CARTESIAN_POINT('Ctrl Pts',(-2.62932398864371,-20.9148372899971,
15.7090951717385));
#93964=CARTESIAN_POINT('Ctrl Pts',(-2.62370631841184,-20.9189376969414,
15.7111775798599));
#93965=CARTESIAN_POINT('Ctrl Pts',(-2.61775168794802,-20.9229543962997,
15.7133695690179));
#93966=CARTESIAN_POINT('Ctrl Pts',(-2.61173828221312,-20.9270107425505,
15.7155831942383));
#93967=CARTESIAN_POINT('Ctrl Pts',(-2.60538119420661,-20.9309816775041,
15.7179085866684));
#93968=CARTESIAN_POINT('Ctrl Pts',(-2.59867000660302,-20.9348109629388,
15.7203441452));
#93969=CARTESIAN_POINT('Ctrl Pts',(-2.59692526996035,-20.9358064789351,
15.7209773279489));
#93970=CARTESIAN_POINT('Ctrl Pts',(-2.59515662848469,-20.9367923932735,
15.7216179421837));
#93971=CARTESIAN_POINT('Ctrl Pts',(-2.59336396019278,-20.937767659153,15.7222659288205));
#93972=CARTESIAN_POINT('Ctrl Pts',(-2.59239613536374,-20.938294185191,15.7226157635105));
#93973=CARTESIAN_POINT('Ctrl Pts',(-2.59142541592154,-20.938815485287,15.7229662682405));
#93974=CARTESIAN_POINT('Ctrl Pts',(-2.59042809853723,-20.9393437769894,
15.7233259661923));
#93975=CARTESIAN_POINT('Ctrl Pts',(-2.58679089344647,-20.9412704507842,
15.7246377805071));
#93976=CARTESIAN_POINT('Ctrl Pts',(-2.58285965075778,-20.9432522129818,
15.726049979423));
#93977=CARTESIAN_POINT('Ctrl Pts',(-2.57890122778666,-20.9451356436071,
15.7274652287701));
#93978=CARTESIAN_POINT('Ctrl Pts',(-2.57595883428822,-20.9465356440787,
15.7285172185418));
#93979=CARTESIAN_POINT('Ctrl Pts',(-2.57300196178022,-20.9478822490868,
15.7295707596454));
#93980=CARTESIAN_POINT('Ctrl Pts',(-2.57014764205019,-20.9491296563122,
15.730584465258));
#93981=CARTESIAN_POINT('Ctrl Pts',(-2.56747171730329,-20.9502991005859,
15.7315348142698));
#93982=CARTESIAN_POINT('Ctrl Pts',(-2.56488607804088,-20.9513816261541,
15.7324501148568));
#93983=CARTESIAN_POINT('Ctrl Pts',(-2.56249084795086,-20.9523502970827,
15.7332957897429));
#93984=CARTESIAN_POINT('Ctrl Pts',(-2.56198673178439,-20.9525541700539,
15.7334737761432));
#93985=CARTESIAN_POINT('Ctrl Pts',(-2.56148899337878,-20.9527538885307,
15.7336494084665));
#93986=CARTESIAN_POINT('Ctrl Pts',(-2.56098799203385,-20.9529533606897,
15.7338260904627));
#93987=CARTESIAN_POINT('Ctrl Pts',(-2.54305852071686,-20.960091925069,15.7401490570897));
#93988=CARTESIAN_POINT('Ctrl Pts',(-2.52444947588824,-20.9654910132208,
15.7465790967645));
#93989=CARTESIAN_POINT('Ctrl Pts',(-2.50548871504351,-20.9690589576089,
15.7529798707704));
#93990=CARTESIAN_POINT('Ctrl Pts',(-2.48721902877561,-20.9724968589213,
15.7591473518076));
#93991=CARTESIAN_POINT('Ctrl Pts',(-2.46862329501776,-20.9742356128,15.7652873410953));
#93992=CARTESIAN_POINT('Ctrl Pts',(-2.45,-20.9742356128,15.7712943679));
#93993=CARTESIAN_POINT('Origin',(-2.45,-20.6742356128,13.3490218086));
#93994=CARTESIAN_POINT('',(-2.7328425359048,-20.7742356128,14.7056612864094));
#93995=CARTESIAN_POINT('Ctrl Pts',(-2.45000000049961,-20.9742356128,15.0444077754865));
#93996=CARTESIAN_POINT('Ctrl Pts',(-2.4505642246363,-20.9742356127991,15.0443122060722));
#93997=CARTESIAN_POINT('Ctrl Pts',(-2.45112837604849,-20.9742340210488,
15.0442160442459));
#93998=CARTESIAN_POINT('Ctrl Pts',(-2.45271374680238,-20.9742250770619,
15.0439441126589));
#93999=CARTESIAN_POINT('Ctrl Pts',(-2.45373475694185,-20.9742141013729,
15.0437670015517));
#94000=CARTESIAN_POINT('Ctrl Pts',(-2.45684314513659,-20.9741648228718,
15.0432217654727));
#94001=CARTESIAN_POINT('Ctrl Pts',(-2.4589292490415,-20.9741099489642,15.0428475546937));
#94002=CARTESIAN_POINT('Ctrl Pts',(-2.47343386336903,-20.9735771126508,
15.0401878296793));
#94003=CARTESIAN_POINT('Ctrl Pts',(-2.48577021911375,-20.9723499449582,
15.0376330465997));
#94004=CARTESIAN_POINT('Ctrl Pts',(-2.4979272248846,-20.9703825039113,15.0347954601426));
#94005=CARTESIAN_POINT('Ctrl Pts',(-2.52673836491087,-20.9657198245833,
15.0280706051666));
#94006=CARTESIAN_POINT('Ctrl Pts',(-2.55429827846532,-20.9569165134737,
15.0198723368218));
#94007=CARTESIAN_POINT('Ctrl Pts',(-2.5945651553735,-20.9376298024471,15.0033035455715));
#94008=CARTESIAN_POINT('Ctrl Pts',(-2.60860989911875,-20.929371510587,14.9964054063729));
#94009=CARTESIAN_POINT('Ctrl Pts',(-2.64141722292707,-20.906490382548,14.9765328685671));
#94010=CARTESIAN_POINT('Ctrl Pts',(-2.65833205103465,-20.8911324882057,
14.962552890661));
#94011=CARTESIAN_POINT('Ctrl Pts',(-2.69268191586262,-20.8531499395656,
14.9219853022821));
#94012=CARTESIAN_POINT('Ctrl Pts',(-2.70622600372626,-20.8315298749212,
14.8938483721785));
#94013=CARTESIAN_POINT('Ctrl Pts',(-2.72505121860894,-20.795769394928,14.826784031487));
#94014=CARTESIAN_POINT('Ctrl Pts',(-2.72971376844571,-20.7828404745285,
14.7890007210827));
#94015=CARTESIAN_POINT('Ctrl Pts',(-2.73248325800256,-20.7752696738283,
14.7349347464044));
#94016=CARTESIAN_POINT('Ctrl Pts',(-2.73284271189799,-20.7742356144309,
14.7202906426028));
#94017=CARTESIAN_POINT('Ctrl Pts',(-2.73284271247462,-20.7742356128,14.7056612864095));
#94018=CARTESIAN_POINT('',(-2.73284184833111,-20.7742356128,10.7560440517756));
#94019=CARTESIAN_POINT('',(-2.73284210357,-20.7742356128,12.7308526862));
#94020=CARTESIAN_POINT('',(-2.73249401778459,-20.7752152053705,10.7304528485382));
#94021=CARTESIAN_POINT('Origin',(-2.61837242878611,-21.0942392376549,10.8006651608268));
#94022=CARTESIAN_POINT('Origin',(-2.45,-20.6742356128,10.7304528845));
#94023=CARTESIAN_POINT('Origin',(-6.51383560964,-21.0742356128,10.9320666897));
#94024=CARTESIAN_POINT('',(-4.98919124473,-20.7742356128,9.52235136777));
#94025=CARTESIAN_POINT('',(-8.14487887576,-20.7742356128,12.4401604693));
#94026=CARTESIAN_POINT('',(-6.56703506025,-20.7742356128,10.9812559186));
#94027=CARTESIAN_POINT('Origin',(-8.14487887576,-21.0742356128,12.4401604693));
#94028=CARTESIAN_POINT('Origin',(-4.98919124473,-21.0742356128,9.52235136777));
#94029=CARTESIAN_POINT('Origin',(-4.98919124473,-21.0742356128,9.52235136777));
#94030=CARTESIAN_POINT('Origin',(-4.98919124473,-21.0742356128,9.52235136777));
#94031=CARTESIAN_POINT('Origin',(-0.00234331738803,-21.0742356128,3.08191746407));
#94032=CARTESIAN_POINT('Ctrl Pts',(-2.73249449536286,-20.7752151161147,
10.7304528285094));
#94033=CARTESIAN_POINT('Ctrl Pts',(-2.73245710700268,-20.7753197109045,
10.7290952012981));
#94034=CARTESIAN_POINT('Ctrl Pts',(-2.73240712664869,-20.7754319433538,
10.727752397751));
#94035=CARTESIAN_POINT('Ctrl Pts',(-2.73152298709635,-20.7771409318656,
10.7087546905869));
#94036=CARTESIAN_POINT('Ctrl Pts',(-2.72772545244807,-20.7809744979902,
10.6881339522637));
#94037=CARTESIAN_POINT('Ctrl Pts',(-2.71679996433014,-20.790736326335,10.6559122059645));
#94038=CARTESIAN_POINT('Ctrl Pts',(-2.70771619875055,-20.7984214920223,
10.6384138803735));
#94039=CARTESIAN_POINT('Ctrl Pts',(-2.68765731828287,-20.8146185581327,
10.6112737349406));
#94040=CARTESIAN_POINT('Ctrl Pts',(-2.67249689114102,-20.8263682945712,
10.5972506978324));
#94041=CARTESIAN_POINT('Ctrl Pts',(-2.63942576926425,-20.8502432000307,
10.5761069546454));
#94042=CARTESIAN_POINT('Ctrl Pts',(-2.61427989630385,-20.8668329470141,
10.5673521750875));
#94043=CARTESIAN_POINT('Ctrl Pts',(-2.57563645957668,-20.8884881384831,
10.5611700175102));
#94044=CARTESIAN_POINT('Ctrl Pts',(-2.55565602930818,-20.8983536598198,
10.5602963146483));
#94045=CARTESIAN_POINT('Ctrl Pts',(-2.51151087548645,-20.9166072793448,
10.562148593287));
#94046=CARTESIAN_POINT('Ctrl Pts',(-2.48028974593003,-20.925972433295,10.5670447011082));
#94047=CARTESIAN_POINT('Ctrl Pts',(-2.45000000001651,-20.9304376384374,
10.5743743079454));
#94048=CARTESIAN_POINT('Origin',(-0.00234331738835,-20.7742356128,3.08191746407));
#94049=CARTESIAN_POINT('Origin',(-1.05,-21.0742356128,11.1596805575));
#94050=CARTESIAN_POINT('Origin',(-1.05,-21.0742356128,11.1596805575));
#94051=CARTESIAN_POINT('Origin',(-1.05,-21.0742356128,11.1596805575));
#94052=CARTESIAN_POINT('Origin',(-1.05,-21.0742356128,12.1167294155));
#94053=CARTESIAN_POINT('Origin',(-1.05,-21.0742356128,14.92922515));
#94054=CARTESIAN_POINT('Origin',(-8.14487887576,-21.0742356128,12.4401604693));
#94055=CARTESIAN_POINT('Origin',(-8.14487887576,-21.0742356128,12.4401604693));
#94056=CARTESIAN_POINT('Origin',(-1.05,-21.0742356128,14.92922515));
#94057=CARTESIAN_POINT('Origin',(-1.05,-21.0742356128,14.92922515));
#94058=CARTESIAN_POINT('Origin',(-1.51003344041E-15,-21.0742356128,0.580061096523));
#94059=CARTESIAN_POINT('Origin',(-5.42499920527E-16,-20.7742356128,0.580061096523));
#94060=CARTESIAN_POINT('Origin',(2.93915231795E-16,-20.7742356128,0.729452270839));
#94061=CARTESIAN_POINT('Origin',(-2.45,-20.6742356128,10.7304528845));
#94062=CARTESIAN_POINT('Origin',(-0.75,-23.1742356128,-8.70195642562));
#94063=CARTESIAN_POINT('',(-0.75,-21.0742356128,-4.99584562937));
#94064=CARTESIAN_POINT('',(-0.75,-22.1242356128,-4.99584562937));
#94065=CARTESIAN_POINT('',(-0.75,-21.0742356128,-6.2343884565225));
#94066=CARTESIAN_POINT('',(-0.75,-21.0742356128,-6.03615517446));
#94067=CARTESIAN_POINT('',(-0.75,-22.1242356128,-6.23438845923));
#94068=CARTESIAN_POINT('Origin',(2.32682891838E-16,-21.2742356128,0.729452270839));
#94069=CARTESIAN_POINT('',(-0.992653804111,-22.1242356128,5.82664824081));
#94070=CARTESIAN_POINT('',(-1.19254592572,-22.1242356128,5.7836191207));
#94071=CARTESIAN_POINT('Origin',(-1.05,-22.1242356128,6.12111625914));
#94072=CARTESIAN_POINT('',(-0.75,-21.0742356128,6.12111625914));
#94073=CARTESIAN_POINT('',(-0.75,-21.9742356128,6.12111625914));
#94074=CARTESIAN_POINT('Origin',(-1.05,-21.0742356128,6.12111625914));
#94075=CARTESIAN_POINT('Origin',(-0.75,-23.1742356128,-8.70195642562));
#94076=CARTESIAN_POINT('',(-0.75,-21.0742356128,9.0358656718));
#94077=CARTESIAN_POINT('',(-0.75,-22.1242356128,9.0358656718));
#94078=CARTESIAN_POINT('',(-0.75,-21.0742356128,7.56406439184));
#94079=CARTESIAN_POINT('Origin',(-1.05,-22.1242356128,9.0358656718));
#94080=CARTESIAN_POINT('',(-1.10198928897,-21.0742356128,9.33132652171));
#94081=CARTESIAN_POINT('',(-1.10198928897,-21.2742356128,9.33132652171));
#94082=CARTESIAN_POINT('Origin',(-1.05,-21.0742356128,9.0358656718));
#94083=CARTESIAN_POINT('Origin',(-0.00234331738835,-21.2742356128,3.08191746407));
#94084=CARTESIAN_POINT('',(-3.58772315463,-22.1242356128,8.31731489457));
#94085=CARTESIAN_POINT('Origin',(-0.00234331738835,-21.0742356128,3.08191746407));
#94086=CARTESIAN_POINT('Origin',(-1.2614400074,-22.1242356128,6.07560132137));
#94087=CARTESIAN_POINT('',(-1.46510738459,-21.9742356128,5.8553296721));
#94088=CARTESIAN_POINT('Origin',(-3.41821282746,-22.1242356128,8.06979469543));
#94089=CARTESIAN_POINT('',(-3.62188020465,-21.9742356128,7.84952304616));
#94090=CARTESIAN_POINT('Origin',(-3.88971125292,-23.1742356128,8.09716475273));
#94091=CARTESIAN_POINT('Origin',(-0.00234331738835,-21.2742356128,3.08191746407));
#94092=CARTESIAN_POINT('',(-5.76218263052,-22.1242356128,0.419477620705));
#94093=CARTESIAN_POINT('',(-6.21380646358,-22.1242356128,1.78497474518));
#94094=CARTESIAN_POINT('Origin',(-5.48986775992,-22.1242356128,0.545353000555));
#94095=CARTESIAN_POINT('',(-5.1900363009,-21.9742356128,0.55540766038));
#94096=CARTESIAN_POINT('Origin',(2.32682891838E-16,-21.2742356128,0.729452270839));
#94097=CARTESIAN_POINT('',(-5.08448267152,-22.1242356128,1.78529520144));
#94098=CARTESIAN_POINT('Origin',(-5.92013962829,-22.1242356128,1.84629187045));
#94099=CARTESIAN_POINT('',(-5.92013962829,-21.9742356128,2.14629187045));
#94100=CARTESIAN_POINT('Origin',(-5.3782162351,-22.1242356128,1.84629187045));
#94101=CARTESIAN_POINT('',(-5.3782162351,-21.9742356128,2.14629187045));
#94102=CARTESIAN_POINT('Origin',(-11.4443506127,-23.1742356128,2.14629187045));
#94103=CARTESIAN_POINT('Origin',(2.32682891838E-16,-21.2742356128,0.729452270839));
#94104=CARTESIAN_POINT('',(-3.13117783752,-22.1242356128,4.87221628548));
#94105=CARTESIAN_POINT('',(-4.2092958712,-22.1242356128,3.77060280966));
#94106=CARTESIAN_POINT('Origin',(-3.31206782846,-22.1242356128,5.11154620667));
#94107=CARTESIAN_POINT('',(-3.10840045127,-21.9742356128,5.33181785593));
#94108=CARTESIAN_POINT('Origin',(-9.80058174751,-23.1742356128,11.519536597));
#94109=CARTESIAN_POINT('',(-4.71627105755,-22.1242356128,6.81848575139));
#94110=CARTESIAN_POINT('Origin',(-4.91993843473,-22.1242356128,6.59821410213));
#94111=CARTESIAN_POINT('',(-5.16397092918,-21.0742356128,6.77270806092));
#94112=CARTESIAN_POINT('',(-5.16397092918,-21.2742356128,6.77270806092));
#94113=CARTESIAN_POINT('Origin',(-4.91993843473,-21.0742356128,6.59821410213));
#94114=CARTESIAN_POINT('Origin',(-0.00234331738835,-21.2742356128,3.08191746407));
#94115=CARTESIAN_POINT('',(-6.28256615006,-21.0742356128,3.98918589435));
#94116=CARTESIAN_POINT('',(-6.28256615006,-22.1242356128,3.98918589435));
#94117=CARTESIAN_POINT('Origin',(-0.00234331738835,-21.0742356128,3.08191746407));
#94118=CARTESIAN_POINT('Origin',(-4.452469377,-22.1242356128,3.94629187045));
#94119=CARTESIAN_POINT('',(-4.452469377,-21.0742356128,3.64629187045));
#94120=CARTESIAN_POINT('Origin',(-4.452469377,-21.0742356128,3.94629187045));
#94121=CARTESIAN_POINT('',(-4.452469377,-21.9742356128,3.64629187045));
#94122=CARTESIAN_POINT('Origin',(-5.98564848014,-22.1242356128,3.94629187045));
#94123=CARTESIAN_POINT('',(-5.98564848014,-21.0742356128,3.64629187045));
#94124=CARTESIAN_POINT('',(-5.98564848014,-21.9742356128,3.64629187045));
#94125=CARTESIAN_POINT('Origin',(-5.98564848014,-21.0742356128,3.94629187045));
#94126=CARTESIAN_POINT('Origin',(-11.7190551593,-23.1742356128,3.64629187045));
#94127=CARTESIAN_POINT('',(-4.57919858809,-21.0742356128,3.64629187045));
#94128=CARTESIAN_POINT('Origin',(-4.91993843473,-21.0742356128,6.59821410213));
#94129=CARTESIAN_POINT('Origin',(-4.91993843473,-21.0742356128,6.59821410213));
#94130=CARTESIAN_POINT('Origin',(-0.00234331738835,-21.0742356128,3.08191746407));
#94131=CARTESIAN_POINT('',(-5.98564848014,-20.7742356128,3.94629187045));
#94132=CARTESIAN_POINT('Ctrl Pts',(-5.98564848014,-20.7742356128,3.94629187045));
#94133=CARTESIAN_POINT('Ctrl Pts',(-5.99753462039329,-20.7742356128,3.94800899420363));
#94134=CARTESIAN_POINT('Ctrl Pts',(-6.00894948786785,-20.7749568618164,
3.94963477641195));
#94135=CARTESIAN_POINT('Ctrl Pts',(-6.01980989987418,-20.7762266979977,
3.95115850173577));
#94136=CARTESIAN_POINT('Ctrl Pts',(-6.03099450509648,-20.7775344399486,
3.95272771165195));
#94137=CARTESIAN_POINT('Ctrl Pts',(-6.04159134724835,-20.7794231116068,
3.95418902876826));
#94138=CARTESIAN_POINT('Ctrl Pts',(-6.05155400424851,-20.7817112682625,
3.9555638575554));
#94139=CARTESIAN_POINT('Ctrl Pts',(-6.06195399546318,-20.7840998689256,
3.95699903767931));
#94140=CARTESIAN_POINT('Ctrl Pts',(-6.07166333777175,-20.7869229649579,
3.95834038822613));
#94141=CARTESIAN_POINT('Ctrl Pts',(-6.08067142144271,-20.789995541024,3.95964186007419));
#94142=CARTESIAN_POINT('Ctrl Pts',(-6.08133300126666,-20.790221199933,3.95973744394614));
#94143=CARTESIAN_POINT('Ctrl Pts',(-6.08199081474964,-20.790448216819,3.95983282365959));
#94144=CARTESIAN_POINT('Ctrl Pts',(-6.08264486504496,-20.7906765244433,
3.95992802554191));
#94145=CARTESIAN_POINT('Ctrl Pts',(-6.09230022220808,-20.7940468946914,
3.96133343454936));
#94146=CARTESIAN_POINT('Ctrl Pts',(-6.10113662242138,-20.7976945475709,
3.96265857234215));
#94147=CARTESIAN_POINT('Ctrl Pts',(-6.10919527072438,-20.8014229304912,
3.96388251875472));
#94148=CARTESIAN_POINT('Ctrl Pts',(-6.11214308238635,-20.8027867535841,
3.96433023199061));
#94149=CARTESIAN_POINT('Ctrl Pts',(-6.11498709011435,-20.8041617700191,
3.9647646361173));
#94150=CARTESIAN_POINT('Ctrl Pts',(-6.11773006477687,-20.8055397069305,
3.96518539232357));
#94151=CARTESIAN_POINT('Ctrl Pts',(-6.12285088731743,-20.8081121588352,
3.96597089643143));
#94152=CARTESIAN_POINT('Ctrl Pts',(-6.12761988753479,-20.8106943410743,
3.96670660222514));
#94153=CARTESIAN_POINT('Ctrl Pts',(-6.13205927382818,-20.813239401917,3.96738351325775));
#94154=CARTESIAN_POINT('Ctrl Pts',(-6.13427896697488,-20.8145119323384,
3.96772196877405));
#94155=CARTESIAN_POINT('Ctrl Pts',(-6.1360941609467,-20.8155850054129,3.96799380562841));
#94156=CARTESIAN_POINT('Ctrl Pts',(-6.13799483590152,-20.8167338355379,
3.96827874364878));
#94157=CARTESIAN_POINT('Ctrl Pts',(-6.13974121001297,-20.8177894011852,
3.96854054979343));
#94158=CARTESIAN_POINT('Ctrl Pts',(-6.14155986098848,-20.8189091200391,
3.96881351450609));
#94159=CARTESIAN_POINT('Ctrl Pts',(-6.14380738476804,-20.8203385235072,
3.96913982299513));
#94160=CARTESIAN_POINT('Ctrl Pts',(-6.14400596467851,-20.8204648184169,
3.96916865397398));
#94161=CARTESIAN_POINT('Ctrl Pts',(-6.14420787354382,-20.8205935547799,
3.9691978853907));
#94162=CARTESIAN_POINT('Ctrl Pts',(-6.14441334507419,-20.820724916961,3.96922753607458));
#94163=CARTESIAN_POINT('Ctrl Pts',(-6.15508617823865,-20.8275482790126,
3.97076768522153));
#94164=CARTESIAN_POINT('Ctrl Pts',(-6.16499012109537,-20.834842585959,3.97218466576068));
#94165=CARTESIAN_POINT('Ctrl Pts',(-6.17413375640074,-20.8424304525795,
3.97348871453297));
#94166=CARTESIAN_POINT('Ctrl Pts',(-6.1823369609858,-20.8492379006211,3.97465864077245));
#94167=CARTESIAN_POINT('Ctrl Pts',(-6.18992916790955,-20.8562816337656,
3.97573831638601));
#94168=CARTESIAN_POINT('Ctrl Pts',(-6.19693925316656,-20.8634552142654,
3.97675221889574));
#94169=CARTESIAN_POINT('Ctrl Pts',(-6.20435116306778,-20.8710399911097,
3.97782423924575));
#94170=CARTESIAN_POINT('Ctrl Pts',(-6.21111336229814,-20.8787689847565,
3.978813861966));
#94171=CARTESIAN_POINT('Ctrl Pts',(-6.21728147452881,-20.8865425448021,
3.97972042315571));
#94172=CARTESIAN_POINT('Ctrl Pts',(-6.21977879971208,-20.8896898784658,
3.98008746869649));
#94173=CARTESIAN_POINT('Ctrl Pts',(-6.22230837615001,-20.8930158375082,
3.98047141698488));
#94174=CARTESIAN_POINT('Ctrl Pts',(-6.22470980772358,-20.8963114866291,
3.98082717094525));
#94175=CARTESIAN_POINT('Ctrl Pts',(-6.22724267464651,-20.8997875134873,
3.98120239606049));
#94176=CARTESIAN_POINT('Ctrl Pts',(-6.22963286905179,-20.9032293675739,
3.98154610338506));
#94177=CARTESIAN_POINT('Ctrl Pts',(-6.23173340912521,-20.9063721333557,
3.98184549185762));
#94178=CARTESIAN_POINT('Ctrl Pts',(-6.2325602073125,-20.9076091642909,3.98196333481122));
#94179=CARTESIAN_POINT('Ctrl Pts',(-6.23334256305448,-20.9087996933672,
3.98207473695029));
#94180=CARTESIAN_POINT('Ctrl Pts',(-6.23407297039883,-20.9099270947014,
3.98218035773893));
#94181=CARTESIAN_POINT('Ctrl Pts',(-6.24080352615489,-20.9203158696751,
3.98315363191598));
#94182=CARTESIAN_POINT('Ctrl Pts',(-6.24683001815921,-20.9310048591711,
3.98394041908957));
#94183=CARTESIAN_POINT('Ctrl Pts',(-6.25215756345662,-20.9419326633264,
3.98461729373962));
#94184=CARTESIAN_POINT('Ctrl Pts',(-6.2537092163496,-20.9451153972095,3.98481443415801));
#94185=CARTESIAN_POINT('Ctrl Pts',(-6.25520166000752,-20.9483187118516,
3.9850022549043));
#94186=CARTESIAN_POINT('Ctrl Pts',(-6.25663514487,-20.9515419369133,3.98518260759789));
#94187=CARTESIAN_POINT('Ctrl Pts',(-6.25875058534709,-20.956298555515,3.98544875996417));
#94188=CARTESIAN_POINT('Ctrl Pts',(-6.26080955526559,-20.9612759828185,
3.9857313059189));
#94189=CARTESIAN_POINT('Ctrl Pts',(-6.26272853899919,-20.9662974014104,
3.98599052917547));
#94190=CARTESIAN_POINT('Ctrl Pts',(-6.2646990064388,-20.9714535377876,3.98625670703708));
#94191=CARTESIAN_POINT('Ctrl Pts',(-6.26652172448506,-20.9766556017273,
3.98649806712921));
#94192=CARTESIAN_POINT('Ctrl Pts',(-6.2681448066767,-20.9817049057232,3.98671332194709));
#94193=CARTESIAN_POINT('Ctrl Pts',(-6.26968978634078,-20.9865112377941,
3.98691821872799));
#94194=CARTESIAN_POINT('Ctrl Pts',(-6.27105457364326,-20.9911787935128,
3.98710015778145));
#94195=CARTESIAN_POINT('Ctrl Pts',(-6.27222390388891,-20.9955360949015,
3.98729080196867));
#94196=CARTESIAN_POINT('Ctrl Pts',(-6.274855029626,-21.0053405174507,3.98771977302239));
#94197=CARTESIAN_POINT('Ctrl Pts',(-6.27692564331862,-21.0150164297704,
3.98807174964736));
#94198=CARTESIAN_POINT('Ctrl Pts',(-6.27851136625063,-21.0246215233591,
3.98836052942438));
#94199=CARTESIAN_POINT('Ctrl Pts',(-6.28014978966751,-21.0345458360744,
3.98865890661213));
#94200=CARTESIAN_POINT('Ctrl Pts',(-6.2812705008667,-21.0443956961073,3.98888987925294));
#94201=CARTESIAN_POINT('Ctrl Pts',(-6.28191433142828,-21.0542422738849,
3.98903308895698));
#94202=CARTESIAN_POINT('Ctrl Pts',(-6.2823497481363,-21.0609014241911,3.98912994036729));
#94203=CARTESIAN_POINT('Ctrl Pts',(-6.28256615006486,-21.0675591942924,
3.9891858943507));
#94204=CARTESIAN_POINT('Ctrl Pts',(-6.28256615006486,-21.0742356128,3.9891858943507));
#94205=CARTESIAN_POINT('Origin',(-0.00234331738835,-20.7742356128,3.08191746407));
#94206=CARTESIAN_POINT('Origin',(-4.452469377,-21.0742356128,3.94629187045));
#94207=CARTESIAN_POINT('Origin',(-4.452469377,-21.0742356128,3.94629187045));
#94208=CARTESIAN_POINT('Origin',(-5.98564848014,-21.0742356128,3.94629187045));
#94209=CARTESIAN_POINT('Origin',(-5.98564848014,-21.0742356128,3.94629187045));
#94210=CARTESIAN_POINT('Origin',(-4.57919858809,-21.0742356128,3.94629187045));
#94211=CARTESIAN_POINT('',(-5.21905892857,-20.7742356128,3.94629187045));
#94212=CARTESIAN_POINT('Origin',(2.93915231795E-16,-20.7742356128,0.729452270839));
#94213=CARTESIAN_POINT('',(-1.05,-20.7742356128,9.0358656718));
#94214=CARTESIAN_POINT('Origin',(-0.00234331738835,-20.7742356128,3.08191746407));
#94215=CARTESIAN_POINT('',(-1.05,-20.7742356128,7.56406439184));
#94216=CARTESIAN_POINT('Origin',(-10.3267865236,-19.6742356128,-3.3434289261));
#94217=CARTESIAN_POINT('Origin',(-1.05,-21.0742356128,-4.99584562937));
#94218=CARTESIAN_POINT('',(-1.01141425905,-21.0742356128,-4.69833741));
#94219=CARTESIAN_POINT('',(-1.05,-20.7742356128,-4.99584562937));
#94220=CARTESIAN_POINT('Origin',(-1.05,-21.0742356128,-4.99584562937));
#94221=CARTESIAN_POINT('Origin',(-1.05,-21.0742356128,-4.99584562937));
#94222=CARTESIAN_POINT('Origin',(-1.05,-21.0742356128,-4.99584562937));
#94223=CARTESIAN_POINT('Origin',(2.93915231795E-16,-20.7742356128,0.729452270839));
#94224=CARTESIAN_POINT('Origin',(2.93915231795E-16,-20.7742356128,0.729452270839));
#94225=CARTESIAN_POINT('Origin',(-1.05,-22.1242356128,-4.99584562937));
#94226=CARTESIAN_POINT('',(-1.01141425905,-21.2742356128,-4.69833741));
#94227=CARTESIAN_POINT('Origin',(-11.0821857629,-20.8742356128,-2.71007990903));
#94228=CARTESIAN_POINT('Origin',(-11.0821857629,-22.0742356128,-2.71007990903));
#94229=CARTESIAN_POINT('Origin',(-1.05,-21.0742356128,6.12111625914));
#94230=CARTESIAN_POINT('Origin',(-1.05,-21.0742356128,6.12111625914));
#94231=CARTESIAN_POINT('Origin',(-0.00234331738835,-21.0742356128,3.08191746407));
#94232=CARTESIAN_POINT('Ctrl Pts',(-1.05,-20.7742356128,9.0358656718));
#94233=CARTESIAN_POINT('Ctrl Pts',(-1.0523959262998,-20.7742356127999,9.0494810158149));
#94234=CARTESIAN_POINT('Ctrl Pts',(-1.05479609358863,-20.7751955471885,
9.06312046382714));
#94235=CARTESIAN_POINT('Ctrl Pts',(-1.05716675141005,-20.7770995761648,
9.07659420488324));
#94236=CARTESIAN_POINT('Ctrl Pts',(-1.05765242878117,-20.777489655146,9.07935457421036));
#94237=CARTESIAN_POINT('Ctrl Pts',(-1.05813687069917,-20.7779191854724,
9.08210800638467));
#94238=CARTESIAN_POINT('Ctrl Pts',(-1.05861979407081,-20.778387763992,9.08485290999588));
#94239=CARTESIAN_POINT('Ctrl Pts',(-1.06123562797834,-20.7809258966483,
9.09972113207978));
#94240=CARTESIAN_POINT('Ctrl Pts',(-1.06382481858908,-20.7846312659766,
9.11444090215554));
#94241=CARTESIAN_POINT('Ctrl Pts',(-1.06635220403382,-20.7894619264883,
9.12879872839508));
#94242=CARTESIAN_POINT('Ctrl Pts',(-1.06656892432023,-20.7898761498636,
9.1300298948645));
#94243=CARTESIAN_POINT('Ctrl Pts',(-1.06678519130229,-20.7902986162517,
9.13125840625777));
#94244=CARTESIAN_POINT('Ctrl Pts',(-1.06700098355357,-20.7907292818386,
9.13248413206188));
#94245=CARTESIAN_POINT('Ctrl Pts',(-1.06973333853196,-20.7961823565126,
9.14800423523072));
#94246=CARTESIAN_POINT('Ctrl Pts',(-1.0723842253386,-20.8029406104611,9.16304733867516));
#94247=CARTESIAN_POINT('Ctrl Pts',(-1.07491156867559,-20.8109185406861,
9.17744085776139));
#94248=CARTESIAN_POINT('Ctrl Pts',(-1.07743891201258,-20.818896470911,9.19183437684762));
#94249=CARTESIAN_POINT('Ctrl Pts',(-1.0798437756864,-20.8281006365983,9.20558435730489));
#94250=CARTESIAN_POINT('Ctrl Pts',(-1.08213257646722,-20.8383966814998,
9.21847863961296));
#94251=CARTESIAN_POINT('Ctrl Pts',(-1.08442137724805,-20.8486927264013,
9.23137292192103));
#94252=CARTESIAN_POINT('Ctrl Pts',(-1.08659398041548,-20.8600780828836,
9.24341074044898));
#94253=CARTESIAN_POINT('Ctrl Pts',(-1.08846412215442,-20.8724030816455,
9.25446151045095));
#94254=CARTESIAN_POINT('Ctrl Pts',(-1.09033426389336,-20.8847280804074,
9.26551228045291));
#94255=CARTESIAN_POINT('Ctrl Pts',(-1.09190173768304,-20.8979944937689,
9.27557482824863));
#94256=CARTESIAN_POINT('Ctrl Pts',(-1.09373094217068,-20.9119964096905,
9.28439342814165));
#94257=CARTESIAN_POINT('Ctrl Pts',(-1.09481843980888,-20.920320820984,9.28963625726252));
#94258=CARTESIAN_POINT('Ctrl Pts',(-1.09599868490452,-20.9289044572172,
9.29444075987992));
#94259=CARTESIAN_POINT('Ctrl Pts',(-1.0969443005408,-20.9377134971514,9.29884544678996));
#94260=CARTESIAN_POINT('Ctrl Pts',(-1.09780280437058,-20.9457110325453,
9.30284436605073));
#94261=CARTESIAN_POINT('Ctrl Pts',(-1.09846784732843,-20.9538940657016,
9.30651334732055));
#94262=CARTESIAN_POINT('Ctrl Pts',(-1.09896829273513,-20.962228930443,9.30983126609625));
#94263=CARTESIAN_POINT('Ctrl Pts',(-1.09986705170843,-20.9771976650487,
9.31578997654175));
#94264=CARTESIAN_POINT('Ctrl Pts',(-1.1002349936443,-20.9926630556998,9.32061678088581));
#94265=CARTESIAN_POINT('Ctrl Pts',(-1.10081734141703,-21.0084193812886,
9.32411179976513));
#94266=CARTESIAN_POINT('Ctrl Pts',(-1.10121648140339,-21.019218735,9.32650727864078));
#94267=CARTESIAN_POINT('Ctrl Pts',(-1.10171607543104,-21.0301449616615,
9.32827562220263));
#94268=CARTESIAN_POINT('Ctrl Pts',(-1.10194569498976,-21.0411252195446,
9.32947326775938));
#94269=CARTESIAN_POINT('Ctrl Pts',(-1.10217531916459,-21.0521056981675,
9.33067093739279));
#94270=CARTESIAN_POINT('Ctrl Pts',(-1.10213545468708,-21.0631759320558,
9.33130080239825));
#94271=CARTESIAN_POINT('Ctrl Pts',(-1.10198928897115,-21.0742356128,9.33132652171654));
#94272=CARTESIAN_POINT('Origin',(-0.45,-22.1242356128,-6.23438845923));
#94273=CARTESIAN_POINT('Origin',(-0.45,-21.0742356128,-6.23438845923));
#94274=CARTESIAN_POINT('Ctrl Pts',(-0.530881089940139,-21.0742435944873,
-6.52327990521127));
#94275=CARTESIAN_POINT('Ctrl Pts',(-0.605869334571474,-21.074241803815,
-6.50228543550801));
#94276=CARTESIAN_POINT('Ctrl Pts',(-0.674045596111476,-21.0742407617281,
-6.45695987785349));
#94277=CARTESIAN_POINT('Ctrl Pts',(-0.724740690411004,-21.0742407618033,
-6.390119097022));
#94278=CARTESIAN_POINT('Ctrl Pts',(-0.750003689199869,-21.0742418040299,
-6.31224618327166));
#94279=CARTESIAN_POINT('Ctrl Pts',(-0.750000029081184,-21.0742435948102,
-6.23437446321454));
#94280=CARTESIAN_POINT('Ctrl Pts',(-0.529863965484531,-20.9334730733702,
-6.5229624048105));
#94281=CARTESIAN_POINT('Ctrl Pts',(-0.604729632930939,-20.9650040286309,
-6.5017257304758));
#94282=CARTESIAN_POINT('Ctrl Pts',(-0.672745476661423,-20.9833541286166,
-6.45604164489109));
#94283=CARTESIAN_POINT('Ctrl Pts',(-0.723524938742467,-20.9833528049852,
-6.38909475830119));
#94284=CARTESIAN_POINT('Ctrl Pts',(-0.749174751443758,-20.9650002442128,
-6.31129794540516));
#94285=CARTESIAN_POINT('Ctrl Pts',(-0.749435926165564,-20.9334673875941,
-6.23350231178913));
#94286=CARTESIAN_POINT('Ctrl Pts',(-0.68296904973928,-20.8341940751783,
-6.57017290017678));
#94287=CARTESIAN_POINT('Ctrl Pts',(-0.709063502037876,-20.8613416651734,
-6.52452364681565));
#94288=CARTESIAN_POINT('Ctrl Pts',(-0.735145295108947,-20.874961887123,
-6.4799295145159));
#94289=CARTESIAN_POINT('Ctrl Pts',(-0.764898754103171,-20.8749609046628,
-6.43990412638473));
#94290=CARTESIAN_POINT('Ctrl Pts',(-0.799929343938473,-20.8613387211769,
-6.40244473945582));
#94291=CARTESIAN_POINT('Ctrl Pts',(-0.835971167587679,-20.8341891797982,
-6.36498507291063));
#94292=CARTESIAN_POINT('Ctrl Pts',(-0.784928027206935,-20.8055941305548,
-6.60113592908881));
#94293=CARTESIAN_POINT('Ctrl Pts',(-0.811295647961892,-20.8073540418052,
-6.57624029892075));
#94294=CARTESIAN_POINT('Ctrl Pts',(-0.837074174388714,-20.8079529197238,
-6.54898974260409));
#94295=CARTESIAN_POINT('Ctrl Pts',(-0.85992459713757,-20.8079528765283,
-6.51819337189669));
#94296=CARTESIAN_POINT('Ctrl Pts',(-0.878603960261464,-20.8073538919411,
-6.48545637104955));
#94297=CARTESIAN_POINT('Ctrl Pts',(-0.89485605580427,-20.8055938131957,
-6.45271958057142));
#94298=CARTESIAN_POINT('Ctrl Pts',(-0.922335918992876,-20.7721966680782,
-6.64273052609052));
#94299=CARTESIAN_POINT('Ctrl Pts',(-0.931743355474937,-20.7721716130412,
-6.62722231169815));
#94300=CARTESIAN_POINT('Ctrl Pts',(-0.941283625175912,-20.7721536510732,
-6.61227372299854));
#94301=CARTESIAN_POINT('Ctrl Pts',(-0.951544288548907,-20.7721534830166,
-6.59819859894796));
#94302=CARTESIAN_POINT('Ctrl Pts',(-0.962831436656691,-20.7721713423069,
-6.58460198829503));
#94303=CARTESIAN_POINT('Ctrl Pts',(-0.97469324757036,-20.7721966726456,
-6.57099919715921));
#94304=CARTESIAN_POINT('Ctrl Pts',(-1.05,-20.7742356128,-6.68100624476));
#94305=CARTESIAN_POINT('Ctrl Pts',(-1.05,-20.7742356128,-6.68100624476));
#94306=CARTESIAN_POINT('Ctrl Pts',(-1.05,-20.7742356128,-6.68100624476));
#94307=CARTESIAN_POINT('Ctrl Pts',(-1.05,-20.7742356128,-6.68100624476));
#94308=CARTESIAN_POINT('Ctrl Pts',(-1.05,-20.7742356128,-6.68100624476));
#94309=CARTESIAN_POINT('Ctrl Pts',(-1.05,-20.7742356128,-6.68100624476));
#94310=CARTESIAN_POINT('Ctrl Pts',(-1.05,-20.7742356128,-6.68100624476));
#94311=CARTESIAN_POINT('Ctrl Pts',(-1.00503272302771,-20.7742356128,-6.61525813211032));
#94312=CARTESIAN_POINT('Ctrl Pts',(-0.966555030638054,-20.784200008547,
-6.55977739297378));
#94313=CARTESIAN_POINT('Ctrl Pts',(-0.920872678369823,-20.8029478256253,
-6.49195734453869));
#94314=CARTESIAN_POINT('Ctrl Pts',(-0.907564542264599,-20.8098627882809,
-6.47191750510528));
#94315=CARTESIAN_POINT('Ctrl Pts',(-0.89025216397347,-20.8202162407514,
-6.44570801102259));
#94316=CARTESIAN_POINT('Ctrl Pts',(-0.882255155685331,-20.8253927093966,
-6.4335658302481));
#94317=CARTESIAN_POINT('Ctrl Pts',(-0.874005385604677,-20.8312552684653,
-6.42108444364487));
#94318=CARTESIAN_POINT('Ctrl Pts',(-0.870692640879228,-20.8337138929026,
-6.41609624030784));
#94319=CARTESIAN_POINT('Ctrl Pts',(-0.868532729530181,-20.8353392827204,
-6.41285098527206));
#94320=CARTESIAN_POINT('Ctrl Pts',(-0.868536031383549,-20.835325974443,
-6.41285141739827));
#94321=CARTESIAN_POINT('Ctrl Pts',(-0.84971875761109,-20.84988186283,-6.38472311999057));
#94322=CARTESIAN_POINT('Ctrl Pts',(-0.834869826129459,-20.8642005359298,
-6.36250843958396));
#94323=CARTESIAN_POINT('Ctrl Pts',(-0.815482968411093,-20.8868838228403,
-6.33336879490777));
#94324=CARTESIAN_POINT('Ctrl Pts',(-0.806507337791894,-20.898528185668,
-6.31984456655309));
#94325=CARTESIAN_POINT('Ctrl Pts',(-0.797271494820506,-20.9124718813195,
-6.3058960896103));
#94326=CARTESIAN_POINT('Ctrl Pts',(-0.793573962211397,-20.9185076218975,
-6.30031026866431));
#94327=CARTESIAN_POINT('Ctrl Pts',(-0.791166377172266,-20.9225429112605,
-6.29667352086561));
#94328=CARTESIAN_POINT('Ctrl Pts',(-0.790466771165988,-20.9237252585396,
-6.29561659938596));
#94329=CARTESIAN_POINT('Ctrl Pts',(-0.762891354789432,-20.9725020900793,
-6.25398143917688));
#94330=CARTESIAN_POINT('Ctrl Pts',(-0.75,-21.0240629896735,-6.23438843361193));
#94331=CARTESIAN_POINT('Ctrl Pts',(-0.75,-21.0742356128,-6.23438845562));
#94332=CARTESIAN_POINT('Origin',(-1.05,-21.0742356128,7.56406439184));
#94333=CARTESIAN_POINT('Ctrl Pts',(-1.05,-20.7742356128,9.0358656718));
#94334=CARTESIAN_POINT('Ctrl Pts',(-1.03689721887064,-20.7742356128,9.0358656718));
#94335=CARTESIAN_POINT('Ctrl Pts',(-1.02436620890084,-20.7750936657409,
9.03591396069315));
#94336=CARTESIAN_POINT('Ctrl Pts',(-1.01250197740514,-20.776588361968,9.03597690865791));
#94337=CARTESIAN_POINT('Ctrl Pts',(-0.999990657744915,-20.7781645805625,
9.03604328987352));
#94338=CARTESIAN_POINT('Ctrl Pts',(-0.988220470098179,-20.780447884538,
9.03612571051123));
#94339=CARTESIAN_POINT('Ctrl Pts',(-0.9772443658479,-20.783191773756,9.03618418968654));
#94340=CARTESIAN_POINT('Ctrl Pts',(-0.967775256719244,-20.785558932982,
9.03623463979891));
#94341=CARTESIAN_POINT('Ctrl Pts',(-0.958895821169001,-20.7882689318648,
9.03626719339298));
#94342=CARTESIAN_POINT('Ctrl Pts',(-0.950612352771678,-20.7911774179081,
9.03625795098188));
#94343=CARTESIAN_POINT('Ctrl Pts',(-0.940691041670133,-20.7946609822179,
9.03624688112183));
#94344=CARTESIAN_POINT('Ctrl Pts',(-0.931618460909888,-20.7984298272103,
9.03619870448758));
#94345=CARTESIAN_POINT('Ctrl Pts',(-0.923353302993488,-20.8022787377616,
9.03613447787256));
#94346=CARTESIAN_POINT('Ctrl Pts',(-0.920375997747112,-20.8036652063196,
9.03611134192769));
#94347=CARTESIAN_POINT('Ctrl Pts',(-0.917503214531104,-20.8050624512225,
9.03608633983968));
#94348=CARTESIAN_POINT('Ctrl Pts',(-0.914732311286345,-20.8064621746117,
9.03606109662758));
#94349=CARTESIAN_POINT('Ctrl Pts',(-0.909500772179841,-20.8091048896405,
9.03601343677098));
#94350=CARTESIAN_POINT('Ctrl Pts',(-0.904632123230069,-20.8117561091739,
9.03596471449331));
#94351=CARTESIAN_POINT('Ctrl Pts',(-0.900104656732014,-20.8143676035612,
9.035927646362));
#94352=CARTESIAN_POINT('Ctrl Pts',(-0.897840923482987,-20.8156733507549,
9.03590911229635));
#94353=CARTESIAN_POINT('Ctrl Pts',(-0.895976722356037,-20.8167827050556,
9.03589341635984));
#94354=CARTESIAN_POINT('Ctrl Pts',(-0.89403431412729,-20.8179648486727,
9.03588251977217));
#94355=CARTESIAN_POINT('Ctrl Pts',(-0.892198750878441,-20.8190819667667,
9.0358722225671));
#94356=CARTESIAN_POINT('Ctrl Pts',(-0.890293122601369,-20.8202640633863,
9.03586615670055));
#94357=CARTESIAN_POINT('Ctrl Pts',(-0.887937645634305,-20.8217761243718,
9.03586587241935));
#94358=CARTESIAN_POINT('Ctrl Pts',(-0.887800537371023,-20.8218641388414,
9.03586585587183));
#94359=CARTESIAN_POINT('Ctrl Pts',(-0.887661913346612,-20.8219532839679,
9.03586585902197));
#94360=CARTESIAN_POINT('Ctrl Pts',(-0.88752170207832,-20.8220436170816,
9.03586588222689));
#94361=CARTESIAN_POINT('Ctrl Pts',(-0.875790229627156,-20.8296017858925,
9.03586782378187));
#94362=CARTESIAN_POINT('Ctrl Pts',(-0.865002652397592,-20.837709857829,
9.03588740175503));
#94363=CARTESIAN_POINT('Ctrl Pts',(-0.85513457659743,-20.8461403144017,
9.03590580540881));
#94364=CARTESIAN_POINT('Ctrl Pts',(-0.847849685717023,-20.8523639143666,
9.03591939150323));
#94365=CARTESIAN_POINT('Ctrl Pts',(-0.841064842089272,-20.8587638439859,
9.03593188650693));
#94366=CARTESIAN_POINT('Ctrl Pts',(-0.83475747530647,-20.865260371867,9.03593079134057));
#94367=CARTESIAN_POINT('Ctrl Pts',(-0.827331828577942,-20.8729087174712,
9.03592950200402));
#94368=CARTESIAN_POINT('Ctrl Pts',(-0.820566291017425,-20.8806916527784,
9.03591648427122));
#94369=CARTESIAN_POINT('Ctrl Pts',(-0.814403529620822,-20.8885091959321,
9.03590063301748));
#94370=CARTESIAN_POINT('Ctrl Pts',(-0.811809679859459,-20.8917995281612,
9.03589396137013));
#94371=CARTESIAN_POINT('Ctrl Pts',(-0.809174848559519,-20.8952906291691,
9.03588689130171));
#94372=CARTESIAN_POINT('Ctrl Pts',(-0.806688716921365,-20.8987374096837,
9.03588082404002));
#94373=CARTESIAN_POINT('Ctrl Pts',(-0.804046067395552,-20.902401187077,
9.03587437480541));
#94374=CARTESIAN_POINT('Ctrl Pts',(-0.801571639184609,-20.9060145063025,
9.03586906588609));
#94375=CARTESIAN_POINT('Ctrl Pts',(-0.799442290801424,-20.9092482364348,
9.03586681334286));
#94376=CARTESIAN_POINT('Ctrl Pts',(-0.798815366061185,-20.9102003142814,
9.03586615014697));
#94377=CARTESIAN_POINT('Ctrl Pts',(-0.798218038451281,-20.9111193010546,
9.03586575284659));
#94378=CARTESIAN_POINT('Ctrl Pts',(-0.797654124306548,-20.9119964097062,
9.03586567179813));
#94379=CARTESIAN_POINT('Ctrl Pts',(-0.790082400390862,-20.9237734233107,
9.03586458355345));
#94380=CARTESIAN_POINT('Ctrl Pts',(-0.783434264015833,-20.9359220630882,
9.0359759557514));
#94381=CARTESIAN_POINT('Ctrl Pts',(-0.777682618896556,-20.9483658587849,
9.03608697054653));
#94382=CARTESIAN_POINT('Ctrl Pts',(-0.776930171717263,-20.9499937928416,
9.03610149382948));
#94383=CARTESIAN_POINT('Ctrl Pts',(-0.776193089454086,-20.9516268154847,
9.03611595308919));
#94384=CARTESIAN_POINT('Ctrl Pts',(-0.775471332291151,-20.9532647869322,
9.0361300481624));
#94385=CARTESIAN_POINT('Ctrl Pts',(-0.773245359604993,-20.9583164578959,
9.03617351880543));
#94386=CARTESIAN_POINT('Ctrl Pts',(-0.771079574482088,-20.9636200439308,
9.03621337543365));
#94387=CARTESIAN_POINT('Ctrl Pts',(-0.769078220880423,-20.9689606816328,
9.03624367184624));
#94388=CARTESIAN_POINT('Ctrl Pts',(-0.767021713500409,-20.9744484978983,
9.03627480317457));
#94389=CARTESIAN_POINT('Ctrl Pts',(-0.765139169078809,-20.9799749931927,
9.03629581098497));
#94390=CARTESIAN_POINT('Ctrl Pts',(-0.763489899487749,-20.9852874610062,
9.03629994928468));
#94391=CARTESIAN_POINT('Ctrl Pts',(-0.762245712563468,-20.9892951156826,
9.03630307116263));
#94392=CARTESIAN_POINT('Ctrl Pts',(-0.761132979627602,-20.9931804778751,
9.03629658488695));
#94393=CARTESIAN_POINT('Ctrl Pts',(-0.760158087745634,-20.9968308572201,
9.03627763582184));
#94394=CARTESIAN_POINT('Ctrl Pts',(-0.757461543130412,-21.0069277827854,
9.03622522283076));
#94395=CARTESIAN_POINT('Ctrl Pts',(-0.755364431579379,-21.0168797090857,
9.03615294405315));
#94396=CARTESIAN_POINT('Ctrl Pts',(-0.753782303417459,-21.0267484683918,
9.03608326612259));
#94397=CARTESIAN_POINT('Ctrl Pts',(-0.752161163936008,-21.0368605665955,
9.03601187010871));
#94398=CARTESIAN_POINT('Ctrl Pts',(-0.751080542463713,-21.0468862667509,
9.03594335399294));
#94399=CARTESIAN_POINT('Ctrl Pts',(-0.750500652262316,-21.0569110834329,
9.0359029130572));
#94400=CARTESIAN_POINT('Ctrl Pts',(-0.750166935726296,-21.062680187807,
9.03587964001525));
#94401=CARTESIAN_POINT('Ctrl Pts',(-0.75,-21.0684492707566,9.0358656718));
#94402=CARTESIAN_POINT('Ctrl Pts',(-0.75,-21.0742356128,9.0358656718));
#94403=CARTESIAN_POINT('Origin',(-1.05,-21.0742356128,-6.03615517446));
#94404=CARTESIAN_POINT('',(-1.05,-20.7742356128,-5.83842593707));
#94405=CARTESIAN_POINT('Origin',(-1.05,-21.0742356128,9.0358656718));
#94406=CARTESIAN_POINT('Origin',(-11.0821857629,-22.0742356128,-2.71007990903));
#94407=CARTESIAN_POINT('Origin',(-2.45,-19.6742356128,10.7304528845));
#94408=CARTESIAN_POINT('Origin',(-4.57526812267,-21.0742356128,-3.65872047634));
#94409=CARTESIAN_POINT('',(-4.79320888776,-21.0742356128,-3.4525607739));
#94410=CARTESIAN_POINT('',(-4.57526812267,-20.7742356128,-3.65872047634));
#94411=CARTESIAN_POINT('Origin',(-4.57526812267,-21.0742356128,-3.65872047634));
#94412=CARTESIAN_POINT('',(-4.40684492179,-21.0742356128,-3.41045927235));
#94413=CARTESIAN_POINT('Origin',(-4.57526812267,-21.0742356128,-3.65872047634));
#94414=CARTESIAN_POINT('Origin',(-4.57526812267,-21.0742356128,-3.65872047634));
#94415=CARTESIAN_POINT('Origin',(-4.57526812267,-22.1242356128,-3.65872047634));
#94416=CARTESIAN_POINT('',(-4.79320888776,-21.9742356128,-3.4525607739));
#94417=CARTESIAN_POINT('',(-4.40684492179,-21.2742356128,-3.41045927235));
#94418=CARTESIAN_POINT('Origin',(-0.00234331738835,-21.2742356128,3.08191746407));
#94419=CARTESIAN_POINT('Origin',(-0.00234331738835,-21.0742356128,3.08191746407));
#94420=CARTESIAN_POINT('Origin',(-0.00234331738835,-21.0742356128,3.08191746407));
#94421=CARTESIAN_POINT('Origin',(-0.00234331738835,-20.7742356128,3.08191746407));
#94422=CARTESIAN_POINT('Origin',(-3.69394702409,-21.0742356128,-6.14889144395));
#94423=CARTESIAN_POINT('',(-3.69394702409,-20.7742356128,-7.0794205347));
#94424=CARTESIAN_POINT('',(-3.69394702409,-20.7742356128,-7.27665075431));
#94425=CARTESIAN_POINT('',(-3.69394702409,-20.7742356128,-7.17803564451));
#94426=CARTESIAN_POINT('Origin',(-3.69394702409,-21.0742356128,-7.27665075431));
#94427=CARTESIAN_POINT('Origin',(-3.69394702409,-21.0742356128,-7.0794205347));
#94428=CARTESIAN_POINT('Origin',(-3.09394702409,-21.0742356128,-7.0794205347));
#94429=CARTESIAN_POINT('',(-2.83839294143,-20.7742356128,-6.53656501909));
#94430=CARTESIAN_POINT('Origin',(-3.09394702409,-20.7742356128,-7.0794205347));
#94431=CARTESIAN_POINT('Origin',(-2.83839294143,-21.0742356128,-6.53656501909));
#94432=CARTESIAN_POINT('Origin',(2.84607155346,-21.0742356128,5.53854202767));
#94433=CARTESIAN_POINT('',(-2.48410064475,-20.7742356128,-6.69708673107));
#94434=CARTESIAN_POINT('Origin',(2.84607155346,-20.7742356128,5.53854202767));
#94435=CARTESIAN_POINT('Origin',(-2.48410064475,-21.0742356128,-6.69708673107));
#94436=CARTESIAN_POINT('Origin',(-2.72372695744,-21.0742356128,-7.24715875387));
#94437=CARTESIAN_POINT('',(-2.12372695744,-20.7742356128,-7.24715875387));
#94438=CARTESIAN_POINT('Origin',(-2.72372695744,-20.7742356128,-7.24715875387));
#94439=CARTESIAN_POINT('Origin',(-2.12372695744,-21.0742356128,-7.24715875387));
#94440=CARTESIAN_POINT('Origin',(-2.12372695744,-21.0742356128,-6.11170048962));
#94441=CARTESIAN_POINT('',(-2.12372695744,-20.7742356128,-7.96338790087));
#94442=CARTESIAN_POINT('',(-2.12372695744,-20.7742356128,-7.60527332737));
#94443=CARTESIAN_POINT('Origin',(-2.12372695744,-21.0742356128,-7.96338790087));
#94444=CARTESIAN_POINT('Origin',(2.93915231795E-16,-20.7742356128,0.729452270839));
#94445=CARTESIAN_POINT('Origin',(2.84607155346,-20.7742356128,5.53854202767));
#94446=CARTESIAN_POINT('',(-6.34552156645,-20.7742356128,-5.5301356238));
#94447=CARTESIAN_POINT('',(-5.6152263525,-20.7742356128,-4.75810745444));
#94448=CARTESIAN_POINT('Origin',(2.84607155346,-20.7742356128,5.53854202767));
#94449=CARTESIAN_POINT('Origin',(-3.69394702409,-21.0742356128,-7.27665075431));
#94450=CARTESIAN_POINT('',(-3.83031550589,-21.0742356128,-7.54386534443));
#94451=CARTESIAN_POINT('Origin',(-3.69394702409,-21.0742356128,-7.27665075431));
#94452=CARTESIAN_POINT('Origin',(-3.69394702409,-21.0742356128,-7.27665075431));
#94453=CARTESIAN_POINT('',(-3.69394702409,-20.7869530199367,-7.36307246360657));
#94454=CARTESIAN_POINT('Origin',(-3.69394702409,-21.0742356128,-7.27665075431));
#94455=CARTESIAN_POINT('Origin',(2.84607155346,-21.0742356128,5.53854202767));
#94456=CARTESIAN_POINT('',(-6.53717906469,-21.0742356128,-5.76093294477));
#94457=CARTESIAN_POINT('Ctrl Pts',(-6.34552156645,-20.7742356128,-5.5301356238));
#94458=CARTESIAN_POINT('Ctrl Pts',(-6.35462138301445,-20.7742356127979,
-5.54109378251365));
#94459=CARTESIAN_POINT('Ctrl Pts',(-6.36368064291087,-20.7752517639833,
-5.55208549333866));
#94460=CARTESIAN_POINT('Ctrl Pts',(-6.37260695645825,-20.777273789321,-5.56300022566799));
#94461=CARTESIAN_POINT('Ctrl Pts',(-6.37610580132191,-20.7780663620813,
-5.56727847053874));
#94462=CARTESIAN_POINT('Ctrl Pts',(-6.37970394101495,-20.7790449225188,
-5.5716935505611));
#94463=CARTESIAN_POINT('Ctrl Pts',(-6.38325357036565,-20.7801826608097,
-5.57606224502158));
#94464=CARTESIAN_POINT('Ctrl Pts',(-6.38688094104391,-20.7813453169938,
-5.58052661936114));
#94465=CARTESIAN_POINT('Ctrl Pts',(-6.39045731242105,-20.7826741723983,
-5.58494214445669));
#94466=CARTESIAN_POINT('Ctrl Pts',(-6.39383252904759,-20.7840858569653,
-5.58912237105533));
#94467=CARTESIAN_POINT('Ctrl Pts',(-6.39558079613565,-20.7848170697852,
-5.59128761062115));
#94468=CARTESIAN_POINT('Ctrl Pts',(-6.3972752542099,-20.7855696092156,-5.5933899123615));
#94469=CARTESIAN_POINT('Ctrl Pts',(-6.39889617916021,-20.7863267818342,
-5.59540473642287));
#94470=CARTESIAN_POINT('Ctrl Pts',(-6.4067087739043,-20.7899762307613,-5.6051158608454));
#94471=CARTESIAN_POINT('Ctrl Pts',(-6.41448410644142,-20.7944359352525,
-5.61454942787996));
#94472=CARTESIAN_POINT('Ctrl Pts',(-6.42215737836493,-20.7996683893748,
-5.62362561625228));
#94473=CARTESIAN_POINT('Ctrl Pts',(-6.42599401432668,-20.8022846164359,
-5.62816371043844));
#94474=CARTESIAN_POINT('Ctrl Pts',(-6.42980518073347,-20.8050938211416,
-5.63261251725625));
#94475=CARTESIAN_POINT('Ctrl Pts',(-6.43358309418349,-20.8080900855734,
-5.63696245862029));
#94476=CARTESIAN_POINT('Ctrl Pts',(-6.4354720509085,-20.8095882177892,-5.63913742930231));
#94477=CARTESIAN_POINT('Ctrl Pts',(-6.43735269856414,-20.8111331027077,
-5.64128768864255));
#94478=CARTESIAN_POINT('Ctrl Pts',(-6.4392240870303,-20.8127239260744,-5.64341206858515));
#94479=CARTESIAN_POINT('Ctrl Pts',(-6.44015978126338,-20.8135193377577,
-5.64447425855645));
#94480=CARTESIAN_POINT('Ctrl Pts',(-6.44109316094471,-20.8143262332724,
-5.64552997897415));
#94481=CARTESIAN_POINT('Ctrl Pts',(-6.44202410895548,-20.8151445063426,
-5.64657908588352));
#94482=CARTESIAN_POINT('Ctrl Pts',(-6.44261778414038,-20.8156663275514,
-5.64724811222139));
#94483=CARTESIAN_POINT('Ctrl Pts',(-6.44354427447535,-20.8164900898511,
-5.6482879742904));
#94484=CARTESIAN_POINT('Ctrl Pts',(-6.44416414274481,-20.8170490495453,
-5.64898306931919));
#94485=CARTESIAN_POINT('Ctrl Pts',(-6.44451629612468,-20.8173666001529,
-5.6493779597754));
#94486=CARTESIAN_POINT('Ctrl Pts',(-6.44476996974886,-20.8175974114304,
-5.64966216020775));
#94487=CARTESIAN_POINT('Ctrl Pts',(-6.44480954196002,-20.8176333489548,
-5.64970642349396));
#94488=CARTESIAN_POINT('Ctrl Pts',(-6.44518816390414,-20.817977194673,-5.65012992905467));
#94489=CARTESIAN_POINT('Ctrl Pts',(-6.44607338207147,-20.8188020664663,
-5.65117043428081));
#94490=CARTESIAN_POINT('Ctrl Pts',(-6.44745013086571,-20.8201458282837,
-5.65280979040693));
#94491=CARTESIAN_POINT('Ctrl Pts',(-6.4488238952052,-20.8214866771541,-5.65444559280981));
#94492=CARTESIAN_POINT('Ctrl Pts',(-6.45068728558032,-20.8233444260723,
-5.65667792254751));
#94493=CARTESIAN_POINT('Ctrl Pts',(-6.45300569216522,-20.8257983946515,
-5.65946510923294));
#94494=CARTESIAN_POINT('Ctrl Pts',(-6.45372613691793,-20.8265609652885,
-5.66033122738298));
#94495=CARTESIAN_POINT('Ctrl Pts',(-6.45449036269108,-20.8273813968179,
-5.66125073558712));
#94496=CARTESIAN_POINT('Ctrl Pts',(-6.45529687830475,-20.8282628146959,
-5.66222183861902));
#94497=CARTESIAN_POINT('Ctrl Pts',(-6.45785966141141,-20.8310636071537,
-5.66530761452068));
#94498=CARTESIAN_POINT('Ctrl Pts',(-6.46085151790742,-20.8344780402339,
-5.66891683889509));
#94499=CARTESIAN_POINT('Ctrl Pts',(-6.46420753902736,-20.8386266302964,
-5.67297137007079));
#94500=CARTESIAN_POINT('Ctrl Pts',(-6.46478199801265,-20.8393367553977,
-5.67366539486438));
#94501=CARTESIAN_POINT('Ctrl Pts',(-6.46536705973206,-20.8400684559734,
-5.6743723861403));
#94502=CARTESIAN_POINT('Ctrl Pts',(-6.46596231189143,-20.8408224112228,
-5.67509184754763));
#94503=CARTESIAN_POINT('Ctrl Pts',(-6.46799868596679,-20.8434017129518,
-5.67755314489032));
#94504=CARTESIAN_POINT('Ctrl Pts',(-6.47015463099074,-20.8462413196276,
-5.68016075620037));
#94505=CARTESIAN_POINT('Ctrl Pts',(-6.47241108890313,-20.8493698313455,
-5.6828917376211));
#94506=CARTESIAN_POINT('Ctrl Pts',(-6.47353931785933,-20.8509340872045,
-5.68425722833147));
#94507=CARTESIAN_POINT('Ctrl Pts',(-6.47469263688536,-20.8525706359401,
-5.68565351562601));
#94508=CARTESIAN_POINT('Ctrl Pts',(-6.47586823453987,-20.8542831556721,
-5.68707721476377));
#94509=CARTESIAN_POINT('Ctrl Pts',(-6.47645603336713,-20.8551394155382,
-5.68778906433264));
#94510=CARTESIAN_POINT('Ctrl Pts',(-6.47704939965348,-20.8560146721983,
-5.68850776421543));
#94511=CARTESIAN_POINT('Ctrl Pts',(-6.47764795866675,-20.8569093949851,
-5.68923286325865));
#94512=CARTESIAN_POINT('Ctrl Pts',(-6.47806170308007,-20.857527857904,-5.68973407645831));
#94513=CARTESIAN_POINT('Ctrl Pts',(-6.4787652989644,-20.8585915532641,-5.69058656106244));
#94514=CARTESIAN_POINT('Ctrl Pts',(-6.4791619845149,-20.8591977964133,-5.69106721237673));
#94515=CARTESIAN_POINT('Ctrl Pts',(-6.47933917912821,-20.8594685978585,
-5.69128191347602));
#94516=CARTESIAN_POINT('Ctrl Pts',(-6.47945556311053,-20.8596474323066,
-5.69142293700902));
#94517=CARTESIAN_POINT('Ctrl Pts',(-6.47945882540606,-20.8596524399293,
-5.69142689015969));
#94518=CARTESIAN_POINT('Ctrl Pts',(-6.47953375728477,-20.859767460343,-5.69151769033493));
#94519=CARTESIAN_POINT('Ctrl Pts',(-6.48003658343336,-20.8605308716777,
-5.69212361565121));
#94520=CARTESIAN_POINT('Ctrl Pts',(-6.48095350691224,-20.8619644430849,
-5.69322805168281));
#94521=CARTESIAN_POINT('Ctrl Pts',(-6.48186934924366,-20.8633963241633,
-5.69433118547028));
#94522=CARTESIAN_POINT('Ctrl Pts',(-6.48319846339372,-20.8654970458354,
-5.69593183623601));
#94523=CARTESIAN_POINT('Ctrl Pts',(-6.484902500209,-20.8683231621742,-5.69798382309152));
#94524=CARTESIAN_POINT('Ctrl Pts',(-6.48534133346799,-20.8690509597383,
-5.69851226242518));
#94525=CARTESIAN_POINT('Ctrl Pts',(-6.48580489668337,-20.8698270318595,
-5.69907047190041));
#94526=CARTESIAN_POINT('Ctrl Pts',(-6.48629224595167,-20.8706526761846,
-5.69965731484674));
#94527=CARTESIAN_POINT('Ctrl Pts',(-6.48816837764793,-20.8738311307117,
-5.70191646392924));
#94528=CARTESIAN_POINT('Ctrl Pts',(-6.49039934096965,-20.8777425180432,
-5.70460275764763));
#94529=CARTESIAN_POINT('Ctrl Pts',(-6.492913072037,-20.8824761327407,-5.70762941498989));
#94530=CARTESIAN_POINT('Ctrl Pts',(-6.4932628924439,-20.8831348806239,-5.70805061617435));
#94531=CARTESIAN_POINT('Ctrl Pts',(-6.49361814054776,-20.8838095846428,
-5.70847835057653));
#94532=CARTESIAN_POINT('Ctrl Pts',(-6.49397857387117,-20.8845005141774,
-5.70891232619948));
#94533=CARTESIAN_POINT('Ctrl Pts',(-6.49545378708667,-20.8873284113619,
-5.7106885398085));
#94534=CARTESIAN_POINT('Ctrl Pts',(-6.49701614826464,-20.8904280304556,
-5.71256964974964));
#94535=CARTESIAN_POINT('Ctrl Pts',(-6.49864678920395,-20.8938186014525,
-5.71453293450427));
#94536=CARTESIAN_POINT('Ctrl Pts',(-6.4994621096736,-20.895513886951,-5.71551457688158));
#94537=CARTESIAN_POINT('Ctrl Pts',(-6.50029445787025,-20.8972819591972,
-5.71651671212822));
#94538=CARTESIAN_POINT('Ctrl Pts',(-6.50114109704214,-20.8991252361538,
-5.71753604458659));
#94539=CARTESIAN_POINT('Ctrl Pts',(-6.50164636287223,-20.9002252854929,
-5.718144372051));
#94540=CARTESIAN_POINT('Ctrl Pts',(-6.50233258152216,-20.9017422885018,
-5.71897055637223));
#94541=CARTESIAN_POINT('Ctrl Pts',(-6.50288249303833,-20.9029801780563,
-5.71963262872614));
#94542=CARTESIAN_POINT('Ctrl Pts',(-6.50325403039707,-20.903816534819,-5.72007994544244));
#94543=CARTESIAN_POINT('Ctrl Pts',(-6.50356421322428,-20.9045245122334,
-5.72045339232661));
#94544=CARTESIAN_POINT('Ctrl Pts',(-6.50372095659478,-20.9048832171215,
-5.72064210415655));
#94545=CARTESIAN_POINT('Ctrl Pts',(-6.50683086732657,-20.9120002018932,
-5.72438629405919));
#94546=CARTESIAN_POINT('Ctrl Pts',(-6.50969750337871,-20.9193271435348,
-5.72793343384607));
#94547=CARTESIAN_POINT('Ctrl Pts',(-6.51230992256894,-20.9268368343399,
-5.73127059607242));
#94548=CARTESIAN_POINT('Ctrl Pts',(-6.51361613216405,-20.9305916797424,
-5.73293917718559));
#94549=CARTESIAN_POINT('Ctrl Pts',(-6.51485881169394,-20.9343921918088,
-5.73455529299171));
#94550=CARTESIAN_POINT('Ctrl Pts',(-6.51603673967929,-20.9382348374568,
-5.73611749502398));
#94551=CARTESIAN_POINT('Ctrl Pts',(-6.51662570367197,-20.9401561602808,
-5.73689859604012));
#94552=CARTESIAN_POINT('Ctrl Pts',(-6.51719848126221,-20.9420880150999,
-5.7376662203995));
#94553=CARTESIAN_POINT('Ctrl Pts',(-6.5177549292471,-20.9440299532835,-5.73842019816372));
#94554=CARTESIAN_POINT('Ctrl Pts',(-6.518068227445,-20.9451233272374,-5.73884471201084));
#94555=CARTESIAN_POINT('Ctrl Pts',(-6.51851504736597,-20.9467195697101,
-5.73945651069025));
#94556=CARTESIAN_POINT('Ctrl Pts',(-6.51885870560263,-20.9479763409979,
-5.73992904768629));
#94557=CARTESIAN_POINT('Ctrl Pts',(-6.51912541772417,-20.9489517174058,
-5.74029578222449));
#94558=CARTESIAN_POINT('Ctrl Pts',(-6.51933137464634,-20.9497215873646,
-5.74058029811398));
#94559=CARTESIAN_POINT('Ctrl Pts',(-6.51937514746328,-20.94988556466,-5.74064102913961));
#94560=CARTESIAN_POINT('Ctrl Pts',(-6.51953189131393,-20.9504727426052,
-5.74085849777596));
#94561=CARTESIAN_POINT('Ctrl Pts',(-6.51995825601406,-20.9519071351304,
-5.7413568825184));
#94562=CARTESIAN_POINT('Ctrl Pts',(-6.52062847809654,-20.9542065208781,
-5.74210513476412));
#94563=CARTESIAN_POINT('Ctrl Pts',(-6.52081492568855,-20.9548461818904,
-5.74231328939388));
#94564=CARTESIAN_POINT('Ctrl Pts',(-6.52102006186129,-20.9555529011717,
-5.74254056006038));
#94565=CARTESIAN_POINT('Ctrl Pts',(-6.52124290425209,-20.9563273184521,
-5.74278576272304));
#94566=CARTESIAN_POINT('Ctrl Pts',(-6.5217203956944,-20.9579866868641,-5.74331116622743));
#94567=CARTESIAN_POINT('Ctrl Pts',(-6.52240651959259,-20.9604015063807,
-5.74405486018587));
#94568=CARTESIAN_POINT('Ctrl Pts',(-6.52310449530053,-20.9629612481078,
-5.74480417864417));
#94569=CARTESIAN_POINT('Ctrl Pts',(-6.52376236227997,-20.9653738959107,
-5.74551043799561));
#94570=CARTESIAN_POINT('Ctrl Pts',(-6.52443037325414,-20.9679152808702,
-5.74622123045526));
#94571=CARTESIAN_POINT('Ctrl Pts',(-6.52497603397311,-20.9700535545329,
-5.74679738364521));
#94572=CARTESIAN_POINT('Ctrl Pts',(-6.52509285049939,-20.9705113219565,
-5.74692072808235));
#94573=CARTESIAN_POINT('Ctrl Pts',(-6.52520417807828,-20.9709505462195,
-5.74703804466427));
#94574=CARTESIAN_POINT('Ctrl Pts',(-6.52530888899692,-20.9713659136585,
-5.74714817548923));
#94575=CARTESIAN_POINT('Ctrl Pts',(-6.52622696913516,-20.9750077554146,
-5.74811377606193));
#94576=CARTESIAN_POINT('Ctrl Pts',(-6.52695772118715,-20.9781122602895,
-5.74888261750753));
#94577=CARTESIAN_POINT('Ctrl Pts',(-6.52759396873366,-20.9809631998065,
-5.74956650069956));
#94578=CARTESIAN_POINT('Ctrl Pts',(-6.52829065852984,-20.9840849728992,
-5.75031535143271));
#94579=CARTESIAN_POINT('Ctrl Pts',(-6.5288736745872,-20.9869032273788,-5.75096189958322));
#94580=CARTESIAN_POINT('Ctrl Pts',(-6.52942882700837,-20.9898113882429,
-5.75160948203996));
#94581=CARTESIAN_POINT('Ctrl Pts',(-6.52959567907912,-20.9906854412845,
-5.75180411412616));
#94582=CARTESIAN_POINT('Ctrl Pts',(-6.5297597991612,-20.9915677238951,-5.75199858061829));
#94583=CARTESIAN_POINT('Ctrl Pts',(-6.52992296280191,-20.9924691784577,
-5.75219501960245));
#94584=CARTESIAN_POINT('Ctrl Pts',(-6.5330537311515,-21.0097662024811,-5.75596427206302));
#94585=CARTESIAN_POINT('Ctrl Pts',(-6.53518820255804,-21.027504551347,-5.75853433457631));
#94586=CARTESIAN_POINT('Ctrl Pts',(-6.53629205249415,-21.0453989597899,
-5.7598638744019));
#94587=CARTESIAN_POINT('Ctrl Pts',(-6.53688316709687,-21.0549814635267,
-5.76057584654602));
#94588=CARTESIAN_POINT('Ctrl Pts',(-6.53717929485058,-21.0646085312747,
-5.76093275370235));
#94589=CARTESIAN_POINT('Ctrl Pts',(-6.53717906472003,-21.0742356128,-5.76093294480616));
#94590=CARTESIAN_POINT('Origin',(2.84607155346,-21.0742356128,5.53854202767));
#94591=CARTESIAN_POINT('Origin',(-2.12372695744,-21.0742356128,-7.96338790087));
#94592=CARTESIAN_POINT('Origin',(-2.12372695744,-21.0742356128,-7.96338790086));
#94593=CARTESIAN_POINT('Ctrl Pts',(4.9961481711E-16,-20.7742356128,-8.56468050289));
#94594=CARTESIAN_POINT('Ctrl Pts',(4.9961481711E-16,-20.7742356128,-8.56468050289));
#94595=CARTESIAN_POINT('Ctrl Pts',(4.9961481711E-16,-20.7742356128,-8.56468050289));
#94596=CARTESIAN_POINT('Ctrl Pts',(4.9961481711E-16,-20.7742356128,-8.56468050289));
#94597=CARTESIAN_POINT('Ctrl Pts',(4.9961481711E-16,-20.7742356128,-8.56468050289));
#94598=CARTESIAN_POINT('Ctrl Pts',(4.9961481711E-16,-20.7742356128,-8.56468050289));
#94599=CARTESIAN_POINT('Ctrl Pts',(-0.0739219411499,-20.7751437694,-8.66437291113));
#94600=CARTESIAN_POINT('Ctrl Pts',(-0.0443506287058,-20.7751432313524,-8.66431384724197));
#94601=CARTESIAN_POINT('Ctrl Pts',(-0.0147838746951,-20.7751431251168,-8.66430218528719));
#94602=CARTESIAN_POINT('Ctrl Pts',(0.0147838753332,-20.7751431251168,-8.66430218528719));
#94603=CARTESIAN_POINT('Ctrl Pts',(0.0443506291288,-20.7751432313524,-8.66431384724197));
#94604=CARTESIAN_POINT('Ctrl Pts',(0.0739219411508,-20.7751437694,-8.66437291113));
#94605=CARTESIAN_POINT('Ctrl Pts',(-0.152819706761,-20.8273615349,-8.76362621195));
#94606=CARTESIAN_POINT('Ctrl Pts',(-0.0916409326323,-20.8166811403,-8.76306421395));
#94607=CARTESIAN_POINT('Ctrl Pts',(-0.0305356341741,-20.8113350481,-8.76271543885));
#94608=CARTESIAN_POINT('Ctrl Pts',(0.0305356341745,-20.8113350481,-8.76271543885));
#94609=CARTESIAN_POINT('Ctrl Pts',(0.0916409326401,-20.8166811403,-8.76306421395));
#94610=CARTESIAN_POINT('Ctrl Pts',(0.15281970676,-20.8273615349,-8.76362621195));
#94611=CARTESIAN_POINT('Ctrl Pts',(-0.208944325295,-20.9488183216,-8.82888814763));
#94612=CARTESIAN_POINT('Ctrl Pts',(-0.12665670177,-20.9401545709,-8.84731068645));
#94613=CARTESIAN_POINT('Ctrl Pts',(-0.042439220578,-20.9357432811,-8.85664858235));
#94614=CARTESIAN_POINT('Ctrl Pts',(0.0424392246749,-20.9357432811,-8.85664858234));
#94615=CARTESIAN_POINT('Ctrl Pts',(0.126656704487,-20.9401545709,-8.84731068645));
#94616=CARTESIAN_POINT('Ctrl Pts',(0.208944325295,-20.9488183216,-8.82888814763));
#94617=CARTESIAN_POINT('Ctrl Pts',(-0.207931718075,-21.0742356128,-8.82796731988));
#94618=CARTESIAN_POINT('Ctrl Pts',(-0.125978962059,-21.0742356128,-8.8453886697));
#94619=CARTESIAN_POINT('Ctrl Pts',(-0.0422016682077,-21.0742356128,-8.85422710799));
#94620=CARTESIAN_POINT('Ctrl Pts',(0.0422016682077,-21.0742356128,-8.85422710799));
#94621=CARTESIAN_POINT('Ctrl Pts',(0.125978962059,-21.0742356128,-8.8453886697));
#94622=CARTESIAN_POINT('Ctrl Pts',(0.207931718075,-21.0742356128,-8.82796731988));
#94623=CARTESIAN_POINT('',(-0.207931718075,-21.0742356128,-8.82796731988));
#94624=CARTESIAN_POINT('Ctrl Pts',(-0.207931718084929,-21.0742356128,-8.82796731992671));
#94625=CARTESIAN_POINT('Ctrl Pts',(-0.20793171808493,-21.058807737806,-8.82796731992671));
#94626=CARTESIAN_POINT('Ctrl Pts',(-0.206991629534422,-21.0430697565,-8.82694819743859));
#94627=CARTESIAN_POINT('Ctrl Pts',(-0.205085678166485,-21.0272270718591,
-8.82478346590272));
#94628=CARTESIAN_POINT('Ctrl Pts',(-0.203232437820272,-21.0118225327598,
-8.82267860221707));
#94629=CARTESIAN_POINT('Ctrl Pts',(-0.200465888764402,-20.9963193501386,
-8.81949003333179));
#94630=CARTESIAN_POINT('Ctrl Pts',(-0.19677085228483,-20.980944658764,-8.81513107578119));
#94631=CARTESIAN_POINT('Ctrl Pts',(-0.195150931677628,-20.9742043249338,
-8.81322008919115));
#94632=CARTESIAN_POINT('Ctrl Pts',(-0.193352680913129,-20.9674891605202,
-8.81108459728923));
#94633=CARTESIAN_POINT('Ctrl Pts',(-0.191375454563993,-20.9608204182865,
-8.80871960777743));
#94634=CARTESIAN_POINT('Ctrl Pts',(-0.187012508935183,-20.9461051785314,
-8.80350102435265));
#94635=CARTESIAN_POINT('Ctrl Pts',(-0.181777358262892,-20.9316143647805,
-8.79716206443024));
#94636=CARTESIAN_POINT('Ctrl Pts',(-0.175670860520978,-20.9175956542866,
-8.78967869242846));
#94637=CARTESIAN_POINT('Ctrl Pts',(-0.173991508311643,-20.9137403589218,
-8.78762068506718));
#94638=CARTESIAN_POINT('Ctrl Pts',(-0.172246322135771,-20.9099209095847,
-8.78547638336927));
#94639=CARTESIAN_POINT('Ctrl Pts',(-0.170435476972045,-20.9061427547366,
-8.78324590276991));
#94640=CARTESIAN_POINT('Ctrl Pts',(-0.166237736720972,-20.8973845720942,
-8.77807540096295));
#94641=CARTESIAN_POINT('Ctrl Pts',(-0.161687020782996,-20.888848122063,
-8.77244120058218));
#94642=CARTESIAN_POINT('Ctrl Pts',(-0.156787037910526,-20.8806033711716,
-8.76635090530234));
#94643=CARTESIAN_POINT('Ctrl Pts',(-0.154337046474292,-20.8764809957259,
-8.76330575766242));
#94644=CARTESIAN_POINT('Ctrl Pts',(-0.151799750460363,-20.8724314930626,
-8.7601466442437));
#94645=CARTESIAN_POINT('Ctrl Pts',(-0.149175845791688,-20.868463921362,
-8.75687546171829));
#94646=CARTESIAN_POINT('Ctrl Pts',(-0.147863893457352,-20.8664801355117,
-8.75523987045558));
#94647=CARTESIAN_POINT('Ctrl Pts',(-0.146530289983459,-20.8645168283287,
-8.7535762667923));
#94648=CARTESIAN_POINT('Ctrl Pts',(-0.145175132487716,-20.8625751257222,
-8.75188493254781));
#94649=CARTESIAN_POINT('Ctrl Pts',(-0.144417055132561,-20.8614889340574,
-8.75093879736075));
#94650=CARTESIAN_POINT('Ctrl Pts',(-0.143420664491045,-20.8600877544966,
-8.74969906130205));
#94651=CARTESIAN_POINT('Ctrl Pts',(-0.142574027140396,-20.8589148254055,
-8.74864098373894));
#94652=CARTESIAN_POINT('Ctrl Pts',(-0.141907194996003,-20.8579909979599,
-8.74780761614677));
#94653=CARTESIAN_POINT('Ctrl Pts',(-0.141333533377844,-20.8572073668546,
-8.74708833579977));
#94654=CARTESIAN_POINT('Ctrl Pts',(-0.141045101226366,-20.8568159508745,
-8.74672804704856));
#94655=CARTESIAN_POINT('Ctrl Pts',(-0.137764128976178,-20.8523635173909,
-8.74262969189393));
#94656=CARTESIAN_POINT('Ctrl Pts',(-0.133874809386624,-20.8474708462403,
-8.73788048463094));
#94657=CARTESIAN_POINT('Ctrl Pts',(-0.129357595883939,-20.8422910728369,
-8.7323721476904));
#94658=CARTESIAN_POINT('Ctrl Pts',(-0.124987989632303,-20.8372805569,-8.72704380456091));
#94659=CARTESIAN_POINT('Ctrl Pts',(-0.120030647505103,-20.832001217571,
-8.72100417194565));
#94660=CARTESIAN_POINT('Ctrl Pts',(-0.114469013595954,-20.8266392802401,
-8.7141550459496));
#94661=CARTESIAN_POINT('Ctrl Pts',(-0.109120501929856,-20.821482812764,
-8.7075683789933));
#94662=CARTESIAN_POINT('Ctrl Pts',(-0.103212926652253,-20.8162500078874,
-8.700232109932));
#94663=CARTESIAN_POINT('Ctrl Pts',(-0.0967355344333589,-20.8111521065984,
-8.69207251981437));
#94664=CARTESIAN_POINT('Ctrl Pts',(-0.0906551254465784,-20.8063666429791,
-8.68441301064724));
#94665=CARTESIAN_POINT('Ctrl Pts',(-0.0840724678907984,-20.8017004470412,
-8.67602728380219));
#94666=CARTESIAN_POINT('Ctrl Pts',(-0.0769845460691857,-20.7973657450748,
-8.66687829516898));
#94667=CARTESIAN_POINT('Ctrl Pts',(-0.070136880226554,-20.7931779744784,
-8.65803942553482));
#94668=CARTESIAN_POINT('Ctrl Pts',(-0.0628174889399522,-20.7892999888431,
-8.64848743646407));
#94669=CARTESIAN_POINT('Ctrl Pts',(-0.0550312825271058,-20.7859539936799,
-8.63822244714815));
#94670=CARTESIAN_POINT('Ctrl Pts',(-0.047498167146639,-20.7827167602583,
-8.62829112182797));
#94671=CARTESIAN_POINT('Ctrl Pts',(-0.0395279866114865,-20.7799780356088,
-8.61769177993309));
#94672=CARTESIAN_POINT('Ctrl Pts',(-0.0311341756824106,-20.7779617380583,
-8.60646612885158));
#94673=CARTESIAN_POINT('Ctrl Pts',(-0.0230959746664929,-20.776030862422,
-8.59571606065369));
#94674=CARTESIAN_POINT('Ctrl Pts',(-0.0146692297076344,-20.7747631710937,
-8.58439126306306));
#94675=CARTESIAN_POINT('Ctrl Pts',(-0.00587517811084473,-20.7743676687153,
-8.5725740159694));
#94676=CARTESIAN_POINT('Ctrl Pts',(-0.00393453439359006,-20.7742803904912,
-8.56996622295441));
#94677=CARTESIAN_POINT('Ctrl Pts',(-0.00197604276587682,-20.7742356127995,
-8.56733464308287));
#94678=CARTESIAN_POINT('Ctrl Pts',(2.94663555151017E-14,-20.7742356128,
-8.56468050289));
#94679=CARTESIAN_POINT('Origin',(1.59370492737E-14,-21.0742356128,-7.84982397628));
#94680=CARTESIAN_POINT('Origin',(2.84607155346,-21.0742356128,5.53854202767));
#94681=CARTESIAN_POINT('Origin',(2.84607155346,-21.0742356128,5.53854202767));
#94682=CARTESIAN_POINT('Origin',(-3.69394702409,-23.1223803511,-7.27665075431));
#94683=CARTESIAN_POINT('',(-3.83031550589,-22.5742356128,-7.54386534443));
#94684=CARTESIAN_POINT('Origin',(2.84607155346,-21.2742356128,5.53854202767));
#94685=CARTESIAN_POINT('',(-6.53717906469,-22.1242356128,-5.76093294477));
#94686=CARTESIAN_POINT('Origin',(1.56676269779E-14,-23.2742356128,-7.84982397628));
#94687=CARTESIAN_POINT('',(-0.207931718075,-22.6642356128,-8.82796731988));
#94688=CARTESIAN_POINT('Origin',(2.84607155346,-22.6642356128,5.53854202767));
#94689=CARTESIAN_POINT('Origin',(-6.34552156645,-22.1242356128,-5.5301356238));
#94690=CARTESIAN_POINT('',(-6.56346233154,-21.0742356128,-5.32397592135));
#94691=CARTESIAN_POINT('Origin',(-6.34552156645,-21.0742356128,-5.5301356238));
#94692=CARTESIAN_POINT('',(-6.56346233154,-21.9742356128,-5.32397592135));
#94693=CARTESIAN_POINT('Origin',(-6.34552156645,-21.0742356128,-5.5301356238));
#94694=CARTESIAN_POINT('Origin',(-6.34552156645,-21.0742356128,-5.5301356238));
#94695=CARTESIAN_POINT('Origin',(-5.6152263525,-21.0742356128,-4.75810745444));
#94696=CARTESIAN_POINT('',(-5.67833560965,-21.0742356128,-4.38826834763));
#94697=CARTESIAN_POINT('Origin',(-6.78099426296,-23.1742356128,-5.55393878512));
#94698=CARTESIAN_POINT('',(-6.4527882763,-22.8742356128,-5.20697736155));
#94699=CARTESIAN_POINT('Origin',(-6.6707290414,-22.8742356128,-5.00081765911));
#94700=CARTESIAN_POINT('',(-5.89627637474,-23.1742356128,-4.18210864518));
#94701=CARTESIAN_POINT('Ctrl Pts',(-8.01224741424,-22.8742356128,11.9089404858));
#94702=CARTESIAN_POINT('Ctrl Pts',(-8.01224741424,-22.8742356128,11.9089404858));
#94703=CARTESIAN_POINT('Ctrl Pts',(-8.01224741424,-22.8742356128,11.9089404858));
#94704=CARTESIAN_POINT('Ctrl Pts',(-8.01224741424,-22.8742356128,11.9089404858));
#94705=CARTESIAN_POINT('Ctrl Pts',(-8.01224741424,-22.8742356128,11.9089404858));
#94706=CARTESIAN_POINT('Ctrl Pts',(-8.01224741424,-22.8742356128,11.9089404858));
#94707=CARTESIAN_POINT('Ctrl Pts',(-7.9829584197,-22.9540055384,11.8818593216));
#94708=CARTESIAN_POINT('Ctrl Pts',(-7.97710218322187,-22.9460296098,11.8764445334088));
#94709=CARTESIAN_POINT('Ctrl Pts',(-7.97124593377672,-22.9380536813,11.871029733228));
#94710=CARTESIAN_POINT('Ctrl Pts',(-7.96538971029938,-22.9300777704,11.8656149570576));
#94711=CARTESIAN_POINT('Ctrl Pts',(-7.95953347384813,-22.9221018241,11.8602001688912));
#94712=CARTESIAN_POINT('Ctrl Pts',(-7.95367723737,-22.9141258956,11.8547853807));
#94713=CARTESIAN_POINT('Ctrl Pts',(-7.95813278234,-23.0338190575,11.8499462819));
#94714=CARTESIAN_POINT('Ctrl Pts',(-7.94826431478,-23.0178581995,11.8371231287));
#94715=CARTESIAN_POINT('Ctrl Pts',(-7.9374729589,-23.0018973414,11.825280653));
#94716=CARTESIAN_POINT('Ctrl Pts',(-7.92575194148,-22.985933847,11.8144431763));
#94717=CARTESIAN_POINT('Ctrl Pts',(-7.91310342567,-22.9699706625,11.8046126985));
#94718=CARTESIAN_POINT('Ctrl Pts',(-7.8995407209,-22.9540193262,11.7957709419));
#94719=CARTESIAN_POINT('Ctrl Pts',(-7.93828028322,-23.1128615217,11.8131880532));
#94720=CARTESIAN_POINT('Ctrl Pts',(-7.92684545497,-23.0884116462,11.7921000842));
#94721=CARTESIAN_POINT('Ctrl Pts',(-7.91214424925,-23.0639617707,11.7733048715));
#94722=CARTESIAN_POINT('Ctrl Pts',(-7.89441627707,-23.0398170763,11.7569132495));
#94723=CARTESIAN_POINT('Ctrl Pts',(-7.87387109886,-23.0162629748,11.743118982));
#94724=CARTESIAN_POINT('Ctrl Pts',(-7.85067760242,-22.993550642,11.7321889401));
#94725=CARTESIAN_POINT('Ctrl Pts',(-7.91959338184,-23.2114810387,11.7607695014));
#94726=CARTESIAN_POINT('Ctrl Pts',(-7.91104746367,-23.1749621125,11.7286518091));
#94727=CARTESIAN_POINT('Ctrl Pts',(-7.89353608553,-23.1384431864,11.699923838));
#94728=CARTESIAN_POINT('Ctrl Pts',(-7.86773087157,-23.1032976549,11.6760638439));
#94729=CARTESIAN_POINT('Ctrl Pts',(-7.83466815185,-23.0709369526,11.6580300375));
#94730=CARTESIAN_POINT('Ctrl Pts',(-7.79578364279,-23.0428577871,11.6462926502));
#94731=CARTESIAN_POINT('Ctrl Pts',(-7.9155846643,-23.3039994083,11.6969647216));
#94732=CARTESIAN_POINT('Ctrl Pts',(-7.91452330598,-23.2518708228,11.6602860726));
#94733=CARTESIAN_POINT('Ctrl Pts',(-7.89660201748,-23.1997422373,11.6241805214));
#94734=CARTESIAN_POINT('Ctrl Pts',(-7.86189143973,-23.152468004,11.5920864577));
#94735=CARTESIAN_POINT('Ctrl Pts',(-7.813878937,-23.1147977551,11.5672283653));
#94736=CARTESIAN_POINT('Ctrl Pts',(-7.7578101336,-23.0891176504,11.5510833748));
#94737=CARTESIAN_POINT('Ctrl Pts',(-7.91547477954,-23.3227166577,11.6832984902));
#94738=CARTESIAN_POINT('Ctrl Pts',(-7.91611333971,-23.2672089627,11.6460479894));
#94739=CARTESIAN_POINT('Ctrl Pts',(-7.8981958921,-23.2117012676,11.6085883389));
#94740=CARTESIAN_POINT('Ctrl Pts',(-7.86161748026,-23.161883129,11.5747672402));
#94741=CARTESIAN_POINT('Ctrl Pts',(-7.81044715471,-23.1232964092,11.5483470151));
#94742=CARTESIAN_POINT('Ctrl Pts',(-7.75082874056,-23.0984762171,11.5310636155));
#94743=CARTESIAN_POINT('Ctrl Pts',(-7.91677660432,-23.3563766548,11.6571003353));
#94744=CARTESIAN_POINT('Ctrl Pts',(-7.92076615745,-23.2943123864,11.6196720445));
#94745=CARTESIAN_POINT('Ctrl Pts',(-7.90299820073,-23.232248118,11.5801462658));
#94746=CARTESIAN_POINT('Ctrl Pts',(-7.86292199155,-23.177666138,11.5430910367));
#94747=CARTESIAN_POINT('Ctrl Pts',(-7.80583878281,-23.1377865125,11.5134079972));
#94748=CARTESIAN_POINT('Ctrl Pts',(-7.73977321638,-23.1153060651,11.4934396195));
#94749=CARTESIAN_POINT('Ctrl Pts',(-7.92150726931,-23.3879026248,11.6287650914));
#94750=CARTESIAN_POINT('Ctrl Pts',(-7.92877089289,-23.3187255874,11.5933170483));
#94751=CARTESIAN_POINT('Ctrl Pts',(-7.91117889789,-23.2495485499,11.5529211001));
#94752=CARTESIAN_POINT('Ctrl Pts',(-7.86756066908,-23.1901424998,11.512590852));
#94753=CARTESIAN_POINT('Ctrl Pts',(-7.80474013232,-23.1498013146,11.4786358364));
#94754=CARTESIAN_POINT('Ctrl Pts',(-7.73293017851,-23.1310691765,11.4544031088));
#94755=CARTESIAN_POINT('Ctrl Pts',(-7.92449811306,-23.4017307742,11.6153459759));
#94756=CARTESIAN_POINT('Ctrl Pts',(-7.93315539553,-23.3292061538,11.5813393505));
#94757=CARTESIAN_POINT('Ctrl Pts',(-7.91560788059,-23.2566815335,11.5408618336));
#94758=CARTESIAN_POINT('Ctrl Pts',(-7.8703758173,-23.195077514,11.4990394033));
#94759=CARTESIAN_POINT('Ctrl Pts',(-7.80503619115,-23.1547136059,11.4628778853));
#94760=CARTESIAN_POINT('Ctrl Pts',(-7.73084447823,-23.1379833031,11.4362901237));
#94761=CARTESIAN_POINT('Ctrl Pts',(-7.93181038161,-23.4257772831,11.589727728));
#94762=CARTESIAN_POINT('Ctrl Pts',(-7.94259323556,-23.3469662924,11.5595945247));
#94763=CARTESIAN_POINT('Ctrl Pts',(-7.92493476604,-23.2681553018,11.519738107));
#94764=CARTESIAN_POINT('Ctrl Pts',(-7.87677950673,-23.2025700218,11.4752128338));
#94765=CARTESIAN_POINT('Ctrl Pts',(-7.80718493183,-23.1625463217,11.4343934188));
#94766=CARTESIAN_POINT('Ctrl Pts',(-7.7293286586,-23.1500063561,11.4025092567));
#94767=CARTESIAN_POINT('Ctrl Pts',(-7.9432480685,-23.4460266432,11.5624437668));
#94768=CARTESIAN_POINT('Ctrl Pts',(-7.95448793125,-23.3612017167,11.5386017188));
#94769=CARTESIAN_POINT('Ctrl Pts',(-7.93590497166,-23.2763767903,11.501049282));
#94770=CARTESIAN_POINT('Ctrl Pts',(-7.88511487967,-23.2072029876,11.4540877922));
#94771=CARTESIAN_POINT('Ctrl Pts',(-7.81267918242,-23.1680646299,11.4074826391));
#94772=CARTESIAN_POINT('Ctrl Pts',(-7.73333253621,-23.160131205,11.3683518533));
#94773=CARTESIAN_POINT('Ctrl Pts',(-7.94999449773,-23.4537301075,11.5494738265));
#94774=CARTESIAN_POINT('Ctrl Pts',(-7.96070319611,-23.3664896798,11.5290641468));
#94775=CARTESIAN_POINT('Ctrl Pts',(-7.94047144087,-23.2792492521,11.4940040546));
#94776=CARTESIAN_POINT('Ctrl Pts',(-7.88862227931,-23.2086330447,11.4460633288));
#94777=CARTESIAN_POINT('Ctrl Pts',(-7.81641530283,-23.1699761106,11.3956528028));
#94778=CARTESIAN_POINT('Ctrl Pts',(-7.73725084228,-23.1639828938,11.3527669762));
#94779=CARTESIAN_POINT('Ctrl Pts',(-7.96049908281,-23.4651088112,11.5297325584));
#94780=CARTESIAN_POINT('Ctrl Pts',(-7.97007721933,-23.3740670261,11.5152608651));
#94781=CARTESIAN_POINT('Ctrl Pts',(-7.94978862977,-23.283025241,11.4814426691));
#94782=CARTESIAN_POINT('Ctrl Pts',(-7.89640547391,-23.2103198029,11.4320835828));
#94783=CARTESIAN_POINT('Ctrl Pts',(-7.82205263778,-23.1724642569,11.3783945077));
#94784=CARTESIAN_POINT('Ctrl Pts',(-7.74357804624,-23.1696721938,11.3291632218));
#94785=CARTESIAN_POINT('Ctrl Pts',(-7.97506561416,-23.4709827428,11.5096523074));
#94786=CARTESIAN_POINT('Ctrl Pts',(-7.9810664946,-23.3778924556,11.5016653458));
#94787=CARTESIAN_POINT('Ctrl Pts',(-7.95750099919,-23.2848021685,11.4721994645));
#94788=CARTESIAN_POINT('Ctrl Pts',(-7.90326281492,-23.2109322204,11.4220498027));
#94789=CARTESIAN_POINT('Ctrl Pts',(-7.83108568197,-23.1736253884,11.3629902197));
#94790=CARTESIAN_POINT('Ctrl Pts',(-7.75598816389,-23.1726091877,11.3070891094));
#94791=CARTESIAN_POINT('Ctrl Pts',(-7.97859188254,-23.4732430341,11.5041738872));
#94792=CARTESIAN_POINT('Ctrl Pts',(-7.98384179584,-23.3793507423,11.4980345926));
#94793=CARTESIAN_POINT('Ctrl Pts',(-7.96094423,-23.2854584504,11.4680769659));
#94794=CARTESIAN_POINT('Ctrl Pts',(-7.90642284084,-23.2112027901,11.4176654474));
#94795=CARTESIAN_POINT('Ctrl Pts',(-7.83310388244,-23.1740525381,11.3586594366));
#94796=CARTESIAN_POINT('Ctrl Pts',(-7.75868462277,-23.1737393161,11.3008434315));
#94797=CARTESIAN_POINT('Ctrl Pts',(-7.98964252128,-23.4742356128,11.4914912894));
#94798=CARTESIAN_POINT('Ctrl Pts',(-7.99152767193,-23.3799878332,11.4894524491));
#94799=CARTESIAN_POINT('Ctrl Pts',(-7.96481831906,-23.2857400536,11.4638652708));
#94800=CARTESIAN_POINT('Ctrl Pts',(-7.91010101675,-23.2112175685,11.4132726072));
#94801=CARTESIAN_POINT('Ctrl Pts',(-7.84045640218,-23.1742356128,11.3497690655));
#94802=CARTESIAN_POINT('Ctrl Pts',(-7.76937087202,-23.1742356128,11.2878239122));
#94803=CARTESIAN_POINT('Ctrl Pts',(-7.99564314217,-23.4742356128,11.4850014593));
#94804=CARTESIAN_POINT('Ctrl Pts',(-7.99564314217,-23.3799878332,11.4850014593));
#94805=CARTESIAN_POINT('Ctrl Pts',(-7.96846821668,-23.2857400536,11.4598750038));
#94806=CARTESIAN_POINT('Ctrl Pts',(-7.91377225193,-23.2112466293,11.4093020693));
#94807=CARTESIAN_POINT('Ctrl Pts',(-7.84457187242,-23.1742356128,11.3453180757));
#94808=CARTESIAN_POINT('Ctrl Pts',(-7.77537149291,-23.1742356128,11.2813340821));
#94809=CARTESIAN_POINT('',(-7.77537149291,-23.1742356128,11.2813340821));
#94810=CARTESIAN_POINT('Ctrl Pts',(-7.77537149291,-23.1742356128,11.2813340821));
#94811=CARTESIAN_POINT('Ctrl Pts',(-7.76937087202,-23.1742356128,11.2878239122));
#94812=CARTESIAN_POINT('Ctrl Pts',(-7.75868462277,-23.1737393161,11.3008434315));
#94813=CARTESIAN_POINT('Ctrl Pts',(-7.75598816389,-23.1726091877,11.3070891094));
#94814=CARTESIAN_POINT('Ctrl Pts',(-7.74357804624,-23.1696721938,11.3291632218));
#94815=CARTESIAN_POINT('Ctrl Pts',(-7.73725084228,-23.1639828938,11.3527669762));
#94816=CARTESIAN_POINT('Ctrl Pts',(-7.73333253621,-23.160131205,11.3683518533));
#94817=CARTESIAN_POINT('Ctrl Pts',(-7.7293286586,-23.1500063561,11.4025092567));
#94818=CARTESIAN_POINT('Ctrl Pts',(-7.73084447823,-23.1379833031,11.4362901237));
#94819=CARTESIAN_POINT('Ctrl Pts',(-7.73293017851,-23.1310691765,11.4544031088));
#94820=CARTESIAN_POINT('Ctrl Pts',(-7.73977321638,-23.1153060651,11.4934396195));
#94821=CARTESIAN_POINT('Ctrl Pts',(-7.75082874056,-23.0984762171,11.5310636155));
#94822=CARTESIAN_POINT('Ctrl Pts',(-7.7578101336,-23.0891176504,11.5510833748));
#94823=CARTESIAN_POINT('Ctrl Pts',(-7.79578364279,-23.0428577871,11.6462926502));
#94824=CARTESIAN_POINT('Ctrl Pts',(-7.85067760242,-22.993550642,11.7321889401));
#94825=CARTESIAN_POINT('Ctrl Pts',(-7.8995407209,-22.9540193262,11.7957709419));
#94826=CARTESIAN_POINT('Ctrl Pts',(-7.95367723737,-22.9141258956,11.8547853807));
#94827=CARTESIAN_POINT('Ctrl Pts',(-8.01224741424,-22.8742356128,11.9089404858));
#94828=CARTESIAN_POINT('Origin',(-7.77692939202971,-23.472114284594,11.2827738681602));
#94829=CARTESIAN_POINT('Origin',(-6.6707290414,-22.8742356128,10.2599605573));
#94830=CARTESIAN_POINT('',(-5.39652599911,-23.1742356128,9.08180806924));
#94831=CARTESIAN_POINT('',(-6.58594874601,-23.1742356128,10.1815710757));
#94832=CARTESIAN_POINT('Origin',(-5.39652599911,-22.8742356128,9.08180806924));
#94833=CARTESIAN_POINT('Origin',(-4.98919124473,-22.8742356128,9.52235136777));
#94834=CARTESIAN_POINT('',(-4.62185483489,-23.1742356128,9.04794230167));
#94835=CARTESIAN_POINT('Origin',(-4.98919124473,-23.1742356128,9.52235136777));
#94836=CARTESIAN_POINT('Origin',(-4.62185483489,-22.8742356128,9.04794230167));
#94837=CARTESIAN_POINT('Origin',(-0.00234331738803,-22.8742356128,3.08191746407));
#94838=CARTESIAN_POINT('',(-0.972828518105,-23.1742356128,10.5646641188));
#94839=CARTESIAN_POINT('Origin',(-0.00234331738835,-23.1742356128,3.08191746407));
#94840=CARTESIAN_POINT('Origin',(-0.972828518105,-22.8742356128,10.5646641188));
#94841=CARTESIAN_POINT('Origin',(-1.05,-22.8742356128,11.1596805575));
#94842=CARTESIAN_POINT('',(-0.45,-23.1742356128,11.1596805575));
#94843=CARTESIAN_POINT('Origin',(-1.05,-23.1742356128,11.1596805575));
#94844=CARTESIAN_POINT('Origin',(-0.45,-22.8742356128,11.1596805575));
#94845=CARTESIAN_POINT('Origin',(-0.45,-22.8742356128,2.93538176615));
#94846=CARTESIAN_POINT('',(-0.45,-23.1742356128,14.92922515));
#94847=CARTESIAN_POINT('',(-0.45,-23.1742356128,13.0444528538));
#94848=CARTESIAN_POINT('Origin',(-0.45,-22.8742356128,14.92922515));
#94849=CARTESIAN_POINT('Ctrl Pts',(-8.78908955148,-23.4742356128,12.6272235745));
#94850=CARTESIAN_POINT('Ctrl Pts',(-8.78908955148,-23.3799878332,12.6272235745));
#94851=CARTESIAN_POINT('Ctrl Pts',(-8.76403540825,-23.2856521198,12.6543202923));
#94852=CARTESIAN_POINT('Ctrl Pts',(-8.71344985896,-23.2111401141,12.7090299003));
#94853=CARTESIAN_POINT('Ctrl Pts',(-8.64940616788,-23.1742356128,12.7782948442));
#94854=CARTESIAN_POINT('Ctrl Pts',(-8.58542217429,-23.1742356128,12.8474952237));
#94855=CARTESIAN_POINT('Ctrl Pts',(-8.71988917196,-23.4742356128,12.5632395809));
#94856=CARTESIAN_POINT('Ctrl Pts',(-8.72947215345,-23.3790967554,12.5721001887));
#94857=CARTESIAN_POINT('Ctrl Pts',(-8.71152123069,-23.285897088,12.6066774531));
#94858=CARTESIAN_POINT('Ctrl Pts',(-8.66821560358,-23.2117943285,12.6661101146));
#94859=CARTESIAN_POINT('Ctrl Pts',(-8.60980196734,-23.1742356128,12.7407571089));
#94860=CARTESIAN_POINT('Ctrl Pts',(-8.55126681507,-23.1742356128,12.8159145257));
#94861=CARTESIAN_POINT('Ctrl Pts',(-8.65068769611,-23.4557342571,12.4992545736));
#94862=CARTESIAN_POINT('Ctrl Pts',(-8.67114447119,-23.3616092561,12.5181692988));
#94863=CARTESIAN_POINT('Ctrl Pts',(-8.6616791149,-23.2705882254,12.5620766304));
#94864=CARTESIAN_POINT('Ctrl Pts',(-8.62409294795,-23.1983198307,12.6285650769));
#94865=CARTESIAN_POINT('Ctrl Pts',(-8.568611422,-23.16211697,12.707808508));
#94866=CARTESIAN_POINT('Ctrl Pts',(-8.51298776904,-23.1652660131,12.7860692819));
#94867=CARTESIAN_POINT('Ctrl Pts',(-8.58504814405,-23.4187037356,12.4385629891));
#94868=CARTESIAN_POINT('Ctrl Pts',(-8.61720687318,-23.3287980114,12.4682975647));
#94869=CARTESIAN_POINT('Ctrl Pts',(-8.61787660959,-23.2418003868,12.5228744536));
#94870=CARTESIAN_POINT('Ctrl Pts',(-8.58556282332,-23.1726965799,12.5981338043));
#94871=CARTESIAN_POINT('Ctrl Pts',(-8.53069999004,-23.1387145708,12.6814672949));
#94872=CARTESIAN_POINT('Ctrl Pts',(-8.47363957019,-23.1456118409,12.7605886079));
#94873=CARTESIAN_POINT('Ctrl Pts',(-8.46797276655,-23.3115821157,12.3303128573));
#94874=CARTESIAN_POINT('Ctrl Pts',(-8.52237213304,-23.2378310806,12.3806115513));
#94875=CARTESIAN_POINT('Ctrl Pts',(-8.54446981637,-23.1647358306,12.4578324878));
#94876=CARTESIAN_POINT('Ctrl Pts',(-8.52245288296,-23.1060736658,12.5529815994));
#94877=CARTESIAN_POINT('Ctrl Pts',(-8.46636077569,-23.0779179681,12.6438102103));
#94878=CARTESIAN_POINT('Ctrl Pts',(-8.40034769996,-23.089880852,12.7198837328));
#94879=CARTESIAN_POINT('Ctrl Pts',(-8.38931991359,-23.1521307593,12.2575889261));
#94880=CARTESIAN_POINT('Ctrl Pts',(-8.45970633708,-23.1061611813,12.3226695586));
#94881=CARTESIAN_POINT('Ctrl Pts',(-8.4993062219,-23.0588540528,12.4194802488));
#94882=CARTESIAN_POINT('Ctrl Pts',(-8.48540796624,-23.0202466991,12.5332516118));
#94883=CARTESIAN_POINT('Ctrl Pts',(-8.42613724507,-23.0015045278,12.6297956016));
#94884=CARTESIAN_POINT('Ctrl Pts',(-8.34720486119,-23.0113292253,12.6980018322));
#94885=CARTESIAN_POINT('Ctrl Pts',(-8.36213066678,-23.0627326652,12.2324492288));
#94886=CARTESIAN_POINT('Ctrl Pts',(-8.43792182062,-23.0327194928,12.3025271783));
#94887=CARTESIAN_POINT('Ctrl Pts',(-8.48363550117,-23.0005841899,12.4073998633));
#94888=CARTESIAN_POINT('Ctrl Pts',(-8.47259449573,-22.9739829087,12.5290848856));
#94889=CARTESIAN_POINT('Ctrl Pts',(-8.41152527253,-22.9610560938,12.6277894396));
#94890=CARTESIAN_POINT('Ctrl Pts',(-8.32640121972,-22.9690248134,12.6908033837));
#94891=CARTESIAN_POINT('Ctrl Pts',(-8.34854625295,-22.9684833924,12.2198888201));
#94892=CARTESIAN_POINT('Ctrl Pts',(-8.42693586094,-22.9542535279,12.29236935));
#94893=CARTESIAN_POINT('Ctrl Pts',(-8.47477476029,-22.9392158893,12.4011922791));
#94894=CARTESIAN_POINT('Ctrl Pts',(-8.46499990031,-22.9265127562,12.5267357874));
#94895=CARTESIAN_POINT('Ctrl Pts',(-8.40290084109,-22.9193127846,12.6268959398));
#94896=CARTESIAN_POINT('Ctrl Pts',(-8.31471092647,-22.9207536636,12.6874600337));
#94897=CARTESIAN_POINT('Ctrl Pts',(-8.34854625295,-22.8742356128,12.2198888201));
#94898=CARTESIAN_POINT('Ctrl Pts',(-8.4275605919,-22.8742356128,12.2929469882));
#94899=CARTESIAN_POINT('Ctrl Pts',(-8.47411942559,-22.8742356128,12.4014233916));
#94900=CARTESIAN_POINT('Ctrl Pts',(-8.4651120838,-22.8742356128,12.5258960706));
#94901=CARTESIAN_POINT('Ctrl Pts',(-8.40342053421,-22.8742356128,12.6265390425));
#94902=CARTESIAN_POINT('Ctrl Pts',(-8.31471092647,-22.8742356128,12.6874600337));
#94903=CARTESIAN_POINT('',(-8.58542217429,-23.1742356128,12.8474952237));
#94904=CARTESIAN_POINT('Ctrl Pts',(-8.31471092647,-22.8742356128,12.6874600337));
#94905=CARTESIAN_POINT('Ctrl Pts',(-8.31471092647,-22.9207536636,12.6874600337));
#94906=CARTESIAN_POINT('Ctrl Pts',(-8.32640121972,-22.9690248134,12.6908033837));
#94907=CARTESIAN_POINT('Ctrl Pts',(-8.34720486119,-23.0113292253,12.6980018322));
#94908=CARTESIAN_POINT('Ctrl Pts',(-8.40034769996,-23.089880852,12.7198837328));
#94909=CARTESIAN_POINT('Ctrl Pts',(-8.47363957019,-23.1456118409,12.7605886079));
#94910=CARTESIAN_POINT('Ctrl Pts',(-8.51298776904,-23.1652660131,12.7860692819));
#94911=CARTESIAN_POINT('Ctrl Pts',(-8.55126681507,-23.1742356128,12.8159145257));
#94912=CARTESIAN_POINT('Ctrl Pts',(-8.58542217429,-23.1742356128,12.8474952237));
#94913=CARTESIAN_POINT('Origin',(-8.58542217429,-23.4742356128,12.8474952237));
#94914=CARTESIAN_POINT('Origin',(-8.14487887576,-22.8742356128,12.4401604693));
#94915=CARTESIAN_POINT('',(-8.48454297717,-23.1742356128,12.9347595981));
#94916=CARTESIAN_POINT('Origin',(-8.48454297717,-22.8742356128,12.9347595981));
#94917=CARTESIAN_POINT('Origin',(-8.14487887576,-23.1742356128,12.4401604693));
#94918=CARTESIAN_POINT('Origin',(-1.05,-22.8742356128,14.92922515));
#94919=CARTESIAN_POINT('',(-1.09378792023,-23.1742356128,15.5276251985));
#94920=CARTESIAN_POINT('Origin',(-1.05,-23.1742356128,14.92922515));
#94921=CARTESIAN_POINT('Origin',(-1.09378792023,-22.8742356128,15.5276251985));
#94922=CARTESIAN_POINT('Origin',(2.71042223425E-15,-22.8742356128,0.580061096523));
#94923=CARTESIAN_POINT('Origin',(-3.80460715967E-16,-23.1742356128,0.580061096523));
#94924=CARTESIAN_POINT('Origin',(-8.21591479143,-23.4742356128,11.6886688365));
#94925=CARTESIAN_POINT('',(-7.85913400544,-23.1742356128,11.2062712093));
#94926=CARTESIAN_POINT('Origin',(-8.21591479143,-23.1742356128,11.6886688365));
#94927=CARTESIAN_POINT('Origin',(-7.85913400544,-23.4742356128,11.2062712093));
#94928=CARTESIAN_POINT('Origin',(-2.3120230745E-14,-23.4742356128,0.580061096523));
#94929=CARTESIAN_POINT('',(-8.48602987721,-23.1742356128,10.7126632105));
#94930=CARTESIAN_POINT('Origin',(8.85900795181E-16,-23.1742356128,0.580061096523));
#94931=CARTESIAN_POINT('Origin',(-8.48739188241962,-23.4721143216659,10.7142894999642));
#94932=CARTESIAN_POINT('Ctrl Pts',(-12.9732843937,-22.9031898545,8.97133867634));
#94933=CARTESIAN_POINT('Ctrl Pts',(-12.9781011914,-22.9849535816,8.94914145692));
#94934=CARTESIAN_POINT('Ctrl Pts',(-12.9535953066,-23.0667173088,8.92058122207));
#94935=CARTESIAN_POINT('Ctrl Pts',(-12.8986935104,-23.1346740075,8.88934991896));
#94936=CARTESIAN_POINT('Ctrl Pts',(-12.8237786321,-23.1759719524,8.86135389883));
#94937=CARTESIAN_POINT('Ctrl Pts',(-12.7426122303,-23.1887127298,8.84011906693));
#94938=CARTESIAN_POINT('Ctrl Pts',(-12.9823757633,-22.8915014019,8.92944287783));
#94939=CARTESIAN_POINT('Ctrl Pts',(-12.9862583246,-22.9763016188,8.91126726307));
#94940=CARTESIAN_POINT('Ctrl Pts',(-12.9595430587,-23.0611018356,8.88653324147));
#94941=CARTESIAN_POINT('Ctrl Pts',(-12.9012478152,-23.1309752745,8.85841244838));
#94942=CARTESIAN_POINT('Ctrl Pts',(-12.822883741,-23.172105454,8.83249977476));
#94943=CARTESIAN_POINT('Ctrl Pts',(-12.7392305459,-23.1828685028,8.81230742555));
#94944=CARTESIAN_POINT('Ctrl Pts',(-12.9914751666,-22.882822481,8.8868408148));
#94945=CARTESIAN_POINT('Ctrl Pts',(-12.9944056315,-22.9704026765,8.87289342313));
#94946=CARTESIAN_POINT('Ctrl Pts',(-12.9654027633,-23.0579828719,8.85218917069));
#94947=CARTESIAN_POINT('Ctrl Pts',(-12.9035898329,-23.1294730391,8.82727742946));
#94948=CARTESIAN_POINT('Ctrl Pts',(-12.8217308477,-23.1700741969,8.8033687928));
#94949=CARTESIAN_POINT('Ctrl Pts',(-12.7356821525,-23.1785290452,8.78399143876));
#94950=CARTESIAN_POINT('Ctrl Pts',(-13.000513389,-22.8770866751,8.84380834125));
#94951=CARTESIAN_POINT('Ctrl Pts',(-13.0024779758,-22.9671810863,8.834295766));
#94952=CARTESIAN_POINT('Ctrl Pts',(-12.9711165232,-23.0572754975,8.81782605389));
#94953=CARTESIAN_POINT('Ctrl Pts',(-12.9056733165,-23.1300795876,8.79620887499));
#94954=CARTESIAN_POINT('Ctrl Pts',(-12.820300204,-23.1698045819,8.77418794581));
#94955=CARTESIAN_POINT('Ctrl Pts',(-12.731982211,-23.1756611501,8.75535198255));
#94956=CARTESIAN_POINT('Ctrl Pts',(-13.0094376369,-22.8742356128,8.80057964365));
#94957=CARTESIAN_POINT('Ctrl Pts',(-13.0104250706,-22.9665621944,8.79571296462));
#94958=CARTESIAN_POINT('Ctrl Pts',(-12.97663939,-23.0588887759,8.78368803172));
#94959=CARTESIAN_POINT('Ctrl Pts',(-12.9074626588,-23.1326978759,8.76544020738));
#94960=CARTESIAN_POINT('Ctrl Pts',(-12.8185800084,-23.171217802,8.7451543519));
#94961=CARTESIAN_POINT('Ctrl Pts',(-12.728148167,-23.1742356128,8.7265439874));
#94962=CARTESIAN_POINT('Ctrl Pts',(-13.018207968,-22.8742356128,8.75735407375));
#94963=CARTESIAN_POINT('Ctrl Pts',(-13.018207968,-22.9684833924,8.75735407375));
#94964=CARTESIAN_POINT('Ctrl Pts',(-12.9819360276,-23.0627311721,8.74999461196));
#94965=CARTESIAN_POINT('Ctrl Pts',(-12.9089301686,-23.1372245963,8.73518195451));
#94966=CARTESIAN_POINT('Ctrl Pts',(-12.8165644307,-23.1742356128,8.71644123897));
#94967=CARTESIAN_POINT('Ctrl Pts',(-12.7241986928,-23.1742356128,8.69770052342));
#94968=CARTESIAN_POINT('',(-12.7426122126818,-23.1887126399569,8.84011909764617));
#94969=CARTESIAN_POINT('Origin',(-12.6820772987135,-22.9047704876882,8.9076975331626));
#94970=CARTESIAN_POINT('',(-12.7241986928,-23.1742356128,8.69770052342));
#94971=CARTESIAN_POINT('Origin',(-12.726277687684,-22.8763569532575,8.69812226440674));
#94972=CARTESIAN_POINT('Origin',(-12.6973454005032,-23.4896761342038,8.67085289361702));
#94973=CARTESIAN_POINT('Ctrl Pts',(-12.8222448424,-23.4742356815,9.46100292006));
#94974=CARTESIAN_POINT('Ctrl Pts',(-12.8494736832,-23.4742356636,9.39375104048));
#94975=CARTESIAN_POINT('Ctrl Pts',(-12.8563714436,-23.4742356458,9.31826754191));
#94976=CARTESIAN_POINT('Ctrl Pts',(-12.8394938336,-23.4742356301,9.24276446755));
#94977=CARTESIAN_POINT('Ctrl Pts',(-12.8011121316,-23.4742356188,9.17740252767));
#94978=CARTESIAN_POINT('Ctrl Pts',(-12.7478394439,-23.4742356125,9.1281455822));
#94979=CARTESIAN_POINT('Ctrl Pts',(-12.8222448265,-23.4046541603,9.4610029458));
#94980=CARTESIAN_POINT('Ctrl Pts',(-12.8494736715,-23.4136498524,9.39375106135));
#94981=CARTESIAN_POINT('Ctrl Pts',(-12.8563714358,-23.4226455445,9.31826755752));
#94982=CARTESIAN_POINT('Ctrl Pts',(-12.8394938286,-23.4305372305,9.24276447831));
#94983=CARTESIAN_POINT('Ctrl Pts',(-12.801112128,-23.4362628909,9.17740253498));
#94984=CARTESIAN_POINT('Ctrl Pts',(-12.7478394405,-23.4394448584,9.12814558784));
#94985=CARTESIAN_POINT('Ctrl Pts',(-12.8267376752,-23.3350444003,9.44989804488));
#94986=CARTESIAN_POINT('Ctrl Pts',(-12.8532287465,-23.3530402345,9.38369795688));
#94987=CARTESIAN_POINT('Ctrl Pts',(-12.8592761475,-23.3710360687,9.30931517965));
#94988=CARTESIAN_POINT('Ctrl Pts',(-12.8415116196,-23.3868230014,9.23486539817));
#94989=CARTESIAN_POINT('Ctrl Pts',(-12.8023354301,-23.3982761819,9.17041054742));
#94990=CARTESIAN_POINT('Ctrl Pts',(-12.7484601992,-23.4046400789,9.12185309334));
#94991=CARTESIAN_POINT('Ctrl Pts',(-12.8357660159,-23.2683909506,9.42765504858));
#94992=CARTESIAN_POINT('Ctrl Pts',(-12.8607726482,-23.2950473443,9.36356310571));
#94993=CARTESIAN_POINT('Ctrl Pts',(-12.8651123819,-23.3217037379,9.29138732719));
#94994=CARTESIAN_POINT('Ctrl Pts',(-12.8455698325,-23.3450683354,9.21904951484));
#94995=CARTESIAN_POINT('Ctrl Pts',(-12.8048034097,-23.3619761005,9.15641249749));
#94996=CARTESIAN_POINT('Ctrl Pts',(-12.7497239393,-23.3713130963,9.10925542748));
#94997=CARTESIAN_POINT('Ctrl Pts',(-12.8654176334,-23.1205674467,9.35093873948));
#94998=CARTESIAN_POINT('Ctrl Pts',(-12.8856609251,-23.1667016048,9.29404448239));
#94999=CARTESIAN_POINT('Ctrl Pts',(-12.88434645,-23.2128357629,9.22937157743));
#95000=CARTESIAN_POINT('Ctrl Pts',(-12.8587400955,-23.2531200257,9.16420855068));
#95001=CARTESIAN_POINT('Ctrl Pts',(-12.8124201304,-23.2819402616,9.10778516284));
#95002=CARTESIAN_POINT('Ctrl Pts',(-12.7530521925,-23.2974017916,9.06547349059));
#95003=CARTESIAN_POINT('Ctrl Pts',(-12.9068680488,-23.010101918,9.22909905079));
#95004=CARTESIAN_POINT('Ctrl Pts',(-12.9207907755,-23.0719215919,9.18344085273));
#95005=CARTESIAN_POINT('Ctrl Pts',(-12.9112658476,-23.1337412658,9.13042485238));
#95006=CARTESIAN_POINT('Ctrl Pts',(-12.8761980932,-23.187134812,9.07635129743));
#95007=CARTESIAN_POINT('Ctrl Pts',(-12.8208608743,-23.2240649689,9.02951363011));
#95008=CARTESIAN_POINT('Ctrl Pts',(-12.7544308643,-23.2421683956,8.99467312589));
#95009=CARTESIAN_POINT('Ctrl Pts',(-12.9314667335,-22.9612266295,9.14763068363));
#95010=CARTESIAN_POINT('Ctrl Pts',(-12.9418297489,-23.0307478118,9.10939417332));
#95011=CARTESIAN_POINT('Ctrl Pts',(-12.9272163182,-23.1002689941,9.06405821655));
#95012=CARTESIAN_POINT('Ctrl Pts',(-12.8858996435,-23.1597742276,9.01725069446));
#95013=CARTESIAN_POINT('Ctrl Pts',(-12.8244369644,-23.1997556874,8.97665312932));
#95014=CARTESIAN_POINT('Ctrl Pts',(-12.7531935733,-23.2177311451,8.94663366293));
#95015=CARTESIAN_POINT('Ctrl Pts',(-12.9538489501,-22.9261034781,9.0609030715));
#95016=CARTESIAN_POINT('Ctrl Pts',(-12.9611499959,-23.0022194475,9.03052977793));
#95017=CARTESIAN_POINT('Ctrl Pts',(-12.941507993,-23.078335417,8.99337186849));
#95018=CARTESIAN_POINT('Ctrl Pts',(-12.8935474744,-23.1426522193,8.95421942683));
#95019=CARTESIAN_POINT('Ctrl Pts',(-12.8254935651,-23.1840524297,8.91999612505));
#95020=CARTESIAN_POINT('Ctrl Pts',(-12.7492414901,-23.2001695455,8.89463935599));
#95021=CARTESIAN_POINT('Ctrl Pts',(-12.9732844032,-22.9031895891,8.9713386779));
#95022=CARTESIAN_POINT('Ctrl Pts',(-12.9781011912,-22.9849533577,8.94914147504));
#95023=CARTESIAN_POINT('Ctrl Pts',(-12.9535952945,-23.0667171263,8.92058125628));
#95024=CARTESIAN_POINT('Ctrl Pts',(-12.8986934857,-23.1346738584,8.88934996626));
#95025=CARTESIAN_POINT('Ctrl Pts',(-12.8237785974,-23.1759718213,8.86135395422));
#95026=CARTESIAN_POINT('Ctrl Pts',(-12.7426121901,-23.188712601,8.84011912524));
#95027=CARTESIAN_POINT('Ctrl Pts',(-12.7478394439013,-23.4742356125,9.12814558220122));
#95028=CARTESIAN_POINT('Ctrl Pts',(-12.7478394423705,-23.4585747866676,
9.12814558473974));
#95029=CARTESIAN_POINT('Ctrl Pts',(-12.7479941055707,-23.4430020566137,
9.12661399498703));
#95030=CARTESIAN_POINT('Ctrl Pts',(-12.7482793501886,-23.4277199381803,
9.12361011238638));
#95031=CARTESIAN_POINT('Ctrl Pts',(-12.7485863803035,-23.4112706512066,
9.12037680889192));
#95032=CARTESIAN_POINT('Ctrl Pts',(-12.7490439774559,-23.3951575737632,
9.11543863325741));
#95033=CARTESIAN_POINT('Ctrl Pts',(-12.7495774547234,-23.3795881719316,
9.10888164768596));
#95034=CARTESIAN_POINT('Ctrl Pts',(-12.7501402959479,-23.3631617902941,
9.10196374881271));
#95035=CARTESIAN_POINT('Ctrl Pts',(-12.7507868072288,-23.347340616678,9.09324434020817));
#95036=CARTESIAN_POINT('Ctrl Pts',(-12.7513935053284,-23.3323249264688,
9.0828266307671));
#95037=CARTESIAN_POINT('Ctrl Pts',(-12.7516567580278,-23.3258094602383,
9.07830627684944));
#95038=CARTESIAN_POINT('Ctrl Pts',(-12.7519121450063,-23.3194451133931,
9.07346616307184));
#95039=CARTESIAN_POINT('Ctrl Pts',(-12.7521482626982,-23.3132454913329,
9.06831467777211));
#95040=CARTESIAN_POINT('Ctrl Pts',(-12.7524122220315,-23.3063148454626,
9.06255575892657));
#95041=CARTESIAN_POINT('Ctrl Pts',(-12.7526520218503,-23.2995900663332,
9.05640783074764));
#95042=CARTESIAN_POINT('Ctrl Pts',(-12.7528502599117,-23.2930878600365,
9.04988322236555));
#95043=CARTESIAN_POINT('Ctrl Pts',(-12.7532355027692,-23.280451898429,9.03720372601321));
#95044=CARTESIAN_POINT('Ctrl Pts',(-12.7534629873913,-23.2686667930293,
9.02310682296249));
#95045=CARTESIAN_POINT('Ctrl Pts',(-12.7534091553356,-23.2578545455587,
9.00772645227283));
#95046=CARTESIAN_POINT('Ctrl Pts',(-12.7533534964837,-23.2466753834094,
8.99182414719493));
#95047=CARTESIAN_POINT('Ctrl Pts',(-12.7529967102063,-23.2365359417805,
8.97455013960297));
#95048=CARTESIAN_POINT('Ctrl Pts',(-12.7522140218396,-23.2275144867261,
8.95606210733663));
#95049=CARTESIAN_POINT('Ctrl Pts',(-12.7513879506109,-23.2179929903313,
8.93654932015219));
#95050=CARTESIAN_POINT('Ctrl Pts',(-12.7500865167735,-23.2097159112915,
8.91568541081658));
#95051=CARTESIAN_POINT('Ctrl Pts',(-12.7481861664673,-23.2027216494298,
8.89365486866089));
#95052=CARTESIAN_POINT('Ctrl Pts',(-12.7467056778765,-23.197272693596,8.87649173499866));
#95053=CARTESIAN_POINT('Ctrl Pts',(-12.7448619117108,-23.1926006117108,
8.85862103845975));
#95054=CARTESIAN_POINT('Ctrl Pts',(-12.7426122052017,-23.1887125986295,
8.84011912919091));
#95055=CARTESIAN_POINT('Origin',(-6.6707290414,-23.4742356128,3.1005467775));
#95056=CARTESIAN_POINT('',(-11.9421544921,-23.1742356128,7.97460750747));
#95057=CARTESIAN_POINT('',(-12.3331765925,-23.1742356128,8.33615401544));
#95058=CARTESIAN_POINT('Origin',(-11.9407143760008,-23.4721143158025,7.97616506106996));
#95059=CARTESIAN_POINT('Ctrl Pts',(-3.81744045688,-22.8742356128,-9.21387212773));
#95060=CARTESIAN_POINT('Ctrl Pts',(-3.81744045688,-22.9684833924,-9.21387212773));
#95061=CARTESIAN_POINT('Ctrl Pts',(-3.80220506528,-23.0627311721,-9.18014234586));
#95062=CARTESIAN_POINT('Ctrl Pts',(-3.77154023633,-23.1372245963,-9.11225318231));
#95063=CARTESIAN_POINT('Ctrl Pts',(-3.73274363021,-23.1742356128,-9.02636099807));
#95064=CARTESIAN_POINT('Ctrl Pts',(-3.69394702409,-23.1742356128,-8.94046881382));
#95065=CARTESIAN_POINT('Ctrl Pts',(-3.71160470889,-22.8742356128,-9.26167703413));
#95066=CARTESIAN_POINT('Ctrl Pts',(-3.72515638761,-22.9642074605,-9.25555588183));
#95067=CARTESIAN_POINT('Ctrl Pts',(-3.7250970863,-23.0541793081,-9.21865622161));
#95068=CARTESIAN_POINT('Ctrl Pts',(-3.70844285493,-23.1271496569,-9.15193510136));
#95069=CARTESIAN_POINT('Ctrl Pts',(-3.67843010495,-23.1675189946,-9.06966143177));
#95070=CARTESIAN_POINT('Ctrl Pts',(-3.64200986566,-23.1742356128,-8.98738776219));
#95071=CARTESIAN_POINT('Ctrl Pts',(-3.60518947181,-22.8967702026,-9.30860522068));
#95072=CARTESIAN_POINT('Ctrl Pts',(-3.63104913481,-22.9796757788,-9.29721692608));
#95073=CARTESIAN_POINT('Ctrl Pts',(-3.64474315,-23.0625813551,-9.25775017492));
#95074=CARTESIAN_POINT('Ctrl Pts',(-3.64141126432,-23.131420749,-9.19204052568));
#95075=CARTESIAN_POINT('Ctrl Pts',(-3.62129881914,-23.1730680404,-9.11274337915));
#95076=CARTESIAN_POINT('Ctrl Pts',(-3.58978817426,-23.1855028319,-9.03344623294));
#95077=CARTESIAN_POINT('Ctrl Pts',(-3.50276689342,-22.9419634255,-9.35255588844));
#95078=CARTESIAN_POINT('Ctrl Pts',(-3.53957219131,-23.0156863099,-9.33675316789));
#95079=CARTESIAN_POINT('Ctrl Pts',(-3.56543990858,-23.0894091943,-9.29523917398));
#95080=CARTESIAN_POINT('Ctrl Pts',(-3.57431565494,-23.1517903264,-9.2303724476));
#95081=CARTESIAN_POINT('Ctrl Pts',(-3.56438630978,-23.1921341626,-9.15347743429));
#95082=CARTESIAN_POINT('Ctrl Pts',(-3.53952573637,-23.2081001313,-9.07658241785));
#95083=CARTESIAN_POINT('Ctrl Pts',(-3.34853990601,-23.0590627588,-9.41717252271));
#95084=CARTESIAN_POINT('Ctrl Pts',(-3.40101481294,-23.1138397009,-9.39536923091));
#95085=CARTESIAN_POINT('Ctrl Pts',(-3.44422712818,-23.1686166429,-9.35116723508));
#95086=CARTESIAN_POINT('Ctrl Pts',(-3.47088045966,-23.2161685094,-9.28743732801));
#95087=CARTESIAN_POINT('Ctrl Pts',(-3.47682492232,-23.2495777226,-9.21371939274));
#95088=CARTESIAN_POINT('Ctrl Pts',(-3.4638420321,-23.2666487717,-9.14000145959));
#95089=CARTESIAN_POINT('Ctrl Pts',(-3.24903060406,-23.2324009559,-9.45772855228));
#95090=CARTESIAN_POINT('Ctrl Pts',(-3.31106586193,-23.2635682408,-9.43250094395));
#95091=CARTESIAN_POINT('Ctrl Pts',(-3.36479660614,-23.2947355258,-9.38683384758));
#95092=CARTESIAN_POINT('Ctrl Pts',(-3.40250113652,-23.322122922,-9.32374506153));
#95093=CARTESIAN_POINT('Ctrl Pts',(-3.41904507547,-23.3420909713,-9.25177549042));
#95094=CARTESIAN_POINT('Ctrl Pts',(-3.41500902577,-23.3533185645,-9.17980591789));
#95095=CARTESIAN_POINT('Ctrl Pts',(-3.22037852073,-23.3101536719,-9.46927274181));
#95096=CARTESIAN_POINT('Ctrl Pts',(-3.28511942878,-23.331162522,-9.44310189027));
#95097=CARTESIAN_POINT('Ctrl Pts',(-3.34181908965,-23.3521713721,-9.39703707137));
#95098=CARTESIAN_POINT('Ctrl Pts',(-3.38266593906,-23.3706950509,-9.33412380265));
#95099=CARTESIAN_POINT('Ctrl Pts',(-3.40228901679,-23.384336583,-9.2626299648));
#95100=CARTESIAN_POINT('Ctrl Pts',(-3.40094883361,-23.3921942807,-9.19113612813));
#95101=CARTESIAN_POINT('Ctrl Pts',(-3.2061108834,-23.3922234913,-9.47502541989));
#95102=CARTESIAN_POINT('Ctrl Pts',(-3.27219964976,-23.4027249383,-9.44838409371));
#95103=CARTESIAN_POINT('Ctrl Pts',(-3.33037855145,-23.4132263854,-9.4021208728));
#95104=CARTESIAN_POINT('Ctrl Pts',(-3.37279084839,-23.422485337,-9.33929519246));
#95105=CARTESIAN_POINT('Ctrl Pts',(-3.393947035,-23.4293033961,-9.26803870195));
#95106=CARTESIAN_POINT('Ctrl Pts',(-3.39394702816,-23.4332296702,-9.19678221123));
#95107=CARTESIAN_POINT('Ctrl Pts',(-3.20611087388,-23.4742356128,-9.47502544833));
#95108=CARTESIAN_POINT('Ctrl Pts',(-3.27219964627,-23.4742356465,-9.44838411889));
#95109=CARTESIAN_POINT('Ctrl Pts',(-3.33037855462,-23.4742356801,-9.40212089616));
#95110=CARTESIAN_POINT('Ctrl Pts',(-3.37279085872,-23.4742357098,-9.33929521563));
#95111=CARTESIAN_POINT('Ctrl Pts',(-3.39394705252,-23.4742357316,-9.26803872592));
#95112=CARTESIAN_POINT('Ctrl Pts',(-3.39394705213,-23.4742357442,-9.19678223621));
#95113=CARTESIAN_POINT('',(-3.69394702409,-23.1742356128,-8.94046881382));
#95114=CARTESIAN_POINT('Origin',(-3.69482026935181,-22.8763568962883,-8.94240201772957));
#95115=CARTESIAN_POINT('Ctrl Pts',(-3.69394702409,-23.1742356128,-8.94046881382));
#95116=CARTESIAN_POINT('Ctrl Pts',(-3.67899884906695,-23.1742356128,-8.95397268413816));
#95117=CARTESIAN_POINT('Ctrl Pts',(-3.66455031612627,-23.175353499792,-8.96691364760397));
#95118=CARTESIAN_POINT('Ctrl Pts',(-3.65070330540787,-23.1773700763482,
-8.97922431578443));
#95119=CARTESIAN_POINT('Ctrl Pts',(-3.63641423969004,-23.1794510305355,
-8.99192799242906));
#95120=CARTESIAN_POINT('Ctrl Pts',(-3.62276587287881,-23.1824896811564,
-9.0039606699122));
#95121=CARTESIAN_POINT('Ctrl Pts',(-3.60983308751173,-23.1862642542778,
-9.01528450778334));
#95122=CARTESIAN_POINT('Ctrl Pts',(-3.59620581883196,-23.1902415198566,
-9.02721642939002));
#95123=CARTESIAN_POINT('Ctrl Pts',(-3.58337317073403,-23.1950359774261,
-9.03836150991428));
#95124=CARTESIAN_POINT('Ctrl Pts',(-3.5713794826881,-23.2004026426052,-9.04871270075273));
#95125=CARTESIAN_POINT('Ctrl Pts',(-3.55873745080754,-23.2060594140692,
-9.05962344681185));
#95126=CARTESIAN_POINT('Ctrl Pts',(-3.54702870580604,-23.2123510615671,
-9.0696513765444));
#95127=CARTESIAN_POINT('Ctrl Pts',(-3.53625798419655,-23.2190072933907,
-9.07882473415894));
#95128=CARTESIAN_POINT('Ctrl Pts',(-3.52548726258705,-23.2256635252143,
-9.08799809177348));
#95129=CARTESIAN_POINT('Ctrl Pts',(-3.51565445515374,-23.2326833770868,
-9.09631707780529));
#95130=CARTESIAN_POINT('Ctrl Pts',(-3.50671897808822,-23.2398231608574,
-9.1038423601356));
#95131=CARTESIAN_POINT('Ctrl Pts',(-3.50370542903012,-23.242231100411,-9.10638031164196));
#95132=CARTESIAN_POINT('Ctrl Pts',(-3.50079412602067,-23.2446525516423,
-9.1088296778814));
#95133=CARTESIAN_POINT('Ctrl Pts',(-3.49798326952153,-23.2470782891206,
-9.11119791470152));
#95134=CARTESIAN_POINT('Ctrl Pts',(-3.49657784127196,-23.2482911578598,
-9.11238203311158));
#95135=CARTESIAN_POINT('Ctrl Pts',(-3.49553564848842,-23.249208117903,-9.11325991246051));
#95136=CARTESIAN_POINT('Ctrl Pts',(-3.49434510622956,-23.2502694936275,
-9.11426032900786));
#95137=CARTESIAN_POINT('Ctrl Pts',(-3.4932901731775,-23.2512099729124,-9.11514679269596));
#95138=CARTESIAN_POINT('Ctrl Pts',(-3.49211846283781,-23.2522635690391,
-9.11612972241234));
#95139=CARTESIAN_POINT('Ctrl Pts',(-3.49049264692078,-23.2537643261086,
-9.11749010669963));
#95140=CARTESIAN_POINT('Ctrl Pts',(-3.4902836520405,-23.253957244963,-9.11766498095708));
#95141=CARTESIAN_POINT('Ctrl Pts',(-3.49006718960407,-23.2541576045751,
-9.11784605897054));
#95142=CARTESIAN_POINT('Ctrl Pts',(-3.489842580416,-23.2543661668826,-9.11803390325523));
#95143=CARTESIAN_POINT('Ctrl Pts',(-3.47856184707405,-23.264840964448,-9.12746816239441));
#95144=CARTESIAN_POINT('Ctrl Pts',(-3.46818823610973,-23.2760891770451,
-9.13608324636035));
#95145=CARTESIAN_POINT('Ctrl Pts',(-3.4587908077671,-23.2879520814553,-9.14385003815369));
#95146=CARTESIAN_POINT('Ctrl Pts',(-3.44763144110507,-23.3020391800917,
-9.15307303770734));
#95147=CARTESIAN_POINT('Ctrl Pts',(-3.43785049160989,-23.3169954292007,
-9.16109877651924));
#95148=CARTESIAN_POINT('Ctrl Pts',(-3.42952044756393,-23.3325442547886,
-9.16790677016603));
#95149=CARTESIAN_POINT('Ctrl Pts',(-3.42150473969357,-23.3475063417778,
-9.17445786256781));
#95150=CARTESIAN_POINT('Ctrl Pts',(-3.41483311376225,-23.363015262272,-9.17988102525593));
#95151=CARTESIAN_POINT('Ctrl Pts',(-3.40953111081634,-23.3788158559842,
-9.18418102289095));
#95152=CARTESIAN_POINT('Ctrl Pts',(-3.40427986614197,-23.3944651840644,
-9.18843985486654));
#95153=CARTESIAN_POINT('Ctrl Pts',(-3.40037230162103,-23.4104000145971,
-9.19159685104193));
#95154=CARTESIAN_POINT('Ctrl Pts',(-3.3977890626441,-23.4263809625103,-9.19368246110308));
#95155=CARTESIAN_POINT('Ctrl Pts',(-3.39520582366718,-23.4423619104235,
-9.19576807116422));
#95156=CARTESIAN_POINT('Ctrl Pts',(-3.3939470498033,-23.4583889758006,-9.19678222096313));
#95157=CARTESIAN_POINT('Ctrl Pts',(-3.39394705212995,-23.4742356127999,
-9.1967822362099));
#95158=CARTESIAN_POINT('Origin',(-3.69394702409,-23.4742356128,3.39628270998));
#95159=CARTESIAN_POINT('',(-3.69394702409,-23.1742356128,-8.44362980932));
#95160=CARTESIAN_POINT('Ctrl Pts',(-9.06991786197,-22.8742351711,13.3798726472));
#95161=CARTESIAN_POINT('Ctrl Pts',(-9.06991791346,-22.9684830268,13.3798726085));
#95162=CARTESIAN_POINT('Ctrl Pts',(-9.04851963512,-23.0627308825,13.3496744364));
#95163=CARTESIAN_POINT('Ctrl Pts',(-9.00545047601,-23.1372243637,13.2888935201));
#95164=CARTESIAN_POINT('Ctrl Pts',(-8.95096009845,-23.1742354012,13.2119945921));
#95165=CARTESIAN_POINT('Ctrl Pts',(-8.89646970336,-23.1742353894,13.1350956831));
#95166=CARTESIAN_POINT('Ctrl Pts',(-9.22406041417,-22.8742363569,13.2706476151));
#95167=CARTESIAN_POINT('Ctrl Pts',(-9.20132424908,-22.9647386701,13.2867584141));
#95168=CARTESIAN_POINT('Ctrl Pts',(-9.15852680885,-23.0552409834,13.275328887));
#95169=CARTESIAN_POINT('Ctrl Pts',(-9.10021479707,-23.128400233,13.232683254));
#95170=CARTESIAN_POINT('Ctrl Pts',(-9.0393710411,-23.168352818,13.1677082076));
#95171=CARTESIAN_POINT('Ctrl Pts',(-8.986120014,-23.1742360128,13.0945214235));
#95172=CARTESIAN_POINT('Ctrl Pts',(-9.3768173424,-22.9427255764,13.1589191215));
#95173=CARTESIAN_POINT('Ctrl Pts',(-9.33383370545,-23.019699187,13.1904054535));
#95174=CARTESIAN_POINT('Ctrl Pts',(-9.27188264132,-23.0966727976,13.1965141601));
#95175=CARTESIAN_POINT('Ctrl Pts',(-9.19881019143,-23.1602830893,13.1710975036));
#95176=CARTESIAN_POINT('Ctrl Pts',(-9.1296041316,-23.1981089887,13.1188723071));
#95177=CARTESIAN_POINT('Ctrl Pts',(-9.07411181992,-23.2084805514,13.051815332));
#95178=CARTESIAN_POINT('Ctrl Pts',(-9.5056235281,-23.0835945845,13.0599834668));
#95179=CARTESIAN_POINT('Ctrl Pts',(-9.44694848687,-23.1391655975,13.1046059873));
#95180=CARTESIAN_POINT('Ctrl Pts',(-9.36995382261,-23.1947366105,13.1251829804));
#95181=CARTESIAN_POINT('Ctrl Pts',(-9.2844923694,-23.2410848235,13.113878162));
#95182=CARTESIAN_POINT('Ctrl Pts',(-9.20688851793,-23.2696054116,13.0728111063));
#95183=CARTESIAN_POINT('Ctrl Pts',(-9.14715364651,-23.2789180606,13.0124182766));
#95184=CARTESIAN_POINT('Ctrl Pts',(-9.57074430825,-23.2789184576,13.0098414435));
#95185=CARTESIAN_POINT('Ctrl Pts',(-9.50407307406,-23.3067030636,13.0611772932));
#95186=CARTESIAN_POINT('Ctrl Pts',(-9.41940322383,-23.3344876695,13.0891378612));
#95187=CARTESIAN_POINT('Ctrl Pts',(-9.32764499777,-23.3576610293,13.0850021715));
#95188=CARTESIAN_POINT('Ctrl Pts',(-9.2458338001,-23.3719208617,13.049538037));
#95189=CARTESIAN_POINT('Ctrl Pts',(-9.18405109086,-23.3765770352,12.9924125631));
#95190=CARTESIAN_POINT('Ctrl Pts',(-9.57074430825,-23.4742356128,13.0098414435));
#95191=CARTESIAN_POINT('Ctrl Pts',(-9.50407307406,-23.4742356128,13.0611772932));
#95192=CARTESIAN_POINT('Ctrl Pts',(-9.41940322382,-23.4742356128,13.0891378611));
#95193=CARTESIAN_POINT('Ctrl Pts',(-9.32764499778,-23.4742356128,13.0850021715));
#95194=CARTESIAN_POINT('Ctrl Pts',(-9.2458338001,-23.4742356128,13.049538037));
#95195=CARTESIAN_POINT('Ctrl Pts',(-9.18405109086,-23.4742356128,12.9924125631));
#95196=CARTESIAN_POINT('',(-8.89646969686788,-23.17423555695,13.1350956958597));
#95197=CARTESIAN_POINT('Origin',(-8.89769520903801,-22.8763558982741,13.1368257591445));
#95198=CARTESIAN_POINT('Ctrl Pts',(-8.89646970862946,-23.1742353894,13.1350956905365));
#95199=CARTESIAN_POINT('Ctrl Pts',(-8.91309680047625,-23.1742355049141,
13.1275705378248));
#95200=CARTESIAN_POINT('Ctrl Pts',(-8.92916239855924,-23.1756511702746,
13.120179101675));
#95201=CARTESIAN_POINT('Ctrl Pts',(-8.94451183302731,-23.1782464117074,
13.1130138149001));
#95202=CARTESIAN_POINT('Ctrl Pts',(-8.95958315050042,-23.1807946298606,
13.1059783562325));
#95203=CARTESIAN_POINT('Ctrl Pts',(-8.97396381020449,-23.1844790085148,
13.0991617725664));
#95204=CARTESIAN_POINT('Ctrl Pts',(-8.98755390972639,-23.189062385306,13.0926394475502));
#95205=CARTESIAN_POINT('Ctrl Pts',(-8.99701199211221,-23.1922522041315,
13.0881002101994));
#95206=CARTESIAN_POINT('Ctrl Pts',(-9.00608818080905,-23.1958771858743,
13.0837031896146));
#95207=CARTESIAN_POINT('Ctrl Pts',(-9.01476254474212,-23.1998570495597,
13.079467854496));
#95208=CARTESIAN_POINT('Ctrl Pts',(-9.027482024044,-23.2056928427269,13.0732574559246));
#95209=CARTESIAN_POINT('Ctrl Pts',(-9.03934274711023,-23.212293430192,13.0673924478358));
#95210=CARTESIAN_POINT('Ctrl Pts',(-9.05033294399465,-23.2194260101855,
13.0619070683858));
#95211=CARTESIAN_POINT('Ctrl Pts',(-9.05395907702327,-23.2217793514555,
13.0600972085801));
#95212=CARTESIAN_POINT('Ctrl Pts',(-9.05749078373108,-23.2241907687581,
13.0583284758369));
#95213=CARTESIAN_POINT('Ctrl Pts',(-9.06092859580915,-23.2266524199078,
13.0566015206519));
#95214=CARTESIAN_POINT('Ctrl Pts',(-9.06785721579022,-23.2316136699572,
13.0531209882874));
#95215=CARTESIAN_POINT('Ctrl Pts',(-9.07440401191121,-23.2367786623744,
13.0498105322997));
#95216=CARTESIAN_POINT('Ctrl Pts',(-9.08059335916827,-23.2420847942466,
13.0466889651196));
#95217=CARTESIAN_POINT('Ctrl Pts',(-9.0836880327968,-23.2447378601827,13.0451281815295));
#95218=CARTESIAN_POINT('Ctrl Pts',(-9.08668953155372,-23.247426726068,13.0436101398472));
#95219=CARTESIAN_POINT('Ctrl Pts',(-9.08959773920902,-23.2501447149073,
13.0421324470578));
#95220=CARTESIAN_POINT('Ctrl Pts',(-9.09117417163362,-23.2516180367067,
13.0413314441367));
#95221=CARTESIAN_POINT('Ctrl Pts',(-9.09249083656084,-23.2528771175428,
13.0406611989853));
#95222=CARTESIAN_POINT('Ctrl Pts',(-9.09392855283527,-23.2542797644668,
13.0399269440846));
#95223=CARTESIAN_POINT('Ctrl Pts',(-9.09514314021191,-23.2554647251424,
13.0393066431604));
#95224=CARTESIAN_POINT('Ctrl Pts',(-9.09644407818803,-23.2567523375043,
13.0386406609476));
#95225=CARTESIAN_POINT('Ctrl Pts',(-9.09804347097728,-23.2583792358661,
13.037819360047));
#95226=CARTESIAN_POINT('Ctrl Pts',(-9.11048146896409,-23.2710311364403,
13.0314323492911));
#95227=CARTESIAN_POINT('Ctrl Pts',(-9.12170996655921,-23.284815934694,13.0255917484038));
#95228=CARTESIAN_POINT('Ctrl Pts',(-9.13160827419955,-23.2994894912599,
13.0204003640024));
#95229=CARTESIAN_POINT('Ctrl Pts',(-9.14140778591686,-23.3140165897021,
13.0152607952883));
#95230=CARTESIAN_POINT('Ctrl Pts',(-9.14990355505978,-23.3294146670775,
13.0107577262315));
#95231=CARTESIAN_POINT('Ctrl Pts',(-9.15701840945915,-23.3454289145785,
13.0069645198718));
#95232=CARTESIAN_POINT('Ctrl Pts',(-9.16410040151333,-23.3613691948975,
13.0031888337099));
#95233=CARTESIAN_POINT('Ctrl Pts',(-9.16981423379896,-23.377919961051,13.0001165870717));
#95234=CARTESIAN_POINT('Ctrl Pts',(-9.17412316825768,-23.3948130306609,
12.9977916560662));
#95235=CARTESIAN_POINT('Ctrl Pts',(-9.17839082006171,-23.4115442526573,
12.9954889995522));
#95236=CARTESIAN_POINT('Ctrl Pts',(-9.18128041821572,-23.4286113244906,
12.9939194681916));
#95237=CARTESIAN_POINT('Ctrl Pts',(-9.18279429024485,-23.4457365917114,
12.9930964360048));
#95238=CARTESIAN_POINT('Ctrl Pts',(-9.18363397469894,-23.4552352946272,
12.9926399328664));
#95239=CARTESIAN_POINT('Ctrl Pts',(-9.18405109086,-23.4647515930551,12.9924125631));
#95240=CARTESIAN_POINT('Ctrl Pts',(-9.18405109086,-23.4742356128,12.9924125631));
#95241=CARTESIAN_POINT('Origin',(-6.6707290414,-23.4742356128,11.0771333555));
#95242=CARTESIAN_POINT('',(-8.74094594938,-23.1742356128,12.9912954789));
#95243=CARTESIAN_POINT('Origin',(2.84607155346,-22.8742356128,5.53854202767));
#95244=CARTESIAN_POINT('Origin',(2.84607155346,-23.1742356128,5.53854202767));
#95245=CARTESIAN_POINT('Origin',(4.58869751468E-17,-22.8742356128,0.580061096523));
#95246=CARTESIAN_POINT('Origin',(-7.30083966106E-16,-23.1742356128,0.580061096523));
#95247=CARTESIAN_POINT('Origin',(-3.23631964477E-15,-23.0742356128,-4.23765442876));
#95248=CARTESIAN_POINT('',(0.153073372946,-23.1742356128,-4.17424936164));
#95249=CARTESIAN_POINT('Origin',(0.153073372946,-23.0742356128,-4.17424936164));
#95250=CARTESIAN_POINT('',(3.35920145722,-23.1742356128,-2.84622762644));
#95251=CARTESIAN_POINT('',(1.75613741508,-23.1742356128,-3.51023849404));
#95252=CARTESIAN_POINT('Origin',(3.35920145722,-23.0742356128,-2.84622762644));
#95253=CARTESIAN_POINT('Origin',(-2.06825793744E-15,-23.0742356128,5.69655897044));
#95254=CARTESIAN_POINT('',(0.153073372946,-23.1742356128,5.63315390332));
#95255=CARTESIAN_POINT('',(1.7388152851,-23.1742356128,4.97631809688));
#95256=CARTESIAN_POINT('Origin',(0.153073372946,-23.0742356128,5.63315390332));
#95257=CARTESIAN_POINT('Origin',(3.81389112164,-23.0742356128,3.51356095948));
#95258=CARTESIAN_POINT('',(4.23969076488,-23.1742356128,2.48558968592));
#95259=CARTESIAN_POINT('Origin',(6.12032227755,-23.0742356128,3.51356095948));
#95260=CARTESIAN_POINT('',(3.57567989727,-23.1742356128,-2.62974918638));
#95261=CARTESIAN_POINT('Origin',(3.57567989727,-23.0742356128,-2.62974918638));
#95262=CARTESIAN_POINT('',(4.23277615087,-23.1742356128,-1.04337849916));
#95263=CARTESIAN_POINT('Origin',(3.20612808427,-23.0742356128,-2.47667581343));
#95264=CARTESIAN_POINT('Origin',(3.20612808427,-23.1742356128,-2.47667581343));
#95265=CARTESIAN_POINT('Origin',(1.12255033962E-15,-23.0742356128,-3.80469754864));
#95266=CARTESIAN_POINT('',(-0.153073372946,-23.1742356128,-4.17424936164));
#95267=CARTESIAN_POINT('Origin',(-0.153073372946,-23.0742356128,-4.17424936164));
#95268=CARTESIAN_POINT('Origin',(1.11225582468E-15,-23.1742356128,-3.80469754864));
#95269=CARTESIAN_POINT('Origin',(-1.45996280537E-15,-23.0742356128,-4.23765442876));
#95270=CARTESIAN_POINT('',(-3.35920145722,-23.1742356128,-2.84622762644));
#95271=CARTESIAN_POINT('Origin',(-3.35920145722,-23.0742356128,-2.84622762644));
#95272=CARTESIAN_POINT('',(-1.75613741508,-23.1742356128,-3.51023849404));
#95273=CARTESIAN_POINT('Origin',(-1.5436783271E-16,-23.0742356128,5.26360209032));
#95274=CARTESIAN_POINT('',(-0.153073372946,-23.1742356128,5.63315390332));
#95275=CARTESIAN_POINT('Origin',(-2.77636603164E-16,-23.1742356128,5.26360209032));
#95276=CARTESIAN_POINT('Origin',(-0.153073372946,-23.0742356128,5.63315390332));
#95277=CARTESIAN_POINT('Origin',(-2.06825793744E-15,-23.0742356128,5.69655897044));
#95278=CARTESIAN_POINT('',(-1.7388152851,-23.1742356128,4.97631809688));
#95279=CARTESIAN_POINT('Origin',(-3.81389112164,-23.0742356128,3.51356095948));
#95280=CARTESIAN_POINT('',(-4.23969076488,-23.1742356128,2.48558968592));
#95281=CARTESIAN_POINT('Origin',(-6.12032227755,-23.0742356128,3.51356095948));
#95282=CARTESIAN_POINT('',(-3.57567989727,-23.1742356128,-2.62974918638));
#95283=CARTESIAN_POINT('',(-4.23277615087,-23.1742356128,-1.04337849916));
#95284=CARTESIAN_POINT('Origin',(-3.57567989727,-23.0742356128,-2.62974918638));
#95285=CARTESIAN_POINT('Origin',(-3.20612808427,-23.0742356128,-2.47667581343));
#95286=CARTESIAN_POINT('Origin',(-3.20612808427,-23.1742356128,-2.47667581343));
#95287=CARTESIAN_POINT('Origin',(0.,-23.1742356128,0.729452270839));
#95288=CARTESIAN_POINT('',(-6.06355150788,-23.1742356128,8.47279340685));
#95289=CARTESIAN_POINT('',(-6.6707290414,-23.1742356128,9.03420135995));
#95290=CARTESIAN_POINT('',(-5.99440665492,-23.1742356128,7.66760345225));
#95291=CARTESIAN_POINT('Origin',(-6.47088626226,-23.1742356128,8.03225010833));
#95292=CARTESIAN_POINT('',(-7.50515696478,-23.1742356128,3.88262115182));
#95293=CARTESIAN_POINT('Origin',(-0.00234331738835,-23.1742356128,3.08191746407));
#95294=CARTESIAN_POINT('',(-8.10176909975,-23.1742356128,3.34629187045));
#95295=CARTESIAN_POINT('Origin',(-8.10176909975,-23.1742356128,3.94629187045));
#95296=CARTESIAN_POINT('',(-11.4530804658,-23.1742356128,3.34629187045));
#95297=CARTESIAN_POINT('',(-6.6707290414,-23.1742356128,3.34629187045));
#95298=CARTESIAN_POINT('',(-12.0493948734,-23.1742356128,3.87989061057));
#95299=CARTESIAN_POINT('Origin',(-11.4530804658,-23.1742356128,3.94629187045));
#95300=CARTESIAN_POINT('Origin',(2.84607155346,-23.1742356128,5.53854202767));
#95301=CARTESIAN_POINT('Origin',(-10.1862176145,-22.8742356128,9.72278707155));
#95302=CARTESIAN_POINT('',(-10.9304145503,-22.8742356128,10.3907473403));
#95303=CARTESIAN_POINT('',(-11.1383462684,-22.8742356128,10.0284846777));
#95304=CARTESIAN_POINT('Origin',(-10.1862176145,-22.8742356128,9.72278707155));
#95305=CARTESIAN_POINT('Ctrl Pts',(-10.9304145503437,-22.8742356128,10.3907473403392));
#95306=CARTESIAN_POINT('Ctrl Pts',(-10.9481405479233,-22.8882672659973,
10.3709982119854));
#95307=CARTESIAN_POINT('Ctrl Pts',(-10.9645717766644,-22.9013026990597,
10.3525880372788));
#95308=CARTESIAN_POINT('Ctrl Pts',(-10.9810103536057,-22.9142753573368,
10.3340804995609));
#95309=CARTESIAN_POINT('Ctrl Pts',(-10.992000443497,-22.9229482905903,10.3217071959644));
#95310=CARTESIAN_POINT('Ctrl Pts',(-11.002992272732,-22.9315950772944,10.3092917362859));
#95311=CARTESIAN_POINT('Ctrl Pts',(-11.0143770648586,-22.9404798718002,
10.2963873039649));
#95312=CARTESIAN_POINT('Ctrl Pts',(-11.0200212309283,-22.944884629931,10.2899897555297));
#95313=CARTESIAN_POINT('Ctrl Pts',(-11.0257621179678,-22.9493475068719,
10.2834716325873));
#95314=CARTESIAN_POINT('Ctrl Pts',(-11.031648508022,-22.9538972342928,10.2767748704144));
#95315=CARTESIAN_POINT('Ctrl Pts',(-11.138346268408,-22.8742356128,10.0284846777026));
#95316=CARTESIAN_POINT('Ctrl Pts',(-11.1304025349713,-22.8879754443996,
10.0532263049571));
#95317=CARTESIAN_POINT('Ctrl Pts',(-11.1227115500163,-22.9011602400043,
10.0769601464436));
#95318=CARTESIAN_POINT('Ctrl Pts',(-11.1149362788915,-22.9142785484054,
10.1007522253721));
#95319=CARTESIAN_POINT('Ctrl Pts',(-11.1089402979403,-22.9243948679554,
10.1190997337428));
#95320=CARTESIAN_POINT('Ctrl Pts',(-11.1028949842124,-22.9344737618983,
10.1374798306995));
#95321=CARTESIAN_POINT('Ctrl Pts',(-11.0966317645807,-22.9447233863069,
10.1563922783035));
#95322=CARTESIAN_POINT('Ctrl Pts',(-11.0947731720942,-22.947764932993,10.1620044929607));
#95323=CARTESIAN_POINT('Ctrl Pts',(-11.0928952369663,-22.9508212969781,
10.1676637551768));
#95324=CARTESIAN_POINT('Ctrl Pts',(-11.090993057621,-22.9538972342935,10.1733836478105));
#95325=CARTESIAN_POINT('Ctrl Pts',(-11.9005548436,-23.1693861532,7.89557218486));
#95326=CARTESIAN_POINT('Ctrl Pts',(-11.8339499555,-23.1595472711,7.96980237474));
#95327=CARTESIAN_POINT('Ctrl Pts',(-11.7599452826,-23.1908783468,8.04284981847));
#95328=CARTESIAN_POINT('Ctrl Pts',(-11.6942870876,-23.2663663442,8.09701806802));
#95329=CARTESIAN_POINT('Ctrl Pts',(-11.6548578916,-23.3654515188,8.11755397837));
#95330=CARTESIAN_POINT('Ctrl Pts',(-11.6438378503,-23.4645366935,8.10736463748));
#95331=CARTESIAN_POINT('Ctrl Pts',(-11.8668157199,-23.1614761236,7.83132058431));
#95332=CARTESIAN_POINT('Ctrl Pts',(-11.8129234492,-23.1460753827,7.92069454621));
#95333=CARTESIAN_POINT('Ctrl Pts',(-11.7451516804,-23.1734640687,8.00787961054));
#95334=CARTESIAN_POINT('Ctrl Pts',(-11.6772007057,-23.2482114783,8.07033400293));
#95335=CARTESIAN_POINT('Ctrl Pts',(-11.6288782137,-23.3484640563,8.08997448939));
#95336=CARTESIAN_POINT('Ctrl Pts',(-11.6054955414,-23.4487166343,8.07191260584));
#95337=CARTESIAN_POINT('Ctrl Pts',(-11.8201190291,-23.1436931675,7.77911937176));
#95338=CARTESIAN_POINT('Ctrl Pts',(-11.7896480761,-23.1271929291,7.88233980762));
#95339=CARTESIAN_POINT('Ctrl Pts',(-11.7361184989,-23.1516755686,7.98200912796));
#95340=CARTESIAN_POINT('Ctrl Pts',(-11.6667987778,-23.2222222498,8.05091722103));
#95341=CARTESIAN_POINT('Ctrl Pts',(-11.6024958012,-23.3176864267,8.06826984747));
#95342=CARTESIAN_POINT('Ctrl Pts',(-11.5554237252,-23.4131506081,8.04186749464));
#95343=CARTESIAN_POINT('Ctrl Pts',(-11.7752729456,-23.1083028984,7.76843597189));
#95344=CARTESIAN_POINT('Ctrl Pts',(-11.7595402729,-23.1052304081,7.86585583205));
#95345=CARTESIAN_POINT('Ctrl Pts',(-11.7167014673,-23.1327309513,7.95914759566));
#95346=CARTESIAN_POINT('Ctrl Pts',(-11.6496136328,-23.1915820263,8.02617572742));
#95347=CARTESIAN_POINT('Ctrl Pts',(-11.5756983226,-23.2669761984,8.04953640203));
#95348=CARTESIAN_POINT('Ctrl Pts',(-11.5102889752,-23.3423703627,8.03319245204));
#95349=CARTESIAN_POINT('Ctrl Pts',(-11.717675025,-23.0445100599,7.76252036052));
#95350=CARTESIAN_POINT('Ctrl Pts',(-11.7084114695,-23.0501289834,7.8515782493));
#95351=CARTESIAN_POINT('Ctrl Pts',(-11.6708968566,-23.0738598269,7.93631728547));
#95352=CARTESIAN_POINT('Ctrl Pts',(-11.6066799831,-23.1148476696,8.0001560579));
#95353=CARTESIAN_POINT('Ctrl Pts',(-11.5292674801,-23.1648160129,8.02969505599));
#95354=CARTESIAN_POINT('Ctrl Pts',(-11.4529027709,-23.2147843626,8.02583184946));
#95355=CARTESIAN_POINT('Ctrl Pts',(-11.6840057838,-22.9724912879,7.77196745159));
#95356=CARTESIAN_POINT('Ctrl Pts',(-11.6739934323,-22.9791841994,7.85280062059));
#95357=CARTESIAN_POINT('Ctrl Pts',(-11.6374046012,-22.9945001244,7.92955173236));
#95358=CARTESIAN_POINT('Ctrl Pts',(-11.575491188,-23.017355905,7.98966707089));
#95359=CARTESIAN_POINT('Ctrl Pts',(-11.4989860406,-23.044051495,8.02274251311));
#95360=CARTESIAN_POINT('Ctrl Pts',(-11.4203500465,-23.0707470797,8.02802946276));
#95361=CARTESIAN_POINT('Ctrl Pts',(-11.674734675,-22.9402340389,7.77528500471));
#95362=CARTESIAN_POINT('Ctrl Pts',(-11.6632751245,-22.9448939304,7.85395206414));
#95363=CARTESIAN_POINT('Ctrl Pts',(-11.6261291027,-22.9551888401,7.92866239052));
#95364=CARTESIAN_POINT('Ctrl Pts',(-11.5648099781,-22.9704904338,7.98774399745));
#95365=CARTESIAN_POINT('Ctrl Pts',(-11.4893943947,-22.9883613924,8.02148806052));
#95366=CARTESIAN_POINT('Ctrl Pts',(-11.4114432261,-23.0062323557,8.02896986926));
#95367=CARTESIAN_POINT('Ctrl Pts',(-11.6698654776,-22.907226316,7.77708988832));
#95368=CARTESIAN_POINT('Ctrl Pts',(-11.6579204713,-22.9095613324,7.85454768026));
#95369=CARTESIAN_POINT('Ctrl Pts',(-11.6206811584,-22.914710848,7.92810475864));
#95370=CARTESIAN_POINT('Ctrl Pts',(-11.5596933648,-22.9223583919,7.98661599137));
#95371=CARTESIAN_POINT('Ctrl Pts',(-11.4846565636,-22.931287768,8.02077577683));
#95372=CARTESIAN_POINT('Ctrl Pts',(-11.4067703651,-22.9402171391,8.02950137053));
#95373=CARTESIAN_POINT('Ctrl Pts',(-11.6698655273,-22.8742356121,7.77708987718));
#95374=CARTESIAN_POINT('Ctrl Pts',(-11.6579205194,-22.8742356226,7.85454767439));
#95375=CARTESIAN_POINT('Ctrl Pts',(-11.6206812044,-22.8742356357,7.92810475784));
#95376=CARTESIAN_POINT('Ctrl Pts',(-11.5596934089,-22.87423565,7.98661599254));
#95377=CARTESIAN_POINT('Ctrl Pts',(-11.4846566078,-22.8742356631,8.02077577467));
#95378=CARTESIAN_POINT('Ctrl Pts',(-11.4067704135,-22.8742356736,8.02950136067));
#95379=CARTESIAN_POINT('',(-11.9005548348204,-23.1693861585525,7.895572186247));
#95380=CARTESIAN_POINT('Ctrl Pts',(-11.6438378503,-23.4645366935,8.10736463748));
#95381=CARTESIAN_POINT('Ctrl Pts',(-11.6457407548972,-23.4474269895683,
8.10912409945425));
#95382=CARTESIAN_POINT('Ctrl Pts',(-11.6486630325428,-23.4303180321677,
8.10978091601121));
#95383=CARTESIAN_POINT('Ctrl Pts',(-11.65256298317,-23.4134680180269,8.10932257821117));
#95384=CARTESIAN_POINT('Ctrl Pts',(-11.6565377789634,-23.3962946300209,
8.10885544430778));
#95385=CARTESIAN_POINT('Ctrl Pts',(-11.6615279369715,-23.37939060852,8.10723006852047));
#95386=CARTESIAN_POINT('Ctrl Pts',(-11.6674552116862,-23.3630165572466,
8.10447292972245));
#95387=CARTESIAN_POINT('Ctrl Pts',(-11.6735237627704,-23.3462522310777,
8.10165007462501));
#95388=CARTESIAN_POINT('Ctrl Pts',(-11.6805744213503,-23.3300439067293,
8.09764098964143));
#95389=CARTESIAN_POINT('Ctrl Pts',(-11.6884909237533,-23.3146514397464,
8.09251343822578));
#95390=CARTESIAN_POINT('Ctrl Pts',(-11.6964815336893,-23.2991148816364,
8.0873378870539));
#95391=CARTESIAN_POINT('Ctrl Pts',(-11.7053539547591,-23.2844099860543,
8.08102307394607));
#95392=CARTESIAN_POINT('Ctrl Pts',(-11.7149602963441,-23.2707770127254,
8.073675339938));
#95393=CARTESIAN_POINT('Ctrl Pts',(-11.7245993021421,-23.2570976835241,
8.06630262160609));
#95394=CARTESIAN_POINT('Ctrl Pts',(-11.7349768686908,-23.2444980259262,
8.05789023480772));
#95395=CARTESIAN_POINT('Ctrl Pts',(-11.745920364852,-23.2331869359498,8.04857827595082));
#95396=CARTESIAN_POINT('Ctrl Pts',(-11.756829296706,-23.2219115713012,8.03929572829864));
#95397=CARTESIAN_POINT('Ctrl Pts',(-11.7683002094792,-23.2119170519958,
8.02911960219298));
#95398=CARTESIAN_POINT('Ctrl Pts',(-11.7801446348235,-23.2033704216458,
8.01821646048037));
#95399=CARTESIAN_POINT('Ctrl Pts',(-11.7918096503827,-23.1949532487468,
8.00747847074888));
#95400=CARTESIAN_POINT('Ctrl Pts',(-11.8038365705567,-23.1879407235758,
7.99603566767177));
#95401=CARTESIAN_POINT('Ctrl Pts',(-11.8160340495087,-23.1824486649995,
7.98406915540297));
#95402=CARTESIAN_POINT('Ctrl Pts',(-11.8280723255703,-23.1770282893999,
7.97225883142102));
#95403=CARTESIAN_POINT('Ctrl Pts',(-11.840276398251,-23.1730892198954,7.95993868610934));
#95404=CARTESIAN_POINT('Ctrl Pts',(-11.8524564888357,-23.1706957080467,
7.94729963439745));
#95405=CARTESIAN_POINT('Ctrl Pts',(-11.8643709607006,-23.1683543929817,
7.93493621025267));
#95406=CARTESIAN_POINT('Ctrl Pts',(-11.8762621855935,-23.1674921212114,
7.92226792528629));
#95407=CARTESIAN_POINT('Ctrl Pts',(-11.8879515998144,-23.1681206308898,
7.90948528184542));
#95408=CARTESIAN_POINT('Ctrl Pts',(-11.892181889249,-23.1683480826509,7.90485936300359));
#95409=CARTESIAN_POINT('Ctrl Pts',(-11.8963857612096,-23.1687702957837,
7.90021856034556));
#95410=CARTESIAN_POINT('Ctrl Pts',(-11.9005548359276,-23.1693861518639,
7.89557218635399));
#95411=CARTESIAN_POINT('',(-11.6698655452447,-22.8742356128,7.77708987356263));
#95412=CARTESIAN_POINT('Ctrl Pts',(-11.6698655273,-22.8742356128,7.77708987718));
#95413=CARTESIAN_POINT('Ctrl Pts',(-11.6698655124336,-22.8841203453796,
7.77708988050861));
#95414=CARTESIAN_POINT('Ctrl Pts',(-11.6703872773143,-22.8945390468658,
7.77689324751285));
#95415=CARTESIAN_POINT('Ctrl Pts',(-11.6715891474942,-22.9054209100778,
7.7764658141757));
#95416=CARTESIAN_POINT('Ctrl Pts',(-11.6718882682496,-22.908129181902,7.7763594348139));
#95417=CARTESIAN_POINT('Ctrl Pts',(-11.6722296873662,-22.910866176731,7.77623891315925));
#95418=CARTESIAN_POINT('Ctrl Pts',(-11.6726162016286,-22.9136308753537,
7.77610410993981));
#95419=CARTESIAN_POINT('Ctrl Pts',(-11.6728244048813,-22.9151201328075,
7.77603149562384));
#95420=CARTESIAN_POINT('Ctrl Pts',(-11.6730453375116,-22.9166151485335,
7.77595486411559));
#95421=CARTESIAN_POINT('Ctrl Pts',(-11.6732805949692,-22.9181230332283,
7.77587382906681));
#95422=CARTESIAN_POINT('Ctrl Pts',(-11.674145482278,-22.9236665358625,7.77557591636307));
#95423=CARTESIAN_POINT('Ctrl Pts',(-11.6752247585291,-22.9294892000468,
7.77521098652493));
#95424=CARTESIAN_POINT('Ctrl Pts',(-11.6765188200825,-22.9353811920076,
7.77479159710103));
#95425=CARTESIAN_POINT('Ctrl Pts',(-11.6777949650932,-22.9411916081532,
7.77437801420816));
#95426=CARTESIAN_POINT('Ctrl Pts',(-11.6792803566587,-22.9470693851126,
7.77391183617433));
#95427=CARTESIAN_POINT('Ctrl Pts',(-11.6809271617018,-22.9528173364117,
7.77342261518714));
#95428=CARTESIAN_POINT('Ctrl Pts',(-11.6822016511858,-22.9572657703755,
7.77304399902602));
#95429=CARTESIAN_POINT('Ctrl Pts',(-11.6835717755419,-22.9616365225724,
7.77265209353309));
#95430=CARTESIAN_POINT('Ctrl Pts',(-11.6849943332863,-22.9658401362469,
7.7722646214258));
#95431=CARTESIAN_POINT('Ctrl Pts',(-11.6869904334254,-22.9717385497725,
7.77172092952276));
#95432=CARTESIAN_POINT('Ctrl Pts',(-11.6891111912027,-22.9774017432891,
7.77119600464548));
#95433=CARTESIAN_POINT('Ctrl Pts',(-11.6914115443287,-22.9830234104527,
7.77067661915821));
#95434=CARTESIAN_POINT('Ctrl Pts',(-11.6936439591363,-22.9884790480577,
7.77017257313175));
#95435=CARTESIAN_POINT('Ctrl Pts',(-11.6960457876511,-22.993895771449,7.76967272729939));
#95436=CARTESIAN_POINT('Ctrl Pts',(-11.6987131473567,-22.9994417956824,
7.76916948557355));
#95437=CARTESIAN_POINT('Ctrl Pts',(-11.700426214222,-23.0030036363776,7.76884628704733));
#95438=CARTESIAN_POINT('Ctrl Pts',(-11.7022496933578,-23.0066186583115,
7.76852175128625));
#95439=CARTESIAN_POINT('Ctrl Pts',(-11.7042191449779,-23.0103284488021,
7.76819851840486));
#95440=CARTESIAN_POINT('Ctrl Pts',(-11.7083171006155,-23.0180476314926,
7.76752594843917));
#95441=CARTESIAN_POINT('Ctrl Pts',(-11.7126643864249,-23.025476754061,7.76701456578987));
#95442=CARTESIAN_POINT('Ctrl Pts',(-11.7172052293534,-23.032615071251,7.76669876886871));
#95443=CARTESIAN_POINT('Ctrl Pts',(-11.7177627166421,-23.0334914550323,
7.76665999792417));
#95444=CARTESIAN_POINT('Ctrl Pts',(-11.7183231854258,-23.0343635452706,
7.76662416222729));
#95445=CARTESIAN_POINT('Ctrl Pts',(-11.7188864419448,-23.0352312083239,
7.76659140543157));
#95446=CARTESIAN_POINT('Ctrl Pts',(-11.7198925864243,-23.0367811138495,
7.76653289200462));
#95447=CARTESIAN_POINT('Ctrl Pts',(-11.7209076421493,-23.0383169059184,
7.7664841882737));
#95448=CARTESIAN_POINT('Ctrl Pts',(-11.7219315119051,-23.0398385808136,
7.76644546906638));
#95449=CARTESIAN_POINT('Ctrl Pts',(-11.7223273569165,-23.0404268855398,
7.76643049957931));
#95450=CARTESIAN_POINT('Ctrl Pts',(-11.72272451719,-23.041013078508,7.76641702418818));
#95451=CARTESIAN_POINT('Ctrl Pts',(-11.7231229790036,-23.0415971536289,
7.76640505882331));
#95452=CARTESIAN_POINT('Ctrl Pts',(-11.7234037527934,-23.0420087187517,
7.76639662749884));
#95453=CARTESIAN_POINT('Ctrl Pts',(-11.7236851727353,-23.0424192322473,
7.76638894600219));
#95454=CARTESIAN_POINT('Ctrl Pts',(-11.7239672327341,-23.042828691091,7.76638202072213));
#95455=CARTESIAN_POINT('Ctrl Pts',(-11.7241736706056,-23.0431283713454,
7.76637695215487));
#95456=CARTESIAN_POINT('Ctrl Pts',(-11.7243799312776,-23.0434267115443,
7.76637230938042));
#95457=CARTESIAN_POINT('Ctrl Pts',(-11.7245799519957,-23.043715051258,7.76636818977289));
#95458=CARTESIAN_POINT('Ctrl Pts',(-11.7257206878381,-23.045359478142,7.7663446952869));
#95459=CARTESIAN_POINT('Ctrl Pts',(-11.7267188556241,-23.0467712679517,
7.76633475147523));
#95460=CARTESIAN_POINT('Ctrl Pts',(-11.7278501756133,-23.0483433079471,
7.76633514799306));
#95461=CARTESIAN_POINT('Ctrl Pts',(-11.7288494912053,-23.0497319195634,
7.76633549824449));
#95462=CARTESIAN_POINT('Ctrl Pts',(-11.7299524098615,-23.0512456217772,
7.76634351678061));
#95463=CARTESIAN_POINT('Ctrl Pts',(-11.7313750775217,-23.0531480387012,
7.76637596130601));
#95464=CARTESIAN_POINT('Ctrl Pts',(-11.7373284520788,-23.0611089988252,
7.76651173047928));
#95465=CARTESIAN_POINT('Ctrl Pts',(-11.7434317507374,-23.0685194797057,
7.76705223096266));
#95466=CARTESIAN_POINT('Ctrl Pts',(-11.7495966028089,-23.0754143832906,
7.76800907885379));
#95467=CARTESIAN_POINT('Ctrl Pts',(-11.7555268124262,-23.0820468576914,
7.76892950784386));
#95468=CARTESIAN_POINT('Ctrl Pts',(-11.7615104447489,-23.088199390884,7.77023684976931));
#95469=CARTESIAN_POINT('Ctrl Pts',(-11.7674655798331,-23.0938978810723,
7.77190303623388));
#95470=CARTESIAN_POINT('Ctrl Pts',(-11.7687515475446,-23.0951284282023,
7.77226283697134));
#95471=CARTESIAN_POINT('Ctrl Pts',(-11.770036266467,-23.0963378510776,7.77263919924583));
#95472=CARTESIAN_POINT('Ctrl Pts',(-11.7713190725072,-23.0975265031653,
7.7730315672446));
#95473=CARTESIAN_POINT('Ctrl Pts',(-11.7780184940438,-23.1037342081074,
7.77508069902199));
#95474=CARTESIAN_POINT('Ctrl Pts',(-11.7846643103656,-23.1093783289844,
7.77758924145152));
#95475=CARTESIAN_POINT('Ctrl Pts',(-11.791166992,-23.1145134944792,7.78054542587794));
#95476=CARTESIAN_POINT('Ctrl Pts',(-11.7944183328172,-23.1170810772266,
7.78202351809116));
#95477=CARTESIAN_POINT('Ctrl Pts',(-11.7976341986518,-23.1195214885636,
7.7836135664346));
#95478=CARTESIAN_POINT('Ctrl Pts',(-11.8008050898331,-23.1218418377442,
7.78531434295865));
#95479=CARTESIAN_POINT('Ctrl Pts',(-11.8022440127623,-23.122894792087,7.78608614060103));
#95480=CARTESIAN_POINT('Ctrl Pts',(-11.8034616587886,-23.1237701018227,
7.78676260102076));
#95481=CARTESIAN_POINT('Ctrl Pts',(-11.8047441929008,-23.1246798089907,
7.78749652651521));
#95482=CARTESIAN_POINT('Ctrl Pts',(-11.8059201430297,-23.1255139156638,
7.78816945971175));
#95483=CARTESIAN_POINT('Ctrl Pts',(-11.8071508091656,-23.1263770130773,
7.78889062389471));
#95484=CARTESIAN_POINT('Ctrl Pts',(-11.8086641746866,-23.1274176790227,
7.78981460459052));
#95485=CARTESIAN_POINT('Ctrl Pts',(-11.8091374815276,-23.1277431485171,
7.79010358063638));
#95486=CARTESIAN_POINT('Ctrl Pts',(-11.8096384931628,-23.1280858563205,
7.79041271122205));
#95487=CARTESIAN_POINT('Ctrl Pts',(-11.8101743388709,-23.1284499143557,
7.7907477664464));
#95488=CARTESIAN_POINT('Ctrl Pts',(-11.8201336553098,-23.1352163568592,
7.79697515793818));
#95489=CARTESIAN_POINT('Ctrl Pts',(-11.8299458768997,-23.141070908697,7.8045010798013));
#95490=CARTESIAN_POINT('Ctrl Pts',(-11.8395088976496,-23.1461218781324,
7.81333714787196));
#95491=CARTESIAN_POINT('Ctrl Pts',(-11.8490941108826,-23.1511845691311,
7.82219372141846));
#95492=CARTESIAN_POINT('Ctrl Pts',(-11.8584352736138,-23.1554412136267,
7.8323669370134));
#95493=CARTESIAN_POINT('Ctrl Pts',(-11.8674423905467,-23.1589852725995,
7.84387767342908));
#95494=CARTESIAN_POINT('Ctrl Pts',(-11.8733075965803,-23.1612930738889,
7.85137317295236));
#95495=CARTESIAN_POINT('Ctrl Pts',(-11.8790314091254,-23.1632979472643,
7.8594372001096));
#95496=CARTESIAN_POINT('Ctrl Pts',(-11.8845698557022,-23.1650229769109,
7.86806183689275));
#95497=CARTESIAN_POINT('Ctrl Pts',(-11.8894630610363,-23.1665470367987,
7.87568168446672));
#95498=CARTESIAN_POINT('Ctrl Pts',(-11.8942119030766,-23.1678521919875,
7.88374041620657));
#95499=CARTESIAN_POINT('Ctrl Pts',(-11.8987644056655,-23.1689586903633,
7.89220348632107));
#95500=CARTESIAN_POINT('Ctrl Pts',(-11.8993647202297,-23.1691045984824,
7.89331946685021));
#95501=CARTESIAN_POINT('Ctrl Pts',(-11.8999615824553,-23.1692470654513,
7.89444241478444));
#95502=CARTESIAN_POINT('Ctrl Pts',(-11.9005548359869,-23.1693861518727,
7.89557218628791));
#95503=CARTESIAN_POINT('Origin',(-11.3748953755427,-22.8742356445387,7.7329560039236));
#95504=CARTESIAN_POINT('Ctrl Pts',(-11.9421544921,-23.1742356128,7.97460750747));
#95505=CARTESIAN_POINT('Ctrl Pts',(-11.8781704985,-23.1742356128,8.04380788698));
#95506=CARTESIAN_POINT('Ctrl Pts',(-11.8141865049,-23.2112466293,8.11300826649));
#95507=CARTESIAN_POINT('Ctrl Pts',(-11.7636135705,-23.2857400536,8.16770423124));
#95508=CARTESIAN_POINT('Ctrl Pts',(-11.7384871149,-23.3799878332,8.19487915673));
#95509=CARTESIAN_POINT('Ctrl Pts',(-11.7384871149,-23.4742356128,8.19487915673));
#95510=CARTESIAN_POINT('Ctrl Pts',(-11.9338050766,-23.1742356128,7.95878179633));
#95511=CARTESIAN_POINT('Ctrl Pts',(-11.8690129979,-23.1723658919,8.02885614127));
#95512=CARTESIAN_POINT('Ctrl Pts',(-11.8029049395,-23.2084420454,8.09871370492));
#95513=CARTESIAN_POINT('Ctrl Pts',(-11.7493954495,-23.283359451,8.15328464759));
#95514=CARTESIAN_POINT('Ctrl Pts',(-11.7215525483,-23.3787975319,8.17922113275));
#95515=CARTESIAN_POINT('Ctrl Pts',(-11.7194707712,-23.4742356128,8.17729628178));
#95516=CARTESIAN_POINT('Ctrl Pts',(-11.925456866,-23.1737486504,7.94293960289));
#95517=CARTESIAN_POINT('Ctrl Pts',(-11.8599896787,-23.169946111,8.01395123592));
#95518=CARTESIAN_POINT('Ctrl Pts',(-11.7918088017,-23.204981018,8.08451905773));
#95519=CARTESIAN_POINT('Ctrl Pts',(-11.7353200262,-23.2802129884,8.13897414048));
#95520=CARTESIAN_POINT('Ctrl Pts',(-11.704689803,-23.37673734,8.16362951651));
#95521=CARTESIAN_POINT('Ctrl Pts',(-11.7004667677,-23.4732616915,8.15972481694));
#95522=CARTESIAN_POINT('Ctrl Pts',(-11.9171250584,-23.1727778426,7.92710974195));
#95523=CARTESIAN_POINT('Ctrl Pts',(-11.8511250917,-23.166992891,7.99912450114));
#95524=CARTESIAN_POINT('Ctrl Pts',(-11.7809316294,-23.2008856654,8.07045852272));
#95525=CARTESIAN_POINT('Ctrl Pts',(-11.721423774,-23.276320039,8.12480753543));
#95526=CARTESIAN_POINT('Ctrl Pts',(-11.6879347422,-23.3738200593,8.14813746342));
#95527=CARTESIAN_POINT('Ctrl Pts',(-11.6815098074,-23.471320079,8.14219684908));
#95528=CARTESIAN_POINT('Ctrl Pts',(-11.9088198181,-23.171323915,7.91131175397));
#95529=CARTESIAN_POINT('Ctrl Pts',(-11.8424378979,-23.1635210449,7.98439851249));
#95530=CARTESIAN_POINT('Ctrl Pts',(-11.7703001202,-23.1961765665,8.0565580465));
#95531=CARTESIAN_POINT('Ctrl Pts',(-11.7077347865,-23.2716977713,8.11081129139));
#95532=CARTESIAN_POINT('Ctrl Pts',(-11.6713131361,-23.3700549965,8.13276881012));
#95533=CARTESIAN_POINT('Ctrl Pts',(-11.6626231066,-23.4684122213,8.12473384452));
#95534=CARTESIAN_POINT('Ctrl Pts',(-11.9005548343,-23.1693861722,7.89557218484));
#95535=CARTESIAN_POINT('Ctrl Pts',(-11.8339499495,-23.1595472906,7.96980237485));
#95536=CARTESIAN_POINT('Ctrl Pts',(-11.7599452801,-23.1908783692,8.04284981853));
#95537=CARTESIAN_POINT('Ctrl Pts',(-11.6942870876,-23.2663663719,8.09701806797));
#95538=CARTESIAN_POINT('Ctrl Pts',(-11.6548578924,-23.3654515527,8.11755397832));
#95539=CARTESIAN_POINT('Ctrl Pts',(-11.6438378503,-23.4645367334,8.10736463748));
#95540=CARTESIAN_POINT('Origin',(-11.9551818975745,-22.3491879643317,7.96775954099132));
#95541=CARTESIAN_POINT('Origin',(2.84607155346,-22.8742356128,5.53854202767));
#95542=CARTESIAN_POINT('',(-11.7512376696,-22.8742356128,3.91309124051));
#95543=CARTESIAN_POINT('Origin',(-12.0493948734,-22.8742356128,3.87989061057));
#95544=CARTESIAN_POINT('Origin',(2.84607155346,-22.8742356128,5.53854202767));
#95545=CARTESIAN_POINT('Origin',(-11.4530804658,-22.8742356128,3.94629187045));
#95546=CARTESIAN_POINT('',(-11.4530804658,-22.8742356128,3.64629187045));
#95547=CARTESIAN_POINT('Origin',(-11.4530804658,-22.8742356128,3.34629187045));
#95548=CARTESIAN_POINT('Origin',(-11.4530804658,-22.8742356128,3.94629187045));
#95549=CARTESIAN_POINT('Origin',(-6.6707290414,-22.8742356128,3.34629187045));
#95550=CARTESIAN_POINT('',(-8.10176909975,-22.8742356128,3.64629187045));
#95551=CARTESIAN_POINT('Origin',(-8.10176909975,-22.8742356128,3.34629187045));
#95552=CARTESIAN_POINT('',(-9.77742478279,-22.8742356128,3.64629187045));
#95553=CARTESIAN_POINT('Origin',(-8.10176909975,-22.8742356128,3.94629187045));
#95554=CARTESIAN_POINT('',(-7.80346303227,-22.8742356128,3.91445651114));
#95555=CARTESIAN_POINT('Origin',(-7.50515696478,-22.8742356128,3.88262115182));
#95556=CARTESIAN_POINT('Origin',(-8.10176909975,-22.8742356128,3.94629187045));
#95557=CARTESIAN_POINT('Origin',(-0.00234331738835,-22.8742356128,3.08191746407));
#95558=CARTESIAN_POINT('',(-6.23264645859,-22.8742356128,7.84992678029));
#95559=CARTESIAN_POINT('Origin',(-5.99440665492,-22.8742356128,7.66760345225));
#95560=CARTESIAN_POINT('Origin',(-0.00234331738835,-22.8742356128,3.08191746407));
#95561=CARTESIAN_POINT('Origin',(-6.47088626226,-22.8742356128,8.03225010833));
#95562=CARTESIAN_POINT('',(-6.26721888507,-22.8742356128,8.25252175759));
#95563=CARTESIAN_POINT('Origin',(-6.06355150788,-22.8742356128,8.47279340685));
#95564=CARTESIAN_POINT('Origin',(-6.47088626226,-22.8742356128,8.03225010833));
#95565=CARTESIAN_POINT('Ctrl Pts',(-8.73611662316,-23.4697910609,10.8942571942));
#95566=CARTESIAN_POINT('Ctrl Pts',(-8.72752432309,-23.3771104598,10.9015348722));
#95567=CARTESIAN_POINT('Ctrl Pts',(-8.69545860941,-23.2844298587,10.881098933));
#95568=CARTESIAN_POINT('Ctrl Pts',(-8.6413960311,-23.2107990757,10.8311116668));
#95569=CARTESIAN_POINT('Ctrl Pts',(-8.57793853593,-23.1733813929,10.7632250691));
#95570=CARTESIAN_POINT('Ctrl Pts',(-8.51747666777,-23.1720133445,10.6920986219));
#95571=CARTESIAN_POINT('Ctrl Pts',(-8.72470175689,-23.4715681133,10.9039255852));
#95572=CARTESIAN_POINT('Ctrl Pts',(-8.7177987489,-23.3784476295,10.9097561006));
#95573=CARTESIAN_POINT('Ctrl Pts',(-8.68736831632,-23.2853271458,10.8877470417));
#95574=CARTESIAN_POINT('Ctrl Pts',(-8.63454393537,-23.211417996,10.8363489167));
#95575=CARTESIAN_POINT('Ctrl Pts',(-8.57168882428,-23.1740163051,10.7675887259));
#95576=CARTESIAN_POINT('Ctrl Pts',(-8.51124350946,-23.1729018671,10.696222277));
#95577=CARTESIAN_POINT('Ctrl Pts',(-8.71323427675,-23.4729019084,10.9136114204));
#95578=CARTESIAN_POINT('Ctrl Pts',(-8.70803661002,-23.3794040149,10.9179891886));
#95579=CARTESIAN_POINT('Ctrl Pts',(-8.67925545718,-23.2859061213,10.8943982297));
#95580=CARTESIAN_POINT('Ctrl Pts',(-8.62767478659,-23.2117711836,10.8415808992));
#95581=CARTESIAN_POINT('Ctrl Pts',(-8.5654164258,-23.1744185718,10.771945772));
#95582=CARTESIAN_POINT('Ctrl Pts',(-8.50497501432,-23.1735687617,10.7003455662));
#95583=CARTESIAN_POINT('Ctrl Pts',(-8.70172748022,-23.4737911951,10.9233030613));
#95584=CARTESIAN_POINT('Ctrl Pts',(-8.69824977302,-23.3799791247,10.9262239001));
#95585=CARTESIAN_POINT('Ctrl Pts',(-8.67113050266,-23.2861670544,10.9010437414));
#95586=CARTESIAN_POINT('Ctrl Pts',(-8.62079773014,-23.2118592846,10.8468003207));
#95587=CARTESIAN_POINT('Ctrl Pts',(-8.55912932234,-23.1745884938,10.7762902146));
#95588=CARTESIAN_POINT('Ctrl Pts',(-8.49867834935,-23.1740134037,10.7044634205));
#95589=CARTESIAN_POINT('Ctrl Pts',(-8.69019480669,-23.4742356128,10.9329890024));
#95590=CARTESIAN_POINT('Ctrl Pts',(-8.68845018412,-23.3801733377,10.9344501196));
#95591=CARTESIAN_POINT('Ctrl Pts',(-8.66300395829,-23.2861110626,10.9076749542));
#95592=CARTESIAN_POINT('Ctrl Pts',(-8.61392194556,-23.2116837148,10.8520000359));
#95593=CARTESIAN_POINT('Ctrl Pts',(-8.55283556198,-23.1745270026,10.7806162216));
#95594=CARTESIAN_POINT('Ctrl Pts',(-8.49236081888,-23.1742356128,10.7085709021));
#95595=CARTESIAN_POINT('Ctrl Pts',(-8.67864985337,-23.4742356128,10.942657873));
#95596=CARTESIAN_POINT('Ctrl Pts',(-8.67864985337,-23.3799878332,10.942657873));
#95597=CARTESIAN_POINT('Ctrl Pts',(-8.65488631632,-23.2857400536,10.9142834188));
#95598=CARTESIAN_POINT('Ctrl Pts',(-8.60705657762,-23.2112466293,10.8571731189));
#95599=CARTESIAN_POINT('Ctrl Pts',(-8.54654322741,-23.1742356128,10.7849181647));
#95600=CARTESIAN_POINT('Ctrl Pts',(-8.48602987721,-23.1742356128,10.7126632105));
#95601=CARTESIAN_POINT('',(-8.51747674095254,-23.1720132750395,10.6920985878956));
#95602=CARTESIAN_POINT('Origin',(-8.46564327939413,-22.8727019153709,10.6937226627841));
#95603=CARTESIAN_POINT('Origin',(-8.54339070302529,-23.4677320541598,10.6671045573098));
#95604=CARTESIAN_POINT('Ctrl Pts',(-8.73611663424,-23.4697908757,10.8942572059));
#95605=CARTESIAN_POINT('Ctrl Pts',(-8.72752435034,-23.3771103023,10.9015348641));
#95606=CARTESIAN_POINT('Ctrl Pts',(-8.69545865342,-23.2844297289,10.881098906));
#95607=CARTESIAN_POINT('Ctrl Pts',(-8.64139608915,-23.2107989673,10.8311116257));
#95608=CARTESIAN_POINT('Ctrl Pts',(-8.57793860163,-23.1733812942,10.7632250217));
#95609=CARTESIAN_POINT('Ctrl Pts',(-8.51747673428,-23.1720132443,10.6920985753));
#95610=CARTESIAN_POINT('Ctrl Pts',(-8.85271909481,-23.4283765706,10.7986501186));
#95611=CARTESIAN_POINT('Ctrl Pts',(-8.80174479507,-23.3522217493,10.8290472717));
#95612=CARTESIAN_POINT('Ctrl Pts',(-8.74702097884,-23.2760669279,10.8249995844));
#95613=CARTESIAN_POINT('Ctrl Pts',(-8.69926483364,-23.2110252232,10.7808433397));
#95614=CARTESIAN_POINT('Ctrl Pts',(-8.66655321101,-23.1680969408,10.704046549));
#95615=CARTESIAN_POINT('Ctrl Pts',(-8.64928312709,-23.1513060056,10.6105493344));
#95616=CARTESIAN_POINT('Ctrl Pts',(-8.95374236957,-23.2551805764,10.8169485727));
#95617=CARTESIAN_POINT('Ctrl Pts',(-8.90906105284,-23.2232432649,10.7961844516));
#95618=CARTESIAN_POINT('Ctrl Pts',(-8.87369407635,-23.1913059533,10.770178964));
#95619=CARTESIAN_POINT('Ctrl Pts',(-8.84720879161,-23.1552341963,10.7456901634));
#95620=CARTESIAN_POINT('Ctrl Pts',(-8.82709666423,-23.1116114836,10.7203986113));
#95621=CARTESIAN_POINT('Ctrl Pts',(-8.81389010608,-23.0647081339,10.6876384968));
#95622=CARTESIAN_POINT('Ctrl Pts',(-9.01791018836,-23.1549008445,10.8214049608));
#95623=CARTESIAN_POINT('Ctrl Pts',(-8.99622746462,-23.1216722312,10.8155316644));
#95624=CARTESIAN_POINT('Ctrl Pts',(-8.97425273896,-23.0884436179,10.8039507789));
#95625=CARTESIAN_POINT('Ctrl Pts',(-8.95224692858,-23.0584727018,10.783603786));
#95626=CARTESIAN_POINT('Ctrl Pts',(-8.93220449355,-23.0344758471,10.7563348016));
#95627=CARTESIAN_POINT('Ctrl Pts',(-8.91487253124,-23.0145682268,10.7261343735));
#95628=CARTESIAN_POINT('Ctrl Pts',(-9.08532173979,-23.0061361581,10.858062108));
#95629=CARTESIAN_POINT('Ctrl Pts',(-9.07401122054583,-22.994360504385,10.847601774363));
#95630=CARTESIAN_POINT('Ctrl Pts',(-9.06350105813443,-22.9825848532249,
10.8378821902984));
#95631=CARTESIAN_POINT('Ctrl Pts',(-9.05419277619886,-22.9699073952249,
10.8292755748936));
#95632=CARTESIAN_POINT('Ctrl Pts',(-9.04554579428692,-22.955591884285,10.8212820971294));
#95633=CARTESIAN_POINT('Ctrl Pts',(-9.03689844897,-22.9401858313,10.8132890077));
#95634=CARTESIAN_POINT('Ctrl Pts',(-9.1336794452,-22.8742356128,10.9029059811));
#95635=CARTESIAN_POINT('Ctrl Pts',(-9.1336794452,-22.8742356128,10.9029059811));
#95636=CARTESIAN_POINT('Ctrl Pts',(-9.1336794452,-22.8742356128,10.9029059811));
#95637=CARTESIAN_POINT('Ctrl Pts',(-9.1336794452,-22.8742356128,10.9029059811));
#95638=CARTESIAN_POINT('Ctrl Pts',(-9.1336794452,-22.8742356128,10.9029059811));
#95639=CARTESIAN_POINT('Ctrl Pts',(-9.1336794452,-22.8742356128,10.9029059811));
#95640=CARTESIAN_POINT('Ctrl Pts',(-9.1336794452,-22.8742356128,10.9029059811));
#95641=CARTESIAN_POINT('Ctrl Pts',(-9.12359832874988,-22.8811058500385,
10.8935710990721));
#95642=CARTESIAN_POINT('Ctrl Pts',(-9.113191622868,-22.8880836120972,10.8842714443679));
#95643=CARTESIAN_POINT('Ctrl Pts',(-9.10255323648157,-22.8951026557958,
10.8751006061354));
#95644=CARTESIAN_POINT('Ctrl Pts',(-9.09148992869508,-22.9024020560981,
10.865563463721));
#95645=CARTESIAN_POINT('Ctrl Pts',(-9.08017585698654,-22.9097463028922,
10.8561652636545));
#95646=CARTESIAN_POINT('Ctrl Pts',(-9.068677710726,-22.9170878993633,10.8469738134868));
#95647=CARTESIAN_POINT('Ctrl Pts',(-9.05606690031054,-22.9251399348085,
10.8368929158462));
#95648=CARTESIAN_POINT('Ctrl Pts',(-9.04323465488263,-22.9331888946587,
10.8270603983741));
#95649=CARTESIAN_POINT('Ctrl Pts',(-9.03022424765914,-22.9412018306295,
10.8175265503564));
#95650=CARTESIAN_POINT('Ctrl Pts',(-9.02087653152683,-22.9469589640962,
10.8106766721483));
#95651=CARTESIAN_POINT('Ctrl Pts',(-9.01143583423362,-22.9526981799119,
10.8039800671005));
#95652=CARTESIAN_POINT('Ctrl Pts',(-9.0019065535912,-22.9584144908771,10.7974466868649));
#95653=CARTESIAN_POINT('Ctrl Pts',(-8.9847535490042,-22.9687040302333,10.7856863971478));
#95654=CARTESIAN_POINT('Ctrl Pts',(-8.96731630136919,-22.9789182402692,
10.7744552003213));
#95655=CARTESIAN_POINT('Ctrl Pts',(-8.94956526595337,-22.9890573569769,
10.7637843427106));
#95656=CARTESIAN_POINT('Ctrl Pts',(-8.93276576605315,-22.9986529713243,
10.7536854911695));
#95657=CARTESIAN_POINT('Ctrl Pts',(-8.91568265292127,-23.0081832742568,
10.744085552575));
#95658=CARTESIAN_POINT('Ctrl Pts',(-8.89826151733235,-23.0176556306316,
10.7350216727571));
#95659=CARTESIAN_POINT('Ctrl Pts',(-8.88417397090941,-23.0253154217791,
10.7276921948907));
#95660=CARTESIAN_POINT('Ctrl Pts',(-8.86986440346832,-23.0329378192506,
10.7207128487755));
#95661=CARTESIAN_POINT('Ctrl Pts',(-8.85530486807876,-23.0405181524084,
10.7141276263695));
#95662=CARTESIAN_POINT('Ctrl Pts',(-8.84127764671044,-23.047821339523,10.707783167568));
#95663=CARTESIAN_POINT('Ctrl Pts',(-8.82701783103774,-23.055085911662,10.7018038913073));
#95664=CARTESIAN_POINT('Ctrl Pts',(-8.81251122931992,-23.0622926242237,
10.6962618555677));
#95665=CARTESIAN_POINT('Ctrl Pts',(-8.79876011359606,-23.0691240200497,
10.6910084422402));
#95666=CARTESIAN_POINT('Ctrl Pts',(-8.78478689488389,-23.0759036692302,
10.6861475775762));
#95667=CARTESIAN_POINT('Ctrl Pts',(-8.77059576001363,-23.0825967640568,
10.681777295819));
#95668=CARTESIAN_POINT('Ctrl Pts',(-8.75729431827173,-23.0888702447702,
10.6776810026951));
#95669=CARTESIAN_POINT('Ctrl Pts',(-8.7438012610872,-23.0950677771167,10.6740156131765));
#95670=CARTESIAN_POINT('Ctrl Pts',(-8.73013818703274,-23.1011418674376,
10.6708977038454));
#95671=CARTESIAN_POINT('Ctrl Pts',(-8.71719988970545,-23.1068937492069,
10.6679451883422));
#95672=CARTESIAN_POINT('Ctrl Pts',(-8.70410903249947,-23.1125349926791,
10.6654835591288));
#95673=CARTESIAN_POINT('Ctrl Pts',(-8.69090263710776,-23.1180067844081,
10.6636460594846));
#95674=CARTESIAN_POINT('Ctrl Pts',(-8.67775361963559,-23.1234548028049,
10.6618165432381));
#95675=CARTESIAN_POINT('Ctrl Pts',(-8.66448983074481,-23.1287350304218,
10.6606054381024));
#95676=CARTESIAN_POINT('Ctrl Pts',(-8.6511695285881,-23.1337685681875,10.6601821897177));
#95677=CARTESIAN_POINT('Ctrl Pts',(-8.63836928290993,-23.1386055845909,
10.6597754659631));
#95678=CARTESIAN_POINT('Ctrl Pts',(-8.62551678329554,-23.1432148356153,
10.6600962419175));
#95679=CARTESIAN_POINT('Ctrl Pts',(-8.61268579786253,-23.1475055628669,
10.6613321230521));
#95680=CARTESIAN_POINT('Ctrl Pts',(-8.6001045595605,-23.1517127737878,10.662543948531));
#95681=CARTESIAN_POINT('Ctrl Pts',(-8.58754389183535,-23.1556138260663,
10.6646354720753));
#95682=CARTESIAN_POINT('Ctrl Pts',(-8.57509640895897,-23.1591018128687,
10.6678214861139));
#95683=CARTESIAN_POINT('Ctrl Pts',(-8.56297826588685,-23.1624975133107,
10.6709232034919));
#95684=CARTESIAN_POINT('Ctrl Pts',(-8.55096733469553,-23.1655017591573,
10.675062205123));
#95685=CARTESIAN_POINT('Ctrl Pts',(-8.53917239193139,-23.1679945890078,
10.6804742569932));
#95686=CARTESIAN_POINT('Ctrl Pts',(-8.5318464032349,-23.1695429172763,10.6838357511198));
#95687=CARTESIAN_POINT('Ctrl Pts',(-8.52460420271352,-23.1708935277647,
10.6876891087437));
#95688=CARTESIAN_POINT('Ctrl Pts',(-8.51747674491568,-23.1720132445407,
10.6920985878117));
#95689=CARTESIAN_POINT('Origin',(-6.6707290414,-22.8742356128,9.03420135995));
#95690=CARTESIAN_POINT('',(-7.70044916513,-22.8742356128,9.57771386935));
#95691=CARTESIAN_POINT('Origin',(7.16045579301E-17,-22.6642356128,0.580061096523));
#95692=CARTESIAN_POINT('',(-10.9304145503,-21.0742356128,10.3907473403));
#95693=CARTESIAN_POINT('',(-10.9304145503,-21.9742356128,10.3907473403));
#95694=CARTESIAN_POINT('',(-10.0062431967,-21.0742356128,11.3317411468));
#95695=CARTESIAN_POINT('Origin',(2.04268023839E-15,-21.0742356128,0.580061096523));
#95696=CARTESIAN_POINT('',(-10.0062431967,-23.2742356128,11.3317411468));
#95697=CARTESIAN_POINT('Origin',(-10.1862176145,-21.9742356128,9.72278707155));
#95698=CARTESIAN_POINT('',(-11.1383462684,-21.0742356128,10.0284846777));
#95699=CARTESIAN_POINT('',(-11.1383462684,-22.6642356128,10.0284846777));
#95700=CARTESIAN_POINT('Origin',(-10.1862176145,-21.0742356128,9.72278707155));
#95701=CARTESIAN_POINT('Origin',(2.84607155346,-22.6642356128,5.53854202767));
#95702=CARTESIAN_POINT('Origin',(2.84607155346,-21.0742356128,5.53854202767));
#95703=CARTESIAN_POINT('Origin',(-11.3733704264,-23.1237854196,7.73136642019));
#95704=CARTESIAN_POINT('',(-11.669865565,-21.0742356128,7.77708985809));
#95705=CARTESIAN_POINT('',(-11.669865565,-22.5742356128,7.77708985809));
#95706=CARTESIAN_POINT('Origin',(-11.3733704264,-21.0742356128,7.73136642019));
#95707=CARTESIAN_POINT('Origin',(2.84607155346,-21.2742356128,5.53854202767));
#95708=CARTESIAN_POINT('',(-11.7512376696,-21.0742356128,3.91309124051));
#95709=CARTESIAN_POINT('',(-11.7512376696,-22.1242356128,3.91309124051));
#95710=CARTESIAN_POINT('Origin',(2.84607155346,-21.0742356128,5.53854202767));
#95711=CARTESIAN_POINT('Origin',(-11.4530804658,-22.1242356128,3.94629187045));
#95712=CARTESIAN_POINT('',(-11.4530804658,-21.0742356128,3.64629187045));
#95713=CARTESIAN_POINT('',(-11.4530804658,-21.9742356128,3.64629187045));
#95714=CARTESIAN_POINT('Origin',(-11.4530804658,-21.0742356128,3.94629187045));
#95715=CARTESIAN_POINT('Origin',(-11.7190551593,-23.1742356128,3.64629187045));
#95716=CARTESIAN_POINT('',(-8.10176909975,-21.0742356128,3.64629187045));
#95717=CARTESIAN_POINT('',(-8.10176909975,-22.1242356128,3.64629187045));
#95718=CARTESIAN_POINT('',(-8.95225019493,-21.0742356128,3.64629187045));
#95719=CARTESIAN_POINT('Origin',(-8.10176909975,-22.1242356128,3.94629187045));
#95720=CARTESIAN_POINT('',(-7.80346303227,-21.0742356128,3.91445651114));
#95721=CARTESIAN_POINT('',(-7.80346303227,-21.2742356128,3.91445651114));
#95722=CARTESIAN_POINT('Origin',(-8.10176909975,-21.0742356128,3.94629187045));
#95723=CARTESIAN_POINT('Origin',(-0.00234331738835,-21.2742356128,3.08191746407));
#95724=CARTESIAN_POINT('',(-6.23264645859,-21.0742356128,7.84992678029));
#95725=CARTESIAN_POINT('',(-6.23264645859,-22.1242356128,7.84992678029));
#95726=CARTESIAN_POINT('Origin',(-0.00234331738835,-21.0742356128,3.08191746407));
#95727=CARTESIAN_POINT('Origin',(-6.47088626226,-22.1242356128,8.03225010833));
#95728=CARTESIAN_POINT('',(-6.26721888507,-21.0742356128,8.25252175759));
#95729=CARTESIAN_POINT('',(-6.26721888507,-21.9742356128,8.25252175759));
#95730=CARTESIAN_POINT('Origin',(-6.47088626226,-21.0742356128,8.03225010833));
#95731=CARTESIAN_POINT('Origin',(-9.80058174751,-23.1742356128,11.519536597));
#95732=CARTESIAN_POINT('',(-9.59819339216,-21.0742356128,11.3324044552));
#95733=CARTESIAN_POINT('',(-9.59819339216,-23.2742356128,11.3324044552));
#95734=CARTESIAN_POINT('',(-8.22276378328,-21.0742356128,10.0606559488));
#95735=CARTESIAN_POINT('Origin',(-9.80186076935,-23.2742356128,11.1121328059));
#95736=CARTESIAN_POINT('Origin',(-9.80186076935,-21.0742356128,11.1121328059));
#95737=CARTESIAN_POINT('Origin',(-9.80186076935,-21.0742356128,11.1121328059));
#95738=CARTESIAN_POINT('',(-9.80186076935,-20.7742356128,11.1121328059));
#95739=CARTESIAN_POINT('Origin',(-9.80186076935,-21.0742356128,11.1121328059));
#95740=CARTESIAN_POINT('Origin',(-9.80186076935,-21.0742356128,11.1121328059));
#95741=CARTESIAN_POINT('Origin',(2.04268023839E-15,-21.0742356128,0.580061096523));
#95742=CARTESIAN_POINT('',(-10.7071554695,-20.7742356128,10.1903592597));
#95743=CARTESIAN_POINT('Origin',(-10.7071554695,-21.0742356128,10.1903592597));
#95744=CARTESIAN_POINT('Origin',(-5.42499920527E-16,-20.7742356128,0.580061096523));
#95745=CARTESIAN_POINT('Origin',(-10.1862176145,-21.0742356128,9.72278707155));
#95746=CARTESIAN_POINT('',(-10.8527076722,-20.7742356128,9.93677539585));
#95747=CARTESIAN_POINT('Origin',(-10.8527076722,-21.0742356128,9.93677539585));
#95748=CARTESIAN_POINT('Origin',(-10.1862176145,-20.7742356128,9.72278707155));
#95749=CARTESIAN_POINT('Origin',(-10.8795671881,-21.0742356128,9.85222376962));
#95750=CARTESIAN_POINT('',(-10.8795671881,-20.7742356128,9.85222376962));
#95751=CARTESIAN_POINT('Origin',(-10.8795671881,-21.0742356128,9.85222376962));
#95752=CARTESIAN_POINT('Origin',(-10.8795671881,-21.0742356128,9.85222376962));
#95753=CARTESIAN_POINT('Origin',(2.84607155346,-21.0742356128,5.53854202767));
#95754=CARTESIAN_POINT('Origin',(2.84607155346,-20.7742356128,5.53854202767));
#95755=CARTESIAN_POINT('Origin',(-11.3733704264,-21.0742356128,7.73136642019));
#95756=CARTESIAN_POINT('',(-11.3733704264,-20.7742356128,7.73136642019));
#95757=CARTESIAN_POINT('Origin',(-11.3733704264,-21.0742356128,7.73136642019));
#95758=CARTESIAN_POINT('Origin',(-11.3733704264,-21.0742356128,7.73136642019));
#95759=CARTESIAN_POINT('Origin',(2.84607155346,-21.0742356128,5.53854202767));
#95760=CARTESIAN_POINT('',(-11.4530804658,-20.7742356128,3.94629187045));
#95761=CARTESIAN_POINT('Origin',(-11.4530804658806,-21.0742356128,3.9462918704403));
#95762=CARTESIAN_POINT('Origin',(2.84607155346,-20.7742356128,5.53854202767));
#95763=CARTESIAN_POINT('Origin',(-11.4530804658,-21.0742356128,3.94629187045));
#95764=CARTESIAN_POINT('Origin',(-11.4530804658,-21.0742356128,3.94629187045));
#95765=CARTESIAN_POINT('Origin',(-8.95225019493,-21.0742356128,3.94629187045));
#95766=CARTESIAN_POINT('',(-8.10176909975,-20.7742356128,3.94629187045));
#95767=CARTESIAN_POINT('Origin',(-8.10176909975,-21.0742356128,3.94629187045));
#95768=CARTESIAN_POINT('',(-9.77742478279,-20.7742356128,3.94629187045));
#95769=CARTESIAN_POINT('Origin',(-8.10176909975,-21.0742356128,3.94629187045));
#95770=CARTESIAN_POINT('Origin',(-8.10176909975,-21.0742356128,3.94629187045));
#95771=CARTESIAN_POINT('Origin',(-0.00234331738835,-21.0742356128,3.08191746407));
#95772=CARTESIAN_POINT('',(-6.47088626226,-20.7742356128,8.03225010833));
#95773=CARTESIAN_POINT('Origin',(-6.47088626225866,-21.0742356128,8.0322501083283));
#95774=CARTESIAN_POINT('Origin',(-0.00234331738835,-20.7742356128,3.08191746407));
#95775=CARTESIAN_POINT('Origin',(-6.47088626226,-21.0742356128,8.03225010833));
#95776=CARTESIAN_POINT('Origin',(-6.47088626226,-21.0742356128,8.03225010833));
#95777=CARTESIAN_POINT('Origin',(-8.42643116047,-21.0742356128,9.84038429957));
#95778=CARTESIAN_POINT('',(-8.1363735158,-20.7742356128,9.57219145714));
#95779=CARTESIAN_POINT('Origin',(-9.00617217252,-21.0742356128,8.1200469301));
#95780=CARTESIAN_POINT('',(-10.5002881066,-20.7742356128,9.5015350813));
#95781=CARTESIAN_POINT('Origin',(-10.5002881066,-21.0742356128,9.5015350813));
#95782=CARTESIAN_POINT('',(-10.6899276473,-20.7742356128,9.67687942546));
#95783=CARTESIAN_POINT('Origin',(-10.9076228609,-21.0742356128,9.06099178277));
#95784=CARTESIAN_POINT('',(-10.4339531167,-20.7742356128,8.69270253038));
#95785=CARTESIAN_POINT('Origin',(-10.4339531167,-21.0742356128,8.69270253038));
#95786=CARTESIAN_POINT('Origin',(-10.9076228609,-20.7742356128,9.06099178277));
#95787=CARTESIAN_POINT('Origin',(5.59539391719E-15,-21.0742356128,0.580061096523));
#95788=CARTESIAN_POINT('',(-10.9433745451,-20.7742356128,7.99119341506));
#95789=CARTESIAN_POINT('Origin',(-10.9433745451,-21.0742356128,7.99119341506));
#95790=CARTESIAN_POINT('Origin',(8.04064645258E-16,-20.7742356128,0.580061096523));
#95791=CARTESIAN_POINT('Origin',(-11.4401704731,-21.0742356128,8.32763628675));
#95792=CARTESIAN_POINT('Origin',(-11.4401704731,-20.7742356128,8.32763628675));
#95793=CARTESIAN_POINT('Origin',(2.93915231795E-16,-20.7742356128,0.729452270839));
#98287=UNCERTAINTY_MEASURE_WITH_UNIT(LENGTH_MEASURE(0.01),#98303,
'DISTANCE_ACCURACY_VALUE',
'Maximum model space distance between geometric entities at asserted c
onnectivities');
#98290=UNCERTAINTY_MEASURE_WITH_UNIT(LENGTH_MEASURE(0.01),#98303,
'DISTANCE_ACCURACY_VALUE',
'Maximum model space distance between geometric entities at asserted c
onnectivities');
#98299=(
GEOMETRIC_REPRESENTATION_CONTEXT(3)
GLOBAL_UNCERTAINTY_ASSIGNED_CONTEXT((#98287))
GLOBAL_UNIT_ASSIGNED_CONTEXT((#98303,#98305,#98306))
REPRESENTATION_CONTEXT('','3D')
);
#98302=(
GEOMETRIC_REPRESENTATION_CONTEXT(3)
GLOBAL_UNCERTAINTY_ASSIGNED_CONTEXT((#98290))
GLOBAL_UNIT_ASSIGNED_CONTEXT((#98303,#98305,#98306))
REPRESENTATION_CONTEXT('','3D')
);
#98303=(
LENGTH_UNIT()
NAMED_UNIT(*)
SI_UNIT(.MILLI.,.METRE.)
);
#98305=(
NAMED_UNIT(*)
PLANE_ANGLE_UNIT()
SI_UNIT($,.RADIAN.)
);
#98306=(
NAMED_UNIT(*)
SI_UNIT($,.STERADIAN.)
SOLID_ANGLE_UNIT()
);
#98315=SHAPE_DEFINITION_REPRESENTATION(#98326,#98347);
#98326=PRODUCT_DEFINITION_SHAPE('',$,#98359);
#98347=SHAPE_REPRESENTATION('',(#36602),#98299);
#98350=PRODUCT_DEFINITION_CONTEXT('part definition',#98385,'design');
#98359=PRODUCT_DEFINITION('Disc Carrier','Disc Carrier',#98370,#98350);
#98370=PRODUCT_DEFINITION_FORMATION('',$,#98395);
#98385=APPLICATION_CONTEXT(
'Core Data for Automotive Mechanical Design Process');
#98386=PRODUCT_CONTEXT('part definition',#98385,'mechanical');
#98395=PRODUCT('Disc Carrier','Disc Carrier',$,(#98386));
#98399=PRESENTATION_STYLE_ASSIGNMENT((#98401));
#98401=SURFACE_STYLE_USAGE(.BOTH.,#98403);
#98403=SURFACE_SIDE_STYLE('',(#98405));
#98405=SURFACE_STYLE_FILL_AREA(#98407);
#98407=FILL_AREA_STYLE('Opaque(202,209,238)',(#98409));
#98409=FILL_AREA_STYLE_COLOUR('Opaque(202,209,238)',#98411);
#98411=COLOUR_RGB('Opaque(202,209,238)', 0.31764706, 0.68627451, 0.89019608);
ENDSEC;
END-ISO-10303-21;
